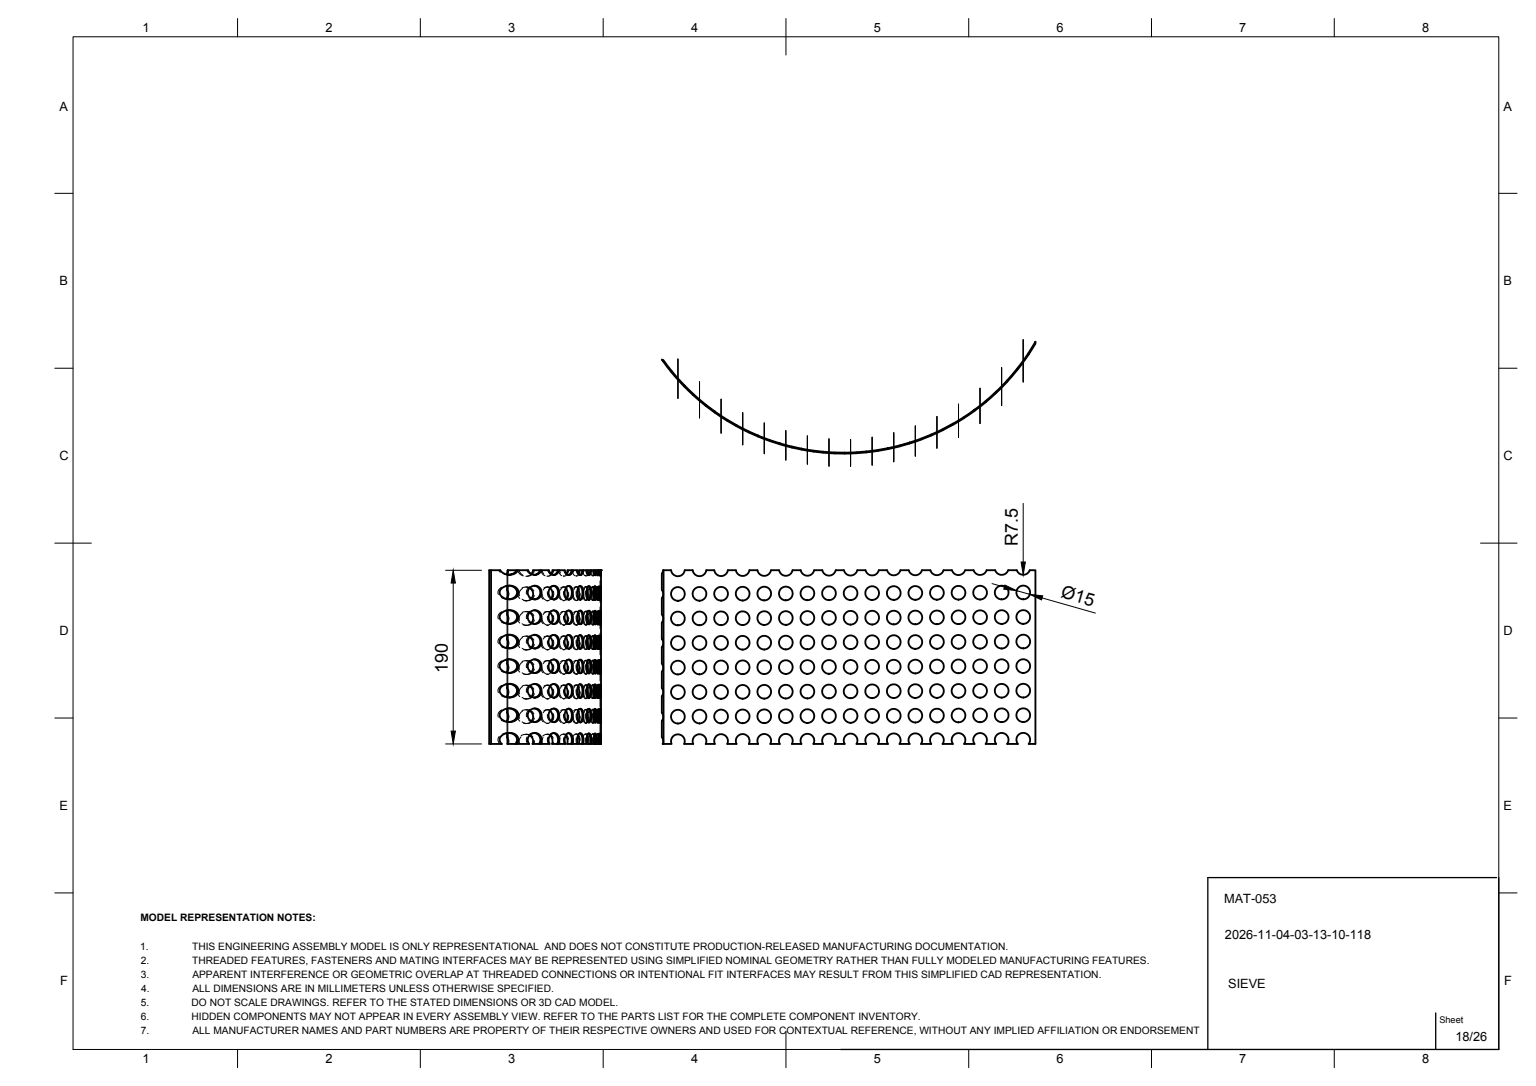
ISO-10303-21;
HEADER;
FILE_DESCRIPTION (('STEP AP214'),
    '1' );
FILE_NAME ('SIEVE.step',
    '2026-10-10T03:43:58',
    ( '' ),
    ( '' ),
    'SwSTEP 2.0',
    'SolidWorks 2026',
    '' );
FILE_SCHEMA (( 'AUTOMOTIVE_DESIGN' ));
ENDSEC;

DATA;
#1=CARTESIAN_POINT ( 'NONE',  ( 39.40195752203892710, -170.0000000000000000, -43.11981746542777927 ) ) ;
#3=EDGE_LOOP ( 'NONE', ( #61802, #31194, #2413, #55543 ) ) ;
#7=CARTESIAN_POINT ( 'NONE',  ( 157.4703587214989113, 58.92748579479261650, -51.12418429913766005 ) ) ;
#8=CARTESIAN_POINT ( 'NONE',  ( 66.29961816943398389, 13.45804302849872869, 30.55285179693984432 ) ) ;
#10=ADVANCED_FACE ( 'NONE', ( #11603 ), #16546, .F. ) ;
#11=CARTESIAN_POINT ( 'NONE',  ( -189.2739965869454579, 107.1373753350176656, -69.83507040438288982 ) ) ;
#12=EDGE_CURVE ( 'NONE', #54401, #54282, #16885, .T. ) ;
#15=CARTESIAN_POINT ( 'NONE',  ( -95.04120270830171080, 29.25306318840327791, 66.89222559579708616 ) ) ;
#20=CARTESIAN_POINT ( 'NONE',  ( -124.1095621208148572, 46.52671329146387080, 18.61778521462535352 ) ) ;
#21=AXIS2_PLACEMENT_3D ( 'NONE', #6201, #49094, #933 ) ;
#22=CARTESIAN_POINT ( 'NONE',  ( -173.9548930713590380, 88.06040582145359963, 57.70099677511350933 ) ) ;
#23=CARTESIAN_POINT ( 'NONE',  ( 15.78827728214693416, 6.500811158483328356, 18.17015708224157322 ) ) ;
#24=ORIENTED_EDGE ( 'NONE', *, *, #58760, .T. ) ;
#25=CARTESIAN_POINT ( 'NONE',  ( -24.85653282846401879, 8.603185326828743484, 94.99999999999866418 ) ) ;
#26=CARTESIAN_POINT ( 'NONE',  ( 156.5909039492010209, 56.96742803863246962, 44.40946747225338953 ) ) ;
#27=CARTESIAN_POINT ( 'NONE',  ( 70.12389542974193546, 15.47520081968151651, 34.86987470614429441 ) ) ;
#30=DIRECTION ( 'NONE',  ( -0.000000000000000000, 1.000000000000000000, -0.000000000000000000 ) ) ;
#31=CARTESIAN_POINT ( 'NONE',  ( -23.93880457192868860, 8.479983864459173404, 37.95612845895288956 ) ) ;
#32=CARTESIAN_POINT ( 'NONE',  ( -142.0084862216822614, 59.34995487985342066, -68.57895708802404044 ) ) ;
#33=ORIENTED_EDGE ( 'NONE', *, *, #68760, .T. ) ;
#35=FACE_BOUND ( 'NONE', #6574, .T. ) ;
#37=CARTESIAN_POINT ( 'NONE',  ( -180.0154536325057677, 96.73346874014741559, 68.13326579958136620 ) ) ;
#38=CARTESIAN_POINT ( 'NONE',  ( 110.2429982417149432, 28.88204397445230853, -89.61153874658103291 ) ) ;
#39=CARTESIAN_POINT ( 'NONE',  ( 133.8566784816069344, 41.42467568809808398, 29.51034083899533300 ) ) ;
#43=CARTESIAN_POINT ( 'NONE',  ( -78.66644367742111399, 22.32174330031318732, -88.80455181264524356 ) ) ;
#44=CARTESIAN_POINT ( 'NONE',  ( 70.02892116572940040, 14.40944430928136377, 13.13782541409767646 ) ) ;
#45=CARTESIAN_POINT ( 'NONE',  ( 161.7048274740120917, 61.01946783654758377, 3.857278696179094801 ) ) ;
#46=CARTESIAN_POINT ( 'NONE',  ( 92.21252738308859875, 22.47457138983956426, -21.50906452630309929 ) ) ;
#48=EDGE_CURVE ( 'NONE', #37583, #44986, #40434, .T. ) ;
#53=CARTESIAN_POINT ( 'NONE',  ( -125.8938041572051105, 46.49392987655495091, 45.61994787315711619 ) ) ;
#54=CARTESIAN_POINT ( 'NONE',  ( 114.5134543485688710, 32.02763527597250715, 84.62599922377962969 ) ) ;
#55=CARTESIAN_POINT ( 'NONE',  ( 39.40195752203891999, 9.424259417798147354, -8.775266874964067654 ) ) ;
#56=CARTESIAN_POINT ( 'NONE',  ( 66.73594759725092729, 13.56641407806656829, -9.859353299932527293 ) ) ;
#58=CARTESIAN_POINT ( 'NONE',  ( 135.6793972494602656, 43.71805072851429941, -50.81300272974607424 ) ) ;
#60=CARTESIAN_POINT ( 'NONE',  ( 208.3163574534978295, 113.2160455531247152, -90.93580564839912483 ) ) ;
#62=CARTESIAN_POINT ( 'NONE',  ( -125.8938041572051389, -170.0000000000000000, -96.10280507916131398 ) ) ;
#65=EDGE_CURVE ( 'NONE', #33282, #48266, #62999, .T. ) ;
#66=CARTESIAN_POINT ( 'NONE',  ( 35.66087318222937341, 8.964867769223225480, 57.73931627539139555 ) ) ;
#67=VECTOR ( 'NONE', #58761, 1000.000000000000000 ) ;
#68=CARTESIAN_POINT ( 'NONE',  ( 178.1321887506117889, 77.08201292995904907, 83.59636689041089141 ) ) ;
#69=DIRECTION ( 'NONE',  ( -0.000000000000000000, 1.000000000000000000, -0.000000000000000000 ) ) ;
#70=EDGE_CURVE ( 'NONE', #25573, #51909, #66497, .T. ) ;
#71=B_SPLINE_CURVE_WITH_KNOTS ( 'NONE', 3,
 ( #62149, #40352, #67112, #40690, #61801, #51606, #19236, #61465, #13288, #2379, #13619, #2725 ),
 .UNSPECIFIED., .F., .F.,
 ( 4, 2, 2, 2, 2, 4 ),
 ( 0.01013073868447747147, 0.01266158667236432465, 0.01519243466025117784, 0.01645785865419460356, 0.01772328264813802928, 0.02025413063602488073 ),
 .UNSPECIFIED. ) ;
#75=CARTESIAN_POINT ( 'NONE',  ( 70.16127872101215246, 15.48516972826856097, -94.59315289484993627 ) ) ;
#78=CARTESIAN_POINT ( 'NONE',  ( 188.5653887627528036, 88.01608521313129074, -17.48984807395640573 ) ) ;
#79=CARTESIAN_POINT ( 'NONE',  ( -82.93267503967653909, 23.99263498936122829, -9.597822780125905950 ) ) ;
#82=CARTESIAN_POINT ( 'NONE',  ( 157.4703587214989398, 58.92748579479258808, 17.56491688178971700 ) ) ;
#83=LINE ( 'NONE', #53188, #15134 ) ;
#84=CYLINDRICAL_SURFACE ( 'NONE', #8226, 7.500000000000020428 ) ;
#85=CARTESIAN_POINT ( 'NONE',  ( 164.6598737201887275, 64.78038692612516058, 61.54778376556991759 ) ) ;
#87=CARTESIAN_POINT ( 'NONE',  ( -190.6985136298601731, 109.1272424661242582, -95.00000000000133582 ) ) ;
#88=CARTESIAN_POINT ( 'NONE',  ( 91.11019107624156277, 22.06959540317787827, -37.30231510556647123 ) ) ;
#89=CARTESIAN_POINT ( 'NONE',  ( 152.8373718734504791, 55.38925997611393370, 69.67201452546140672 ) ) ;
#90=FACE_OUTER_BOUND ( 'NONE', #51593, .T. ) ;
#92=CARTESIAN_POINT ( 'NONE',  ( -10.98306470837134796, 8.126405184847016017, 84.49408135793621000 ) ) ;
#101=CARTESIAN_POINT ( 'NONE',  ( 88.52077179907878701, 21.14145351760140557, -62.90458105059150284 ) ) ;
#103=CARTESIAN_POINT ( 'NONE',  ( -55.05276343752909440, 14.68156374112638929, -77.06087458892358200 ) ) ;
#105=CARTESIAN_POINT ( 'NONE',  ( 32.29989959354725926, 7.591763852038291738, -13.85219865116375715 ) ) ;
#106=CARTESIAN_POINT ( 'NONE',  ( 179.4227152810058215, 78.36166152262364903, -51.05095273083168905 ) ) ;
#107=CARTESIAN_POINT ( 'NONE',  ( 163.7460705099150573, 62.69983247170010543, 94.71987145728411406 ) ) ;
#108=CARTESIAN_POINT ( 'NONE',  ( 93.85846834761630930, 22.01563781856521018, 35.19885710929750644 ) ) ;
#110=ORIENTED_EDGE ( 'NONE', *, *, #20958, .T. ) ;
#113=CARTESIAN_POINT ( 'NONE',  ( -52.68206656346369954, 15.09776187114412593, -35.59673745022761437 ) ) ;
#114=CARTESIAN_POINT ( 'NONE',  ( -78.66644367742111399, 23.39876645725287219, 30.41820113967310490 ) ) ;
#115=CARTESIAN_POINT ( 'NONE',  ( 8.683910719548897816, 7.383368463746306176, 35.09835667283063998 ) ) ;
#119=ORIENTED_EDGE ( 'NONE', *, *, #42370, .F. ) ;
#122=CARTESIAN_POINT ( 'NONE',  ( -8.314575874103555364, 6.922894809783093351, -23.57352014148017361 ) ) ;
#123=CARTESIAN_POINT ( 'NONE',  ( -50.51700111023804851, 13.51182830536852997, 43.81040306015482599 ) ) ;
#125=DIRECTION ( 'NONE',  ( 0.000000000000000000, 0.000000000000000000, 1.000000000000000000 ) ) ;
#127=CARTESIAN_POINT ( 'NONE',  ( -38.16652041892307778, 11.81761816422915068, 61.20925241452948740 ) ) ;
#129=CARTESIAN_POINT ( 'NONE',  ( -13.47517652744366856, 8.334971000693553123, -11.11675483260547104 ) ) ;
#130=CARTESIAN_POINT ( 'NONE',  ( 150.0973882686025433, 52.13852366454154463, -69.06737236800162805 ) ) ;
#131=CARTESIAN_POINT ( 'NONE',  ( 15.78827728214693416, 6.500811158483328356, -8.674393508222097537 ) ) ;
#134=CARTESIAN_POINT ( 'NONE',  ( -154.7998111145352595, 68.80117179139330119, -47.64861779563037203 ) ) ;
#136=EDGE_LOOP ( 'NONE', ( #56580, #33322, #40120, #29529 ) ) ;
#137=CARTESIAN_POINT ( 'NONE',  ( 69.49112875363887554, 15.30845942322122433, -20.16820370593556433 ) ) ;
#138=EDGE_CURVE ( 'NONE', #47203, #54495, #17035, .T. ) ;
#139=CARTESIAN_POINT ( 'NONE',  ( -82.93126516400695891, 25.07709093823493873, -48.78959211302295529 ) ) ;
#140=DIRECTION ( 'NONE',  ( 0.000000000000000000, 0.000000000000000000, 1.000000000000000000 ) ) ;
#141=CARTESIAN_POINT ( 'NONE',  ( -156.9900125991010498, 72.16580261738670288, 10.78960814776965549 ) ) ;
#142=CARTESIAN_POINT ( 'NONE',  ( 187.2465631085773907, 85.06582225041681511, -39.42042871992538267 ) ) ;
#144=CARTESIAN_POINT ( 'NONE',  ( -156.4614183966801022, 71.67647641794694380, 89.09562039624624674 ) ) ;
#145=VERTEX_POINT ( 'NONE', #21389 ) ;
#147=EDGE_LOOP ( 'NONE', ( #11378, #55449, #7164, #22820 ) ) ;
#148=CARTESIAN_POINT ( 'NONE',  ( -156.0209085498132140, 71.27066046086522988, -19.22534495811094146 ) ) ;
#149=CARTESIAN_POINT ( 'NONE',  ( 87.02964419696034781, 20.62171628682589386, -89.51066537983909654 ) ) ;
#153=CARTESIAN_POINT ( 'NONE',  ( -33.83558513595455253, 9.996963989836508802, 71.67202419627825805 ) ) ;
#154=CARTESIAN_POINT ( 'NONE',  ( -150.3791492925491013, 64.92185203933371440, -22.93029560069632211 ) ) ;
#156=CARTESIAN_POINT ( 'NONE',  ( 187.0788993276711665, 86.37277723143233743, 59.13935664661273250 ) ) ;
#157=CARTESIAN_POINT ( 'NONE',  ( -155.1302201283146758, 69.09929365814132041, 70.03478143350771745 ) ) ;
#159=CARTESIAN_POINT ( 'NONE',  ( 16.28382582968306380, 7.523443033994204221, 18.17015708224156612 ) ) ;
#160=CARTESIAN_POINT ( 'NONE',  ( 104.7147873368644753, 26.40702926859708199, 15.35902160271893813 ) ) ;
#161=CARTESIAN_POINT ( 'NONE',  ( -124.9927180788553756, 45.90286323198618845, 18.73480619198342367 ) ) ;
#163=CARTESIAN_POINT ( 'NONE',  ( 21.25987915030395925, 6.737472588634914494, 59.22395766586208055 ) ) ;
#165=CARTESIAN_POINT ( 'NONE',  ( 8.336882341125875229, 6.376438415325264231, -70.84698747820850429 ) ) ;
#168=VERTEX_POINT ( 'NONE', #37218 ) ;
#173=CARTESIAN_POINT ( 'NONE',  ( 218.0000000000000000, 0.000000000000000000, 0.000000000000000000 ) ) ;
#174=CARTESIAN_POINT ( 'NONE',  ( 44.34263167748003553, 9.103379693481556956, -75.62813062877941661 ) ) ;
#176=EDGE_LOOP ( 'NONE', ( #13726, #7536, #23044, #10848 ) ) ;
#177=ORIENTED_EDGE ( 'NONE', *, *, #64499, .T. ) ;
#178=CARTESIAN_POINT ( 'NONE',  ( -25.48237668717799309, 8.689083390666777262, -11.38912287515594812 ) ) ;
#179=CARTESIAN_POINT ( 'NONE',  ( 174.1688711713896964, 71.88855623114105242, 93.40745146404465515 ) ) ;
#182=CARTESIAN_POINT ( 'NONE',  ( 116.0773578185793582, 31.67580513411752463, 59.21665166914974776 ) ) ;
#184=CARTESIAN_POINT ( 'NONE',  ( 115.0485321076020568, 32.28990710985444679, 69.73487632334627051 ) ) ;
#186=CARTESIAN_POINT ( 'NONE',  ( 140.2058232509808704, 46.59155168125935376, 67.87841396662895477 ) ) ;
#188=CARTESIAN_POINT ( 'NONE',  ( -98.46684543088103680, 30.88557736720387936, 44.48182062113936297 ) ) ;
#189=CARTESIAN_POINT ( 'NONE',  ( 88.98408042523108463, 20.23787745328938570, -50.44636354873872364 ) ) ;
#191=ORIENTED_EDGE ( 'NONE', *, *, #28368, .T. ) ;
#197=CARTESIAN_POINT ( 'NONE',  ( -165.7690020878297616, 80.74028011998674970, -70.56799682258439077 ) ) ;
#198=CARTESIAN_POINT ( 'NONE',  ( -142.0251973982164202, 58.08401473564112649, -42.89990999809938188 ) ) ;
#199=ORIENTED_EDGE ( 'NONE', *, *, #29609, .T. ) ;
#208=CARTESIAN_POINT ( 'NONE',  ( 79.19345177405116942, 17.01649702043280143, -15.46643930101046038 ) ) ;
#209=CARTESIAN_POINT ( 'NONE',  ( 93.71772995179813392, 21.96265635001558181, -67.70285364061378175 ) ) ;
#210=CARTESIAN_POINT ( 'NONE',  ( 60.43099056502398980, 12.08801636090767850, -89.86627097950946563 ) ) ;
#212=CARTESIAN_POINT ( 'NONE',  ( -98.69283175933881580, 30.99524616306738878, 4.570732717346438712 ) ) ;
#213=CARTESIAN_POINT ( 'NONE',  ( -95.63568360745009045, 29.53168204475774417, -72.84711776369148595 ) ) ;
#217=ADVANCED_FACE ( 'NONE', ( #3847 ), #69303, .F. ) ;
#218=CARTESIAN_POINT ( 'NONE',  ( 188.2133404574783242, 86.12414067617878288, -68.22339036842659254 ) ) ;
#219=VECTOR ( 'NONE', #12666, 1000.000000000000000 ) ;
#224=CARTESIAN_POINT ( 'NONE',  ( 79.23200707685336397, 17.02828389812517429, 38.47447533467553171 ) ) ;
#226=CARTESIAN_POINT ( 'NONE',  ( -124.1007047332777944, 46.52282960291164926, 30.82329275154649295 ) ) ;
#227=CARTESIAN_POINT ( 'NONE',  ( 211.1200456646897123, 115.5868795682033436, 67.43584021203363932 ) ) ;
#231=CARTESIAN_POINT ( 'NONE',  ( -14.76369756425703983, 7.442560416198673146, -40.03899903455366882 ) ) ;
#233=CARTESIAN_POINT ( 'NONE',  ( 89.87840278991589571, 21.62393877508911899, 57.29260026085291457 ) ) ;
#235=CARTESIAN_POINT ( 'NONE',  ( 150.0433793199863146, 52.09973307442953683, -17.85989976896762244 ) ) ;
#236=CARTESIAN_POINT ( 'NONE',  ( 31.96192885395475614, 8.569232728322420556, 11.54728592230744688 ) ) ;
#237=CARTESIAN_POINT ( 'NONE',  ( -94.77890319529970498, 30.24118571794803145, -69.85920485586603945 ) ) ;
#243=CARTESIAN_POINT ( 'NONE',  ( 60.63380853769237433, 13.16344960520422092, 57.04161213523420315 ) ) ;
#245=CARTESIAN_POINT ( 'NONE',  ( -9.524904342798460988, 8.016391612076530393, 3.461975196507860453 ) ) ;
#246=B_SPLINE_CURVE_WITH_KNOTS ( 'NONE', 3,
 ( #24990, #25339, #47115, #47446, #36574, #58023, #9495, #14429, #20379, #68579, #26018, #52401, #25686, #36915, #46776, #68907, #62260, #42187, #63654, #14763, #4219, #36227, #52729, #30264, #15462, #41848, #9150, #30605, #9841, #46080, #14077, #8811, #4554, #29912, #62955, #67550, #35539, #52058, #68246, #56993, #8460, #20051, #41504, #51371, #3188, #24647, #19349, #57685, #51713, #46422 ),
 .UNSPECIFIED., .F., .F.,
 ( 4, 2, 2, 2, 2, 2, 2, 2, 2, 2, 2, 2, 2, 2, 2, 2, 2, 2, 2, 2, 2, 2, 2, 2, 4 ),
 ( 0.02688458561150007531, 0.02770990876165290578, 0.02853523191180573973, 0.03018587821211139027, 0.03183652451241704429, 0.03266184766256987476, 0.03348717081272270524, 0.03513781711302831068, 0.03678846341333391612, 0.03761378656348669802, 0.03843910971363948686, 0.03926443286379226877, 0.04008975601394505761, 0.04174040231425062836, 0.04256572546440341026, 0.04339104861455619216, 0.04421637176470897407, 0.04504169491486175597, 0.04586701806501453788, 0.04669234121516731978, 0.04834298751547294604, 0.04916831066562572794, 0.04999363381577851678, 0.05164428011608407365, 0.05329492641638964440 ),
 .UNSPECIFIED. ) ;
#248=CARTESIAN_POINT ( 'NONE',  ( -3.857727530059799737, 6.665032499723453796, 43.98489318319101926 ) ) ;
#250=CARTESIAN_POINT ( 'NONE',  ( 92.81046075878417412, 22.69711000191779959, 86.64015653787805604 ) ) ;
#256=CARTESIAN_POINT ( 'NONE',  ( -104.1393288135077455, 34.86912007524090029, 72.14469141808412189 ) ) ;
#258=CARTESIAN_POINT ( 'NONE',  ( -131.6253556217205016, 51.61436399519948282, -47.27706506024894395 ) ) ;
#262=B_SPLINE_CURVE_WITH_KNOTS ( 'NONE', 3,
 ( #59638, #61313, #13475, #23684, #67303, #64945, #7519, #45827, #34603, #2920, #19089, #8197, #59303, #16738, #39855, #45475, #23348, #40208, #56375, #13139, #2235, #38197, #11115, #12783, #11452, #571, #34245, #7855, #60962, #44791, #54360, #29302, #28970, #1895, #29646, #32580, #50755, #2576 ),
 .UNSPECIFIED., .F., .F.,
 ( 4, 2, 2, 2, 2, 2, 2, 2, 2, 2, 2, 2, 2, 2, 2, 2, 2, 2, 4 ),
 ( 1.430489624538199204E-17, 0.003908178031105532212, 0.005862267046658249312, 0.007816356062210967279, 0.009770445077763688715, 0.01172453409331640842, 0.01270157860109274485, 0.01367862310886907781, 0.01465566761664541424, 0.01563271212442174721, 0.01660975663219808884, 0.01758680113997443048, 0.01954089015552709294, 0.02051793466330344151, 0.02149497917107979009, 0.02344906818663248377, 0.02540315720218518786, 0.02735724621773788501, 0.03126542424884325155 ),
 .UNSPECIFIED. ) ;
#263=CARTESIAN_POINT ( 'NONE',  ( -1.088326810997878091, 6.545818265928947888, -19.40564166976581006 ) ) ;
#266=CARTESIAN_POINT ( 'NONE',  ( -153.9421172888672231, 68.03407102037994036, 85.85448269280857403 ) ) ;
#268=CARTESIAN_POINT ( 'NONE',  ( 141.3445468829085030, 46.13338528906589886, 37.51412908544414648 ) ) ;
#271=CARTESIAN_POINT ( 'NONE',  ( 82.73618382051373032, 19.18661415186669217, 16.78260538844248728 ) ) ;
#272=CARTESIAN_POINT ( 'NONE',  ( 164.4761273435911733, 64.62485394454745347, 7.335242511255203546 ) ) ;
#274=AXIS2_PLACEMENT_3D ( 'NONE', #4193, #20028, #68878 ) ;
#275=VERTEX_POINT ( 'NONE', #57999 ) ;
#276=EDGE_CURVE ( 'NONE', #33643, #59523, #9303, .T. ) ;
#277=CARTESIAN_POINT ( 'NONE',  ( 174.9099402067542997, 73.96774984027638311, 67.91937322613915740 ) ) ;
#279=CARTESIAN_POINT ( 'NONE',  ( -104.5730787903383003, 33.96058035148152499, -35.35797728948608665 ) ) ;
#281=CARTESIAN_POINT ( 'NONE',  ( 150.4542242713869200, 53.63744268572192198, 12.72894179764149847 ) ) ;
#282=ORIENTED_EDGE ( 'NONE', *, *, #4760, .T. ) ;
#283=CARTESIAN_POINT ( 'NONE',  ( 157.4703587214989113, 57.65129005721576760, 29.40946747225336466 ) ) ;
#285=CYLINDRICAL_SURFACE ( 'NONE', #42881, 7.500000000000020428 ) ;
#286=ORIENTED_EDGE ( 'NONE', *, *, #5924, .T. ) ;
#292=CARTESIAN_POINT ( 'NONE',  ( -37.79823708645147917, 10.72197716414928870, -73.64561661794576253 ) ) ;
#302=DIRECTION ( 'NONE',  ( -0.000000000000000000, 1.000000000000000000, -0.000000000000000000 ) ) ;
#303=CARTESIAN_POINT ( 'NONE',  ( 70.49702515974807682, 14.53327724265703402, 91.86127284075526234 ) ) ;
#307=CYLINDRICAL_SURFACE ( 'NONE', #24291, 7.500000000000013323 ) ;
#311=AXIS2_PLACEMENT_3D ( 'NONE', #60560, #44374, #50365 ) ;
#312=CARTESIAN_POINT ( 'NONE',  ( 211.5066273949820186, 116.1727691518062073, -73.86407362358771422 ) ) ;
#313=B_SPLINE_CURVE_WITH_KNOTS ( 'NONE', 3,
 ( #22788, #6611, #12241, #1333, #32645, #43534, #50221, #60425, #55133, #1685, #44592, #50913, #45283, #9047, #13622, #19590, #7670, #2728, #34407, #66764, #61804, #18557, #55849, #61471, #62513, #3420, #35784, #41053, #18214, #24879, #2383, #14325, #29453, #29115, #40694, #57233, #40009, #13291, #30495, #29808, #39665, #46316, #50565, #44937 ),
 .UNSPECIFIED., .F., .F.,
 ( 4, 2, 2, 2, 2, 2, 2, 2, 2, 2, 2, 2, 2, 2, 2, 2, 2, 2, 2, 2, 2, 4 ),
 ( 0.02895403260893131964, 0.03071603688922221187, 0.03247804116951310410, 0.03424004544980399634, 0.03600204973009488857, 0.03776405401038577386, 0.03864505615053119569, 0.03952605829067662446, 0.04040706043082205323, 0.04128806257096747506, 0.04216906471111290383, 0.04305006685125832566, 0.04393106899140375443, 0.04481207113154918320, 0.04569307327169461197, 0.04657407541184004074, 0.04745507755198546257, 0.04833607969213089134, 0.05009808397242175582, 0.05186008825271262723, 0.05362209253300349171, 0.05714610109358524842 ),
 .UNSPECIFIED. ) ;
#316=CARTESIAN_POINT ( 'NONE',  ( 63.01563776193091826, -170.0000000000000000, -89.40979201309708913 ) ) ;
#317=CARTESIAN_POINT ( 'NONE',  ( -124.1095621208148714, 46.52671329146387791, 72.30688639555273767 ) ) ;
#318=CARTESIAN_POINT ( 'NONE',  ( 22.62427395637551086, 7.823784829753564374, 34.41962451814575275 ) ) ;
#326=FACE_OUTER_BOUND ( 'NONE', #64859, .T. ) ;
#328=ORIENTED_EDGE ( 'NONE', *, *, #4703, .T. ) ;
#331=CARTESIAN_POINT ( 'NONE',  ( 46.85361596800672146, 10.51535167202354693, 38.39853853478529544 ) ) ;
#332=CARTESIAN_POINT ( 'NONE',  ( -27.70562707895080123, 9.007984652865424380, 58.03756985863584106 ) ) ;
#333=CARTESIAN_POINT ( 'NONE',  ( -142.3393481102175713, 58.33014244976924090, 9.152932767281312110 ) ) ;
#335=ORIENTED_EDGE ( 'NONE', *, *, #3794, .F. ) ;
#336=CARTESIAN_POINT ( 'NONE',  ( -127.6881387055492354, 48.89937523111242257, 30.83417093567260636 ) ) ;
#340=CARTESIAN_POINT ( 'NONE',  ( 55.61382797299289393, 11.07686102552912644, 62.92265474384031876 ) ) ;
#342=CARTESIAN_POINT ( 'NONE',  ( -29.96307832726302678, 10.37242130382201921, -89.14992242554669133 ) ) ;
#343=CARTESIAN_POINT ( 'NONE',  ( -188.8754233303960746, 108.3048424661242137, -95.00000000000133582 ) ) ;
#347=VERTEX_POINT ( 'NONE', #65712 ) ;
#350=VECTOR ( 'NONE', #31052, 1000.000000000000000 ) ;
#353=CARTESIAN_POINT ( 'NONE',  ( 70.26722489419890394, 14.47234958177329567, 35.33543539248424281 ) ) ;
#355=ORIENTED_EDGE ( 'NONE', *, *, #33274, .T. ) ;
#358=CARTESIAN_POINT ( 'NONE',  ( 80.30232379693107703, 17.35837133860831472, 6.332652209273762267 ) ) ;
#361=CARTESIAN_POINT ( 'NONE',  ( -71.97434903038468690, 19.88430675376529067, 34.49547489334918993 ) ) ;
#362=ORIENTED_EDGE ( 'NONE', *, *, #55841, .F. ) ;
#364=VECTOR ( 'NONE', #18440, 1000.000000000000000 ) ;
#368=CARTESIAN_POINT ( 'NONE',  ( -179.5178913137217194, 94.54206947403389449, 69.12039320224292283 ) ) ;
#370=ORIENTED_EDGE ( 'NONE', *, *, #14642, .F. ) ;
#374=DIRECTION ( 'NONE',  ( -0.000000000000000000, 1.000000000000000000, -0.000000000000000000 ) ) ;
#375=CARTESIAN_POINT ( 'NONE',  ( 150.9184679586219033, 52.73111408630721542, 40.56872817287094790 ) ) ;
#376=CARTESIAN_POINT ( 'NONE',  ( 68.63585058221465829, 15.08566240483130727, 32.32217050974968942 ) ) ;
#381=CARTESIAN_POINT ( 'NONE',  ( -23.95096213915836358, 8.481591526885939203, 38.20520003450658209 ) ) ;
#382=CARTESIAN_POINT ( 'NONE',  ( -144.7530445311634537, 61.54314312182906122, -74.96293479194935117 ) ) ;
#384=FACE_BOUND ( 'NONE', #4499, .T. ) ;
#385=CARTESIAN_POINT ( 'NONE',  ( -2.190131154568200511, 6.589492063460817839, -74.71788358249716566 ) ) ;
#386=CARTESIAN_POINT ( 'NONE',  ( -179.8926034784145997, 96.58272071140105197, 61.93007157060646506 ) ) ;
#388=CARTESIAN_POINT ( 'NONE',  ( -118.9668643994983483, 43.27909474462860828, -39.52642719331304022 ) ) ;
#389=CARTESIAN_POINT ( 'NONE',  ( -85.66184035008926401, 26.20110535976566268, 13.79000864225666589 ) ) ;
#392=CARTESIAN_POINT ( 'NONE',  ( -5.888165822225391643, 7.780336669456525023, -8.823856489658712832 ) ) ;
#393=CARTESIAN_POINT ( 'NONE',  ( 67.55134213333077753, 13.77030723107740506, 4.475137186144926282 ) ) ;
#394=CARTESIAN_POINT ( 'NONE',  ( 159.6593397521790791, 59.37286298965126718, 2.877594456964315039 ) ) ;
#395=CARTESIAN_POINT ( 'NONE',  ( 39.81822037269075309, 9.478622457786777034, -89.30891864635511013 ) ) ;
#398=CARTESIAN_POINT ( 'NONE',  ( -38.54712373114178092, 11.89174538567466932, 8.428869490921766072 ) ) ;
#399=ORIENTED_EDGE ( 'NONE', *, *, #56528, .T. ) ;
#402=CARTESIAN_POINT ( 'NONE',  ( 85.67165909753201447, 20.15791549876375655, -62.71191053415395089 ) ) ;
#404=CARTESIAN_POINT ( 'NONE',  ( 110.9260829236403936, 30.30898941444543837, 83.30420403083246583 ) ) ;
#405=CARTESIAN_POINT ( 'NONE',  ( -142.0084862216822330, 59.34995487985343487, 65.64379586429438973 ) ) ;
#406=CARTESIAN_POINT ( 'NONE',  ( 70.25990036603482736, 14.47042233282419765, -14.41847716369608001 ) ) ;
#409=CARTESIAN_POINT ( 'NONE',  ( -31.43908319763710679, 10.61114334766715928, -35.31719736520183517 ) ) ;
#410=CARTESIAN_POINT ( 'NONE',  ( -53.14657859411972396, 15.21831473227210196, -62.30310801584961666 ) ) ;
#413=EDGE_CURVE ( 'NONE', #65743, #4867, #71, .T. ) ;
#414=CARTESIAN_POINT ( 'NONE',  ( -118.4106078162223668, 42.93830006159888768, -14.99940221450364319 ) ) ;
#415=ORIENTED_EDGE ( 'NONE', *, *, #36605, .F. ) ;
#419=CARTESIAN_POINT ( 'NONE',  ( 33.31166872005967150, 8.707041209322234465, 59.87445300413067173 ) ) ;
#420=DIRECTION ( 'NONE',  ( -0.8118923937861950435, -0.5838071093367415143, 0.000000000000000000 ) ) ;
#422=CARTESIAN_POINT ( 'NONE',  ( -172.3038663181180823, 87.72015621195184565, -7.867406574286301080 ) ) ;
#427=CARTESIAN_POINT ( 'NONE',  ( 187.2296622856351860, 86.53808614709454616, -21.18754879403664404 ) ) ;
#428=CARTESIAN_POINT ( 'NONE',  ( 212.1669304543882788, 119.0398299474539243, 9.162465270872496959 ) ) ;
#432=CARTESIAN_POINT ( 'NONE',  ( -149.5074843970971301, 64.17983161892345834, -76.65738112195568021 ) ) ;
#439=CARTESIAN_POINT ( 'NONE',  ( -47.94536219817735656, 13.92422159065987408, 62.21613247434213179 ) ) ;
#441=CYLINDRICAL_SURFACE ( 'NONE', #8272, 7.500000000000013323 ) ;
#442=DIRECTION ( 'NONE',  ( -0.000000000000000000, 1.000000000000000000, -0.000000000000000000 ) ) ;
#443=B_SPLINE_CURVE_WITH_KNOTS ( 'NONE', 3,
 ( #41840, #54634, #27027, #15107, #63647, #41496, #62947, #36907, #10161, #9488, #16130, #30946, #14755, #4211, #4546, #53400, #25676, #4886, #47438, #68897, #47107, #68570, #47789, #42521, #63298, #15455, #36566, #20724, #31293, #26353, #52719, #58345, #5235, #53749, #63976, #9834, #21078, #15790, #26011, #42179, #37233, #69251, #58684 ),
 .UNSPECIFIED., .F., .F.,
 ( 4, 2, 2, 2, 2, 2, 2, 2, 2, 2, 2, 1, 2, 2, 2, 2, 2, 2, 2, 2, 2, 4 ),
 ( 0.02515559250233022348, 0.02674001423437969566, 0.02753222510040442828, 0.02832443596642916436, 0.02990885769847856715, 0.03149327943052796647, 0.03307770116257736925, 0.03386991202860207412, 0.03466212289462677898, 0.03624654462667613319, 0.03703875549270080336, 0.03783096635872546659, 0.03862317722475013676, 0.03941538809077479999, 0.04099980982282412645, 0.04258423155487345985, 0.04337644242089812308, 0.04416865328692278631, 0.04575307501897205031, 0.04733749675102130738, 0.04892191848307056445, 0.05050634021511982846 ),
 .UNSPECIFIED. ) ;
#445=CARTESIAN_POINT ( 'NONE',  ( 62.53328835682435738, 12.56090025569836932, 2.968410348757586803 ) ) ;
#446=CARTESIAN_POINT ( 'NONE',  ( -58.10608953386396536, 15.52134062643864176, 57.80724698423686903 ) ) ;
#448=EDGE_LOOP ( 'NONE', ( #53193, #25137, #33362, #38103 ) ) ;
#449=EDGE_CURVE ( 'NONE', #11991, #8386, #8441, .T. ) ;
#453=CARTESIAN_POINT ( 'NONE',  ( 91.11019107624153435, 22.06959540317787116, -64.14686569603014732 ) ) ;
#457=CARTESIAN_POINT ( 'NONE',  ( 35.44781468922820977, 7.928097401423690016, -22.65291149958800432 ) ) ;
#458=CARTESIAN_POINT ( 'NONE',  ( 173.8576514579035290, 72.97529922124003576, -41.69686196060180094 ) ) ;
#459=CARTESIAN_POINT ( 'NONE',  ( 158.7623625177564008, 58.66148101564576223, 83.18577911345145992 ) ) ;
#464=ORIENTED_EDGE ( 'NONE', *, *, #60521, .F. ) ;
#466=CARTESIAN_POINT ( 'NONE',  ( -51.34542473642584071, 14.75635007918829800, -49.24053308027907860 ) ) ;
#470=CARTESIAN_POINT ( 'NONE',  ( 13.83281508467570653, 7.452090093180185448, 44.77217603759554265 ) ) ;
#479=CARTESIAN_POINT ( 'NONE',  ( -14.32120159453990027, 7.401444311907543039, -19.83056408198577003 ) ) ;
#480=CARTESIAN_POINT ( 'NONE',  ( -49.11825192196926082, 13.17012322555986970, 42.42977472503392988 ) ) ;
#484=CARTESIAN_POINT ( 'NONE',  ( -31.93169728792083362, 10.69234447276976852, 72.06100499665291181 ) ) ;
#485=CARTESIAN_POINT ( 'NONE',  ( -15.32584732649904247, 8.506915958926388299, -15.58511460959460315 ) ) ;
#486=CARTESIAN_POINT ( 'NONE',  ( 152.8430172091323698, 54.14068524174424368, -76.37591427044367265 ) ) ;
#487=CARTESIAN_POINT ( 'NONE',  ( 16.28371206594635368, 6.516665886438622657, -8.674393508222101090 ) ) ;
#490=ORIENTED_EDGE ( 'NONE', *, *, #33090, .F. ) ;
#495=CARTESIAN_POINT ( 'NONE',  ( 110.2429982417149574, 29.99119854320843714, -9.077886975189997543 ) ) ;
#502=B_SPLINE_CURVE_WITH_KNOTS ( 'NONE', 3,
 ( #8600, #68036, #40941, #9632, #31090, #57466, #24771, #51838, #62400, #25125, #24434, #68374, #3652, #67689, #40590, #46555, #46208, #58156, #9974, #30049, #19479, #31425, #41631, #52186, #41293, #62751, #57127, #35321, #14553, #52530, #68700, #19136, #2972, #8939, #19836, #9276, #47243, #4353, #56781, #45874, #67345, #51509, #4005 ),
 .UNSPECIFIED., .F., .F.,
 ( 4, 2, 2, 2, 2, 2, 2, 2, 2, 2, 2, 2, 1, 2, 2, 2, 2, 2, 2, 2, 2, 4 ),
 ( 0.02390068823634509954, 0.02538837671117074798, 0.02613222094858357047, 0.02687606518599639643, 0.02836375366082206570, 0.02985144213564773497, 0.03059528637306056092, 0.03133913061047338688, 0.03282681908529903880, 0.03431450756012469072, 0.03580219603495034264, 0.03654604027236316860, 0.03728988450977599456, 0.03803372874718882052, 0.03877757298460164648, 0.04026526145942728452, 0.04175294993425292950, 0.04324063840907856754, 0.04398448264649139350, 0.04472832688390421252, 0.04621601535872984362, 0.04770370383355547472 ),
 .UNSPECIFIED. ) ;
#503=ORIENTED_EDGE ( 'NONE', *, *, #6828, .T. ) ;
#504=AXIS2_PLACEMENT_3D ( 'NONE', #27279, #48719, #561 ) ;
#505=CARTESIAN_POINT ( 'NONE',  ( -9.763294602873864747, 7.024900256480051119, 18.02051675412898391 ) ) ;
#506=CARTESIAN_POINT ( 'NONE',  ( 36.98541457540711974, 9.120571655722418569, -36.00309299526835360 ) ) ;
#507=CARTESIAN_POINT ( 'NONE',  ( -38.89042640463648581, 10.93374343663409043, 65.54896640531427465 ) ) ;
#512=CARTESIAN_POINT ( 'NONE',  ( -153.1121305730337383, 67.29834700374530598, 71.64627490104848562 ) ) ;
#516=CARTESIAN_POINT ( 'NONE',  ( -125.4433371161043311, 46.19736518073187170, 18.77539728269342589 ) ) ;
#517=CARTESIAN_POINT ( 'NONE',  ( -84.23431294393863311, 24.52078568147203441, -47.66442666584986654 ) ) ;
#519=CARTESIAN_POINT ( 'NONE',  ( 23.23895241123074484, 6.853530908437178049, 63.37105988032327986 ) ) ;
#521=CARTESIAN_POINT ( 'NONE',  ( 9.827939172326081163, 6.382931149346556587, -65.28444710517328531 ) ) ;
#524=ORIENTED_EDGE ( 'NONE', *, *, #39838, .T. ) ;
#530=CARTESIAN_POINT ( 'NONE',  ( 56.28782924480456984, 12.23883190161850720, -66.71350665837964300 ) ) ;
#542=CARTESIAN_POINT ( 'NONE',  ( 112.1009898303695138, 30.86414810229296890, 71.23698475841351296 ) ) ;
#543=CARTESIAN_POINT ( 'NONE',  ( 104.6431565033459492, 27.47282014102828995, -92.10596456002596710 ) ) ;
#545=CARTESIAN_POINT ( 'NONE',  ( -71.59086462055189770, 19.75139532313338719, -45.11543775482815732 ) ) ;
#546=CARTESIAN_POINT ( 'NONE',  ( -96.43148989374459745, 29.90755650959363621, 42.74068095059843841 ) ) ;
#549=ORIENTED_EDGE ( 'NONE', *, *, #6542, .T. ) ;
#550=EDGE_LOOP ( 'NONE', ( #10734, #24849 ) ) ;
#551=CARTESIAN_POINT ( 'NONE',  ( 110.2429982417149290, 28.88204397445231209, -50.92243756565370916 ) ) ;
#559=CARTESIAN_POINT ( 'NONE',  ( -142.0062637385109667, 58.06920992247430036, -41.76235797465353272 ) ) ;
#561=DIRECTION ( 'NONE',  ( 0.000000000000000000, 0.000000000000000000, 1.000000000000000000 ) ) ;
#564=VERTEX_POINT ( 'NONE', #57576 ) ;
#569=CARTESIAN_POINT ( 'NONE',  ( 137.3958226571046737, 43.60243650158411555, -23.30772740699958945 ) ) ;
#570=CARTESIAN_POINT ( 'NONE',  ( 91.51282003084288874, 21.14522045960329422, -64.45296707595953478 ) ) ;
#571=CARTESIAN_POINT ( 'NONE',  ( 198.2545923567585930, 97.90679023593582997, 6.013806333985140640 ) ) ;
#573=CARTESIAN_POINT ( 'NONE',  ( -99.97541017369788108, 31.62502926470688180, 18.32712433046064149 ) ) ;
#577=CARTESIAN_POINT ( 'NONE',  ( 42.03492317486907837, 8.766487167902370814, 30.38697801852312708 ) ) ;
#582=CARTESIAN_POINT ( 'NONE',  ( -76.10382222627278281, 22.43453174720078636, -62.40726938075579255 ) ) ;
#584=CARTESIAN_POINT ( 'NONE',  ( 46.65974587859241041, 10.48396258569371220, -45.07370360866829628 ) ) ;
#587=CARTESIAN_POINT ( 'NONE',  ( -29.74902699556085039, 10.33856194202127199, 18.18303581849161077 ) ) ;
#592=CARTESIAN_POINT ( 'NONE',  ( 151.1607415860635513, 52.90668588398087024, -20.86606007747752400 ) ) ;
#596=CARTESIAN_POINT ( 'NONE',  ( 208.5494659193436462, 111.7747784805681164, 83.93795935829461996 ) ) ;
#598=ORIENTED_EDGE ( 'NONE', *, *, #20731, .F. ) ;
#599=CARTESIAN_POINT ( 'NONE',  ( 60.61895554631705352, 13.15982272268128028, 71.28075859643588785 ) ) ;
#601=CARTESIAN_POINT ( 'NONE',  ( -8.314488422519705324, 7.931352979988700369, 3.271030448983515804 ) ) ;
#602=CARTESIAN_POINT ( 'NONE',  ( 41.09759788073309750, 9.651672055033843733, -62.65450869435315440 ) ) ;
#603=CARTESIAN_POINT ( 'NONE',  ( -2.190131154568196070, 6.589492063460817839, 32.66031877935753869 ) ) ;
#605=CARTESIAN_POINT ( 'NONE',  ( 79.14363954553030567, 18.05357752518858661, 91.47790248387103418 ) ) ;
#612=CARTESIAN_POINT ( 'NONE',  ( -170.2856292770788968, 85.50720222068218845, -49.16844864926446235 ) ) ;
#615=CARTESIAN_POINT ( 'NONE',  ( -128.1267916618074594, 49.19573276651588856, -35.23903939184793188 ) ) ;
#618=DIRECTION ( 'NONE',  ( -0.000000000000000000, 1.000000000000000000, -0.000000000000000000 ) ) ;
#624=CARTESIAN_POINT ( 'NONE',  ( 86.62931800182292363, 19.42108912189599224, -89.51066537983906812 ) ) ;
#629=VERTEX_POINT ( 'NONE', #36460 ) ;
#631=CARTESIAN_POINT ( 'NONE',  ( 82.94816950786170651, 19.25538918181908343, 16.90648424603243072 ) ) ;
#633=CARTESIAN_POINT ( 'NONE',  ( -100.4347360276019288, 32.97716872911834685, 30.73474136560336234 ) ) ;
#639=CARTESIAN_POINT ( 'NONE',  ( -75.43044859198180063, 21.11535168543637653, -9.000624265271870428 ) ) ;
#641=CARTESIAN_POINT ( 'NONE',  ( -24.85653282846401879, 9.618702155736652770, 94.99999999999866418 ) ) ;
#642=CARTESIAN_POINT ( 'NONE',  ( 154.0281735872262630, 56.28213428456460576, 16.73232576723794907 ) ) ;
#644=CARTESIAN_POINT ( 'NONE',  ( 164.9534461562628564, 63.71129898458568874, 36.33204052779463922 ) ) ;
#649=CARTESIAN_POINT ( 'NONE',  ( -144.2298831394396075, 61.12003712726058069, -90.66825305514043976 ) ) ;
#650=CARTESIAN_POINT ( 'NONE',  ( -35.99432170610150905, 10.38324794858010058, -21.95070075044081648 ) ) ;
#652=CARTESIAN_POINT ( 'NONE',  ( -38.69577193929646342, 10.89562623693160148, -71.62007173369499924 ) ) ;
#663=CARTESIAN_POINT ( 'NONE',  ( 69.20492276531108189, 14.19384449732238807, 86.75300155572325878 ) ) ;
#667=CARTESIAN_POINT ( 'NONE',  ( -52.60225734941438702, 15.07707183530729012, 84.41092461975652839 ) ) ;
#669=VECTOR ( 'NONE', #8748, 1000.000000000000000 ) ;
#673=VECTOR ( 'NONE', #25427, 1000.000000000000000 ) ;
#676=CARTESIAN_POINT ( 'NONE',  ( 210.9747454890631388, 115.3673079504856105, -66.55747008898767092 ) ) ;
#680=DIRECTION ( 'NONE',  ( -0.000000000000000000, 1.000000000000000000, -0.000000000000000000 ) ) ;
#681=CARTESIAN_POINT ( 'NONE',  ( 202.8477687489651373, 103.8400411879524228, 83.10837270847002856 ) ) ;
#683=CARTESIAN_POINT ( 'NONE',  ( 164.9540180502650912, 65.02981548735054673, -69.90027363021420115 ) ) ;
#685=ADVANCED_FACE ( 'NONE', ( #27535 ), #36810, .F. ) ;
#690=CARTESIAN_POINT ( 'NONE',  ( -86.15441609607631790, 25.31657638323081727, 37.42314418770195772 ) ) ;
#691=CARTESIAN_POINT ( 'NONE',  ( 157.0357419681844533, 58.58786672900117765, -77.95933384252394660 ) ) ;
#692=CARTESIAN_POINT ( 'NONE',  ( 46.90170507415073331, 10.52318308703818772, 37.90916503474270627 ) ) ;
#693=CARTESIAN_POINT ( 'NONE',  ( -26.88245755577922935, 8.887394979218516511, 58.58345839708251646 ) ) ;
#694=CARTESIAN_POINT ( 'NONE',  ( 131.6189313563687335, 40.08924984825277704, -9.505401706098517423 ) ) ;
#701=CARTESIAN_POINT ( 'NONE',  ( 206.7099580236349823, 109.1417833474364159, 43.94436230140331645 ) ) ;
#702=CARTESIAN_POINT ( 'NONE',  ( 141.3576134020958932, 47.34559817395930992, 90.83861031058405899 ) ) ;
#703=CARTESIAN_POINT ( 'NONE',  ( -27.40573813655178270, 9.981056867228259577, -90.17953602832123750 ) ) ;
#709=ORIENTED_EDGE ( 'NONE', *, *, #24458, .T. ) ;
#717=CARTESIAN_POINT ( 'NONE',  ( 66.08620257826613908, 13.40585338179127106, 44.15986684989842104 ) ) ;
#721=CARTESIAN_POINT ( 'NONE',  ( 83.37786665291103816, 18.33670623396830024, 17.14338525297940308 ) ) ;
#722=ORIENTED_EDGE ( 'NONE', *, *, #59330, .F. ) ;
#728=EDGE_CURVE ( 'NONE', #63173, #34225, #68915, .T. ) ;
#729=CARTESIAN_POINT ( 'NONE',  ( 94.02921784728462740, 22.08005910033071473, 11.61440990420907404 ) ) ;
#734=CYLINDRICAL_SURFACE ( 'NONE', #62377, 7.500000000000020428 ) ;
#735=CARTESIAN_POINT ( 'NONE',  ( -177.5288247523079406, 93.72924674643516596, -36.12611155980226130 ) ) ;
#737=CARTESIAN_POINT ( 'NONE',  ( -173.1211646369891355, -170.0000000000000000, -22.86740657428632773 ) ) ;
#743=FACE_BOUND ( 'NONE', #56230, .T. ) ;
#745=CARTESIAN_POINT ( 'NONE',  ( -180.5954680880247167, 97.44843622358462198, 64.52607031460266285 ) ) ;
#746=CARTESIAN_POINT ( 'NONE',  ( -146.1201263095600211, 62.66021356509621398, -8.772963640185553302 ) ) ;
#748=CARTESIAN_POINT ( 'NONE',  ( -86.15466590221106458, 26.40813842494317853, 11.56579973364435787 ) ) ;
#751=CARTESIAN_POINT ( 'NONE',  ( -72.43779980922290918, 20.04595627325881324, -92.10289429969509456 ) ) ;
#752=CARTESIAN_POINT ( 'NONE',  ( 66.08620257826611066, 13.40585338179127106, 17.31531625943474495 ) ) ;
#753=CARTESIAN_POINT ( 'NONE',  ( 159.2389084450349515, 59.03884018680375334, 17.36706718780300562 ) ) ;
#754=CARTESIAN_POINT ( 'NONE',  ( 92.95016907945944240, 22.74936990452174967, -20.52150210306960432 ) ) ;
#758=EDGE_LOOP ( 'NONE', ( #20135, #22340, #67146, #6100 ) ) ;
#762=CARTESIAN_POINT ( 'NONE',  ( 116.8402898440648841, 33.18057798316834095, 94.43274024419686441 ) ) ;
#763=CARTESIAN_POINT ( 'NONE',  ( -149.0764453401866660, 65.13297611514532548, 57.56537183036272864 ) ) ;
#764=CARTESIAN_POINT ( 'NONE',  ( 70.51484748609222208, 14.53801151001411540, -16.88811832611002117 ) ) ;
#767=CARTESIAN_POINT ( 'NONE',  ( -51.34542473642583360, 14.75635007918829622, -76.08508367074277601 ) ) ;
#769=CARTESIAN_POINT ( 'NONE',  ( -76.57252593202586866, 22.60812157331044148, -89.09011755351514239 ) ) ;
#770=CARTESIAN_POINT ( 'NONE',  ( -124.1007047332777802, 46.52282960291162084, -22.86580842938086988 ) ) ;
#773=CARTESIAN_POINT ( 'NONE',  ( 32.15284246740099405, 8.588257691344876932, 66.19772994508791442 ) ) ;
#774=CARTESIAN_POINT ( 'NONE',  ( 174.9042454172879957, 72.57746269938726869, 67.93336458024957381 ) ) ;
#776=CARTESIAN_POINT ( 'NONE',  ( -165.6397095829521504, 80.60756690931938806, 64.55706535356031850 ) ) ;
#780=VERTEX_POINT ( 'NONE', #3099 ) ;
#781=CARTESIAN_POINT ( 'NONE',  ( 109.7782172510783312, 29.77507867835874222, -50.92243756565370205 ) ) ;
#782=CARTESIAN_POINT ( 'NONE',  ( -13.47230132170245476, 7.324574289401438065, 69.42015683888705269 ) ) ;
#783=CARTESIAN_POINT ( 'NONE',  ( 205.5049354810106763, 109.1776577097391225, 2.363170148305743457 ) ) ;
#784=CARTESIAN_POINT ( 'NONE',  ( -83.06837433973049656, 25.13241508624138376, -90.21674049272554896 ) ) ;
#785=CARTESIAN_POINT ( 'NONE',  ( 46.50207827473963107, 9.439498081273466568, -18.70419972480020476 ) ) ;
#787=FACE_BOUND ( 'NONE', #41544, .T. ) ;
#789=CARTESIAN_POINT ( 'NONE',  ( 159.2258951716709987, 60.31399909112332836, 56.44886570136385018 ) ) ;
#791=EDGE_CURVE ( 'NONE', #60292, #33533, #43667, .T. ) ;
#792=ORIENTED_EDGE ( 'NONE', *, *, #874, .T. ) ;
#798=CARTESIAN_POINT ( 'NONE',  ( 154.4550750032602195, 55.34393534448155805, 16.93593135338981526 ) ) ;
#799=CARTESIAN_POINT ( 'NONE',  ( -1.184052349595404507, 7.556339067815312838, 87.80471432908419160 ) ) ;
#805=VERTEX_POINT ( 'NONE', #29820 ) ;
#808=CARTESIAN_POINT ( 'NONE',  ( 93.32756701508621688, 22.89083686918420568, -66.75542603816978726 ) ) ;
#814=EDGE_CURVE ( 'NONE', #41171, #10653, #16834, .T. ) ;
#815=CARTESIAN_POINT ( 'NONE',  ( 162.6205203824433170, 63.07332653227189212, 42.36688915199772509 ) ) ;
#819=CARTESIAN_POINT ( 'NONE',  ( -156.4966862384868591, 71.70877417666513054, -66.38460535960628306 ) ) ;
#820=CARTESIAN_POINT ( 'NONE',  ( 70.46579300139244140, 15.56614468937218909, 11.46688215326957305 ) ) ;
#823=CARTESIAN_POINT ( 'NONE',  ( 102.7446498997619955, 26.65764321315727514, -17.11449461936757999 ) ) ;
#824=CARTESIAN_POINT ( 'NONE',  ( -125.8938041572051389, 47.69968343338781125, 72.46449846362081360 ) ) ;
#825=CARTESIAN_POINT ( 'NONE',  ( 8.478575283864731915, 7.382882227715639623, 39.21115070528450985 ) ) ;
#832=CARTESIAN_POINT ( 'NONE',  ( -14.55425570676091951, 7.423011834016145727, -12.75193667354853488 ) ) ;
#833=CARTESIAN_POINT ( 'NONE',  ( -166.2425995121691642, 81.22826102820870631, 94.99999999999866418 ) ) ;
#835=CARTESIAN_POINT ( 'NONE',  ( 39.40195752203892710, -170.0000000000000000, -96.80891864635512434 ) ) ;
#836=CARTESIAN_POINT ( 'NONE',  ( -37.07436112751820190, 11.60822760208522375, 69.53422127808219955 ) ) ;
#837=CARTESIAN_POINT ( 'NONE',  ( -13.92109095214680359, 8.375243258322932149, -20.44991048438748038 ) ) ;
#838=CARTESIAN_POINT ( 'NONE',  ( -72.21652659655761397, 19.96855882996548459, -73.32001115466152896 ) ) ;
#843=ORIENTED_EDGE ( 'NONE', *, *, #16764, .T. ) ;
#844=CARTESIAN_POINT ( 'NONE',  ( 66.07923263163412742, 14.44036440558002532, -23.22621644188427226 ) ) ;
#846=CARTESIAN_POINT ( 'NONE',  ( -25.34321324147440180, 9.685523517558388917, 86.98799891496780390 ) ) ;
#847=CARTESIAN_POINT ( 'NONE',  ( -96.45845418068302024, 29.92035703021965176, -47.26932368623729985 ) ) ;
#849=CARTESIAN_POINT ( 'NONE',  ( -109.7647482398635361, 36.74843029291206165, 11.72205608543185562 ) ) ;
#850=CARTESIAN_POINT ( 'NONE',  ( 23.09541709302172308, 6.844586979481588784, 35.80722948394830496 ) ) ;
#854=ORIENTED_EDGE ( 'NONE', *, *, #55316, .F. ) ;
#857=CARTESIAN_POINT ( 'NONE',  ( -157.0069571479806996, 72.18154199622279066, -15.76883794595808652 ) ) ;
#858=CARTESIAN_POINT ( 'NONE',  ( 35.44311777160621091, 8.940232499250168274, -36.74501715293298076 ) ) ;
#861=CARTESIAN_POINT ( 'NONE',  ( -38.93922791710217268, 10.94334660650241986, 64.31909387702090442 ) ) ;
#862=CARTESIAN_POINT ( 'NONE',  ( 201.5987353083855851, 103.8544727311227405, 56.70899253505132975 ) ) ;
#864=CARTESIAN_POINT ( 'NONE',  ( 188.4374648754671000, 87.87346242052437617, 62.14831556033239934 ) ) ;
#865=CARTESIAN_POINT ( 'NONE',  ( -152.9121563765243934, 67.12206067149026012, 71.75184801906829080 ) ) ;
#866=CARTESIAN_POINT ( 'NONE',  ( -3.253130881186333312, 7.643323950922365384, -48.88322396365997236 ) ) ;
#870=CARTESIAN_POINT ( 'NONE',  ( 22.89234820949994287, 6.832052815347870123, 61.94203120367916426 ) ) ;
#873=CARTESIAN_POINT ( 'NONE',  ( 14.08699529666005823, 6.452200550165255954, -62.55491622521332573 ) ) ;
#874=EDGE_CURVE ( 'NONE', #69029, #46944, #44509, .T. ) ;
#880=CARTESIAN_POINT ( 'NONE',  ( -133.1527834403230486, 51.46311219732124442, -67.35340832687874979 ) ) ;
#881=CARTESIAN_POINT ( 'NONE',  ( -133.3149301983942223, 51.57857650535022032, -41.29510496815424148 ) ) ;
#883=CARTESIAN_POINT ( 'NONE',  ( 57.09527843067915143, 12.40436368789085897, -74.67611128734689885 ) ) ;
#884=ORIENTED_EDGE ( 'NONE', *, *, #38208, .T. ) ;
#889=VERTEX_POINT ( 'NONE', #17803 ) ;
#890=CARTESIAN_POINT ( 'NONE',  ( 175.5493994043409600, 73.18740965572595769, -38.65758324743049457 ) ) ;
#892=ORIENTED_EDGE ( 'NONE', *, *, #45337, .F. ) ;
#893=DIRECTION ( 'NONE',  ( -0.000000000000000000, 1.000000000000000000, -0.000000000000000000 ) ) ;
#894=CARTESIAN_POINT ( 'NONE',  ( 138.1901928158493433, 45.29454828899442731, 69.99416493423962038 ) ) ;
#895=CARTESIAN_POINT ( 'NONE',  ( -72.78737098446266884, 20.16853011470087864, -47.29921101198596745 ) ) ;
#898=CARTESIAN_POINT ( 'NONE',  ( 15.78827728214693416, 6.500811158483284835, -50.51894409868581448 ) ) ;
#899=CARTESIAN_POINT ( 'NONE',  ( -51.13576748034041231, 14.70354244225167761, -22.27226429992984080 ) ) ;
#908=CARTESIAN_POINT ( 'NONE',  ( -165.6754884515988522, 79.20562145685592270, -95.00000000000133582 ) ) ;
#909=CARTESIAN_POINT ( 'NONE',  ( -133.3396229538948887, 51.59616673977242129, 92.77099222264472189 ) ) ;
#911=CARTESIAN_POINT ( 'NONE',  ( 58.09877917144279280, 12.61383386832654629, 4.783940807170354859 ) ) ;
#914=CARTESIAN_POINT ( 'NONE',  ( -147.7860806339125190, 62.73248524776226276, 57.75265429496991487 ) ) ;
#915=DIRECTION ( 'NONE',  ( 0.000000000000000000, 0.000000000000000000, 1.000000000000000000 ) ) ;
#917=CARTESIAN_POINT ( 'NONE',  ( 181.5072453427590347, 79.03352099595184654, -24.38050707541595585 ) ) ;
#918=CARTESIAN_POINT ( 'NONE',  ( 83.37786665291103816, 18.33670623396829313, -9.701165337484269457 ) ) ;
#919=AXIS2_PLACEMENT_3D ( 'NONE', #25441, #41263, #40910 ) ;
#921=CARTESIAN_POINT ( 'NONE',  ( 88.99522780200243233, 20.24180937454203999, -63.04501563759147587 ) ) ;
#922=CARTESIAN_POINT ( 'NONE',  ( -97.85576954355160240, 30.58918648956191078, 17.24970366714013181 ) ) ;
#924=ORIENTED_EDGE ( 'NONE', *, *, #7720, .F. ) ;
#927=CARTESIAN_POINT ( 'NONE',  ( 13.37366753069833436, 6.435102282077984626, 30.39700900802003503 ) ) ;
#932=CARTESIAN_POINT ( 'NONE',  ( 15.78827728214693060, 7.507518794609573831, 18.17015708224157322 ) ) ;
#933=DIRECTION ( 'NONE',  ( 0.000000000000000000, 0.000000000000000000, 1.000000000000000000 ) ) ;
#934=CARTESIAN_POINT ( 'NONE',  ( -119.6801029354225108, 43.71909921132880328, 33.91237456399324657 ) ) ;
#935=CARTESIAN_POINT ( 'NONE',  ( 160.9069879467681687, 60.37290772564309549, -77.15118032727514219 ) ) ;
#938=CARTESIAN_POINT ( 'NONE',  ( -28.81071653159241563, 10.19258396314333837, 17.90053607095121180 ) ) ;
#942=CARTESIAN_POINT ( 'NONE',  ( -86.05211524933166345, 25.27371147724188916, -95.00000000000133582 ) ) ;
#943=CARTESIAN_POINT ( 'NONE',  ( 126.4757069339777757, 38.29528077539266206, 35.65345800163305512 ) ) ;
#944=CARTESIAN_POINT ( 'NONE',  ( 34.45158752686798209, 8.829194381141999060, 16.22471098832457770 ) ) ;
#950=ORIENTED_EDGE ( 'NONE', *, *, #35514, .F. ) ;
#953=LINE ( 'NONE', #37193, #3939 ) ;
#954=CARTESIAN_POINT ( 'NONE',  ( 40.38132770291769447, 9.553709436640064112, -62.51267063216231179 ) ) ;
#956=CARTESIAN_POINT ( 'NONE',  ( -3.868882431147342871, 6.665575841812236391, 31.23930121114426228 ) ) ;
#959=CARTESIAN_POINT ( 'NONE',  ( 85.04045433923197095, 19.94575836658696844, 83.56420614133747904 ) ) ;
#961=AXIS2_PLACEMENT_3D ( 'NONE', #39309, #28758, #55474 ) ;
#963=B_SPLINE_CURVE_WITH_KNOTS ( 'NONE', 3,
 ( #47061, #48411, #15742, #53355, #25961, #243, #10453, #26647, #68849, #54039, #63247, #48081, #47391, #69538, #59335, #11148, #32613, #20672, #11845, #65677, #28373, #38229, #33670, #28732, #18179, #50183, #64975, #1646, #49466, #33324, #23107, #28022, #66038, #1300, #17108, #11483, #54750, #66388, #599, #59671, #32955, #2011, #60731 ),
 .UNSPECIFIED., .F., .F.,
 ( 4, 2, 2, 2, 2, 2, 2, 2, 2, 2, 2, 2, 1, 2, 2, 2, 2, 2, 2, 2, 2, 4 ),
 ( 0.02379577142314830140, 0.02527778373276526672, 0.02601878988757374070, 0.02675979604238221121, 0.02824180835199915571, 0.02972382066161610020, 0.03046482681642458112, 0.03120583297123305858, 0.03268784528085004470, 0.03416985759046703430, 0.03565186990008403778, 0.03639287605489253952, 0.03713388220970104819, 0.03787488836450954993, 0.03861589451931805861, 0.04009790682893510372, 0.04157991913855214883, 0.04306193144816919394, 0.04380293760297770955, 0.04454394375778623905, 0.04602595606740328416, 0.04750796837702032926 ),
 .UNSPECIFIED. ) ;
#964=VERTEX_POINT ( 'NONE', #11816 ) ;
#968=CARTESIAN_POINT ( 'NONE',  ( -171.0950923142953570, 86.38958441093222973, -49.44577119986571745 ) ) ;
#971=CARTESIAN_POINT ( 'NONE',  ( -179.1930439439409781, 94.15101626040424776, 87.59719074105936443 ) ) ;
#972=ORIENTED_EDGE ( 'NONE', *, *, #43163, .F. ) ;
#973=CARTESIAN_POINT ( 'NONE',  ( -120.1497954511983437, 42.82624472369557367, -47.26276959957558432 ) ) ;
#981=CARTESIAN_POINT ( 'NONE',  ( 204.6977192012829789, 106.3443248447423315, -36.32593103262158252 ) ) ;
#982=CARTESIAN_POINT ( 'NONE',  ( -150.3831389294225289, 66.25266777263973950, 30.76890096360532922 ) ) ;
#987=CARTESIAN_POINT ( 'NONE',  ( 175.8874477961783782, 74.89984466412605002, 69.08197011996692538 ) ) ;
#988=VERTEX_POINT ( 'NONE', #32924 ) ;
#990=CARTESIAN_POINT ( 'NONE',  ( -77.71448999903256549, 21.96089801565736011, -8.316135682572610932 ) ) ;
#991=CARTESIAN_POINT ( 'NONE',  ( -37.36812455451343595, 11.66407928272600003, -91.89346562232887550 ) ) ;
#996=CARTESIAN_POINT ( 'NONE',  ( -76.79042791651910704, 22.68960395613479974, -35.34994931789273664 ) ) ;
#999=CARTESIAN_POINT ( 'NONE',  ( -38.16002576456688899, 10.79155573432543314, -19.31033324421229125 ) ) ;
#1000=CARTESIAN_POINT ( 'NONE',  ( 151.0569594231044448, 52.83149886109547566, -93.40118860444637505 ) ) ;
#1001=CARTESIAN_POINT ( 'NONE',  ( -38.55214349681828878, 10.86754840574841907, -72.09035779998554005 ) ) ;
#1002=CARTESIAN_POINT ( 'NONE',  ( 23.09590709048885770, 7.852755081912512480, 66.06499266665456105 ) ) ;
#1005=ORIENTED_EDGE ( 'NONE', *, *, #14250, .F. ) ;
#1006=DIRECTION ( 'NONE',  ( -0.000000000000000000, 1.000000000000000000, -0.000000000000000000 ) ) ;
#1011=LINE ( 'NONE', #66095, #27707 ) ;
#1014=CARTESIAN_POINT ( 'NONE',  ( -128.9786047358387009, 48.55852351614672102, 71.80467742803817544 ) ) ;
#1015=CARTESIAN_POINT ( 'NONE',  ( -49.02322089375218184, 14.18221587516665494, 86.99932311603028268 ) ) ;
#1017=CARTESIAN_POINT ( 'NONE',  ( 84.97343609940686804, 18.86260005312945154, 71.37542944298206748 ) ) ;
#1022=CYLINDRICAL_SURFACE ( 'NONE', #19496, 7.500000000000013323 ) ;
#1024=CARTESIAN_POINT ( 'NONE',  ( 210.5178985598940073, 114.6803933586780744, -65.93383091898544990 ) ) ;
#1027=CARTESIAN_POINT ( 'NONE',  ( -36.00055430895446307, 10.38468809415730831, -90.54901991010069651 ) ) ;
#1028=EDGE_CURVE ( 'NONE', #17268, #36885, #19337, .T. ) ;
#1030=CARTESIAN_POINT ( 'NONE',  ( 153.2384531768736338, 54.43344429203624202, -37.41481437027087509 ) ) ;
#1038=CARTESIAN_POINT ( 'NONE',  ( -85.34215807311493052, 24.97769003780924280, 41.34574464142236394 ) ) ;
#1039=CARTESIAN_POINT ( 'NONE',  ( -29.74902699556085039, 10.33856194202125245, -62.35061595289940328 ) ) ;
#1040=CARTESIAN_POINT ( 'NONE',  ( 42.03719354205839664, 9.783015072457470040, 44.43989967554949772 ) ) ;
#1041=CARTESIAN_POINT ( 'NONE',  ( -24.07146903340142785, 8.497560047608724076, 66.02689600193643571 ) ) ;
#1042=CARTESIAN_POINT ( 'NONE',  ( -149.2910611247328347, 63.99625741915658494, 18.87627064943540134 ) ) ;
#1045=EDGE_LOOP ( 'NONE', ( #10762, #53811 ) ) ;
#1049=CARTESIAN_POINT ( 'NONE',  ( 157.4703587214989113, 58.92748579479258808, -24.27963370867398396 ) ) ;
#1051=CARTESIAN_POINT ( 'NONE',  ( 63.01563776193091826, 12.67277567978498176, 56.65751152968497451 ) ) ;
#1052=CARTESIAN_POINT ( 'NONE',  ( -0.9897066053608937208, 7.549089325901769065, 61.36437911206027707 ) ) ;
#1054=CARTESIAN_POINT ( 'NONE',  ( 32.12337157895397866, -170.0000000000000000, -95.00000000000133582 ) ) ;
#1059=ORIENTED_EDGE ( 'NONE', *, *, #35607, .F. ) ;
#1063=CARTESIAN_POINT ( 'NONE',  ( 134.7720294983483029, 43.15885542353191084, 17.62355008800678746 ) ) ;
#1065=CIRCLE ( 'NONE', #56102, 243.4957430088094839 ) ;
#1069=CARTESIAN_POINT ( 'NONE',  ( -75.43044859198180063, 21.11535168543638363, 44.68847691565546398 ) ) ;
#1070=ORIENTED_EDGE ( 'NONE', *, *, #17625, .F. ) ;
#1075=CARTESIAN_POINT ( 'NONE',  ( 94.07616572255075482, 22.09777530676769075, 9.343156713767100996 ) ) ;
#1080=CARTESIAN_POINT ( 'NONE',  ( 33.46033188299907835, 8.722678254080106441, 32.83038915614411479 ) ) ;
#1081=CARTESIAN_POINT ( 'NONE',  ( -176.3763474213711504, 92.36993073950279154, -48.98273591874998800 ) ) ;
#1082=CARTESIAN_POINT ( 'NONE',  ( -128.7810612886106014, 48.42424427998343361, -22.49492442257137270 ) ) ;
#1091=FACE_BOUND ( 'NONE', #30911, .T. ) ;
#1092=CARTESIAN_POINT ( 'NONE',  ( -6.851003965218987801, 6.829052369041587411, -77.21532479566432983 ) ) ;
#1093=CARTESIAN_POINT ( 'NONE',  ( -177.1381400275771796, 93.26609858452819424, 58.81773603299666320 ) ) ;
#1095=CARTESIAN_POINT ( 'NONE',  ( -124.7710763417278486, 46.96042092553523162, -49.83267132162298196 ) ) ;
#1099=CARTESIAN_POINT ( 'NONE',  ( -75.76780310373240468, 21.23838321961104469, -89.37419894888229521 ) ) ;
#1101=CARTESIAN_POINT ( 'NONE',  ( -7.825402957745081878, 7.899365992529270741, 30.11558103944718923 ) ) ;
#1102=CARTESIAN_POINT ( 'NONE',  ( 116.0773578185793440, 31.67580513411751753, 5.527550488222392033 ) ) ;
#1103=CARTESIAN_POINT ( 'NONE',  ( 86.62931800182292363, 20.48449268398422163, -8.977013608448025650 ) ) ;
#1104=VERTEX_POINT ( 'NONE', #35367 ) ;
#1108=B_SPLINE_CURVE_WITH_KNOTS ( 'NONE', 3,
 ( #42123, #58294, #5180, #69193, #63582, #31920, #4829, #39199, #65944, #31569, #21019, #64265, #60640, #53349, #55003, #38486, #48074, #12457, #6484, #53005, #21350, #20664, #33917, #58630, #63923, #10446, #49720, #38851, #36853, #42798, #16073, #10112, #4493, #42464, #11746, #68841, #1549, #26301, #47385, #47730, #60295, #27932, #54657, #15735, #33226 ),
 .UNSPECIFIED., .F., .F.,
 ( 4, 2, 2, 2, 2, 2, 2, 2, 1, 2, 2, 2, 2, 2, 2, 2, 2, 2, 2, 2, 2, 2, 4 ),
 ( 0.000000000000000000, 0.001470449819620711336, 0.002205674729431056705, 0.002940899639241401856, 0.004411349458862072644, 0.005881799278482742997, 0.007352249098103413351, 0.008087474007913748528, 0.008822698917724084572, 0.009557923827534418881, 0.01029314873734475319, 0.01176359855696538191, 0.01249882346677569887, 0.01323404837658601410, 0.01470449819620668792, 0.01543972310601701009, 0.01617494801582733052, 0.01764539783544796792, 0.01911584765506860531, 0.01985107256487892574, 0.02058629747468924617, 0.02205674729430989051, 0.02352719711393053484 ),
 .UNSPECIFIED. ) ;
#1110=CARTESIAN_POINT ( 'NONE',  ( 81.76212856587197564, 18.87332718082994987, -75.87751552093126861 ) ) ;
#1111=CARTESIAN_POINT ( 'NONE',  ( 117.5606386312644247, 33.54431188492876714, 92.48088064648997886 ) ) ;
#1112=CYLINDRICAL_SURFACE ( 'NONE', #66073, 7.500000000000020428 ) ;
#1113=EDGE_CURVE ( 'NONE', #57471, #44581, #10986, .T. ) ;
#1114=CARTESIAN_POINT ( 'NONE',  ( 65.41496713438823463, 13.24164235279043744, -9.253839073797927028 ) ) ;
#1116=CARTESIAN_POINT ( 'NONE',  ( -29.74902699556085039, 10.33856194202125245, -35.50606536243572009 ) ) ;
#1117=CARTESIAN_POINT ( 'NONE',  ( -125.8938041572051105, 46.49392987655492959, -23.06915330777029638 ) ) ;
#1119=CARTESIAN_POINT ( 'NONE',  ( -190.6985136298601731, 109.1272424661242582, -73.40678087856149148 ) ) ;
#1121=ORIENTED_EDGE ( 'NONE', *, *, #19516, .T. ) ;
#1125=CARTESIAN_POINT ( 'NONE',  ( -165.7140086129057011, 80.68381997492575408, 63.95079900650693361 ) ) ;
#1130=CARTESIAN_POINT ( 'NONE',  ( 104.4006536356073980, 27.36759527624478139, -48.15181421002847628 ) ) ;
#1131=CARTESIAN_POINT ( 'NONE',  ( 188.2091813586561102, 87.61952156613880049, -14.52189767635950091 ) ) ;
#1132=CARTESIAN_POINT ( 'NONE',  ( -84.96580414052108665, 24.82184094495578108, -11.69303817377454635 ) ) ;
#1134=CARTESIAN_POINT ( 'NONE',  ( 46.42281973867195433, 9.426811321855149473, -13.62602333367861007 ) ) ;
#1135=CARTESIAN_POINT ( 'NONE',  ( 207.8675797643809915, 110.7908513421271977, -10.17102767663917540 ) ) ;
#1136=FACE_BOUND ( 'NONE', #24883, .T. ) ;
#1137=CARTESIAN_POINT ( 'NONE',  ( 157.9121974517528599, 59.27335488206246339, 56.25401806271705141 ) ) ;
#1138=ORIENTED_EDGE ( 'NONE', *, *, #24887, .T. ) ;
#1140=CARTESIAN_POINT ( 'NONE',  ( 93.08073375333745503, 22.79826000593201485, -47.15458855754309297 ) ) ;
#1142=CARTESIAN_POINT ( 'NONE',  ( -180.6209674222602075, 97.47999311542515954, 11.31048516350536381 ) ) ;
#1147=CARTESIAN_POINT ( 'NONE',  ( 55.51547041749727640, 11.05727559334830090, 10.22624786746376735 ) ) ;
#1153=CARTESIAN_POINT ( 'NONE',  ( 89.20981392318256553, 21.38519354635262459, -63.11988782574987056 ) ) ;
#1155=ORIENTED_EDGE ( 'NONE', *, *, #59225, .F. ) ;
#1157=CARTESIAN_POINT ( 'NONE',  ( 164.9540180502650912, 65.02981548735056094, 37.47792873164053873 ) ) ;
#1159=CARTESIAN_POINT ( 'NONE',  ( 104.4006536356074264, 27.36759527624477073, 5.537286970898872340 ) ) ;
#1163=CARTESIAN_POINT ( 'NONE',  ( 106.6181401479172308, 28.34160787025143335, -10.00766880435194217 ) ) ;
#1166=CARTESIAN_POINT ( 'NONE',  ( -130.2071229607962550, 50.62285182196875155, -9.415733337548060078 ) ) ;
#1167=CARTESIAN_POINT ( 'NONE',  ( -155.8069098289708165, 71.07457338077841769, -91.92448083599751385 ) ) ;
#1169=CARTESIAN_POINT ( 'NONE',  ( 92.91022130985207639, 21.66059330820416307, 94.99999999999866418 ) ) ;
#1170=CARTESIAN_POINT ( 'NONE',  ( -190.6985136298601731, 109.1272424661242582, 87.66052266422059347 ) ) ;
#1174=VERTEX_POINT ( 'NONE', #20912 ) ;
#1175=CARTESIAN_POINT ( 'NONE',  ( -12.39701069459754201, 7.231688578592713412, -22.03915780541799663 ) ) ;
#1176=CARTESIAN_POINT ( 'NONE',  ( -48.04019567818504299, 12.91272349839804434, 40.48869681787067520 ) ) ;
#1179=ADVANCED_FACE ( 'NONE', ( #58526 ), #31810, .F. ) ;
#1180=CARTESIAN_POINT ( 'NONE',  ( -34.74563762132953570, 11.17960945723135602, 71.29720797180668512 ) ) ;
#1181=EDGE_CURVE ( 'NONE', #67595, #55797, #53243, .T. ) ;
#1183=CARTESIAN_POINT ( 'NONE',  ( -75.01314391403411719, 20.96328762434828263, -76.02809170986127185 ) ) ;
#1184=CARTESIAN_POINT ( 'NONE',  ( 19.54475376904848005, 6.649964688461121654, -9.678301494481228673 ) ) ;
#1189=CARTESIAN_POINT ( 'NONE',  ( -143.8756912989387047, 60.83492035645719653, 16.33554224011767175 ) ) ;
#1191=CARTESIAN_POINT ( 'NONE',  ( -28.32971103059306373, 10.11911997875206204, 84.57276817772938671 ) ) ;
#1193=VECTOR ( 'NONE', #59745, 1000.000000000000000 ) ;
#1194=CARTESIAN_POINT ( 'NONE',  ( -95.52163045714284806, 29.47808868198299237, -45.77603188274618873 ) ) ;
#1195=CARTESIAN_POINT ( 'NONE',  ( -109.7290872258107015, 36.72869630780159156, 10.15525318343610728 ) ) ;
#1196=CARTESIAN_POINT ( 'NONE',  ( 15.29912143387263690, 7.491799981865499447, -50.51894409868582159 ) ) ;
#1204=CARTESIAN_POINT ( 'NONE',  ( 59.29597493004737885, 11.84030339376940510, -9.845320537704525421 ) ) ;
#1205=ADVANCED_FACE ( 'NONE', ( #15972 ), #37421, .F. ) ;
#1206=CARTESIAN_POINT ( 'NONE',  ( -47.56463531432804359, 12.80077789972090230, 38.30749179624960021 ) ) ;
#1208=CARTESIAN_POINT ( 'NONE',  ( 197.1975259970231775, 98.19639476549650681, 63.87880983231196552 ) ) ;
#1210=ORIENTED_EDGE ( 'NONE', *, *, #24253, .T. ) ;
#1211=CARTESIAN_POINT ( 'NONE',  ( 39.40195752203892710, -170.0000000000000000, -8.775266874964069430 ) ) ;
#1212=CARTESIAN_POINT ( 'NONE',  ( -150.3898662070192245, 64.92828409760430475, 72.56537183036274996 ) ) ;
#1214=CARTESIAN_POINT ( 'NONE',  ( -5.417282889646088506, 7.753782747238989970, -35.81092865362596456 ) ) ;
#1216=CARTESIAN_POINT ( 'NONE',  ( -165.7447522913192586, 79.27610653780159566, -94.42765512978321851 ) ) ;
#1218=FACE_BOUND ( 'NONE', #61286, .T. ) ;
#1220=CARTESIAN_POINT ( 'NONE',  ( 9.416656162223560500, 6.380306691996769253, -65.89949783066536781 ) ) ;
#1221=ORIENTED_EDGE ( 'NONE', *, *, #61362, .T. ) ;
#1224=CARTESIAN_POINT ( 'NONE',  ( -128.1219934350341703, 47.97781708504715681, -62.08223023690383258 ) ) ;
#1225=FACE_OUTER_BOUND ( 'NONE', #13546, .T. ) ;
#1227=CARTESIAN_POINT ( 'NONE',  ( 59.94652978725887493, 13.01168383647461724, -63.21766814124692502 ) ) ;
#1232=CARTESIAN_POINT ( 'NONE',  ( 182.3693118667488875, 79.91269779363329917, 83.08661189630149124 ) ) ;
#1233=EDGE_LOOP ( 'NONE', ( #15909, #46873 ) ) ;
#1236=CARTESIAN_POINT ( 'NONE',  ( 174.1364721914477229, 71.85829564941445824, -46.56446820418197774 ) ) ;
#1241=CARTESIAN_POINT ( 'NONE',  ( -75.01314391403410298, 20.96328762434827908, -49.18354111939758155 ) ) ;
#1244=CARTESIAN_POINT ( 'NONE',  ( 86.62931800182292363, 19.42108912189597092, -35.82156419891171595 ) ) ;
#1245=CARTESIAN_POINT ( 'NONE',  ( -50.14523569787234436, 14.45648954445650247, -21.56493559798800774 ) ) ;
#1251=CARTESIAN_POINT ( 'NONE',  ( -143.3980294393558950, 60.45217072626394383, -46.67054387122288261 ) ) ;
#1252=CARTESIAN_POINT ( 'NONE',  ( -167.6524579626394598, 82.69702609844095775, -74.19494829241439504 ) ) ;
#1253=CARTESIAN_POINT ( 'NONE',  ( -121.5946276578746534, 43.72760306970064192, 85.65620857137692212 ) ) ;
#1255=CARTESIAN_POINT ( 'NONE',  ( 56.94505604581133440, 12.37336791557970450, 6.057149477580686003 ) ) ;
#1257=CARTESIAN_POINT ( 'NONE',  ( -132.9409505933031710, 51.31241517713430511, 35.50028265355906143 ) ) ;
#1263=CARTESIAN_POINT ( 'NONE',  ( 81.74909803672915132, 17.81295302817861526, -22.19359623302083051 ) ) ;
#1265=CARTESIAN_POINT ( 'NONE',  ( 88.28780346671263146, 19.99350429399657614, -77.48438020982086982 ) ) ;
#1273=DIRECTION ( 'NONE',  ( -0.000000000000000000, 1.000000000000000000, -0.000000000000000000 ) ) ;
#1276=CARTESIAN_POINT ( 'NONE',  ( 210.6584452238135157, 116.7138338345753823, -48.40461618372044938 ) ) ;
#1279=CARTESIAN_POINT ( 'NONE',  ( -109.6660553119434951, 36.69391917620598775, 66.19210472742473428 ) ) ;
#1280=CARTESIAN_POINT ( 'NONE',  ( -27.70005010046225991, 9.007417901453015574, -36.31107217152676014 ) ) ;
#1288=CARTESIAN_POINT ( 'NONE',  ( -10.23867141318106455, 7.059827648235818209, -50.03618833735410476 ) ) ;
#1289=DIRECTION ( 'NONE',  ( 1.000000000000000000, 0.000000000000000000, -0.000000000000000000 ) ) ;
#1291=CARTESIAN_POINT ( 'NONE',  ( 132.9557829392755082, 42.05591979570418459, 29.55064835711428017 ) ) ;
#1292=CARTESIAN_POINT ( 'NONE',  ( 35.65622260226242446, 8.964590916200316784, 17.07156420890763115 ) ) ;
#1297=CARTESIAN_POINT ( 'NONE',  ( 63.01563776193091826, 13.70579113808094895, 29.81296093922127710 ) ) ;
#1300=CARTESIAN_POINT ( 'NONE',  ( 58.46823952472682606, 12.69204591816735572, 70.14181518529996140 ) ) ;
#1302=CARTESIAN_POINT ( 'NONE',  ( -13.77312480593388777, 8.361845410302541026, 6.195500647299365227 ) ) ;
#1303=EDGE_CURVE ( 'NONE', #59205, #889, #60969, .T. ) ;
#1306=CARTESIAN_POINT ( 'NONE',  ( 80.27480108964937244, 18.40368268764104442, 86.90318297740122944 ) ) ;
#1309=CARTESIAN_POINT ( 'NONE',  ( -125.8938041572051389, 47.69968343338778993, 57.46449846362076386 ) ) ;
#1310=CARTESIAN_POINT ( 'NONE',  ( -132.2352756077771687, 50.81350938245626025, 7.262685974171482428 ) ) ;
#1311=CARTESIAN_POINT ( 'NONE',  ( -169.1116812882276008, 84.24296059722693997, -35.85782011543879122 ) ) ;
#1312=CARTESIAN_POINT ( 'NONE',  ( -130.2071229607962550, 50.62285182196873734, -36.26028392801173084 ) ) ;
#1314=CARTESIAN_POINT ( 'NONE',  ( -118.6849742182705114, 41.92701402439732306, -40.32728246622576052 ) ) ;
#1316=DIRECTION ( 'NONE',  ( -0.000000000000000000, 1.000000000000000000, -0.000000000000000000 ) ) ;
#1317=DIRECTION ( 'NONE',  ( -0.000000000000000000, 1.000000000000000000, -0.000000000000000000 ) ) ;
#1319=ORIENTED_EDGE ( 'NONE', *, *, #24301, .T. ) ;
#1320=CARTESIAN_POINT ( 'NONE',  ( -60.95805269991219433, 17.39401718769329719, 6.342651992393583349 ) ) ;
#1321=CARTESIAN_POINT ( 'NONE',  ( 199.7255144154429161, 99.76581417577205002, -49.45988108201962774 ) ) ;
#1322=CARTESIAN_POINT ( 'NONE',  ( -95.63694837622348643, 30.64472169584718841, 41.50935696543631082 ) ) ;
#1324=CARTESIAN_POINT ( 'NONE',  ( 20.74093720376649941, 6.709541214524366026, -48.67227202248968609 ) ) ;
#1330=AXIS2_PLACEMENT_3D ( 'NONE', #4044, #15288, #14591 ) ;
#1332=VERTEX_POINT ( 'NONE', #12794 ) ;
#1333=CARTESIAN_POINT ( 'NONE',  ( 179.4227152810058215, 78.36166152262364903, 29.48269904055934276 ) ) ;
#1337=CARTESIAN_POINT ( 'NONE',  ( -8.314488422519703548, 7.931352979988683494, -77.26262132240753999 ) ) ;
#1339=CARTESIAN_POINT ( 'NONE',  ( 158.3595886390532428, 58.34525996025801220, 29.44919521104816340 ) ) ;
#1347=CARTESIAN_POINT ( 'NONE',  ( 110.7167338301704120, 30.21148223254619225, 44.61121420573734753 ) ) ;
#1348=CYLINDRICAL_SURFACE ( 'NONE', #27998, 7.500000000000013323 ) ;
#1350=CARTESIAN_POINT ( 'NONE',  ( 22.51798020284706325, 7.817376421459703018, 61.03934684355338192 ) ) ;
#1355=CARTESIAN_POINT ( 'NONE',  ( 209.2403607860319426, 112.7852583139808189, -91.53499439785448999 ) ) ;
#1356=CARTESIAN_POINT ( 'NONE',  ( -48.85180024597538306, 13.10609030261107932, 87.27526625388559012 ) ) ;
#1359=CARTESIAN_POINT ( 'NONE',  ( -103.4984104302275938, 33.40397788071886254, 84.30186542324130983 ) ) ;
#1362=CARTESIAN_POINT ( 'NONE',  ( -74.79539698934964065, 21.95498232236883496, -22.19923502380404301 ) ) ;
#1363=CARTESIAN_POINT ( 'NONE',  ( 80.73012746365746750, 17.49169339352361519, 68.71435551237969719 ) ) ;
#1365=CARTESIAN_POINT ( 'NONE',  ( 32.28603806442400526, 7.590310383548731110, 34.99384699948907240 ) ) ;
#1366=CARTESIAN_POINT ( 'NONE',  ( 187.5325688887157867, 85.37769363979907666, 40.67676355286661050 ) ) ;
#1369=LINE ( 'NONE', #21772, #32585 ) ;
#1370=CARTESIAN_POINT ( 'NONE',  ( -119.6801029354224966, 43.71909921132878907, 60.75692515445694397 ) ) ;
#1371=CARTESIAN_POINT ( 'NONE',  ( -48.56549579811110817, 13.03742088415616429, 14.76862391130607932 ) ) ;
#1374=CARTESIAN_POINT ( 'NONE',  ( 163.5944155533005642, 63.88379440759431560, -74.80571809177408227 ) ) ;
#1375=ORIENTED_EDGE ( 'NONE', *, *, #58489, .F. ) ;
#1382=CARTESIAN_POINT ( 'NONE',  ( -83.51052366780673708, 24.22613130369188994, 43.64917403576246357 ) ) ;
#1383=CARTESIAN_POINT ( 'NONE',  ( 154.6530827109543509, 56.75509330623211923, -63.51432978475487801 ) ) ;
#1384=CARTESIAN_POINT ( 'NONE',  ( 60.62939143133407072, 12.13148391928978143, -50.34764057611634058 ) ) ;
#1385=B_SPLINE_CURVE_WITH_KNOTS ( 'NONE', 3,
 ( #22950, #28571, #54595, #2196, #50023, #28212, #65519, #12396, #49659, #18715, #23994, #60232, #1488, #23308, #40167, #1857, #61275, #18020, #44756, #61624, #29268, #39820, #6419, #49311, #27873, #17674, #44394, #17314, #39471, #45087, #38785, #12045, #34565, #7816, #65881, #39139, #13099, #66573, #56007, #60923, #12746, #34207, #62311, #9194 ),
 .UNSPECIFIED., .F., .F.,
 ( 4, 2, 2, 2, 2, 2, 2, 2, 2, 2, 2, 2, 2, 2, 2, 2, 2, 2, 2, 2, 2, 4 ),
 ( 1.387778780781445676E-17, 0.004120577325733650390, 0.006180865988600449563, 0.008241154651467248737, 0.01030144331433404878, 0.01133158764576740543, 0.01236173197720076035, 0.01339187630863411874, 0.01442202064006747365, 0.01545216497150083031, 0.01648230930293418522, 0.01699738146865086355, 0.01751245363436754535, 0.01854259796580088465, 0.01957274229723423090, 0.02060288662866757020, 0.02266317529153428004, 0.02472346395440098640, 0.02678375261726769971, 0.02781389694870106330, 0.02884404128013443036, 0.03296461860586798881 ),
 .UNSPECIFIED. ) ;
#1387=CARTESIAN_POINT ( 'NONE',  ( -26.50364027666004674, 8.832969329054167318, 58.89264053224560769 ) ) ;
#1389=EDGE_LOOP ( 'NONE', ( #46759, #58270, #47068, #8834 ) ) ;
#1390=CARTESIAN_POINT ( 'NONE',  ( -55.05276343752908730, 15.72344139423347720, -8.371773407996169425 ) ) ;
#1392=CARTESIAN_POINT ( 'NONE',  ( 34.45158752686798209, 8.829194381142000836, -10.61983960213909306 ) ) ;
#1393=CARTESIAN_POINT ( 'NONE',  ( 181.0840389613909736, 78.60582251573003987, 2.464043515047718458 ) ) ;
#1395=CARTESIAN_POINT ( 'NONE',  ( -0.3255842968951683236, 7.525381170773409956, 64.95241148711420465 ) ) ;
#1396=B_SPLINE_CURVE_WITH_KNOTS ( 'NONE', 3,
 ( #47744, #20002, #42479, #31253, #4844, #63599, #41797, #42135, #57973, #47397, #36175, #25284, #4167, #68855, #69208, #36867, #15409, #9789, #14713, #20680, #9443, #63937, #25968, #62908, #57634, #58307, #10124, #30900, #52681, #35834, #52349, #25634, #36517, #53018, #30549, #21032, #4506, #47067, #68528, #31581, #46369, #9101, #26314, #30214, #63255, #67848, #14381, #20332, #15063, #62568 ),
 .UNSPECIFIED., .F., .F.,
 ( 4, 2, 2, 2, 2, 2, 2, 2, 2, 2, 2, 2, 2, 2, 2, 2, 2, 2, 2, 2, 2, 2, 2, 2, 4 ),
 ( 0.02688458561150008225, 0.02770990876165288150, 0.02853523191180568075, 0.03018587821211126537, 0.03183652451241685000, 0.03266184766256963190, 0.03348717081272241380, 0.03513781711302799149, 0.03678846341333356917, 0.03761378656348635108, 0.03843910971363913298, 0.03926443286379191488, 0.04008975601394469679, 0.04174040231425028141, 0.04256572546440307719, 0.04339104861455587991, 0.04421637176470867570, 0.04504169491486147148, 0.04586701806501427420, 0.04669234121516707692, 0.04834298751547272399, 0.04916831066562551977, 0.04999363381577832249, 0.05164428011608399038, 0.05329492641638964440 ),
 .UNSPECIFIED. ) ;
#1397=CARTESIAN_POINT ( 'NONE',  ( 198.3712756463373239, 99.67211044168692524, -93.48022478442567262 ) ) ;
#1402=EDGE_LOOP ( 'NONE', ( #21473, #51203 ) ) ;
#1406=CARTESIAN_POINT ( 'NONE',  ( 133.8566784816069060, 42.60093787723655367, 17.66579024853170310 ) ) ;
#1410=CARTESIAN_POINT ( 'NONE',  ( 80.16939877002758408, 17.31693935407229645, 14.20996114281630618 ) ) ;
#1415=EDGE_CURVE ( 'NONE', #10004, #63684, #40901, .T. ) ;
#1419=CARTESIAN_POINT ( 'NONE',  ( -144.7571537022063524, 60.25265659240449168, -74.96618912951997515 ) ) ;
#1421=DIRECTION ( 'NONE',  ( -0.000000000000000000, 1.000000000000000000, -0.000000000000000000 ) ) ;
#1426=CARTESIAN_POINT ( 'NONE',  ( 66.21212819542179773, 14.47309682125277774, 84.20943056763468348 ) ) ;
#1427=CARTESIAN_POINT ( 'NONE',  ( 35.65622260226241735, 8.964590916200318560, 43.91611479937130724 ) ) ;
#1428=CARTESIAN_POINT ( 'NONE',  ( -175.9944734395087096, 91.92390745845766276, -35.27130985876561198 ) ) ;
#1429=DIRECTION ( 'NONE',  ( -0.000000000000000000, 1.000000000000000000, -0.000000000000000000 ) ) ;
#1433=CARTESIAN_POINT ( 'NONE',  ( 128.0848616812662613, 38.04676222636083338, -65.55253114271090453 ) ) ;
#1434=ORIENTED_EDGE ( 'NONE', *, *, #24309, .T. ) ;
#1435=CARTESIAN_POINT ( 'NONE',  ( 134.7708899521910553, 43.15864772107688907, -77.81547585753226315 ) ) ;
#1436=CARTESIAN_POINT ( 'NONE',  ( -142.8492950481058870, 60.01492924994601452, -72.62007504265284297 ) ) ;
#1437=EDGE_CURVE ( 'NONE', #20980, #32549, #4275, .T. ) ;
#1438=ORIENTED_EDGE ( 'NONE', *, *, #9221, .F. ) ;
#1440=CARTESIAN_POINT ( 'NONE',  ( 8.000000000000007105, 249.8719672152120381, 94.99999999999866418 ) ) ;
#1441=CARTESIAN_POINT ( 'NONE',  ( -0.7174461528505768904, 6.532311451815526304, -67.35691283117644446 ) ) ;
#1442=CARTESIAN_POINT ( 'NONE',  ( -176.3856149167964986, 92.38076834121979175, 71.93273640432624916 ) ) ;
#1445=CARTESIAN_POINT ( 'NONE',  ( -5.183193881612057297, 7.740932022135017299, 44.63904903171023619 ) ) ;
#1448=CARTESIAN_POINT ( 'NONE',  ( -5.417282889646089394, 7.753782747238989081, -8.966378063162283141 ) ) ;
#1449=CARTESIAN_POINT ( 'NONE',  ( -11.79249160485393766, 8.191429102467035150, 43.98525602679245594 ) ) ;
#1450=CARTESIAN_POINT ( 'NONE',  ( 114.6632852039171127, 30.98120524556723510, 4.202855321170513747 ) ) ;
#1456=CARTESIAN_POINT ( 'NONE',  ( 79.39764314491563368, 18.13166883367086157, -72.17018488364679740 ) ) ;
#1457=CARTESIAN_POINT ( 'NONE',  ( 103.0076904570972687, 26.76944391674850365, 92.80592866474482605 ) ) ;
#1460=CARTESIAN_POINT ( 'NONE',  ( -23.93933407965395688, 9.495050561681672718, -42.32159819572655124 ) ) ;
#1466=CARTESIAN_POINT ( 'NONE',  ( 32.30062460741315533, 8.603096374765343057, 61.83302680985992339 ) ) ;
#1468=CARTESIAN_POINT ( 'NONE',  ( 39.81840452174282774, 8.463718892264783022, -89.30891864635512434 ) ) ;
#1470=CARTESIAN_POINT ( 'NONE',  ( -167.1619226259398943, 82.18315278115414912, -19.92833628696023496 ) ) ;
#1471=DIRECTION ( 'NONE',  ( -0.000000000000000000, 1.000000000000000000, -0.000000000000000000 ) ) ;
#1473=CARTESIAN_POINT ( 'NONE',  ( 103.1534365798308386, 26.83148826706846535, -40.92239761178424118 ) ) ;
#1474=CARTESIAN_POINT ( 'NONE',  ( 23.28809538736928175, 7.864824219997535337, -42.52675217981989420 ) ) ;
#1475=CARTESIAN_POINT ( 'NONE',  ( -85.10774223992955001, 24.88053943842882276, -19.62096145546114911 ) ) ;
#1476=CARTESIAN_POINT ( 'NONE',  ( -84.63218004431101349, 25.77252883085057533, -91.73812189727786404 ) ) ;
#1478=CARTESIAN_POINT ( 'NONE',  ( 210.5178985598939789, 114.6803933586780602, -12.24472973805804976 ) ) ;
#1479=FACE_BOUND ( 'NONE', #66534, .T. ) ;
#1480=CARTESIAN_POINT ( 'NONE',  ( -56.02358673658414290, 14.94347049174937503, -50.16887940659524503 ) ) ;
#1481=AXIS2_PLACEMENT_3D ( 'NONE', #48092, #69551, #32624 ) ;
#1486=LINE ( 'NONE', #22948, #64439 ) ;
#1487=DIRECTION ( 'NONE',  ( -0.000000000000000000, 1.000000000000000000, -0.000000000000000000 ) ) ;
#1488=CARTESIAN_POINT ( 'NONE',  ( 211.1046732743772338, 117.3965485104337176, 67.46095300389731619 ) ) ;
#1495=ORIENTED_EDGE ( 'NONE', *, *, #45979, .F. ) ;
#1498=CARTESIAN_POINT ( 'NONE',  ( -61.76386578474846800, 17.63453064612499688, -19.25649393556963318 ) ) ;
#1500=CARTESIAN_POINT ( 'NONE',  ( 103.0103829243729052, 25.67737053862328267, 39.16093723846415742 ) ) ;
#1502=EDGE_CURVE ( 'NONE', #68705, #58537, #3752, .T. ) ;
#1505=CARTESIAN_POINT ( 'NONE',  ( 163.1370549780984334, 63.50181104276889243, 31.97058753488886396 ) ) ;
#1506=CARTESIAN_POINT ( 'NONE',  ( 69.36122620657974380, 14.23458312296499528, 94.99999999999866418 ) ) ;
#1508=CARTESIAN_POINT ( 'NONE',  ( -173.1211646369891639, 87.12891641440852197, -88.40105834567665966 ) ) ;
#1509=CARTESIAN_POINT ( 'NONE',  ( 107.0447263249841541, 28.53200276018955961, -9.789778272522351443 ) ) ;
#1510=CARTESIAN_POINT ( 'NONE',  ( -48.58011387679029269, 14.07568064779664319, 7.175827997749510523 ) ) ;
#1513=CARTESIAN_POINT ( 'NONE',  ( -156.9402586331177361, 72.11962769956262775, -95.00000000000133582 ) ) ;
#1514=EDGE_CURVE ( 'NONE', #4893, #19257, #13498, .T. ) ;
#1516=CARTESIAN_POINT ( 'NONE',  ( 81.80451556658140078, 17.83033755654336261, 85.12011702748436903 ) ) ;
#1519=ORIENTED_EDGE ( 'NONE', *, *, #52020, .T. ) ;
#1522=CARTESIAN_POINT ( 'NONE',  ( -13.78709718204646961, 7.352743657744182926, -20.65034025157325459 ) ) ;
#1523=CARTESIAN_POINT ( 'NONE',  ( -165.6128944859384831, 80.58007050464003385, 92.14767930188499179 ) ) ;
#1524=CARTESIAN_POINT ( 'NONE',  ( -54.08504625707234936, 14.42374043447188114, -8.418564600962227473 ) ) ;
#1525=CARTESIAN_POINT ( 'NONE',  ( 102.7571040248400891, 25.57023079238897267, -16.05041636952068274 ) ) ;
#1526=CARTESIAN_POINT ( 'NONE',  ( -56.73868929054669508, 16.18382781951277849, -35.40422542096111869 ) ) ;
#1530=CARTESIAN_POINT ( 'NONE',  ( 21.88606409348644277, 6.772455198693825729, -20.54785372844966318 ) ) ;
#1537=CARTESIAN_POINT ( 'NONE',  ( -55.48176214950256480, 15.83928188623576894, -88.91464852580686795 ) ) ;
#1539=CARTESIAN_POINT ( 'NONE',  ( -29.85611858039614219, 10.35537958803110925, 84.06752208004112958 ) ) ;
#1548=CARTESIAN_POINT ( 'NONE',  ( -11.14445507968272153, 7.129894202659276203, 4.040923808319601740 ) ) ;
#1549=CARTESIAN_POINT ( 'NONE',  ( 35.44781468922820267, 7.928097401423682911, -76.34201268051539557 ) ) ;
#1550=CARTESIAN_POINT ( 'NONE',  ( 61.33627421985471528, 12.28939706835343770, -9.062593789058455584 ) ) ;
#1551=B_SPLINE_CURVE_WITH_KNOTS ( 'NONE', 3,
 ( #13741, #33813, #35196, #7076, #67235, #55256, #17634, #1814, #55609, #19019, #3200, #2501, #17987, #60542, #45050, #2160, #66535, #34172, #7780, #8120, #34526, #55968, #12356, #28535, #7439, #28891, #50677, #40470, #45755, #39431, #23612, #34864, #40133, #49983, #23270, #44717 ),
 .UNSPECIFIED., .F., .F.,
 ( 4, 2, 2, 2, 2, 2, 2, 2, 2, 2, 2, 2, 2, 2, 2, 2, 2, 4 ),
 ( 1.551583845779545699E-17, 0.001548367318450172845, 0.003096734636900330077, 0.004645101955350487526, 0.006193469273800644541, 0.007741836592250802423, 0.008516020251475891339, 0.009290203910700981990, 0.01083857122915114247, 0.01238693854760130643, 0.01393530586605147038, 0.01548367318450163087, 0.01703204050295179309, 0.01858040782140195704, 0.02012877513985211406, 0.02167714245830226760, 0.02322550977675242809, 0.02477387709520258510 ),
 .UNSPECIFIED. ) ;
#1553=CARTESIAN_POINT ( 'NONE',  ( -47.55235941796723154, 12.79790236059689512, 38.05499662510656123 ) ) ;
#1556=CARTESIAN_POINT ( 'NONE',  ( -56.73868929054668087, 16.18382781951278204, -62.24877601142479477 ) ) ;
#1557=CARTESIAN_POINT ( 'NONE',  ( 199.3764173596862292, 100.9540560740992134, -75.98014011034484838 ) ) ;
#1559=CARTESIAN_POINT ( 'NONE',  ( -4.502148936856956496, 7.704491846230412833, -36.17659697066419255 ) ) ;
#1560=CARTESIAN_POINT ( 'NONE',  ( 108.3906473026530080, 28.03385344351497466, 17.54929269514099133 ) ) ;
#1561=CARTESIAN_POINT ( 'NONE',  ( -167.1534554062404538, 80.72263015867910951, 16.02705747859470264 ) ) ;
#1563=FACE_BOUND ( 'NONE', #48077, .T. ) ;
#1570=CARTESIAN_POINT ( 'NONE',  ( 46.85206196242845778, 9.495795933269487676, -70.95794390456796918 ) ) ;
#1575=CYLINDRICAL_SURFACE ( 'NONE', #59147, 7.500000000000013323 ) ;
#1577=CARTESIAN_POINT ( 'NONE',  ( 188.4662191759685470, 86.40293565635343498, 89.15863815613664656 ) ) ;
#1578=EDGE_CURVE ( 'NONE', #62965, #28360, #26074, .T. ) ;
#1583=CARTESIAN_POINT ( 'NONE',  ( 151.6178224291901699, 54.48737267587419097, 41.60651290194002883 ) ) ;
#1593=CARTESIAN_POINT ( 'NONE',  ( -190.4968431727839118, 108.8425311198514720, 34.24491274770363702 ) ) ;
#1596=CARTESIAN_POINT ( 'NONE',  ( -73.81801970646054656, 21.60231032711191190, 16.80100356717971977 ) ) ;
#1597=EDGE_CURVE ( 'NONE', #58006, #60940, #60454, .T. ) ;
#1600=CARTESIAN_POINT ( 'NONE',  ( -130.5004577019969076, 49.60245395521563694, 85.88294129194291315 ) ) ;
#1601=ORIENTED_EDGE ( 'NONE', *, *, #1028, .F. ) ;
#1602=CARTESIAN_POINT ( 'NONE',  ( 82.14449817946437804, 17.93919511903895980, -37.30520553978547582 ) ) ;
#1603=EDGE_CURVE ( 'NONE', #4848, #2387, #65577, .T. ) ;
#1606=CARTESIAN_POINT ( 'NONE',  ( -147.3641864666714412, 62.38213854487950982, 57.86459567537096405 ) ) ;
#1607=CARTESIAN_POINT ( 'NONE',  ( 82.95856197793163744, 19.25847567427441120, 30.65358330111253338 ) ) ;
#1609=CARTESIAN_POINT ( 'NONE',  ( 91.12448333640237763, 22.07449368110502519, 31.18905971957590495 ) ) ;
#1610=CARTESIAN_POINT ( 'NONE',  ( 138.5721691894143817, 44.34516164557648921, -22.53138726545303427 ) ) ;
#1612=CARTESIAN_POINT ( 'NONE',  ( 88.30010642107258434, 19.99780058782974379, -62.85061619352340045 ) ) ;
#1615=CARTESIAN_POINT ( 'NONE',  ( -54.56685407443679736, 15.59259313022787907, 45.31732777293115078 ) ) ;
#1619=CARTESIAN_POINT ( 'NONE',  ( 46.42281973867196143, 9.426811321855154802, 40.06307784724872789 ) ) ;
#1623=VECTOR ( 'NONE', #26735, 1000.000000000000000 ) ;
#1624=CARTESIAN_POINT ( 'NONE',  ( 212.0779786303465926, 118.9010947973413437, -45.20355168328251239 ) ) ;
#1625=CARTESIAN_POINT ( 'NONE',  ( -72.35078170365746075, 21.08176362823952843, -73.51264129435554651 ) ) ;
#1627=CARTESIAN_POINT ( 'NONE',  ( -25.50312845906834980, 8.692070753302672870, -47.40798146362784848 ) ) ;
#1628=CARTESIAN_POINT ( 'NONE',  ( 162.0835148203876770, 61.32844276806159911, -76.40136503387930134 ) ) ;
#1631=CARTESIAN_POINT ( 'NONE',  ( -24.95010104166214404, 9.631487977190600347, 14.64071932601358128 ) ) ;
#1636=CARTESIAN_POINT ( 'NONE',  ( -85.09761763353363051, 24.87634954265997322, 68.62969091966090218 ) ) ;
#1639=CARTESIAN_POINT ( 'NONE',  ( 127.7121523762017858, -170.0000000000000000, 94.99999999999866418 ) ) ;
#1641=CARTESIAN_POINT ( 'NONE',  ( -190.6985136298601731, 109.1272424661242582, -95.00000000000133582 ) ) ;
#1642=CARTESIAN_POINT ( 'NONE',  ( 212.1739865054640006, 117.1950576737078791, 91.03382279583313164 ) ) ;
#1643=CARTESIAN_POINT ( 'NONE',  ( 133.8566784816069628, 41.42467568809806977, -36.02331093239566684 ) ) ;
#1646=CARTESIAN_POINT ( 'NONE',  ( 55.99998955208977236, 12.18058389017405396, 66.82069825596038015 ) ) ;
#1659=CARTESIAN_POINT ( 'NONE',  ( -165.6291901388946997, 79.15850773921177108, 92.52324537314119368 ) ) ;
#1661=CARTESIAN_POINT ( 'NONE',  ( -119.6995109608661352, 42.54844499216734022, -46.64985785500188342 ) ) ;
#1665=CARTESIAN_POINT ( 'NONE',  ( -6.840165690716690783, 7.836465889224639270, -77.21372475586606754 ) ) ;
#1670=CARTESIAN_POINT ( 'NONE',  ( -56.01329802674224112, 15.98369420723829570, 3.518770225379651784 ) ) ;
#1673=CARTESIAN_POINT ( 'NONE',  ( -99.10674985723791508, 32.31836975419496838, 31.20713615476282143 ) ) ;
#1675=CARTESIAN_POINT ( 'NONE',  ( 19.11168290073779019, 6.629794975642859356, -36.29099477203722302 ) ) ;
#1679=ORIENTED_EDGE ( 'NONE', *, *, #16264, .F. ) ;
#1685=CARTESIAN_POINT ( 'NONE',  ( 175.8947993867356843, 74.90689716047907609, 31.37274126135447716 ) ) ;
#1688=CARTESIAN_POINT ( 'NONE',  ( -38.07133317494998437, 11.79914672408466458, -92.97776376164446788 ) ) ;
#1698=CARTESIAN_POINT ( 'NONE',  ( -33.37566357177428955, 9.916833145467590427, -23.23467432567402824 ) ) ;
#1699=CARTESIAN_POINT ( 'NONE',  ( 157.4703587214989113, 57.65129005721575339, -89.81328548006499091 ) ) ;
#1700=CARTESIAN_POINT ( 'NONE',  ( -128.9843070188472609, 49.78011598923032466, 4.426543353926868818 ) ) ;
#1701=CARTESIAN_POINT ( 'NONE',  ( 22.51849650178394668, 7.817407610814552044, 67.67805970500643298 ) ) ;
#1703=B_SPLINE_CURVE_WITH_KNOTS ( 'NONE', 3,
 ( #20258, #36791, #32534, #68776, #26570, #53964, #47665, #16005, #41716, #48008, #10726, #4426, #48337, #32200, #5794, #31848, #5455, #53280, #64196, #14972, #21628, #64548, #36439, #69471, #57892, #25891, #31177, #47321, #52940, #20592, #15330, #58232, #10048, #31505, #21290, #42737, #27952, #48683, #39561, #21975, #17760, #17394, #61010, #38869 ),
 .UNSPECIFIED., .F., .F.,
 ( 4, 2, 2, 2, 2, 2, 2, 2, 2, 2, 2, 2, 2, 2, 2, 2, 2, 2, 2, 2, 2, 4 ),
 ( 0.000000000000000000, 0.003518733725596350382, 0.004398417156995416619, 0.005278100588394483289, 0.007037467451192677345, 0.007917150882591761363, 0.008796834313990845380, 0.01055620117678905678, 0.01231556803958726992, 0.01319525147098637476, 0.01407493490238548133, 0.01495461833378458789, 0.01583430176518369620, 0.01671398519658279930, 0.01759366862798190934, 0.01935303549078008084, 0.02111240235357825928, 0.02199208578497731728, 0.02287176921637638222, 0.02463113607917447739, 0.02639050294197256910, 0.02814986980477066428 ),
 .UNSPECIFIED. ) ;
#1704=ORIENTED_EDGE ( 'NONE', *, *, #46368, .T. ) ;
#1706=CARTESIAN_POINT ( 'NONE',  ( 205.3819056893079278, 107.2819694648321303, -90.01503221354890627 ) ) ;
#1707=CARTESIAN_POINT ( 'NONE',  ( -109.7686203588201010, 37.90089348911612888, 11.66623203320282975 ) ) ;
#1711=CARTESIAN_POINT ( 'NONE',  ( -146.1260528621668016, 61.36307454672303408, 31.51035454738589792 ) ) ;
#1712=CARTESIAN_POINT ( 'NONE',  ( -130.6002960060537248, 49.67125682092490280, 59.10497990830987192 ) ) ;
#1713=CARTESIAN_POINT ( 'NONE',  ( -71.22896441287285541, 20.69091426169410752, -16.76999692228343974 ) ) ;
#1715=CARTESIAN_POINT ( 'NONE',  ( 83.37786665291103816, 18.33670623396829313, 70.83248643390679433 ) ) ;
#1716=ORIENTED_EDGE ( 'NONE', *, *, #22252, .T. ) ;
#1718=CARTESIAN_POINT ( 'NONE',  ( 33.44983424733138122, 7.709709042132400825, 42.00358695764388983 ) ) ;
#1719=DIRECTION ( 'NONE',  ( 0.000000000000000000, 0.000000000000000000, 1.000000000000000000 ) ) ;
#1725=CARTESIAN_POINT ( 'NONE',  ( -125.4463376280758098, 47.40387005565909107, 57.47446237482950693 ) ) ;
#1726=CARTESIAN_POINT ( 'NONE',  ( -47.60396279792519181, 12.80997843568596295, 9.966546515805026374 ) ) ;
#1727=CARTESIAN_POINT ( 'NONE',  ( 150.8925291903903485, 52.71218673668933974, -47.26666548743844487 ) ) ;
#1728=AXIS2_PLACEMENT_3D ( 'NONE', #2173, #23628, #35212 ) ;
#1735=CARTESIAN_POINT ( 'NONE',  ( 63.01563776193091826, -170.0000000000000000, 64.15751152968499582 ) ) ;
#1737=DIRECTION ( 'NONE',  ( -0.000000000000000000, 1.000000000000000000, -0.000000000000000000 ) ) ;
#1741=CARTESIAN_POINT ( 'NONE',  ( 152.1381498073141358, 54.87048121475574192, -75.76501768209521970 ) ) ;
#1742=CARTESIAN_POINT ( 'NONE',  ( 43.96421756700841144, 10.06386361114660488, 31.44109886963873635 ) ) ;
#1743=CARTESIAN_POINT ( 'NONE',  ( -24.70354720400823112, 8.582324684301861240, 67.89677931424583335 ) ) ;
#1744=B_SPLINE_CURVE_WITH_KNOTS ( 'NONE', 3,
 ( #15560, #52825, #20142, #58123, #31054, #9939, #26801, #52498, #48228, #64084, #10961, #47541, #58792, #26111, #21181, #26460, #31728, #4648, #20829, #41594, #69005, #42288, #25781, #47208, #64427, #63751, #4317, #58449, #42627, #10267, #63052, #53162, #15896, #37340, #16238, #32428, #37690, #57779, #59138, #53855, #46876, #68667, #68340 ),
 .UNSPECIFIED., .F., .F.,
 ( 4, 2, 2, 2, 2, 2, 2, 2, 1, 2, 2, 2, 2, 2, 2, 2, 2, 2, 2, 2, 2, 4 ),
 ( 3.469446951953614189E-18, 0.001466285743483490599, 0.002199428615225229935, 0.002932571486966969922, 0.004398857230450423442, 0.005865142973933877395, 0.007331428717417331348, 0.008064571589159075238, 0.008797714460900817393, 0.009530857332642563018, 0.01026400020438430691, 0.01173028594786779469, 0.01319657169135128420, 0.01466285743483477372, 0.01539600030657651934, 0.01612914317831826497, 0.01759542892180175969, 0.01906171466528525787, 0.01979485753702700523, 0.02052800040876874912, 0.02199428615225222997, 0.02346057189573570734 ),
 .UNSPECIFIED. ) ;
#1745=EDGE_CURVE ( 'NONE', #50582, #41326, #16091, .T. ) ;
#1753=CARTESIAN_POINT ( 'NONE',  ( 140.9255869758567030, 47.06171785931592666, 88.16863402254999471 ) ) ;
#1754=B_SPLINE_CURVE_WITH_KNOTS ( 'NONE', 3,
 ( #19820, #14871, #13503, #35655, #3984, #51486, #45500, #19461, #30026, #41611, #2600, #41273, #67328, #63067, #13840, #36339, #25455, #57791, #40920, #8919, #35992, #3295, #66985, #24060, #18777, #31072, #40233, #62380, #8227, #67665, #40570, #57447, #29674, #61681, #34959, #62021, #62731, #56403, #51136, #2952, #46536, #14196, #20158 ),
 .UNSPECIFIED., .F., .F.,
 ( 4, 2, 2, 2, 2, 2, 2, 2, 2, 2, 2, 2, 1, 2, 2, 2, 2, 2, 2, 2, 2, 4 ),
 ( 0.02362927190606133043, 0.02510248541563190466, 0.02583909217041719872, 0.02657569892520248930, 0.02804891243477306007, 0.02952212594434362736, 0.03025873269912889713, 0.03099533945391416689, 0.03246855296348473419, 0.03394176647305530842, 0.03541497998262588265, 0.03615158673741118711, 0.03688819349219649157, 0.03762480024698179604, 0.03836140700176710744, 0.03983462051133768167, 0.04130783402090825590, 0.04278104753047883013, 0.04351765428526413459, 0.04425426104004942518, 0.04572747454962002023, 0.04720068805919060834 ),
 .UNSPECIFIED. ) ;
#1755=EDGE_CURVE ( 'NONE', #52438, #42077, #26195, .T. ) ;
#1756=CARTESIAN_POINT ( 'NONE',  ( -190.6985136298601731, 109.1272424661242582, -95.00000000000133582 ) ) ;
#1763=CARTESIAN_POINT ( 'NONE',  ( 164.0158927577712689, 62.92463143894076438, -20.47931855560399939 ) ) ;
#1767=DIRECTION ( 'NONE',  ( 1.000000000000000000, 0.000000000000000000, -0.000000000000000000 ) ) ;
#1769=ORIENTED_EDGE ( 'NONE', *, *, #50561, .T. ) ;
#1770=ORIENTED_EDGE ( 'NONE', *, *, #13048, .F. ) ;
#1771=CARTESIAN_POINT ( 'NONE',  ( 9.827939172326081163, 6.382931149346556587, 42.09375525668145457 ) ) ;
#1774=CARTESIAN_POINT ( 'NONE',  ( 63.98689050258324329, 13.93365232918668006, 71.61000602743803256 ) ) ;
#1778=CARTESIAN_POINT ( 'NONE',  ( -142.9728934044261734, 58.82891228489261692, -72.87700524141401104 ) ) ;
#1779=CARTESIAN_POINT ( 'NONE',  ( 92.21267147730743829, 21.40196534721318500, 15.39891977708759008 ) ) ;
#1780=EDGE_CURVE ( 'NONE', #45155, #31339, #43825, .T. ) ;
#1781=DIRECTION ( 'NONE',  ( -0.8160245890732938934, -0.5780171883497599028, 0.000000000000000000 ) ) ;
#1789=CARTESIAN_POINT ( 'NONE',  ( 62.71085615297809568, 13.63476094311646492, 83.50115473030093938 ) ) ;
#1792=CARTESIAN_POINT ( 'NONE',  ( -180.0094637318086939, 96.72611451757710199, -45.19277143581986422 ) ) ;
#1793=CARTESIAN_POINT ( 'NONE',  ( -180.5668408223793904, 97.41302302526328560, -95.00000000000133582 ) ) ;
#1794=CARTESIAN_POINT ( 'NONE',  ( 156.5909039492009640, 56.96742803863245541, 71.25401806271710825 ) ) ;
#1796=CARTESIAN_POINT ( 'NONE',  ( 127.2397149628677937, 37.56999625068102233, -66.79971066083803066 ) ) ;
#1798=CARTESIAN_POINT ( 'NONE',  ( 141.3036441389950539, 47.31002705502925920, -71.40782174165585161 ) ) ;
#1799=CARTESIAN_POINT ( 'NONE',  ( -85.35521056349260505, 26.07297753498038873, 94.99999999999866418 ) ) ;
#1800=ORIENTED_EDGE ( 'NONE', *, *, #68219, .F. ) ;
#1801=CARTESIAN_POINT ( 'NONE',  ( -150.5993571094983281, 66.43939758484179947, -49.73612197178368177 ) ) ;
#1802=CARTESIAN_POINT ( 'NONE',  ( -2.874437057892789138, 6.618922960888051321, -75.41744632663154846 ) ) ;
#1803=CARTESIAN_POINT ( 'NONE',  ( -38.69449158134467837, 11.92067517118077014, 35.75389334926249063 ) ) ;
#1805=CARTESIAN_POINT ( 'NONE',  ( -173.1211646369891355, 87.12891641440857882, -49.71195716475001092 ) ) ;
#1807=CARTESIAN_POINT ( 'NONE',  ( -14.96764630465879797, 7.461781624211967667, -94.16342404306476510 ) ) ;
#1811=CARTESIAN_POINT ( 'NONE',  ( 164.8471526211111211, 63.62172173173269130, 11.44683124855694523 ) ) ;
#1814=CARTESIAN_POINT ( 'NONE',  ( -97.88021438939453844, 31.71889184683102059, -36.42215870048158166 ) ) ;
#1815=ORIENTED_EDGE ( 'NONE', *, *, #68701, .T. ) ;
#1817=CARTESIAN_POINT ( 'NONE',  ( 80.15818551272217007, 18.36718314243333694, -66.34257447059830781 ) ) ;
#1819=DIRECTION ( 'NONE',  ( 0.000000000000000000, 0.000000000000000000, 1.000000000000000000 ) ) ;
#1821=FACE_OUTER_BOUND ( 'NONE', #57597, .T. ) ;
#1823=CARTESIAN_POINT ( 'NONE',  ( -118.3948752128398922, 42.92869324237092599, -15.27178645307563798 ) ) ;
#1828=CARTESIAN_POINT ( 'NONE',  ( 174.1364721914476661, 71.85829564941441561, 60.81373415767276924 ) ) ;
#1831=CARTESIAN_POINT ( 'NONE',  ( -165.6215009671260816, 80.58889799860445180, 65.48035359524065768 ) ) ;
#1833=CARTESIAN_POINT ( 'NONE',  ( -168.1811549361196967, 83.25427431521136157, -21.01567069218833694 ) ) ;
#1836=VERTEX_POINT ( 'NONE', #54735 ) ;
#1837=CARTESIAN_POINT ( 'NONE',  ( 94.06416612695406343, 23.16920323269611970, 11.38599088637463019 ) ) ;
#1839=VECTOR ( 'NONE', #27527, 1000.000000000000000 ) ;
#1840=CARTESIAN_POINT ( 'NONE',  ( -190.6985136298601731, 109.1272424661242582, 94.99999999999866418 ) ) ;
#1842=CARTESIAN_POINT ( 'NONE',  ( -173.1211646369891355, -170.0000000000000000, 11.47714401617735902 ) ) ;
#1843=CARTESIAN_POINT ( 'NONE',  ( 212.1535111375854683, 117.1635556319084657, -16.15046538589425751 ) ) ;
#1844=FACE_BOUND ( 'NONE', #16370, .T. ) ;
#1846=CARTESIAN_POINT ( 'NONE',  ( -62.48965350618343706, 16.80247907725181378, -41.71376395946558091 ) ) ;
#1847=EDGE_CURVE ( 'NONE', #43438, #48157, #42746, .T. ) ;
#1855=CARTESIAN_POINT ( 'NONE',  ( -47.60266343315662851, 13.84328785304053966, 65.66110071374279755 ) ) ;
#1856=CARTESIAN_POINT ( 'NONE',  ( -177.5100621450479252, 93.70693725195826573, 5.377500373651478149 ) ) ;
#1857=CARTESIAN_POINT ( 'NONE',  ( 211.7357196141372242, 118.3691710715567211, 66.16139203830061888 ) ) ;
#1858=CARTESIAN_POINT ( 'NONE',  ( 83.37786665291105237, 18.33670623396829669, -63.39026651841162163 ) ) ;
#1864=ORIENTED_EDGE ( 'NONE', *, *, #9538, .T. ) ;
#1866=CARTESIAN_POINT ( 'NONE',  ( -62.06231780744543869, 17.72446026058425517, -13.19249544724704037 ) ) ;
#1867=FACE_OUTER_BOUND ( 'NONE', #43871, .T. ) ;
#1870=DIRECTION ( 'NONE',  ( -0.000000000000000000, 1.000000000000000000, -0.000000000000000000 ) ) ;
#1872=CARTESIAN_POINT ( 'NONE',  ( -155.5977325361978103, 70.88311713755700794, -64.77305499973000735 ) ) ;
#1873=CARTESIAN_POINT ( 'NONE',  ( 67.93154431625912082, 14.90489441944787252, 4.782582000548346812 ) ) ;
#1875=ORIENTED_EDGE ( 'NONE', *, *, #20675, .F. ) ;
#1881=CARTESIAN_POINT ( 'NONE',  ( -133.0921934900200370, 52.65587531157186874, -13.44671944861685908 ) ) ;
#1886=ORIENTED_EDGE ( 'NONE', *, *, #48178, .F. ) ;
#1892=CARTESIAN_POINT ( 'NONE',  ( -48.04019567818505010, 12.91272349839804789, -13.20040436305664855 ) ) ;
#1893=CARTESIAN_POINT ( 'NONE',  ( 102.7425154123292543, 25.56407025871219574, -16.81959381298093348 ) ) ;
#1895=CARTESIAN_POINT ( 'NONE',  ( 201.5903370237274714, 102.1785392640257868, 3.023677376802185179 ) ) ;
#1896=CARTESIAN_POINT ( 'NONE',  ( 197.9945392102239055, 99.19564887483076632, 87.01074304022465356 ) ) ;
#1898=CARTESIAN_POINT ( 'NONE',  ( -78.19460645047365688, 22.14203592077027594, -76.96000122218154615 ) ) ;
#1899=CARTESIAN_POINT ( 'NONE',  ( -13.47680110791657881, 7.324966777230639714, 32.66010570199217256 ) ) ;
#1901=AXIS2_PLACEMENT_3D ( 'NONE', #15705, #25241, #62867 ) ;
#1907=CARTESIAN_POINT ( 'NONE',  ( -38.73578281104377652, 11.92878435305931539, 89.64055695031605353 ) ) ;
#1911=DIRECTION ( 'NONE',  ( 0.000000000000000000, 0.000000000000000000, 1.000000000000000000 ) ) ;
#1912=CARTESIAN_POINT ( 'NONE',  ( 110.2429982417149574, -170.0000000000000000, -50.92243756565370916 ) ) ;
#1914=VERTEX_POINT ( 'NONE', #24823 ) ;
#1917=LINE ( 'NONE', #33223, #50699 ) ;
#1920=EDGE_CURVE ( 'NONE', #25401, #25095, #25945, .T. ) ;
#1924=CARTESIAN_POINT ( 'NONE',  ( 197.3064269725219617, 98.33232022113060111, 64.86617095098992536 ) ) ;
#1925=ORIENTED_EDGE ( 'NONE', *, *, #34314, .T. ) ;
#1926=CARTESIAN_POINT ( 'NONE',  ( -55.05276343752909440, 15.72344139423347364, -62.06087458892354647 ) ) ;
#1927=CARTESIAN_POINT ( 'NONE',  ( 198.2588776805010298, 99.52972231602372233, -74.52680556020536073 ) ) ;
#1929=CARTESIAN_POINT ( 'NONE',  ( -2.873329055852805514, 7.626065826870670250, -48.57246868976042720 ) ) ;
#1930=CARTESIAN_POINT ( 'NONE',  ( 109.7774723066848281, 28.66666416591278477, 2.766663615273642574 ) ) ;
#1931=CARTESIAN_POINT ( 'NONE',  ( -170.0785278435570547, 83.80419503909187995, -89.03350163840394771 ) ) ;
#1933=FACE_BOUND ( 'NONE', #29391, .T. ) ;
#1934=CARTESIAN_POINT ( 'NONE',  ( -189.2641795714223178, 107.1238410236401677, 91.36523946422995834 ) ) ;
#1936=EDGE_CURVE ( 'NONE', #11965, #32966, #17681, .T. ) ;
#1940=CARTESIAN_POINT ( 'NONE',  ( -133.3392045760936355, 51.59583146030202983, -70.31251124416750997 ) ) ;
#1941=CARTESIAN_POINT ( 'NONE',  ( 133.8566784816069628, 41.42467568809806977, -62.86786152285933582 ) ) ;
#1947=CARTESIAN_POINT ( 'NONE',  ( 188.3602976857901865, 86.28604666859746430, 92.35901500848406442 ) ) ;
#1951=CARTESIAN_POINT ( 'NONE',  ( 175.8855729601531550, 73.50624012737691260, -49.15246532231710574 ) ) ;
#1952=CARTESIAN_POINT ( 'NONE',  ( 149.9683128897950155, 53.28564708287392193, 37.43972384951239718 ) ) ;
#1955=CYLINDRICAL_SURFACE ( 'NONE', #41330, 7.500000000000013323 ) ;
#1956=CARTESIAN_POINT ( 'NONE',  ( -175.1920326508033270, 89.46239303019292777, 4.256113626765591462 ) ) ;
#1957=CARTESIAN_POINT ( 'NONE',  ( -71.41745561414268195, 19.69148172991712542, -40.62644917380843168 ) ) ;
#1958=CARTESIAN_POINT ( 'NONE',  ( -102.2801239173131194, -170.0000000000000000, 18.67452391595144334 ) ) ;
#1959=CARTESIAN_POINT ( 'NONE',  ( -30.94745021534356155, 10.53010394565407459, -8.472646774738157305 ) ) ;
#1960=CARTESIAN_POINT ( 'NONE',  ( -189.2346268516247676, 107.0830361517165130, 38.63455055429937346 ) ) ;
#1963=CARTESIAN_POINT ( 'NONE',  ( -75.65611349188962720, 22.26947559308019464, 4.200113054923877876 ) ) ;
#1964=CARTESIAN_POINT ( 'NONE',  ( 46.84183314611287585, 9.494161546644493299, -42.14055136037359972 ) ) ;
#1966=CARTESIAN_POINT ( 'NONE',  ( -189.8133172329396814, 107.8858115918112901, 94.99999999999866418 ) ) ;
#1968=CARTESIAN_POINT ( 'NONE',  ( 80.17205177205136124, 17.31791394718354482, -47.14471772045799014 ) ) ;
#1970=CARTESIAN_POINT ( 'NONE',  ( -145.3279998500303520, 60.71393190715793509, 58.83337766670971547 ) ) ;
#1972=CARTESIAN_POINT ( 'NONE',  ( 80.73462811483979351, 18.54763808182592300, 32.54810887579326817 ) ) ;
#1975=CARTESIAN_POINT ( 'NONE',  ( -119.2982054035570769, 42.30181775808004119, 61.38488466982619940 ) ) ;
#1977=CARTESIAN_POINT ( 'NONE',  ( 43.35536254672136636, 9.973606330917816010, 4.191193481081563199 ) ) ;
#1978=CARTESIAN_POINT ( 'NONE',  ( -180.0094637318086370, 96.72611451757705936, -18.34822084535621300 ) ) ;
#1980=ORIENTED_EDGE ( 'NONE', *, *, #53959, .F. ) ;
#1983=B_SPLINE_CURVE_WITH_KNOTS ( 'NONE', 3,
 ( #43560, #49173, #65032, #65387, #16830, #38946, #1014, #22464, #17174, #11909, #49526, #63991, #5251, #26710, #48141, #21420, #42863, #64333, #10866, #13316, #66448, #28437, #28799, #13649, #17534, #6984, #55161, #8027, #40382, #7343, #39006, #55515, #50590, #49889, #60450, #1712, #2411, #45666, #35103, #67144, #12266, #56558, #18235, #66098, #23174, #50941 ),
 .UNSPECIFIED., .F., .F.,
 ( 4, 2, 2, 2, 2, 2, 2, 2, 2, 2, 2, 2, 2, 2, 2, 2, 2, 2, 2, 2, 2, 2, 4 ),
 ( 0.000000000000000000, 0.001615199098318991942, 0.003230398196637983884, 0.004037997745797491239, 0.004845597294956999028, 0.006460796393275994656, 0.007268395942435511986, 0.008075995491595029316, 0.009691194589914013668, 0.01049879413907353967, 0.01130639368823306568, 0.01211399323739259168, 0.01292159278655211595, 0.01453679188487112459, 0.01615199098319013496, 0.01695959053234963321, 0.01776719008150913146, 0.01938238917982806203, 0.02099758827814698914, 0.02180518782730647698, 0.02261278737646596829, 0.02422798647478494050, 0.02584318557310391617 ),
 .UNSPECIFIED. ) ;
#1984=CARTESIAN_POINT ( 'NONE',  ( 43.97326221476412655, 9.047815246749992824, 43.37997826269698010 ) ) ;
#1985=CARTESIAN_POINT ( 'NONE',  ( 197.3059626281005592, 96.72682679064189415, -15.67053974981288000 ) ) ;
#1989=CARTESIAN_POINT ( 'NONE',  ( 181.0840389613909736, -170.0000000000000000, -78.06960825634331513 ) ) ;
#1990=CARTESIAN_POINT ( 'NONE',  ( -76.78104518372332166, 22.68568622761702969, -76.73470982633753579 ) ) ;
#1991=CIRCLE ( 'NONE', #26677, 243.4957430088094839 ) ;
#1992=CARTESIAN_POINT ( 'NONE',  ( -102.2801239173131052, 32.78103895658058065, 72.36362509687883460 ) ) ;
#1993=CARTESIAN_POINT ( 'NONE',  ( -25.81763596640061209, 8.735969132042866292, -47.78813171631949785 ) ) ;
#2000=CARTESIAN_POINT ( 'NONE',  ( 15.78827728214693416, -170.0000000000000000, -96.70804527961315955 ) ) ;
#2002=CARTESIAN_POINT ( 'NONE',  ( 126.4219470349616188, 38.26519385429183018, 38.03294307216089720 ) ) ;
#2006=CARTESIAN_POINT ( 'NONE',  ( -98.67557579989349392, 32.10670856967971076, -22.26450473806611541 ) ) ;
#2007=CARTESIAN_POINT ( 'NONE',  ( 39.40195752203892710, 8.409560354027384221, 71.75838489642698903 ) ) ;
#2011=CARTESIAN_POINT ( 'NONE',  ( 62.52762183777206673, 13.59210632617624803, 71.65751152968498161 ) ) ;
#2013=CARTESIAN_POINT ( 'NONE',  ( -15.07533778868020313, 8.482826962130836534, 12.70726733519779827 ) ) ;
#2016=CARTESIAN_POINT ( 'NONE',  ( 132.9557829392755082, 42.05591979570419880, -24.13845282381304003 ) ) ;
#2023=CARTESIAN_POINT ( 'NONE',  ( -175.2564835000419805, 89.53548519733848821, 84.80368869902895312 ) ) ;
#2027=B_SPLINE_CURVE_WITH_KNOTS ( 'NONE', 3,
 ( #27187, #31785, #68718, #15950, #37745, #48618, #25834, #37395, #59190, #37061, #47262, #63457, #58499, #26164, #47596, #69054, #38447, #34222, #6441, #28949, #17695, #59535, #2214, #27534, #44772, #22610, #11352, #64834, #59884, #66249, #12762, #7131, #819, #60247, #33176, #28592, #1872, #49677, #65180, #44055, #18040, #60943, #11703, #12065, #33870, #55666, #23328, #39492 ),
 .UNSPECIFIED., .F., .F.,
 ( 4, 2, 2, 2, 2, 2, 2, 2, 2, 2, 2, 2, 2, 2, 2, 2, 2, 2, 2, 2, 2, 2, 2, 4 ),
 ( 0.02698595842317763963, 0.02784423243973405820, 0.02870250645629048025, 0.03041905448940328272, 0.03127732850595967007, 0.03213560252251606436, 0.03385215055562883907, 0.03471042457218519173, 0.03556869858874154439, 0.03728524662185422889, 0.03814352063841059542, 0.03900179465496696196, 0.03986006867152332850, 0.04071834268807969504, 0.04157661670463606157, 0.04243489072119242811, 0.04415143875430510567, 0.04500971277086143058, 0.04586798678741776936, 0.04758453482053040529, 0.04930108285364304122, 0.05101763088675567714, 0.05273417891986832001, 0.05445072695298095594 ),
 .UNSPECIFIED. ) ;
#2029=CARTESIAN_POINT ( 'NONE',  ( -0.9897066053608880587, 7.549089325901770842, -72.85837384025812469 ) ) ;
#2033=CARTESIAN_POINT ( 'NONE',  ( 163.6472217856825466, 63.92779681097861300, -93.03927632148491966 ) ) ;
#2034=CARTESIAN_POINT ( 'NONE',  ( 197.2197025888162329, 96.62026035493822462, -44.48619938706712418 ) ) ;
#2040=VERTEX_POINT ( 'NONE', #64870 ) ;
#2041=CARTESIAN_POINT ( 'NONE',  ( 63.01563776193091826, 12.67277567978498176, 29.81296093922127710 ) ) ;
#2044=AXIS2_PLACEMENT_3D ( 'NONE', #60547, #2852, #1819 ) ;
#2045=CARTESIAN_POINT ( 'NONE',  ( -73.79615177260652104, 20.52570924097571492, -10.04630520512574599 ) ) ;
#2051=CARTESIAN_POINT ( 'NONE',  ( -74.39861643904069410, 21.81123504700007487, -36.44343603524747266 ) ) ;
#2054=CARTESIAN_POINT ( 'NONE',  ( 175.5371852679042775, 74.56478031408204288, -92.34861066285949960 ) ) ;
#2055=EDGE_CURVE ( 'NONE', #23050, #32357, #4146, .T. ) ;
#2056=CARTESIAN_POINT ( 'NONE',  ( 138.1901928158493433, 45.29454828899442731, 43.14961434377592298 ) ) ;
#2057=CARTESIAN_POINT ( 'NONE',  ( -178.2448732545370831, 94.58403736950705820, 43.81829304766783650 ) ) ;
#2058=CARTESIAN_POINT ( 'NONE',  ( 132.0249343950657135, 41.49728247212333088, 71.18673643823439079 ) ) ;
#2059=CARTESIAN_POINT ( 'NONE',  ( 19.11382977197791533, 7.636807742668411336, 71.09960622632753768 ) ) ;
#2066=CARTESIAN_POINT ( 'NONE',  ( -94.85325982401134581, 29.16540057079190262, 92.80390509532465160 ) ) ;
#2067=CARTESIAN_POINT ( 'NONE',  ( -142.0251973982164770, 58.08401473564112649, 37.63374177329165349 ) ) ;
#2070=CARTESIAN_POINT ( 'NONE',  ( -78.19438069111006939, 23.21811806230638098, -23.27090004125422240 ) ) ;
#2071=ORIENTED_EDGE ( 'NONE', *, *, #14595, .T. ) ;
#2072=CARTESIAN_POINT ( 'NONE',  ( 82.94943325692331371, 18.19803534719805782, 57.51694778251922457 ) ) ;
#2076=CARTESIAN_POINT ( 'NONE',  ( 31.99894129856763314, 7.561773404408285160, 36.18667756713777806 ) ) ;
#2083=DIRECTION ( 'NONE',  ( -0.000000000000000000, 1.000000000000000000, -0.000000000000000000 ) ) ;
#2087=CARTESIAN_POINT ( 'NONE',  ( 162.0862735437574713, 62.63196145447158614, -76.39940893092133933 ) ) ;
#2089=B_SPLINE_CURVE_WITH_KNOTS ( 'NONE', 3,
 ( #49248, #16899, #65454, #54881, #66511, #60164, #1081, #44328, #22533, #28149, #66172, #18303, #28511, #39761, #1792, #17962, #54171, #11272, #39411, #12682, #65815, #34148, #11983, #55584, #28869, #17609, #38718, #5993, #22885, #39075, #43972, #22187, #17248, #33454, #50320, #735, #49596, #2138, #1428, #48892, #32741, #43627, #38360, #59805 ),
 .UNSPECIFIED., .F., .F.,
 ( 4, 2, 2, 2, 2, 2, 2, 2, 2, 2, 2, 2, 2, 2, 2, 2, 2, 2, 2, 2, 2, 4 ),
 ( 0.02908143158676660886, 0.03095422299093871649, 0.03282701439511082064, 0.03469980579928292480, 0.03657259720345503590, 0.03844538860762714005, 0.04031818001179924421, 0.04125457571388527200, 0.04219097141597129980, 0.04312736711805732759, 0.04359556496910033108, 0.04406376282014333456, 0.04500015852222933460, 0.04593655422431534852, 0.04687294992640135549, 0.04780934562848735553, 0.04968213703265940417, 0.05155492843683144588, 0.05342771984100349453, 0.05530051124517554317, 0.05717330264934758488, 0.05904609405351963353 ),
 .UNSPECIFIED. ) ;
#2091=CARTESIAN_POINT ( 'NONE',  ( 15.78827728214693416, 6.500811158483322139, -89.20804527961313113 ) ) ;
#2094=LINE ( 'NONE', #44643, #47644 ) ;
#2095=DIRECTION ( 'NONE',  ( 0.000000000000000000, 0.000000000000000000, 1.000000000000000000 ) ) ;
#2098=CARTESIAN_POINT ( 'NONE',  ( 151.8005253678162489, 54.62151558044536159, -75.40480181429586537 ) ) ;
#2099=CARTESIAN_POINT ( 'NONE',  ( -34.74312654625183683, 10.15703162223800859, 30.97899339878855329 ) ) ;
#2100=CARTESIAN_POINT ( 'NONE',  ( 141.0804878838241336, 45.96076546397620888, -41.43773930307789044 ) ) ;
#2103=EDGE_CURVE ( 'NONE', #5375, #39717, #50083, .T. ) ;
#2104=EDGE_CURVE ( 'NONE', #69562, #64513, #40275, .T. ) ;
#2111=CARTESIAN_POINT ( 'NONE',  ( 140.6568134119880824, 46.88581307642903795, 87.51626415052055563 ) ) ;
#2112=CARTESIAN_POINT ( 'NONE',  ( -25.64812644094277871, 9.728246071458697131, -91.73551276297135360 ) ) ;
#2121=CARTESIAN_POINT ( 'NONE',  ( 163.1313205310725039, 63.49733392291058465, -11.85377922317074528 ) ) ;
#2122=CARTESIAN_POINT ( 'NONE',  ( 8.670103207226933506, 6.377073801252349128, 35.10160029233258427 ) ) ;
#2124=CARTESIAN_POINT ( 'NONE',  ( 65.62985354949972816, 14.32996029952553485, 71.19137513351442692 ) ) ;
#2125=CARTESIAN_POINT ( 'NONE',  ( 126.9829467593605301, 37.42601351122073083, -94.18273480071589177 ) ) ;
#2128=CARTESIAN_POINT ( 'NONE',  ( 163.1370549780984049, 63.50181104276887822, -48.56306423650217852 ) ) ;
#2131=CARTESIAN_POINT ( 'NONE',  ( 159.6725804802005939, 59.38339663535511193, -36.44073469567691603 ) ) ;
#2132=ORIENTED_EDGE ( 'NONE', *, *, #52864, .T. ) ;
#2133=CARTESIAN_POINT ( 'NONE',  ( -95.20053778133910782, 30.43887292928076604, 8.646733277597450140 ) ) ;
#2134=B_SPLINE_CURVE_WITH_KNOTS ( 'NONE', 3,
 ( #66414, #27348, #48787, #982, #60415, #22430, #38609, #60051, #11873, #46657, #40001, #40683, #24535, #68134, #61458, #14315, #29796, #9038, #29442, #50904, #8350, #45971, #61793, #35774, #18548, #8698, #35420, #13614, #67436, #19581, #30485, #56520, #66755, #57223, #50556, #35070, #45274, #51935, #13281, #41040, #30153, #3751, #62142, #51262, #67784, #2374, #23832, #25223 ),
 .UNSPECIFIED., .F., .F.,
 ( 4, 2, 2, 2, 2, 2, 2, 2, 2, 2, 2, 2, 2, 2, 2, 2, 2, 2, 2, 2, 2, 2, 2, 4 ),
 ( 0.02698595842317764310, 0.02784423243973403739, 0.02870250645629042821, 0.03041905448940312312, 0.03127732850595946884, 0.03213560252251581456, 0.03385215055562851294, 0.03471042457218486560, 0.03556869858874121132, 0.03728524662185391664, 0.03814352063841026236, 0.03900179465496660114, 0.03986006867152294686, 0.04071834268807929258, 0.04157661670463563830, 0.04243489072119198402, 0.04415143875430466158, 0.04500971277086100730, 0.04586798678741735302, 0.04758453482053006528, 0.04930108285364277754, 0.05101763088675548286, 0.05273417891986818817, 0.05445072695298090043 ),
 .UNSPECIFIED. ) ;
#2136=ADVANCED_FACE ( 'NONE', ( #46888 ), #35297, .F. ) ;
#2137=CARTESIAN_POINT ( 'NONE',  ( 31.95163392065794739, 8.568192436298495807, 36.42221770829554117 ) ) ;
#2138=CARTESIAN_POINT ( 'NONE',  ( -176.3856149167966407, 92.38076834121984859, -35.44546595752847651 ) ) ;
#2140=CARTESIAN_POINT ( 'NONE',  ( 152.8558173410469294, 54.14978343559392471, 69.68634218349458820 ) ) ;
#2141=CARTESIAN_POINT ( 'NONE',  ( 128.4224537826253822, 38.23837035195744960, -65.17599223679393106 ) ) ;
#2143=CARTESIAN_POINT ( 'NONE',  ( 140.4769819293526893, 46.76840769395180786, -73.90161371371723931 ) ) ;
#2146=CARTESIAN_POINT ( 'NONE',  ( -154.7826623253029936, 70.14150242829518334, -47.64975679370859751 ) ) ;
#2148=CARTESIAN_POINT ( 'NONE',  ( -33.38294402636582703, 10.93918551420889607, 44.97681826711176001 ) ) ;
#2149=CARTESIAN_POINT ( 'NONE',  ( -167.9889421625799741, 81.59140042431236850, -47.70137618540091040 ) ) ;
#2152=CARTESIAN_POINT ( 'NONE',  ( -48.57297291660697880, 13.03920345822339044, -73.36987217233711078 ) ) ;
#2154=CARTESIAN_POINT ( 'NONE',  ( 208.5889601154909201, 111.8333159387241835, -50.25120141670069529 ) ) ;
#2157=CARTESIAN_POINT ( 'NONE',  ( 164.9559213734325169, 63.71338633026442722, 10.60842315000168234 ) ) ;
#2158=ADVANCED_FACE ( 'NONE', ( #31404 ), #64092, .F. ) ;
#2160=CARTESIAN_POINT ( 'NONE',  ( -95.21085197937820510, 30.44372064875429373, -39.95763492157845320 ) ) ;
#2165=CARTESIAN_POINT ( 'NONE',  ( 45.34143264614439772, 9.256465810451185661, 59.67216321036798377 ) ) ;
#2173=CARTESIAN_POINT ( 'NONE',  ( 63.01563776193091826, -170.0000000000000000, 64.15751152968499582 ) ) ;
#2174=CARTESIAN_POINT ( 'NONE',  ( 173.5837434292114096, 71.34409607026155697, 63.36509229591028003 ) ) ;
#2176=CARTESIAN_POINT ( 'NONE',  ( 108.3753929817421096, 29.13179266688723956, 71.23489859707926541 ) ) ;
#2177=CARTESIAN_POINT ( 'NONE',  ( -167.6524579626395166, 82.69702609844094354, -20.50584711148702510 ) ) ;
#2178=AXIS2_PLACEMENT_3D ( 'NONE', #46569, #25483, #26158 ) ;
#2184=CARTESIAN_POINT ( 'NONE',  ( 104.7227067006896561, 27.50728936118535373, -48.52285352452530276 ) ) ;
#2185=CARTESIAN_POINT ( 'NONE',  ( -8.314575874103551811, 6.922894809783093351, 56.96013162991087597 ) ) ;
#2186=CARTESIAN_POINT ( 'NONE',  ( -86.06489347855099936, 25.27905598459107139, -17.02718089029554704 ) ) ;
#2189=FACE_BOUND ( 'NONE', #62448, .T. ) ;
#2195=DIRECTION ( 'NONE',  ( 0.000000000000000000, 0.000000000000000000, 1.000000000000000000 ) ) ;
#2196=CARTESIAN_POINT ( 'NONE',  ( 207.4610690199662031, 111.9701171077052066, 70.53645963308595412 ) ) ;
#2198=CARTESIAN_POINT ( 'NONE',  ( 82.34195123877069022, 18.00239921638039675, -64.00762485161624227 ) ) ;
#2199=ORIENTED_EDGE ( 'NONE', *, *, #61849, .F. ) ;
#2205=CARTESIAN_POINT ( 'NONE',  ( -83.51052366780672287, 24.22613130369187218, -63.72902832609224077 ) ) ;
#2206=CARTESIAN_POINT ( 'NONE',  ( -56.96436614829622158, 16.24647150911285465, -23.12810583680024479 ) ) ;
#2207=DIRECTION ( 'NONE',  ( 0.000000000000000000, 0.000000000000000000, 1.000000000000000000 ) ) ;
#2211=CARTESIAN_POINT ( 'NONE',  ( 45.76405797021009647, 10.34101216371941945, 68.23763830739490288 ) ) ;
#2214=CARTESIAN_POINT ( 'NONE',  ( -156.7435307435793845, 71.93726016406964163, -71.14971855428032654 ) ) ;
#2215=CARTESIAN_POINT ( 'NONE',  ( 66.73467315386238852, 14.60276727483218728, 16.99948571587159307 ) ) ;
#2219=CARTESIAN_POINT ( 'NONE',  ( -47.80251179448168131, 13.89045662648309154, 12.95678486719901912 ) ) ;
#2220=CARTESIAN_POINT ( 'NONE',  ( -130.5904357464317513, 50.88938808445628581, -9.701552378028926782 ) ) ;
#2221=CARTESIAN_POINT ( 'NONE',  ( -154.4602569667544856, 69.84957963938288117, -90.35317075896763583 ) ) ;
#2222=CARTESIAN_POINT ( 'NONE',  ( 116.0773578185793724, 31.67580513411751753, -21.31700010224128050 ) ) ;
#2223=B_SPLINE_CURVE_WITH_KNOTS ( 'NONE', 3,
 ( #69474, #64199, #16008, #53634, #43772, #37124, #17039, #58566, #49042, #31852, #69122, #53285, #37459, #883, #11773, #11074, #21631, #58916, #27251, #43078, #5458, #48340, #10731, #48011, #16360, #59262, #20950, #48686, #530, #43426, #64904, #38508, #38156, #59595, #11415, #59953, #34293, #1227, #38872, #60315, #6849, #12481, #18454 ),
 .UNSPECIFIED., .F., .F.,
 ( 4, 2, 2, 2, 2, 2, 2, 2, 2, 2, 2, 2, 1, 2, 2, 2, 2, 2, 2, 2, 2, 4 ),
 ( 0.02379577142314830487, 0.02527778373276535345, 0.02601878988757387254, 0.02675979604238239162, 0.02824180835199942979, 0.02972382066161646449, 0.03046482681642496276, 0.03120583297123346103, 0.03268784528085046104, 0.03416985759046747145, 0.03565186990008447493, 0.03639287605489297667, 0.03713388220970148534, 0.03787488836450998708, 0.03861589451931848882, 0.04009790682893545760, 0.04157991913855242638, 0.04306193144816939516, 0.04380293760297787609, 0.04454394375778636395, 0.04602595606740334661, 0.04750796837702032926 ),
 .UNSPECIFIED. ) ;
#2225=CARTESIAN_POINT ( 'NONE',  ( 85.37210774275131087, 18.99570166535387727, 83.50014660744342621 ) ) ;
#2226=CARTESIAN_POINT ( 'NONE',  ( -180.5668408223793904, -170.0000000000000000, -95.00000000000133582 ) ) ;
#2231=DIRECTION ( 'NONE',  ( 0.000000000000000000, -1.000000000000000000, 0.000000000000000000 ) ) ;
#2232=CARTESIAN_POINT ( 'NONE',  ( 181.0840389613909736, 80.03940679743416808, 2.464043515047717570 ) ) ;
#2233=CARTESIAN_POINT ( 'NONE',  ( -132.6811329440527061, -170.0000000000000000, 94.99999999999866418 ) ) ;
#2234=CARTESIAN_POINT ( 'NONE',  ( 105.4375968828853729, 26.72149058755202944, -10.81446374568332125 ) ) ;
#2235=CARTESIAN_POINT ( 'NONE',  ( 197.2197025888162045, 96.62026035493816778, 9.202901793860229773 ) ) ;
#2237=CARTESIAN_POINT ( 'NONE',  ( 202.3256005306661223, 104.8219372317010141, 83.25897611976662915 ) ) ;
#2239=CARTESIAN_POINT ( 'NONE',  ( -72.78737098446268305, 20.16853011470087864, -74.14376160244967195 ) ) ;
#2240=CARTESIAN_POINT ( 'NONE',  ( -14.92903005859421128, 7.458185427130750611, 40.03400615406091134 ) ) ;
#2242=CARTESIAN_POINT ( 'NONE',  ( 12.68603346975295132, 7.427591953486040843, -9.341698521599035132 ) ) ;
#2244=ADVANCED_FACE ( 'NONE', ( #10616 ), #59149, .F. ) ;
#2247=CARTESIAN_POINT ( 'NONE',  ( 66.30230369578302430, 14.49551544185123753, -23.12206507395049826 ) ) ;
#2248=CARTESIAN_POINT ( 'NONE',  ( 186.0827296088606886, 85.28826835108064586, -64.97338836740433976 ) ) ;
#2249=CARTESIAN_POINT ( 'NONE',  ( -37.70624945308918541, 11.72883674540529242, 87.27307330636284632 ) ) ;
#2255=CARTESIAN_POINT ( 'NONE',  ( 139.1306635769909690, 45.89653412152168244, -22.01677782650911652 ) ) ;
#2259=CARTESIAN_POINT ( 'NONE',  ( -14.94265033805045562, 7.459411036484909552, 8.355115657452357070 ) ) ;
#2263=CARTESIAN_POINT ( 'NONE',  ( -188.6739852773920347, 108.2139733222100517, 40.12819175787510062 ) ) ;
#2267=CARTESIAN_POINT ( 'NONE',  ( -102.2801239173131194, -170.0000000000000000, 64.86362509687882039 ) ) ;
#2268=CARTESIAN_POINT ( 'NONE',  ( -61.77164219855452387, 17.63686644795249236, -66.19097850481081480 ) ) ;
#2269=CARTESIAN_POINT ( 'NONE',  ( 199.2049631873263138, 100.7347227143600037, -65.55741041441223160 ) ) ;
#2273=LINE ( 'NONE', #23023, #26383 ) ;
#2275=FACE_BOUND ( 'NONE', #51080, .T. ) ;
#2276=EDGE_CURVE ( 'NONE', #17473, #12095, #34441, .T. ) ;
#2278=CARTESIAN_POINT ( 'NONE',  ( -4.725257700476002576, 6.708862164351558910, 71.29377542245961763 ) ) ;
#2279=ORIENTED_EDGE ( 'NONE', *, *, #15630, .F. ) ;
#2281=CARTESIAN_POINT ( 'NONE',  ( -125.8938041572051105, 46.49392987655492959, -76.75825448869764500 ) ) ;
#2286=VERTEX_POINT ( 'NONE', #66207 ) ;
#2287=CARTESIAN_POINT ( 'NONE',  ( -190.6985136298601731, 109.1272424661242582, 7.126870892829554549 ) ) ;
#2291=PLANE ( 'NONE',  #63395 ) ;
#2292=CARTESIAN_POINT ( 'NONE',  ( 154.0281735872262061, 56.28213428456460576, 43.57687635770160739 ) ) ;
#2300=CARTESIAN_POINT ( 'NONE',  ( 87.11228333101213650, 19.58587579906928511, -35.82156419891172305 ) ) ;
#2301=CARTESIAN_POINT ( 'NONE',  ( 141.2470358420065395, 46.06959063280891797, 11.47092469016289407 ) ) ;
#2302=EDGE_CURVE ( 'NONE', #1174, #36237, #24878, .T. ) ;
#2305=CARTESIAN_POINT ( 'NONE',  ( 113.8748103246145007, 30.59837980920002209, -36.84266853766591510 ) ) ;
#2307=CARTESIAN_POINT ( 'NONE',  ( -77.71801202538874520, 23.03755222122951452, 18.52846565512617971 ) ) ;
#2308=CARTESIAN_POINT ( 'NONE',  ( 40.38414441725700499, 8.538832720399529563, -35.66810678251472666 ) ) ;
#2310=CARTESIAN_POINT ( 'NONE',  ( -119.1443287577880739, 42.20738984040679043, 88.47138527478010417 ) ) ;
#2312=CARTESIAN_POINT ( 'NONE',  ( 79.19345177405118363, 17.01649702043280143, -42.31098989147414358 ) ) ;
#2315=CARTESIAN_POINT ( 'NONE',  ( -146.5268141329886191, 61.69196909035591148, 71.95141080427552538 ) ) ;
#2316=CARTESIAN_POINT ( 'NONE',  ( 83.38619203015943526, 19.39783821526630447, 30.43258577136558074 ) ) ;
#2318=CARTESIAN_POINT ( 'NONE',  ( 188.4389256074244372, 86.37278721358589451, -15.38304180145345867 ) ) ;
#2319=CARTESIAN_POINT ( 'NONE',  ( 139.2921620648436942, 44.80435067172500396, -21.86958038675194871 ) ) ;
#2320=CARTESIAN_POINT ( 'NONE',  ( 39.40195752203892710, 9.424259417798131366, 3.069283715499574239 ) ) ;
#2321=CARTESIAN_POINT ( 'NONE',  ( 16.62903674119167263, 7.535646975941353354, -89.24366362108607120 ) ) ;
#2327=CARTESIAN_POINT ( 'NONE',  ( 107.0471828278920441, 27.43080724084231647, 70.75761023996984989 ) ) ;
#2328=CARTESIAN_POINT ( 'NONE',  ( 164.4615316623334991, 63.29763980349832764, 61.02503964407276982 ) ) ;
#2329=CARTESIAN_POINT ( 'NONE',  ( -189.9638655956219964, 108.0957249433520673, 62.03588848252969967 ) ) ;
#2330=DIRECTION ( 'NONE',  ( -0.000000000000000000, 1.000000000000000000, -0.000000000000000000 ) ) ;
#2332=CARTESIAN_POINT ( 'NONE',  ( -108.6909373351217027, 36.15835109565442451, 60.93927029289248765 ) ) ;
#2336=VERTEX_POINT ( 'NONE', #32777 ) ;
#2337=ORIENTED_EDGE ( 'NONE', *, *, #28584, .T. ) ;
#2339=CARTESIAN_POINT ( 'NONE',  ( -71.16326860233392892, 19.60396142827894295, 91.85506027016724317 ) ) ;
#2341=B_SPLINE_CURVE_WITH_KNOTS ( 'NONE', 3,
 ( #56471, #55786, #30099, #35025, #29396, #2327, #13567, #56125, #46605, #68086, #61404, #50849, #24484, #19886, #45922, #41344, #19179, #62796, #7944, #8646, #13229, #40633, #3360, #8989, #2667, #34343, #24818, #46255, #40298, #40992, #45222, #18496, #24128, #67733, #7608, #62450, #66701, #39951, #14264, #35724, #57174, #30436, #29062, #50506 ),
 .UNSPECIFIED., .F., .F.,
 ( 4, 2, 2, 2, 2, 2, 2, 2, 2, 2, 2, 2, 2, 2, 2, 2, 2, 2, 2, 2, 2, 4 ),
 ( 0.000000000000000000, 0.001533942663855623412, 0.003067885327711246824, 0.004601827991566870453, 0.005368799323494680316, 0.006135770655422489311, 0.007669713319278136793, 0.008436684651205958799, 0.009203655983133782539, 0.01073759864698937277, 0.01150456997891716876, 0.01227154131084496475, 0.01303851264277275900, 0.01380548397470055325, 0.01533942663855618338, 0.01687336930241181004, 0.01840731196626744018, 0.01994125463012307031, 0.02070822596205088018, 0.02147519729397868657, 0.02300913995783433405, 0.02454308262168998500 ),
 .UNSPECIFIED. ) ;
#2343=CARTESIAN_POINT ( 'NONE',  ( -78.66644367742111399, 23.39876645725286153, -61.96000122218157458 ) ) ;
#2346=CARTESIAN_POINT ( 'NONE',  ( -95.88693721180811735, 30.76307528361166632, -11.74052076892611218 ) ) ;
#2347=CARTESIAN_POINT ( 'NONE',  ( 37.70762885381311236, 8.195134395012278361, 71.56854745327594003 ) ) ;
#2348=CARTESIAN_POINT ( 'NONE',  ( 32.05329076859800352, 7.567153360545789909, 89.56790089374254649 ) ) ;
#2352=CARTESIAN_POINT ( 'NONE',  ( -5.401648928593171028, 6.744888135494087500, -35.80373528830617857 ) ) ;
#2354=CARTESIAN_POINT ( 'NONE',  ( -189.3111515777349894, 107.1887855376296841, -41.02269173539261260 ) ) ;
#2356=LINE ( 'NONE', #23808, #45615 ) ;
#2357=CARTESIAN_POINT ( 'NONE',  ( 217.9999999999999716, 126.6235316737731580, 94.99999999999866418 ) ) ;
#2358=CARTESIAN_POINT ( 'NONE',  ( 127.4669243510812890, 38.85312661085428232, -12.71959053557455022 ) ) ;
#2362=CARTESIAN_POINT ( 'NONE',  ( -189.3111515777350462, 107.1887855376297125, -14.17814114492894184 ) ) ;
#2363=CARTESIAN_POINT ( 'NONE',  ( -34.74023699876256899, 11.17830703027882855, -49.56910944950720932 ) ) ;
#2365=CARTESIAN_POINT ( 'NONE',  ( -166.2425995121691642, 79.78465616981384301, 94.99999999999866418 ) ) ;
#2366=ORIENTED_EDGE ( 'NONE', *, *, #19208, .F. ) ;
#2367=CARTESIAN_POINT ( 'NONE',  ( -119.2982054035571338, 42.30181775808006961, -45.99331769202854758 ) ) ;
#2369=CARTESIAN_POINT ( 'NONE',  ( -0.5178428571329644070, 7.532057582089303871, -68.05658183845606857 ) ) ;
#2370=CARTESIAN_POINT ( 'NONE',  ( 164.9466788279801790, 65.02358717534978894, 91.30755230343568485 ) ) ;
#2372=CARTESIAN_POINT ( 'NONE',  ( 164.4555644730588710, 64.60768971797665472, -94.57351069396484888 ) ) ;
#2374=CARTESIAN_POINT ( 'NONE',  ( -150.3850953947692233, 66.25368649589884740, 45.68226874722795827 ) ) ;
#2375=CARTESIAN_POINT ( 'NONE',  ( 19.10216788411013411, 6.629360741291161041, -49.75156701922125535 ) ) ;
#2376=CARTESIAN_POINT ( 'NONE',  ( 115.7612476187723871, 32.64200929566223408, 15.36962448049462182 ) ) ;
#2378=B_SPLINE_CURVE_WITH_KNOTS ( 'NONE', 3,
 ( #44626, #17897, #61154, #8032, #56216, #49894, #34082, #45315, #55882, #22821, #60457, #12271, #1718, #61831, #2760, #18588, #33733, #12977, #12620, #23181, #7699, #7349, #40045, #39352, #34443, #2076, #55520, #1365, #65746, #28805, #6990, #24225, #45672, #29146, #67149, #50595, #50253, #18938, #40387, #34779, #2416, #39011, #13655, #23871, #60795 ),
 .UNSPECIFIED., .F., .F.,
 ( 4, 2, 2, 2, 2, 2, 2, 2, 1, 2, 2, 2, 2, 2, 2, 2, 2, 2, 2, 2, 2, 2, 4 ),
 ( 0.000000000000000000, 0.001470449819620651055, 0.002205674729430986882, 0.002940899639241323360, 0.004411349458861975499, 0.005881799278482627638, 0.007352249098103279777, 0.008087474007913614954, 0.008822698917723949263, 0.009557923827534283573, 0.01029314873734461962, 0.01176359855696526915, 0.01249882346677560346, 0.01323404837658594298, 0.01470449819620661507, 0.01543972310601695805, 0.01617494801582729930, 0.01764539783544796098, 0.01911584765506862613, 0.01985107256487894656, 0.02058629747468926699, 0.02205674729430991132, 0.02352719711393055912 ),
 .UNSPECIFIED. ) ;
#2379=CARTESIAN_POINT ( 'NONE',  ( -1.000020675113008961, 7.549072000771346325, -93.38318693586774089 ) ) ;
#2381=VERTEX_POINT ( 'NONE', #22569 ) ;
#2383=CARTESIAN_POINT ( 'NONE',  ( 174.2468109002382448, 73.34092405459588804, 39.90336194450533469 ) ) ;
#2384=ADVANCED_FACE ( 'NONE', ( #38397 ), #59837, .F. ) ;
#2385=CARTESIAN_POINT ( 'NONE',  ( 21.44031696305384571, 6.747195267824409370, -64.90930529496827717 ) ) ;
#2387=VERTEX_POINT ( 'NONE', #18333 ) ;
#2388=CYLINDRICAL_SURFACE ( 'NONE', #7245, 7.500000000000013323 ) ;
#2390=CARTESIAN_POINT ( 'NONE',  ( -23.95089599695169014, 9.496585844566148182, 37.22793919491487458 ) ) ;
#2394=CARTESIAN_POINT ( 'NONE',  ( 204.6977192012829505, 108.0580384837234931, -78.17048162308530834 ) ) ;
#2395=VECTOR ( 'NONE', #42182, 1000.000000000000000 ) ;
#2397=CARTESIAN_POINT ( 'NONE',  ( 136.7507824285649178, 44.38599729999916121, 43.93330792897594250 ) ) ;
#2400=CARTESIAN_POINT ( 'NONE',  ( 22.15926701483429895, 7.796117250416237709, 68.32426611714438991 ) ) ;
#2408=CARTESIAN_POINT ( 'NONE',  ( -34.51918258780364823, 10.11719938103012417, -49.65991457455191238 ) ) ;
#2409=DIRECTION ( 'NONE',  ( 0.000000000000000000, -0.000000000000000000, 1.000000000000000000 ) ) ;
#2410=CARTESIAN_POINT ( 'NONE',  ( -149.5074843970971301, 64.17983161892345834, 30.72082123989904900 ) ) ;
#2411=CARTESIAN_POINT ( 'NONE',  ( -130.2196570250629577, 49.40815211106350091, 58.81961367888054326 ) ) ;
#2412=CARTESIAN_POINT ( 'NONE',  ( -62.20000168511805327, 17.76605013184458315, 93.80264320643617282 ) ) ;
#2413=ORIENTED_EDGE ( 'NONE', *, *, #24190, .F. ) ;
#2416=CARTESIAN_POINT ( 'NONE',  ( 36.99625334683020839, 8.108440754877200618, 30.29321116345249720 ) ) ;
#2417=CARTESIAN_POINT ( 'NONE',  ( 84.74089592029041285, 19.84571403269345424, 56.79428774094038346 ) ) ;
#2418=CARTESIAN_POINT ( 'NONE',  ( 181.5127080940606845, 79.03904173130082711, 44.30859410551142474 ) ) ;
#2421=CARTESIAN_POINT ( 'NONE',  ( -118.3918229753715252, 42.92682904595257298, 64.45486351284331761 ) ) ;
#2422=CARTESIAN_POINT ( 'NONE',  ( -11.13714165684777768, 8.138643170880698108, -49.65174624528041392 ) ) ;
#2425=CARTESIAN_POINT ( 'NONE',  ( -104.3671396759760910, 33.85343629185614134, -88.98748543686591006 ) ) ;
#2429=CARTESIAN_POINT ( 'NONE',  ( -59.58556642339447507, 16.99097764963621060, 70.65714236767303191 ) ) ;
#2433=CARTESIAN_POINT ( 'NONE',  ( 151.6178224291901131, 54.48737267587417676, -65.77168945991468263 ) ) ;
#2434=CARTESIAN_POINT ( 'NONE',  ( -33.37566357177431087, 9.916833145467597532, 30.45442685525332038 ) ) ;
#2435=CARTESIAN_POINT ( 'NONE',  ( 140.4897729434289886, 45.57634363643750675, -39.98413189135570889 ) ) ;
#2436=EDGE_LOOP ( 'NONE', ( #28978, #59934, #27975, #24956 ) ) ;
#2438=CARTESIAN_POINT ( 'NONE',  ( -120.4586945679390482, 43.01762219615311267, 43.31108851025778250 ) ) ;
#2440=CARTESIAN_POINT ( 'NONE',  ( 36.98541457540711264, 9.120571655722415016, -9.158542404804654424 ) ) ;
#2443=CARTESIAN_POINT ( 'NONE',  ( -1.095583923122879888, 7.553030873957006897, 14.09065126040307270 ) ) ;
#2445=CARTESIAN_POINT ( 'NONE',  ( 126.8687677780346093, 38.51583040706892547, 93.44669519883952091 ) ) ;
#2455=CARTESIAN_POINT ( 'NONE',  ( 67.92995549349548412, 13.86623459444475337, 58.47094168735598174 ) ) ;
#2456=CARTESIAN_POINT ( 'NONE',  ( 138.2204650371259049, 44.12203217345472694, -64.24952538475335473 ) ) ;
#2462=EDGE_CURVE ( 'NONE', #66935, #36885, #51734, .T. ) ;
#2463=CARTESIAN_POINT ( 'NONE',  ( 8.336882341125877005, 6.376438415325264231, 36.53121488364622138 ) ) ;
#2466=LINE ( 'NONE', #23918, #19606 ) ;
#2468=CARTESIAN_POINT ( 'NONE',  ( 157.4703587214989113, 58.92748579479260229, -36.12418429913763163 ) ) ;
#2469=EDGE_CURVE ( 'NONE', #68633, #48880, #31068, .T. ) ;
#2474=CARTESIAN_POINT ( 'NONE',  ( -97.86516199987804043, 31.71158167298306907, 5.092746270469413972 ) ) ;
#2475=CARTESIAN_POINT ( 'NONE',  ( 70.47378276567178546, 15.56829108688369345, 91.86182244508080430 ) ) ;
#2476=CARTESIAN_POINT ( 'NONE',  ( 157.4703587214989113, 57.65129005721576760, 29.40946747225336466 ) ) ;
#2477=CARTESIAN_POINT ( 'NONE',  ( 79.18180043629683951, 18.06526831600449157, -17.49560269492410924 ) ) ;
#2478=CARTESIAN_POINT ( 'NONE',  ( -131.6508182719823594, 50.40277850441007246, -20.40230296405928101 ) ) ;
#2479=CARTESIAN_POINT ( 'NONE',  ( -149.5074843970971301, 64.17983161892347255, -88.50193171241930656 ) ) ;
#2480=CARTESIAN_POINT ( 'NONE',  ( 126.8947007444828614, 37.37669340849691224, -73.16922649445019999 ) ) ;
#2484=CYLINDRICAL_SURFACE ( 'NONE', #43335, 7.500000000000020428 ) ;
#2485=ORIENTED_EDGE ( 'NONE', *, *, #16200, .T. ) ;
#2488=DIRECTION ( 'NONE',  ( 0.000000000000000000, 0.000000000000000000, 1.000000000000000000 ) ) ;
#2493=CARTESIAN_POINT ( 'NONE',  ( -8.252323494751598432, 6.918840298267292965, -89.10717191287119476 ) ) ;
#2494=CARTESIAN_POINT ( 'NONE',  ( -51.78153763344965910, 13.82841714689605084, -76.32711335290281340 ) ) ;
#2495=CARTESIAN_POINT ( 'NONE',  ( -1.328627985309863258, 7.561890325089884790, -19.82887340779442198 ) ) ;
#2497=CARTESIAN_POINT ( 'NONE',  ( -7.825402957745085430, 7.899365992529246761, 45.11558103944722120 ) ) ;
#2501=CARTESIAN_POINT ( 'NONE',  ( -96.02159028238557426, 30.82695531378849552, -38.37423410059079032 ) ) ;
#2505=CARTESIAN_POINT ( 'NONE',  ( 41.33434189587760699, 9.684413566891869607, -9.024336741280105656 ) ) ;
#2506=CARTESIAN_POINT ( 'NONE',  ( 46.41758729921143356, 9.425975226414241348, 61.59540596826231962 ) ) ;
#2509=VECTOR ( 'NONE', #66846, 1000.000000000000000 ) ;
#2512=CARTESIAN_POINT ( 'NONE',  ( -169.8791831685531122, 83.59058982490286382, 71.94396900893276836 ) ) ;
#2513=ORIENTED_EDGE ( 'NONE', *, *, #2918, .F. ) ;
#2518=CARTESIAN_POINT ( 'NONE',  ( 102.7938674513918613, 26.67851209377771227, 64.96700818474666050 ) ) ;
#2520=CARTESIAN_POINT ( 'NONE',  ( 58.09877917144281412, 12.61383386832655518, -22.06060978329331235 ) ) ;
#2521=ORIENTED_EDGE ( 'NONE', *, *, #2569, .T. ) ;
#2523=CARTESIAN_POINT ( 'NONE',  ( -14.55390976651257162, 7.422979442794212623, 61.13778679154074780 ) ) ;
#2524=CARTESIAN_POINT ( 'NONE',  ( -84.23431294393863311, 24.52078568147205218, -20.81987607538617624 ) ) ;
#2526=CARTESIAN_POINT ( 'NONE',  ( 212.1707951106656935, 117.1901534358505899, -16.32344178605950091 ) ) ;
#2528=CARTESIAN_POINT ( 'NONE',  ( 9.229352927370984006, 6.379222623903515021, -93.04627149865262936 ) ) ;
#2529=EDGE_CURVE ( 'NONE', #48794, #67246, #9433, .T. ) ;
#2534=CARTESIAN_POINT ( 'NONE',  ( 31.91383250562746099, 8.564461488296995384, -69.47600483345588884 ) ) ;
#2537=CARTESIAN_POINT ( 'NONE',  ( 82.14449817946434962, 17.93919511903895980, -64.14975613024911638 ) ) ;
#2541=CARTESIAN_POINT ( 'NONE',  ( 197.1979149960397706, 98.19687999752001417, -44.16128514133923488 ) ) ;
#2548=CARTESIAN_POINT ( 'NONE',  ( -59.95412189755936794, 17.09836075175410031, -21.56948105266851812 ) ) ;
#2554=CARTESIAN_POINT ( 'NONE',  ( 45.35621884287174055, 10.27694987765648449, 59.67183030682132738 ) ) ;
#2557=CARTESIAN_POINT ( 'NONE',  ( 21.88606409348644277, 6.772455198693823952, 6.296696862013998697 ) ) ;
#2558=B_SPLINE_CURVE_WITH_KNOTS ( 'NONE', 3,
 ( #36675, #58126, #50510, #31395, #4651, #30359, #47546, #45226, #20832, #66704, #65484, #44006, #53858, #27138, #53166, #33128, #26463, #17277, #58452, #21516, #764, #31731, #6386, #43656, #59143, #406, #4999, #64782, #59489, #42630, #32431, #22563, #37693, #48231, #21863, #56, #5675, #22218, #1114, #48571, #53518, #64430, #65134 ),
 .UNSPECIFIED., .F., .F.,
 ( 4, 2, 2, 2, 2, 2, 2, 2, 2, 2, 2, 2, 1, 2, 2, 2, 2, 2, 2, 2, 2, 4 ),
 ( 0.02371951416048007424, 0.02520633211177539593, 0.02594974108742303595, 0.02669315006307067598, 0.02817996801436595949, 0.02966678596566124648, 0.03041019494130889345, 0.03115360391695653694, 0.03264042186825182740, 0.03412723981954712132, 0.03561405777084241525, 0.03635746674649006221, 0.03710087572213770918, 0.03784428469778534920, 0.03858769367343299617, 0.04007451162472830397, 0.04156132957602360484, 0.04304814752731890570, 0.04379155650296656654, 0.04453496547861421351, 0.04602178342990952131, 0.04750860138120482218 ),
 .UNSPECIFIED. ) ;
#2561=CARTESIAN_POINT ( 'NONE',  ( -48.34250119710923599, 14.01879126850789348, 7.613551659782504366 ) ) ;
#2562=CARTESIAN_POINT ( 'NONE',  ( -132.2161740628506266, 52.03204870034953444, -19.61185874996504452 ) ) ;
#2563=CARTESIAN_POINT ( 'NONE',  ( 117.7411475730015553, 32.50808475802735131, -17.12051833154609426 ) ) ;
#2564=LINE ( 'NONE', #55321, #48891 ) ;
#2569=EDGE_CURVE ( 'NONE', #13609, #53396, #62064, .T. ) ;
#2571=CARTESIAN_POINT ( 'NONE',  ( 46.84183314611289006, 9.494161546644502181, 11.54854982055374535 ) ) ;
#2572=CARTESIAN_POINT ( 'NONE',  ( -179.9869519326159946, 96.69839571505836773, 88.97430052463283801 ) ) ;
#2573=CARTESIAN_POINT ( 'NONE',  ( -48.32993240732256623, 12.98137013984324639, -12.50980678800987000 ) ) ;
#2574=CARTESIAN_POINT ( 'NONE',  ( 102.7551177910568470, 25.56939188780867767, -17.07542069066059298 ) ) ;
#2576=CARTESIAN_POINT ( 'NONE',  ( 204.6977192012829789, 106.3443248447423599, 2.363170148305747009 ) ) ;
#2577=CARTESIAN_POINT ( 'NONE',  ( 211.4199041905045249, 117.8812456326728721, 87.06571698777939616 ) ) ;
#2580=CARTESIAN_POINT ( 'NONE',  ( -13.78709718204646428, 7.352743657744177597, 33.03876092935409758 ) ) ;
#2582=CARTESIAN_POINT ( 'NONE',  ( 8.336237313193160858, 7.382629160459395656, -15.19676915959678709 ) ) ;
#2585=CARTESIAN_POINT ( 'NONE',  ( -146.1140637052938587, 62.65471088530799904, 4.672121997598104315 ) ) ;
#2587=CARTESIAN_POINT ( 'NONE',  ( -38.93057666883864698, 11.96714560916617742, 90.92290394697204192 ) ) ;
#2588=CARTESIAN_POINT ( 'NONE',  ( -99.31850058233801803, 31.30166762705811223, -35.62007679328529974 ) ) ;
#2589=AXIS2_PLACEMENT_3D ( 'NONE', #56553, #52313, #9067 ) ;
#2594=ORIENTED_EDGE ( 'NONE', *, *, #1303, .F. ) ;
#2600=CARTESIAN_POINT ( 'NONE',  ( -26.50364027666005029, 8.832969329054181529, -75.33011242007280828 ) ) ;
#2602=CARTESIAN_POINT ( 'NONE',  ( -47.60396279792516339, 12.80997843568594874, 36.81109710626871134 ) ) ;
#2603=CARTESIAN_POINT ( 'NONE',  ( 10.13846145460683523, 6.385368868491637429, 15.62687571206995329 ) ) ;
#2605=CARTESIAN_POINT ( 'NONE',  ( 44.34689728705971845, 10.12166135033765002, -64.30425762756091501 ) ) ;
#2606=CARTESIAN_POINT ( 'NONE',  ( -59.95412189755936083, 17.09836075175411807, -75.25858223359590227 ) ) ;
#2607=CARTESIAN_POINT ( 'NONE',  ( 197.9843579228224542, 99.18296459057403069, -67.31460967885617208 ) ) ;
#2609=CARTESIAN_POINT ( 'NONE',  ( 109.3047266816501377, 28.44977739115299187, 2.810780713438274070 ) ) ;
#2610=CARTESIAN_POINT ( 'NONE',  ( -169.3420190433745063, 83.01791327558585465, -89.40959992967984249 ) ) ;
#2613=EDGE_CURVE ( 'NONE', #65931, #57935, #59366, .T. ) ;
#2617=CARTESIAN_POINT ( 'NONE',  ( 150.2193536046551969, 53.46717047532150957, 61.81829156147041715 ) ) ;
#2623=ADVANCED_FACE ( 'NONE', ( #38664 ), #5943, .F. ) ;
#2630=ADVANCED_FACE ( 'NONE', ( #17556 ), #16849, .F. ) ;
#2636=CARTESIAN_POINT ( 'NONE',  ( -4.081377963939790909, 6.676029627840591729, 4.267774825659859772 ) ) ;
#2638=CARTESIAN_POINT ( 'NONE',  ( 55.51528220483959331, 12.08323518953686104, -42.98226798348757427 ) ) ;
#2640=CARTESIAN_POINT ( 'NONE',  ( 150.7492521598543078, 52.60853770899247905, 87.25043900936348962 ) ) ;
#2642=CARTESIAN_POINT ( 'NONE',  ( 136.1310312718401576, 42.81430973242785853, 17.32757056502941495 ) ) ;
#2647=CARTESIAN_POINT ( 'NONE',  ( -76.78104518372332166, 22.68568622761702969, 3.798941945053491143 ) ) ;
#2650=CARTESIAN_POINT ( 'NONE',  ( -149.5074843970971017, 64.17983161892347255, -34.81283053149196149 ) ) ;
#2655=ORIENTED_EDGE ( 'NONE', *, *, #23784, .F. ) ;
#2657=CARTESIAN_POINT ( 'NONE',  ( 84.26390409839190454, 19.68678207880321906, 44.34546724818678598 ) ) ;
#2659=EDGE_CURVE ( 'NONE', #40482, #29355, #17910, .T. ) ;
#2661=CARTESIAN_POINT ( 'NONE',  ( -125.0023254877051215, 45.90912477771774292, 57.50388153796715329 ) ) ;
#2662=CARTESIAN_POINT ( 'NONE',  ( -125.8938041572051389, -170.0000000000000000, 38.11994787315708777 ) ) ;
#2663=CARTESIAN_POINT ( 'NONE',  ( 19.76786553127199042, 7.667850394326512387, -90.33727694201498082 ) ) ;
#2664=CARTESIAN_POINT ( 'NONE',  ( -48.34500911884043006, 14.01939034823941910, 41.18154736179070596 ) ) ;
#2666=EDGE_LOOP ( 'NONE', ( #64992, #17344, #63519, #7045 ) ) ;
#2667=CARTESIAN_POINT ( 'NONE',  ( 102.7551177910568470, 25.56939188780867056, 63.45823108073047081 ) ) ;
#2672=CARTESIAN_POINT ( 'NONE',  ( -29.04258984626623175, 9.210213971636685315, -49.92821304749501365 ) ) ;
#2677=CARTESIAN_POINT ( 'NONE',  ( -7.825402957745083654, 6.891034867348166060, -50.41807073194384259 ) ) ;
#2678=CARTESIAN_POINT ( 'NONE',  ( -79.92369693322969226, 22.80368560911615816, 84.18822230409878671 ) ) ;
#2680=CARTESIAN_POINT ( 'NONE',  ( 70.26722489419891815, 14.47234958177329212, -45.19821637890682808 ) ) ;
#2682=CARTESIAN_POINT ( 'NONE',  ( -61.77164219855452387, 17.63686644795249236, 41.18722385704388955 ) ) ;
#2683=CARTESIAN_POINT ( 'NONE',  ( -94.83091526606385457, 30.26550147229322363, -16.68601127600661371 ) ) ;
#2688=CARTESIAN_POINT ( 'NONE',  ( -190.6985136298602015, 109.1272424661243434, -91.34903848884556510 ) ) ;
#2690=CARTESIAN_POINT ( 'NONE',  ( -5.871577929436018195, 6.771181646175758573, -35.66018690998220819 ) ) ;
#2694=CARTESIAN_POINT ( 'NONE',  ( -78.66644367742109978, 22.32174330031318732, -50.11545063171791270 ) ) ;
#2697=CARTESIAN_POINT ( 'NONE',  ( -108.6909373351217170, 36.15835109565441741, -73.28348265942591411 ) ) ;
#2699=CARTESIAN_POINT ( 'NONE',  ( 131.6115093721024891, 41.25402743071401801, -23.83854876421534996 ) ) ;
#2703=SHAPE_DEFINITION_REPRESENTATION ( #64721, #45199 ) ;
#2706=CARTESIAN_POINT ( 'NONE',  ( -37.93379515072632557, 11.77251734620211643, -46.60018604761813066 ) ) ;
#2708=CARTESIAN_POINT ( 'NONE',  ( 204.6977192012829789, -170.0000000000000000, 9.863170148305760776 ) ) ;
#2710=CARTESIAN_POINT ( 'NONE',  ( 129.1310456962235094, 39.80382822048398594, 4.321560090366997287 ) ) ;
#2711=CARTESIAN_POINT ( 'NONE',  ( -144.9287131874382055, 60.39056348581543432, -9.508616525343073889 ) ) ;
#2712=CARTESIAN_POINT ( 'NONE',  ( 199.7286177451876199, 101.4075663537892211, 4.226501175219063100 ) ) ;
#2715=CARTESIAN_POINT ( 'NONE',  ( 150.0309095590486663, 53.33084854625626292, 91.62168867483059387 ) ) ;
#2717=CARTESIAN_POINT ( 'NONE',  ( 204.6977192012829789, 108.0580384837234931, 71.05227132923315025 ) ) ;
#2721=CARTESIAN_POINT ( 'NONE',  ( 23.28869764673362042, 6.856674305776598644, -42.53058434114498709 ) ) ;
#2722=CARTESIAN_POINT ( 'NONE',  ( 84.73231936899556160, 18.78199960571076943, 3.095663364362381653 ) ) ;
#2725=CARTESIAN_POINT ( 'NONE',  ( -0.4996266546846081513, 7.531422798935177632, -95.00000000000133582 ) ) ;
#2728=CARTESIAN_POINT ( 'NONE',  ( 173.9457771591584958, 73.05793967547529633, 34.48989055565348139 ) ) ;
#2730=CARTESIAN_POINT ( 'NONE',  ( -34.14504207561676452, 11.07284558078377579, -89.50818587954944405 ) ) ;
#2731=CARTESIAN_POINT ( 'NONE',  ( -14.92860730136983527, 8.468845235798742266, -72.18242109116805239 ) ) ;
#2733=CARTESIAN_POINT ( 'NONE',  ( -95.09829086201085602, 30.39089736475074943, 89.52221081825875615 ) ) ;
#2734=CARTESIAN_POINT ( 'NONE',  ( -24.03640295269299898, 9.507963273819770578, 36.48715109637453224 ) ) ;
#2738=CARTESIAN_POINT ( 'NONE',  ( 174.6490316376289513, 73.72059609105147615, -93.55543838724517514 ) ) ;
#2739=VECTOR ( 'NONE', #26466, 1000.000000000000000 ) ;
#2741=CARTESIAN_POINT ( 'NONE',  ( 141.2361973397653401, 47.26569015399785911, 38.37501290123390874 ) ) ;
#2742=B_SPLINE_CURVE_WITH_KNOTS ( 'NONE', 3,
 ( #61198, #28488, #45360, #12314, #6333, #17939, #49578, #18284, #23568, #22861, #34482, #60842, #65431, #7033, #49935, #66150, #13021, #11960 ),
 .UNSPECIFIED., .F., .F.,
 ( 4, 2, 2, 2, 2, 2, 2, 2, 4 ),
 ( 0.000000000000000000, 0.001486129123402290652, 0.002972258246804581304, 0.004458387370206871522, 0.005944516493609162608, 0.007430645617011453694, 0.008916774740413743044, 0.01040290386381603413, 0.01188903298721832522 ),
 .UNSPECIFIED. ) ;
#2745=CARTESIAN_POINT ( 'NONE',  ( 129.4887940973039804, 40.01039828304092794, 69.97058656504017904 ) ) ;
#2747=ORIENTED_EDGE ( 'NONE', *, *, #46120, .F. ) ;
#2756=CARTESIAN_POINT ( 'NONE',  ( -71.86568654225717978, 20.91200104397924164, -18.94308595472579881 ) ) ;
#2758=CARTESIAN_POINT ( 'NONE',  ( -104.5740066103012254, 35.09687312794776659, 30.87461852538474005 ) ) ;
#2760=CARTESIAN_POINT ( 'NONE',  ( 32.90878072717891456, 7.653588083204844850, 41.17538734954451485 ) ) ;
#2762=EDGE_LOOP ( 'NONE', ( #38333, #62039 ) ) ;
#2763=CARTESIAN_POINT ( 'NONE',  ( 186.6118452967672283, 84.37814701615440072, 41.90269769157806934 ) ) ;
#2766=CARTESIAN_POINT ( 'NONE',  ( 38.42384008295177722, 8.283891555743471358, 18.02114195686916176 ) ) ;
#2767=CARTESIAN_POINT ( 'NONE',  ( -13.79190010541702627, 8.363435739308560102, -38.34741394315791752 ) ) ;
#2768=CARTESIAN_POINT ( 'NONE',  ( 152.1190604254709910, 53.60705199010333644, -48.88494239191637547 ) ) ;
#2772=CARTESIAN_POINT ( 'NONE',  ( -156.9252506979472344, 70.73559306219775067, -16.61248648017295082 ) ) ;
#2775=CARTESIAN_POINT ( 'NONE',  ( -62.41727141396690826, 17.83188754031766976, 66.14490890585253169 ) ) ;
#2776=CYLINDRICAL_SURFACE ( 'NONE', #37568, 7.500000000000020428 ) ;
#2779=CARTESIAN_POINT ( 'NONE',  ( 155.7167524447090727, 57.56687707799949294, -63.16317902508508553 ) ) ;
#2781=CARTESIAN_POINT ( 'NONE',  ( -96.02415295709705845, 29.71480036090586907, -19.81432279787944140 ) ) ;
#2782=CARTESIAN_POINT ( 'NONE',  ( 136.9934874058118055, 43.35050367224292955, -36.69511880788390812 ) ) ;
#2784=ADVANCED_FACE ( 'NONE', ( #326 ), #64702, .F. ) ;
#2792=CARTESIAN_POINT ( 'NONE',  ( 186.2722199822850655, 84.01218714714246971, 15.40014518578409763 ) ) ;
#2794=CARTESIAN_POINT ( 'NONE',  ( 126.4418792563097327, 38.27634703522673476, 89.51384704393026936 ) ) ;
#2798=VECTOR ( 'NONE', #35005, 1000.000000000000000 ) ;
#2800=CARTESIAN_POINT ( 'NONE',  ( -124.9927180788553756, 45.90286323198616003, -61.79884557940761880 ) ) ;
#2802=CARTESIAN_POINT ( 'NONE',  ( 204.6977192012829789, -170.0000000000000000, -90.01503221354893469 ) ) ;
#2804=CARTESIAN_POINT ( 'NONE',  ( 68.63487067129264574, 14.04635751989140502, 69.14883297453368982 ) ) ;
#2805=CARTESIAN_POINT ( 'NONE',  ( 134.7708899521910837, 43.15864772107691749, 2.718175913858767778 ) ) ;
#2811=CARTESIAN_POINT ( 'NONE',  ( 69.49112875363887554, 15.30845942322119591, 60.36544806545548880 ) ) ;
#2812=CARTESIAN_POINT ( 'NONE',  ( 140.6983622512872785, 45.71183921003505191, 93.79223251056832567 ) ) ;
#2814=CARTESIAN_POINT ( 'NONE',  ( 164.8444104055694481, 64.93678790243657772, -45.02061212871966944 ) ) ;
#2817=CARTESIAN_POINT ( 'NONE',  ( 160.9069879467681119, 60.37290772564306707, -50.30662973681143768 ) ) ;
#2818=ORIENTED_EDGE ( 'NONE', *, *, #1514, .F. ) ;
#2823=CARTESIAN_POINT ( 'NONE',  ( 79.22872707466395070, 18.07970189365807201, -15.23444678155258103 ) ) ;
#2824=CARTESIAN_POINT ( 'NONE',  ( -176.7403177620948895, 92.79785224917912956, -89.32883995899774732 ) ) ;
#2825=CARTESIAN_POINT ( 'NONE',  ( -143.1937182229694656, 59.00378877849532699, -91.94668305751585535 ) ) ;
#2826=CARTESIAN_POINT ( 'NONE',  ( 126.3541873520044305, 37.07520218256171773, -70.86737662479835365 ) ) ;
#2828=CARTESIAN_POINT ( 'NONE',  ( -96.02159028238558847, 30.82695531378847775, 69.00396826126393535 ) ) ;
#2832=CARTESIAN_POINT ( 'NONE',  ( -153.6946616617039183, 69.16142959008689672, -48.55193879071696017 ) ) ;
#2841=CARTESIAN_POINT ( 'NONE',  ( -51.13073217147961458, 13.66490163179657635, -63.16339902663095529 ) ) ;
#2842=CARTESIAN_POINT ( 'NONE',  ( 205.5004956747122264, 107.4493581495447785, -51.29378026339399810 ) ) ;
#2843=CARTESIAN_POINT ( 'NONE',  ( 173.7246046907419839, 71.47482343504563573, 11.43823586838169426 ) ) ;
#2844=CARTESIAN_POINT ( 'NONE',  ( -58.33245019990697244, 15.58496056636070293, 17.73516165329973759 ) ) ;
#2849=CARTESIAN_POINT ( 'NONE',  ( 103.5839822277949764, 25.92130892112108853, -66.80704105902555057 ) ) ;
#2850=CARTESIAN_POINT ( 'NONE',  ( 45.35146934743632841, 10.27620685439442028, -11.68218203743552586 ) ) ;
#2851=CARTESIAN_POINT ( 'NONE',  ( 46.76970795284344717, 9.482505412758895247, 65.72351425996377827 ) ) ;
#2852=DIRECTION ( 'NONE',  ( -0.000000000000000000, 1.000000000000000000, -0.000000000000000000 ) ) ;
#2855=CARTESIAN_POINT ( 'NONE',  ( 59.12362561977391096, 12.83186343420200970, -90.44545082695854887 ) ) ;
#2856=CARTESIAN_POINT ( 'NONE',  ( -166.7068579965636843, 80.26142964949320913, 61.27046711184852512 ) ) ;
#2858=EDGE_LOOP ( 'NONE', ( #46250, #47296, #53615, #9063 ) ) ;
#2862=CARTESIAN_POINT ( 'NONE',  ( 177.7960900018544521, 75.34533826015461955, -10.13599328491967277 ) ) ;
#2863=CARTESIAN_POINT ( 'NONE',  ( 102.7446498997619813, 26.65764321315729646, 63.41915715202346604 ) ) ;
#2869=CARTESIAN_POINT ( 'NONE',  ( -12.77647591501652791, 7.263973827022343954, 58.80487624720162643 ) ) ;
#2870=CARTESIAN_POINT ( 'NONE',  ( -86.17927978631391284, 25.32700573188351001, -15.75888056856657471 ) ) ;
#2872=FACE_BOUND ( 'NONE', #12550, .T. ) ;
#2874=B_SPLINE_CURVE_WITH_KNOTS ( 'NONE', 3,
 ( #17395, #12133, #33596, #6845, #44483, #65963, #17761, #7200, #50112, #63086, #9973, #8599, #30738, #68699, #46554, #40589, #14552, #25124, #36709, #67344, #14890, #36011, #19135, #57465, #35320, #62750, #57812, #19478, #36355, #47242, #68035, #62042, #13858, #31424, #9631, #52185, #41974, #62399, #9275, #63436, #40940, #20176, #14213, #35675 ),
 .UNSPECIFIED., .F., .F.,
 ( 4, 2, 2, 2, 2, 2, 2, 2, 2, 2, 2, 2, 2, 2, 2, 2, 2, 2, 2, 2, 2, 4 ),
 ( 0.02477387709520258163, 0.02633314402883776828, 0.02711277749565536854, 0.02789241096247296534, 0.02945167789610817627, 0.03023131136292576265, 0.03101094482974335251, 0.03257021176337856344, 0.03334984523019616370, 0.03412947869701375703, 0.03568874563064895755, 0.03646837909746653006, 0.03724801256428410257, 0.03802764603110168201, 0.03880727949791926146, 0.04036654643155440647, 0.04192581336518955148, 0.04348508029882469650, 0.04504434723245984151, 0.04660361416609498653, 0.04816288109973011766, 0.04972214803336524880 ),
 .UNSPECIFIED. ) ;
#2880=VECTOR ( 'NONE', #59830, 1000.000000000000000 ) ;
#2882=LINE ( 'NONE', #63353, #38839 ) ;
#2883=CARTESIAN_POINT ( 'NONE',  ( 8.290168341070513591, 6.376397093466350086, 91.57150589958799003 ) ) ;
#2885=CARTESIAN_POINT ( 'NONE',  ( 81.03898448521320574, 17.58847173596443625, -75.19045902363498612 ) ) ;
#2888=VERTEX_POINT ( 'NONE', #50960 ) ;
#2892=CARTESIAN_POINT ( 'NONE',  ( 200.4590013143046292, 102.3556155835302945, -50.03054843160261811 ) ) ;
#2895=CARTESIAN_POINT ( 'NONE',  ( -7.825402957745087207, -170.0000000000000000, 18.27103044898354511 ) ) ;
#2897=AXIS2_PLACEMENT_3D ( 'NONE', #60259, #12078, #17706 ) ;
#2898=CARTESIAN_POINT ( 'NONE',  ( -85.46258339457288855, 25.02772366257410752, -72.64209979375846160 ) ) ;
#2901=ORIENTED_EDGE ( 'NONE', *, *, #42078, .F. ) ;
#2903=CARTESIAN_POINT ( 'NONE',  ( 46.90208227351340042, 10.52324439420451263, 64.01647544768613329 ) ) ;
#2904=CARTESIAN_POINT ( 'NONE',  ( -102.2801239173131052, 33.91021738430208643, -88.70367844590326456 ) ) ;
#2905=CARTESIAN_POINT ( 'NONE',  ( 21.25987915030397701, 6.737472588634917159, 5.534856484934720378 ) ) ;
#2906=VERTEX_POINT ( 'NONE', #2091 ) ;
#2907=CARTESIAN_POINT ( 'NONE',  ( 178.1965488566140436, 77.14488558164481447, -77.50486268625550679 ) ) ;
#2910=CARTESIAN_POINT ( 'NONE',  ( 80.15818551272214165, 18.36718314243333694, -39.49802388013461041 ) ) ;
#2911=CARTESIAN_POINT ( 'NONE',  ( 8.000000000000007105, 249.8719672152120381, -95.00000000000133582 ) ) ;
#2915=CARTESIAN_POINT ( 'NONE',  ( 46.13856685535759539, 9.381502944822527112, 13.90276314609397268 ) ) ;
#2916=DIRECTION ( 'NONE',  ( -0.000000000000000000, 1.000000000000000000, -0.000000000000000000 ) ) ;
#2917=CARTESIAN_POINT ( 'NONE',  ( -49.11825192196926082, 13.17012322555987325, -11.25932645589339565 ) ) ;
#2918=EDGE_CURVE ( 'NONE', #60277, #49052, #10721, .T. ) ;
#2919=CARTESIAN_POINT ( 'NONE',  ( 109.3047266816501377, 28.44977739115299542, -24.03376987702539225 ) ) ;
#2920=CARTESIAN_POINT ( 'NONE',  ( 198.7029050523552485, 98.46895521196213963, 14.39901884897147788 ) ) ;
#2922=CARTESIAN_POINT ( 'NONE',  ( 207.5555325562649500, 112.1057321206939292, 83.44071583484532084 ) ) ;
#2929=CARTESIAN_POINT ( 'NONE',  ( 15.78827728214693416, 7.507518794609588042, -23.67439350822212774 ) ) ;
#2930=ORIENTED_EDGE ( 'NONE', *, *, #52098, .F. ) ;
#2933=CIRCLE ( 'NONE', #64677, 242.4895526022646379 ) ;
#2934=CARTESIAN_POINT ( 'NONE',  ( 188.2962140587030149, 87.71627202537840162, -72.64852955523822686 ) ) ;
#2935=CARTESIAN_POINT ( 'NONE',  ( -165.6404838346739439, 80.60836113891892296, 38.93951364949523253 ) ) ;
#2936=CARTESIAN_POINT ( 'NONE',  ( -94.77925136849377452, 29.13093715379786630, -42.28272860464903005 ) ) ;
#2939=CARTESIAN_POINT ( 'NONE',  ( -24.32776401346967887, 9.546905915310563984, 13.30497887696894210 ) ) ;
#2941=CARTESIAN_POINT ( 'NONE',  ( 9.275903038161098735, 7.385619229189525292, -39.26677353779081159 ) ) ;
#2943=CARTESIAN_POINT ( 'NONE',  ( 130.3019683985926349, 39.31883119822049366, -50.14450225213496992 ) ) ;
#2944=ORIENTED_EDGE ( 'NONE', *, *, #30928, .T. ) ;
#2946=ORIENTED_EDGE ( 'NONE', *, *, #38816, .F. ) ;
#2949=CARTESIAN_POINT ( 'NONE',  ( 188.1640390495057602, 87.56943377085097779, 88.01576467520247604 ) ) ;
#2950=CARTESIAN_POINT ( 'NONE',  ( -13.47680110791657349, 7.324966777230637049, 5.815555111528495580 ) ) ;
#2952=CARTESIAN_POINT ( 'NONE',  ( -29.49620345460276027, 9.280093073089044964, -62.40110739915159144 ) ) ;
#2959=CARTESIAN_POINT ( 'NONE',  ( -61.10880364359507411, 17.43879918625640357, -73.99209842384989599 ) ) ;
#2960=CARTESIAN_POINT ( 'NONE',  ( 200.4574930424075490, 102.3536505870638393, -64.46692893376646794 ) ) ;
#2961=CARTESIAN_POINT ( 'NONE',  ( -175.9852529046322616, 90.37283472601130541, -35.26747372587856688 ) ) ;
#2962=CARTESIAN_POINT ( 'NONE',  ( 105.4193882736796155, 26.71329717705294726, 4.502293189513017602 ) ) ;
#2965=CARTESIAN_POINT ( 'NONE',  ( -52.68007207639879397, 14.05813534436550327, 57.54295262752664541 ) ) ;
#2966=ADVANCED_FACE ( 'NONE', ( #16340 ), #20929, .F. ) ;
#2967=CARTESIAN_POINT ( 'NONE',  ( -0.3734056954813063101, 6.520221844775928588, 65.43821756026045477 ) ) ;
#2970=CARTESIAN_POINT ( 'NONE',  ( 156.3797504404255960, 58.07856685387021400, 56.33044317893267561 ) ) ;
#2972=CARTESIAN_POINT ( 'NONE',  ( -50.13771638889890880, 13.41835215703894413, -37.03013167601228162 ) ) ;
#2973=ADVANCED_FACE ( 'NONE', ( #69104 ), #47989, .F. ) ;
#2975=EDGE_CURVE ( 'NONE', #60490, #50015, #69523, .T. ) ;
#2978=ORIENTED_EDGE ( 'NONE', *, *, #21048, .T. ) ;
#2984=CARTESIAN_POINT ( 'NONE',  ( -7.825402957745087207, -170.0000000000000000, 10.77103044898353090 ) ) ;
#2990=CARTESIAN_POINT ( 'NONE',  ( -180.0179082103088319, 95.14811732286301549, 14.43829403818141444 ) ) ;
#2991=CARTESIAN_POINT ( 'NONE',  ( -4.070918861171930914, 6.675509947362630925, 17.26827648209658506 ) ) ;
#2992=CARTESIAN_POINT ( 'NONE',  ( 59.73312635112155533, 12.96464920523511388, -49.98156322790594430 ) ) ;
#2995=CARTESIAN_POINT ( 'NONE',  ( 141.3707934840545022, 46.15056991286792965, 10.13612274068955443 ) ) ;
#2996=CARTESIAN_POINT ( 'NONE',  ( 205.5105258529713694, 107.4632495673648549, 44.17461234944981641 ) ) ;
#3002=CARTESIAN_POINT ( 'NONE',  ( -71.46567093091299228, 20.77283810584936319, 93.80455591633044321 ) ) ;
#3007=CARTESIAN_POINT ( 'NONE',  ( -142.0081215801270389, 58.07066293384868061, 64.76555490188158615 ) ) ;
#3008=LINE ( 'NONE', #45911, #69307 ) ;
#3010=CARTESIAN_POINT ( 'NONE',  ( 188.5837490358996149, 86.53279111916964439, -17.19126881223536785 ) ) ;
#3012=CARTESIAN_POINT ( 'NONE',  ( -80.54915509118116290, 24.12810583352864313, -23.03467912020122554 ) ) ;
#3013=CARTESIAN_POINT ( 'NONE',  ( -180.6215424137752166, 97.48070480470863686, -15.06146349129376638 ) ) ;
#3015=CARTESIAN_POINT ( 'NONE',  ( -47.55316895016325418, 13.83165595246916979, 38.31999599868878192 ) ) ;
#3020=CARTESIAN_POINT ( 'NONE',  ( 163.7464701930790909, 62.69993100427430477, 59.61700847725186492 ) ) ;
#3021=CARTESIAN_POINT ( 'NONE',  ( -173.1211646369891355, -170.0000000000000000, 65.16624519710472896 ) ) ;
#3022=CARTESIAN_POINT ( 'NONE',  ( 184.3941060377211727, 82.01604625189463604, -50.46965181017390023 ) ) ;
#3024=CARTESIAN_POINT ( 'NONE',  ( 158.3604774538084712, 58.34594647925806754, -63.00838262857361372 ) ) ;
#3026=EDGE_CURVE ( 'NONE', #34992, #7668, #60298, .T. ) ;
#3028=ORIENTED_EDGE ( 'NONE', *, *, #67045, .F. ) ;
#3033=CARTESIAN_POINT ( 'NONE',  ( -7.825402957745085430, 7.899365992529246761, 71.96013162991091860 ) ) ;
#3034=CARTESIAN_POINT ( 'NONE',  ( 175.1402005715378891, 72.80033409921840359, -92.83546321808604773 ) ) ;
#3035=CARTESIAN_POINT ( 'NONE',  ( 63.49940197359695304, 12.78497925206076502, -50.72069083216975827 ) ) ;
#3039=CARTESIAN_POINT ( 'NONE',  ( -62.15063206372445137, 17.75106610013994057, 35.34437635207743966 ) ) ;
#3040=CARTESIAN_POINT ( 'NONE',  ( -97.49665543375859045, 31.53324358035374075, -9.872370814404565209 ) ) ;
#3042=CARTESIAN_POINT ( 'NONE',  ( 38.90894112122322213, 8.345444037631242651, 71.75838489642697482 ) ) ;
#3045=AXIS2_PLACEMENT_3D ( 'NONE', #12113, #49371, #37184 ) ;
#3048=CARTESIAN_POINT ( 'NONE',  ( -189.2352924136013144, 107.0839554967701019, -42.55778393734637177 ) ) ;
#3050=LINE ( 'NONE', #24157, #28594 ) ;
#3051=CARTESIAN_POINT ( 'NONE',  ( 18.19858669090299941, 7.596860100017451600, -9.067989001026109719 ) ) ;
#3052=CARTESIAN_POINT ( 'NONE',  ( 197.5334904971816457, 97.00846725096931777, 65.79350108939836161 ) ) ;
#3060=CARTESIAN_POINT ( 'NONE',  ( -175.7433116402202700, 90.09372610121394587, 84.96528934235752217 ) ) ;
#3062=CARTESIAN_POINT ( 'NONE',  ( 127.2358066117906503, 38.72257733469227503, 6.605040416640627576 ) ) ;
#3065=CARTESIAN_POINT ( 'NONE',  ( -143.3925773749111556, 59.16144459815140522, -11.11823926598882650 ) ) ;
#3066=CARTESIAN_POINT ( 'NONE',  ( 203.9228889538744909, 106.9879579748728418, 2.392848837412264285 ) ) ;
#3067=VERTEX_POINT ( 'NONE', #28640 ) ;
#3068=CARTESIAN_POINT ( 'NONE',  ( 155.1915247301153045, 57.16500775723477545, 83.44643162593852992 ) ) ;
#3070=CARTESIAN_POINT ( 'NONE',  ( -62.49137879463567202, 17.85440472148629354, 11.96262358591842734 ) ) ;
#3078=CARTESIAN_POINT ( 'NONE',  ( 55.51597771111714508, 11.05737652677076177, 37.81267142505173240 ) ) ;
#3082=CARTESIAN_POINT ( 'NONE',  ( -169.8972248494843029, 85.08697738648012887, 18.26369148981731882 ) ) ;
#3083=CARTESIAN_POINT ( 'NONE',  ( 16.27765348919936983, 6.516472002017811960, -77.36349468914950478 ) ) ;
#3085=FACE_OUTER_BOUND ( 'NONE', #4736, .T. ) ;
#3086=ORIENTED_EDGE ( 'NONE', *, *, #62668, .F. ) ;
#3087=CARTESIAN_POINT ( 'NONE',  ( -98.33967698037261584, 31.94276620606871475, 85.31931532774478910 ) ) ;
#3088=CARTESIAN_POINT ( 'NONE',  ( -77.71490760329793090, 23.03637365463981013, -50.07002586140477263 ) ) ;
#3092=CARTESIAN_POINT ( 'NONE',  ( 212.0075063341773784, 118.7912820769029594, -72.37935731155032215 ) ) ;
#3095=CARTESIAN_POINT ( 'NONE',  ( 138.5684226926155418, 45.53585076428272771, 42.86542189636780620 ) ) ;
#3098=CARTESIAN_POINT ( 'NONE',  ( -128.7724923851857000, 49.63576597317771189, 18.20476702891221521 ) ) ;
#3099=CARTESIAN_POINT ( 'NONE',  ( 181.0840389613909736, 80.03940679743418229, -63.06960825634327961 ) ) ;
#3102=CARTESIAN_POINT ( 'NONE',  ( -144.9417090887490644, 61.69631066549398213, -21.42304724940910532 ) ) ;
#3104=FACE_OUTER_BOUND ( 'NONE', #8174, .T. ) ;
#3105=CARTESIAN_POINT ( 'NONE',  ( -51.19577760053109472, 14.71865550854504257, -89.96963771126178244 ) ) ;
#3107=CARTESIAN_POINT ( 'NONE',  ( -146.5341851369306312, 61.69744206542953435, 31.32122742849548303 ) ) ;
#3108=CARTESIAN_POINT ( 'NONE',  ( -123.0348077379026961, 45.83489305753316501, 45.05744747576095222 ) ) ;
#3109=CARTESIAN_POINT ( 'NONE',  ( -167.9889421625799741, 81.59140042431229745, -74.54592677586461491 ) ) ;
#3110=EDGE_CURVE ( 'NONE', #61225, #18664, #27538, .T. ) ;
#3111=VERTEX_POINT ( 'NONE', #13507 ) ;
#3112=CARTESIAN_POINT ( 'NONE',  ( -105.8879245385188455, 35.79035667534149923, 44.61188123920754833 ) ) ;
#3114=CARTESIAN_POINT ( 'NONE',  ( -38.87848244732136749, 10.93141945332450327, 9.888487578027829628 ) ) ;
#3115=CARTESIAN_POINT ( 'NONE',  ( 81.76212856587194722, 18.87332718082995342, 58.34523743138716867 ) ) ;
#3123=CARTESIAN_POINT ( 'NONE',  ( 34.84173759613683075, 7.859847277726518477, 16.54372376058861605 ) ) ;
#3124=CARTESIAN_POINT ( 'NONE',  ( -13.92109095214680181, 8.375243258322926820, -47.29446107485116357 ) ) ;
#3132=LINE ( 'NONE', #61171, #3890 ) ;
#3136=CARTESIAN_POINT ( 'NONE',  ( -56.53161132927532861, 15.08292330397246594, -89.04960089425232184 ) ) ;
#3143=( LENGTH_UNIT ( ) NAMED_UNIT ( * ) SI_UNIT ( .MILLI., .METRE. ) );
#3144=CARTESIAN_POINT ( 'NONE',  ( -149.5074843970971017, 65.50121172469319220, 57.56537183036274286 ) ) ;
#3145=CARTESIAN_POINT ( 'NONE',  ( -118.6849742182704972, 41.92701402439728042, 40.20636930516527485 ) ) ;
#3147=CARTESIAN_POINT ( 'NONE',  ( -61.39252081892700375, 16.47343302442958546, -46.73105210731662851 ) ) ;
#3149=CARTESIAN_POINT ( 'NONE',  ( -179.2210908201801374, 95.76260491022615895, -64.66443386884608913 ) ) ;
#3150=CARTESIAN_POINT ( 'NONE',  ( 132.6781767539480654, 41.88870008768979147, 83.26602666350336790 ) ) ;
#3152=CARTESIAN_POINT ( 'NONE',  ( 117.6916924104495479, 32.48309187151382105, 38.12703603328098012 ) ) ;
#3158=CARTESIAN_POINT ( 'NONE',  ( 66.30567821786758032, 13.45988234822862317, 70.90175730764632078 ) ) ;
#3159=CARTESIAN_POINT ( 'NONE',  ( 182.8363374612695793, 80.39432370332461630, -90.11314248946574423 ) ) ;
#3162=CARTESIAN_POINT ( 'NONE',  ( -31.43908319763710679, -170.0000000000000000, 57.06100499665286208 ) ) ;
#3164=CARTESIAN_POINT ( 'NONE',  ( 181.0840389613909736, -170.0000000000000000, 36.80859410551140343 ) ) ;
#3165=CARTESIAN_POINT ( 'NONE',  ( 138.0718262224615103, 44.02755351423877528, 84.46378310921993204 ) ) ;
#3168=CARTESIAN_POINT ( 'NONE',  ( -144.2029146819478456, 59.80706661873672658, -63.83344705439064626 ) ) ;
#3170=CARTESIAN_POINT ( 'NONE',  ( 164.8942204024298803, 63.66138186734713855, -42.52176649176428214 ) ) ;
#3172=CARTESIAN_POINT ( 'NONE',  ( -101.8140949286062380, 33.67224128592400945, 18.67452391595143979 ) ) ;
#3174=CARTESIAN_POINT ( 'NONE',  ( 55.63918192129861495, 12.10794348580856905, 92.51693346615715541 ) ) ;
#3175=VECTOR ( 'NONE', #11581, 1000.000000000000000 ) ;
#3176=CARTESIAN_POINT ( 'NONE',  ( 151.0575564466925869, 54.07682166848538685, -93.41829839593862062 ) ) ;
#3180=CARTESIAN_POINT ( 'NONE',  ( -32.41627406084101892, 9.753381371531530064, -62.20983653673231117 ) ) ;
#3181=CARTESIAN_POINT ( 'NONE',  ( 94.02861641584117081, 23.15570573563316259, 35.96120553985514334 ) ) ;
#3186=EDGE_LOOP ( 'NONE', ( #35248, #68104 ) ) ;
#3188=CARTESIAN_POINT ( 'NONE',  ( 154.6530827109543225, 56.75509330623209792, -9.825228603827484974 ) ) ;
#3189=VECTOR ( 'NONE', #65915, 1000.000000000000000 ) ;
#3191=CARTESIAN_POINT ( 'NONE',  ( -36.00304714721387711, 11.40794940913596278, 43.68818208324128705 ) ) ;
#3192=CARTESIAN_POINT ( 'NONE',  ( -155.1302201283145905, 69.09929365814132041, -64.18797151881071272 ) ) ;
#3193=CARTESIAN_POINT ( 'NONE',  ( 58.68582878687972482, 11.70927268415886502, 84.84224536443331033 ) ) ;
#3194=CARTESIAN_POINT ( 'NONE',  ( -50.52927270563907314, 13.51486287463704450, -75.56336441046521202 ) ) ;
#3195=CARTESIAN_POINT ( 'NONE',  ( -0.3255842968951678240, 7.525381170773407291, -15.58124028427686447 ) ) ;
#3200=CARTESIAN_POINT ( 'NONE',  ( -96.45303203827904781, 31.03218867996498176, -37.76676309982019575 ) ) ;
#3204=CARTESIAN_POINT ( 'NONE',  ( 42.03719354205839664, 9.783015072457470040, -9.249201505377850907 ) ) ;
#3208=CARTESIAN_POINT ( 'NONE',  ( 18.19858669090298520, 7.596860100017449824, 44.62111217990123890 ) ) ;
#3209=CARTESIAN_POINT ( 'NONE',  ( -108.9145525555662459, 37.42858360505776716, -19.17698904105195368 ) ) ;
#3210=ORIENTED_EDGE ( 'NONE', *, *, #30839, .T. ) ;
#3212=CARTESIAN_POINT ( 'NONE',  ( -167.6413528428655013, 81.22881971256910560, 60.01989802298776766 ) ) ;
#3215=CYLINDRICAL_SURFACE ( 'NONE', #1728, 7.500000000000020428 ) ;
#3217=CARTESIAN_POINT ( 'NONE',  ( 180.2572128312847894, 77.77323980479701504, -24.34663789818131363 ) ) ;
#3218=CARTESIAN_POINT ( 'NONE',  ( 104.3759779378692372, 27.35691041569131343, 68.65435695942450423 ) ) ;
#3220=CARTESIAN_POINT ( 'NONE',  ( 57.09527843067914432, 12.40436368789086785, -20.98701010641955733 ) ) ;
#3223=ORIENTED_EDGE ( 'NONE', *, *, #30107, .T. ) ;
#3225=CARTESIAN_POINT ( 'NONE',  ( 10.13563904803030447, 7.391572367417535538, 69.31278184914521034 ) ) ;
#3226=FACE_BOUND ( 'NONE', #24376, .T. ) ;
#3227=B_SPLINE_CURVE_WITH_KNOTS ( 'NONE', 3,
 ( #41962, #5696, #42308, #59503, #64104, #5363, #16601, #21200, #63423, #26820, #48247, #58469, #21530, #15228, #10281, #42975, #64446, #10977, #27154, #7099, #1837, #33500, #65499, #33143, #38405, #39125, #60563, #55629, #12379, #28199, #65149, #38770, #6404, #12031, #7460, #54577, #50368, #39457, #55990, #22934, #34196, #61263, #33839, #16943, #34549 ),
 .UNSPECIFIED., .F., .F.,
 ( 4, 2, 2, 2, 2, 2, 2, 2, 2, 2, 2, 1, 2, 2, 2, 2, 2, 2, 2, 2, 2, 2, 4 ),
 ( 0.000000000000000000, 0.001510509505236004449, 0.002265764257853984665, 0.003021019010471965097, 0.004531528515707889532, 0.005286783268325863892, 0.006042038020943839120, 0.007552547526179752280, 0.009063057031415664572, 0.01057356653665157860, 0.01132882128926953128, 0.01208407604188748395, 0.01283933079450543663, 0.01359458554712339277, 0.01510509505235930854, 0.01586034980497727509, 0.01661560455759524338, 0.01812611406283117996, 0.01963662356806712347, 0.02039187832068507789, 0.02114713307330302883, 0.02265764257853897234, 0.02416815208377491586 ),
 .UNSPECIFIED. ) ;
#3228=VERTEX_POINT ( 'NONE', #59158 ) ;
#3232=CARTESIAN_POINT ( 'NONE',  ( -129.7676077573642317, 50.31906829115933988, 85.38013851079792005 ) ) ;
#3234=DIRECTION ( 'NONE',  ( 0.000000000000000000, 0.000000000000000000, 1.000000000000000000 ) ) ;
#3235=CARTESIAN_POINT ( 'NONE',  ( 22.60048481713442925, 6.814323260940660099, 88.04925594562278945 ) ) ;
#3236=CARTESIAN_POINT ( 'NONE',  ( 23.26327404354069017, 7.863253330465858504, 91.89846529273600595 ) ) ;
#3238=ORIENTED_EDGE ( 'NONE', *, *, #449, .T. ) ;
#3241=CARTESIAN_POINT ( 'NONE',  ( 197.5344630110112689, 98.61758706718750034, -46.07028429264449443 ) ) ;
#3242=EDGE_LOOP ( 'NONE', ( #5036, #23690, #1221, #58718 ) ) ;
#3243=CARTESIAN_POINT ( 'NONE',  ( 109.4689210239672832, 29.63125812599453823, -89.61153874658103291 ) ) ;
#3245=CARTESIAN_POINT ( 'NONE',  ( -86.06489347855097094, 25.27905598459106429, -70.71628207122289211 ) ) ;
#3246=CARTESIAN_POINT ( 'NONE',  ( -55.05276343752910151, -170.0000000000000000, -35.21632399845986328 ) ) ;
#3248=B_SPLINE_CURVE_WITH_KNOTS ( 'NONE', 3,
 ( #59426, #53792, #31670, #11238, #47836, #49214, #32705, #5959, #43597, #65066, #63688, #15503, #60825, #49559, #23899, #11944, #44662, #65416, #40075, #7726, #23211, #61532, #34468, #13350, #33417, #55197, #65778, #17925, #54845, #12298, #28831, #66137, #7020, #22500, #1392, #6669, #66477, #28473, #29177, #28118, #2440, #50622, #55547, #61182, #45346 ),
 .UNSPECIFIED., .F., .F.,
 ( 4, 2, 2, 2, 2, 2, 2, 2, 2, 2, 2, 2, 2, 1, 2, 2, 2, 2, 2, 2, 2, 2, 4 ),
 ( 0.02356759485890610670, 0.02503765354686410607, 0.02577268289084311964, 0.02650771223482212974, 0.02797777092278016728, 0.02944782961073820482, 0.03018285895471723226, 0.03091788829869625971, 0.03238794698665432847, 0.03312297633063336633, 0.03385800567461240418, 0.03532806436257047294, 0.03606309370654950386, 0.03679812305052854171, 0.03753315239450757956, 0.03826818173848661048, 0.03973824042644467924, 0.04120829911440275495, 0.04267835780236083065, 0.04341338714633986851, 0.04414841649031891330, 0.04561847517827700288, 0.04708853386623509246 ),
 .UNSPECIFIED. ) ;
#3250=CARTESIAN_POINT ( 'NONE',  ( 9.288975942802419894, 6.379608420846962780, -39.26802939540083770 ) ) ;
#3253=EDGE_LOOP ( 'NONE', ( #43790, #62406 ) ) ;
#3256=CARTESIAN_POINT ( 'NONE',  ( -52.67596829228261868, 15.09584868440939331, 3.842776829869207766 ) ) ;
#3259=CARTESIAN_POINT ( 'NONE',  ( 117.6916924104495479, 32.48309187151382105, -15.56206514764637205 ) ) ;
#3260=CARTESIAN_POINT ( 'NONE',  ( 86.15454111412294935, 20.32174891186167898, -50.82156419891173726 ) ) ;
#3261=CARTESIAN_POINT ( 'NONE',  ( -171.5972879015330079, 86.93873520575962743, -88.51518996746024470 ) ) ;
#3265=CARTESIAN_POINT ( 'NONE',  ( 9.319975126229035567, -170.0000000000000000, 94.99999999999866418 ) ) ;
#3266=CARTESIAN_POINT ( 'NONE',  ( -179.1803008299640396, 95.71362642995448766, 87.57955674619184094 ) ) ;
#3269=LINE ( 'NONE', #67986, #50541 ) ;
#3270=CARTESIAN_POINT ( 'NONE',  ( -31.22562209718039128, 9.556395044504670366, -89.00629854612922998 ) ) ;
#3271=CARTESIAN_POINT ( 'NONE',  ( 201.2735851903138666, 103.4250806913139940, 83.71735717358380668 ) ) ;
#3272=CARTESIAN_POINT ( 'NONE',  ( 206.3053863259450225, 110.3084416756849748, 44.07829468878483681 ) ) ;
#3273=CYLINDRICAL_SURFACE ( 'NONE', #52235, 7.500000000000013323 ) ;
#3276=CARTESIAN_POINT ( 'NONE',  ( 13.37708032728286511, 7.441924986912760609, -23.28047698542330579 ) ) ;
#3281=AXIS2_PLACEMENT_3D ( 'NONE', #23321, #66243, #2207 ) ;
#3282=CARTESIAN_POINT ( 'NONE',  ( -142.5042386072303771, 59.74110826975217492, 8.639212595881256007 ) ) ;
#3283=CARTESIAN_POINT ( 'NONE',  ( 182.7745872728868335, 81.77554423487160307, -63.21223272561038442 ) ) ;
#3284=CARTESIAN_POINT ( 'NONE',  ( -147.7895256390024770, 64.04409735547015714, 72.42034331570219763 ) ) ;
#3285=CARTESIAN_POINT ( 'NONE',  ( -98.67723517640904163, 30.98797878696539243, -35.93232513735526368 ) ) ;
#3287=CARTESIAN_POINT ( 'NONE',  ( 32.14349651933088126, 7.576119504381656711, -45.07096977590022391 ) ) ;
#3288=CARTESIAN_POINT ( 'NONE',  ( -108.1144194775597640, 35.84457139767598477, 6.435316743732402145 ) ) ;
#3290=CARTESIAN_POINT ( 'NONE',  ( 126.4754729582248132, 37.14269484129875565, -42.16813892752784909 ) ) ;
#3291=ORIENTED_EDGE ( 'NONE', *, *, #18989, .F. ) ;
#3293=CARTESIAN_POINT ( 'NONE',  ( 187.0823097343935331, 86.37667841017882608, 94.99999999999866418 ) ) ;
#3295=CARTESIAN_POINT ( 'NONE',  ( -23.93880457192868860, 8.479983864459175180, -69.42207390290181479 ) ) ;
#3296=CARTESIAN_POINT ( 'NONE',  ( 10.13405324523498763, 6.385324379632245417, 5.717892688488246833 ) ) ;
#3297=CARTESIAN_POINT ( 'NONE',  ( 43.96421756700839722, 10.06386361114659778, -75.93710349221596800 ) ) ;
#3299=CARTESIAN_POINT ( 'NONE',  ( 175.8855729601531550, 73.50624012737689839, -75.99701591278079604 ) ) ;
#3301=CARTESIAN_POINT ( 'NONE',  ( 104.7034219878852213, 26.40210929103715998, 5.186479124812725772 ) ) ;
#3302=CARTESIAN_POINT ( 'NONE',  ( -25.79929641484368830, 9.749255553662434792, 59.59226522692620165 ) ) ;
#3305=CARTESIAN_POINT ( 'NONE',  ( -7.336760511143397778, 6.859209474528205952, 56.96013162991089018 ) ) ;
#3308=CARTESIAN_POINT ( 'NONE',  ( 152.8672128926847904, 55.41186463791521533, 57.82799647549036592 ) ) ;
#3309=DIRECTION ( 'NONE',  ( 0.000000000000000000, 0.000000000000000000, 1.000000000000000000 ) ) ;
#3310=CARTESIAN_POINT ( 'NONE',  ( 86.62931800182293784, -170.0000000000000000, 37.21208757247931942 ) ) ;
#3318=EDGE_CURVE ( 'NONE', #27441, #34992, #35911, .T. ) ;
#3321=CARTESIAN_POINT ( 'NONE',  ( -178.7483298110140595, 93.61800926271538970, -74.02109263234427772 ) ) ;
#3327=CARTESIAN_POINT ( 'NONE',  ( -0.3258398948454875321, 6.518608385615802803, 10.26970237692722598 ) ) ;
#3329=CARTESIAN_POINT ( 'NONE',  ( -81.01931326044683601, 24.31309346877659294, 45.04357807855111417 ) ) ;
#3330=VECTOR ( 'NONE', #15934, 1000.000000000000000 ) ;
#3331=CARTESIAN_POINT ( 'NONE',  ( -28.13527276074847450, 10.08983026464524890, -22.71023329608813057 ) ) ;
#3332=CARTESIAN_POINT ( 'NONE',  ( 133.8566784816069344, 41.42467568809808398, 2.665790248531674678 ) ) ;
#3335=EDGE_CURVE ( 'NONE', #49023, #5910, #12029, .T. ) ;
#3336=CARTESIAN_POINT ( 'NONE',  ( 112.1164716692773453, 29.75790342121400656, -36.14479581440889433 ) ) ;
#3337=CARTESIAN_POINT ( 'NONE',  ( 12.03194517566455701, 6.409266703743584870, 70.86927069785514277 ) ) ;
#3339=CARTESIAN_POINT ( 'NONE',  ( -77.17954427531354611, 22.83512059001850503, 84.24976070025458341 ) ) ;
#3340=CARTESIAN_POINT ( 'NONE',  ( -118.8429087385162148, 42.02330229425614050, 94.38756965892528683 ) ) ;
#3341=ORIENTED_EDGE ( 'NONE', *, *, #16818, .T. ) ;
#3342=CARTESIAN_POINT ( 'NONE',  ( 69.72564955710446100, 15.37006465677308498, 40.67263069985552448 ) ) ;
#3343=ORIENTED_EDGE ( 'NONE', *, *, #29208, .T. ) ;
#3347=CARTESIAN_POINT ( 'NONE',  ( -144.9287131874382055, 60.39056348581544142, 71.02503524604800589 ) ) ;
#3349=CARTESIAN_POINT ( 'NONE',  ( 197.3059626281005592, 96.72682679064187994, -69.35964093074025527 ) ) ;
#3351=CARTESIAN_POINT ( 'NONE',  ( -124.3250225421925563, 45.46958056770280621, 72.30208039458051417 ) ) ;
#3352=CARTESIAN_POINT ( 'NONE',  ( -80.32755469740936860, 24.04130076192507204, -8.453244365720355091 ) ) ;
#3353=CARTESIAN_POINT ( 'NONE',  ( -179.2210908201801089, 95.76260491022613053, -10.97533268791872274 ) ) ;
#3354=B_SPLINE_CURVE_WITH_KNOTS ( 'NONE', 3,
 ( #66889, #66539, #13404, #13745, #2505, #41175, #3204, #61246, #14444, #51036, #13067, #18327, #2850, #46094, #56305, #24317, #34867, #39785, #35201, #67238, #62634, #19364, #62275, #55971, #30278, #51726, #7783, #56656, #55613, #7442, #28894, #50347, #23955, #50681, #45405, #47127, #15478, #31996, #26718, #35897, #68590, #36932, #41863, #36591 ),
 .UNSPECIFIED., .F., .F.,
 ( 4, 2, 2, 2, 2, 2, 2, 2, 2, 2, 2, 2, 2, 2, 2, 2, 2, 2, 2, 2, 2, 4 ),
 ( 0.000000000000000000, 0.001472974678681649233, 0.002209462018022473849, 0.002945949357363298465, 0.004418924036044928616, 0.005891898714726559634, 0.007364873393408188050, 0.008101360732749003993, 0.008837848072089820803, 0.01031082275077145095, 0.01178379742945308284, 0.01252028476879389271, 0.01325677210813470605, 0.01472974678681633447, 0.01546623412615715301, 0.01620272146549796982, 0.01767569614417959997, 0.01914867082286123359, 0.01988515816220204346, 0.02062164550154285333, 0.02209462018022448002, 0.02356759485890610670 ),
 .UNSPECIFIED. ) ;
#3360=CARTESIAN_POINT ( 'NONE',  ( 102.7435092758398127, 25.56449004647817702, 64.22656014339364106 ) ) ;
#3369=CARTESIAN_POINT ( 'NONE',  ( 164.6499013411308852, 63.45576988183555756, -68.28286819017297660 ) ) ;
#3372=VERTEX_POINT ( 'NONE', #38403 ) ;
#3373=CARTESIAN_POINT ( 'NONE',  ( -152.4930836497867404, 68.09400557494208783, -22.35209726688142950 ) ) ;
#3374=CARTESIAN_POINT ( 'NONE',  ( -85.10774223992955001, 24.88053943842881566, 60.91269031592988625 ) ) ;
#3377=CARTESIAN_POINT ( 'NONE',  ( -62.41727141396692247, 17.83188754031766976, 39.30035831538882007 ) ) ;
#3379=VECTOR ( 'NONE', #14810, 1000.000000000000000 ) ;
#3380=CARTESIAN_POINT ( 'NONE',  ( 55.91133443650748802, 12.16263767238152838, 34.85883350782107470 ) ) ;
#3384=CARTESIAN_POINT ( 'NONE',  ( -102.2801239173131194, 33.91021738430207222, -23.17002667451225406 ) ) ;
#3386=CARTESIAN_POINT ( 'NONE',  ( 69.74037587279238437, 14.33355757956373999, -66.70732824439824071 ) ) ;
#3387=CARTESIAN_POINT ( 'NONE',  ( 133.6288034103010034, 41.28708886999548611, -24.17876034193200852 ) ) ;
#3388=CARTESIAN_POINT ( 'NONE',  ( 20.74561700410411191, 7.717362891868937425, -10.52513384833799748 ) ) ;
#3389=CARTESIAN_POINT ( 'NONE',  ( -105.4589068214114462, 34.42476264325678414, -76.16844833364910983 ) ) ;
#3392=CIRCLE ( 'NONE', #57276, 242.4895526022646379 ) ;
#3397=CARTESIAN_POINT ( 'NONE',  ( 186.7642514597452532, 86.02880938169744240, -38.82112059087446454 ) ) ;
#3398=EDGE_LOOP ( 'NONE', ( #5312, #26253 ) ) ;
#3402=CARTESIAN_POINT ( 'NONE',  ( 198.2588776805010582, 99.52972231602373654, 6.006846211185677298 ) ) ;
#3404=ADVANCED_FACE ( 'NONE', ( #59848 ), #16941, .F. ) ;
#3405=CARTESIAN_POINT ( 'NONE',  ( 150.3314594630236343, 53.54839609209004436, 92.90526760572284104 ) ) ;
#3407=CARTESIAN_POINT ( 'NONE',  ( 126.3732561463888686, 38.23795180971327312, -70.93242266372757854 ) ) ;
#3408=CARTESIAN_POINT ( 'NONE',  ( 126.6576865394845584, 37.24426596493989905, 39.13016143230759525 ) ) ;
#3411=DIRECTION ( 'NONE',  ( -0.000000000000000000, 1.000000000000000000, -0.000000000000000000 ) ) ;
#3413=CARTESIAN_POINT ( 'NONE',  ( -78.66644367742111399, 22.32174330031319798, 18.57365054920947500 ) ) ;
#3416=CARTESIAN_POINT ( 'NONE',  ( 61.33627421985470818, 12.28939706835343237, 44.62650739186889837 ) ) ;
#3418=EDGE_CURVE ( 'NONE', #41404, #63707, #39455, .T. ) ;
#3420=CARTESIAN_POINT ( 'NONE',  ( 173.6700117628886346, 72.79957362875113347, 37.97907060391748502 ) ) ;
#3421=CARTESIAN_POINT ( 'NONE',  ( 17.48889770758266593, 6.561062909825351674, -77.17229571346548767 ) ) ;
#3423=CARTESIAN_POINT ( 'NONE',  ( -132.4776673493542773, 52.21763813822160216, 61.36330782950730622 ) ) ;
#3427=ORIENTED_EDGE ( 'NONE', *, *, #48793, .T. ) ;
#3428=CARTESIAN_POINT ( 'NONE',  ( 210.9608386442062908, 117.1762372255315654, -66.53635089985841944 ) ) ;
#3429=CARTESIAN_POINT ( 'NONE',  ( 140.2058232509808704, 46.59155168125933244, 41.03386337616525736 ) ) ;
#3430=CARTESIAN_POINT ( 'NONE',  ( 115.7612476187723729, 32.64200929566222698, 42.21417507095826949 ) ) ;
#3432=CARTESIAN_POINT ( 'NONE',  ( 70.11969827741708627, 15.47408882293423993, -67.61050290499292714 ) ) ;
#3436=CARTESIAN_POINT ( 'NONE',  ( -142.0227972901369071, 59.36121938936274489, -16.02476559944369328 ) ) ;
#3437=CARTESIAN_POINT ( 'NONE',  ( -125.6703656163501677, 47.55170550253210138, -49.91370389823395470 ) ) ;
#3440=EDGE_CURVE ( 'NONE', #63135, #33282, #23294, .T. ) ;
#3444=EDGE_CURVE ( 'NONE', #31875, #38167, #35289, .T. ) ;
#3445=CARTESIAN_POINT ( 'NONE',  ( -146.7345109736526183, 61.86270848728295135, 45.19291357465738201 ) ) ;
#3446=CARTESIAN_POINT ( 'NONE',  ( 157.4703587214989113, 57.65129005721576760, 2.564916881789689018 ) ) ;
#3447=CARTESIAN_POINT ( 'NONE',  ( -171.0814041607219451, 84.88598211196838861, -76.28622867029723409 ) ) ;
#3449=CARTESIAN_POINT ( 'NONE',  ( -109.7790042512817905, 37.90666514836944145, 37.72788903940714533 ) ) ;
#3451=CARTESIAN_POINT ( 'NONE',  ( -37.38262509017739177, 10.64263598035110192, 15.47271197860792036 ) ) ;
#3452=CARTESIAN_POINT ( 'NONE',  ( 79.63513233364429311, 18.20496177163924401, 61.33758711607030989 ) ) ;
#3454=CARTESIAN_POINT ( 'NONE',  ( -79.09141991249970260, 22.48360285952615811, -88.80455181264525777 ) ) ;
#3456=DIRECTION ( 'NONE',  ( -0.000000000000000000, 1.000000000000000000, -0.000000000000000000 ) ) ;
#3459=CARTESIAN_POINT ( 'NONE',  ( -14.33576511807126153, 8.413127487936190363, -39.16238487774285204 ) ) ;
#3461=CARTESIAN_POINT ( 'NONE',  ( -37.07436112751821611, 11.60822760208522553, -10.99943049330883582 ) ) ;
#3464=ORIENTED_EDGE ( 'NONE', *, *, #39061, .F. ) ;
#3466=CARTESIAN_POINT ( 'NONE',  ( -58.75378739419585372, 16.75118858561005553, 58.12022478182042562 ) ) ;
#3467=CARTESIAN_POINT ( 'NONE',  ( -189.9554299271398179, 108.0836897899587825, 14.80701051291223891 ) ) ;
#3468=EDGE_LOOP ( 'NONE', ( #65720, #3807, #12439, #3464 ) ) ;
#3470=CARTESIAN_POINT ( 'NONE',  ( -8.314575874103553588, 6.922894809783094239, -77.26262132240753999 ) ) ;
#3471=CARTESIAN_POINT ( 'NONE',  ( -32.41982179707237322, 9.753975577087190985, 30.26490829174940345 ) ) ;
#3475=CARTESIAN_POINT ( 'NONE',  ( -156.9919426121902575, 72.16759471857098163, 65.62823907942903645 ) ) ;
#3476=CARTESIAN_POINT ( 'NONE',  ( -118.9649285217356294, 42.09781191014327817, 35.23770179663537760 ) ) ;
#3480=CARTESIAN_POINT ( 'NONE',  ( 90.91465859190770971, 20.92790537681858609, 57.89667315351857724 ) ) ;
#3483=CARTESIAN_POINT ( 'NONE',  ( -121.5677746760273834, 43.71038933438990171, -63.11338067390871487 ) ) ;
#3485=CARTESIAN_POINT ( 'NONE',  ( 203.9276061909315274, 105.2889220654478919, 29.20772073876941377 ) ) ;
#3488=CARTESIAN_POINT ( 'NONE',  ( 140.8855094313932739, 47.03549517811091363, 12.79525956615474236 ) ) ;
#3494=CARTESIAN_POINT ( 'NONE',  ( 162.0862735437575850, 62.63196145447161456, -22.71030774999397650 ) ) ;
#3495=ORIENTED_EDGE ( 'NONE', *, *, #8743, .F. ) ;
#3496=CARTESIAN_POINT ( 'NONE',  ( 70.26639875985988226, 15.51307715494295358, 66.13948629930069956 ) ) ;
#3497=CARTESIAN_POINT ( 'NONE',  ( 126.9909055734727019, 37.43041694803015673, 93.80275659116571774 ) ) ;
#3499=EDGE_CURVE ( 'NONE', #37504, #7511, #66212, .T. ) ;
#3502=CARTESIAN_POINT ( 'NONE',  ( 163.1313205310724470, 63.49733392291054201, -38.69832981363442315 ) ) ;
#3505=CARTESIAN_POINT ( 'NONE',  ( 160.4963793545268800, 60.04225845346905999, -50.50113425675434797 ) ) ;
#3507=CARTESIAN_POINT ( 'NONE',  ( -96.02159028238558847, 30.82695531378848841, 15.31486708033657784 ) ) ;
#3508=CARTESIAN_POINT ( 'NONE',  ( 55.59973583101010774, 12.10012336970133262, 89.83280078296678539 ) ) ;
#3509=CARTESIAN_POINT ( 'NONE',  ( 150.6472384575835122, 53.77757500042995531, -94.17017552904665934 ) ) ;
#3510=CARTESIAN_POINT ( 'NONE',  ( 82.34401416830215226, 19.05992892018826623, -22.63702806220790364 ) ) ;
#3511=CARTESIAN_POINT ( 'NONE',  ( -178.9182503768213621, 95.39606678475963975, -91.13644876916208659 ) ) ;
#3512=CARTESIAN_POINT ( 'NONE',  ( 150.0889146124742695, 52.13243511955542431, 62.39775547893556507 ) ) ;
#3513=CARTESIAN_POINT ( 'NONE',  ( -142.0747101610765242, 59.40211529287933701, -95.00000000000133582 ) ) ;
#3515=CARTESIAN_POINT ( 'NONE',  ( -101.8187363387487494, 33.67461140603123937, 57.36362509687881328 ) ) ;
#3516=CARTESIAN_POINT ( 'NONE',  ( 181.0840389613909736, -170.0000000000000000, -97.41415884680698412 ) ) ;
#3519=CARTESIAN_POINT ( 'NONE',  ( -56.33023788822384859, 15.02754539266624789, 84.10929812850636722 ) ) ;
#3522=CARTESIAN_POINT ( 'NONE',  ( 59.54768723222450433, 11.89486923077556035, 84.34372402572785177 ) ) ;
#3524=CARTESIAN_POINT ( 'NONE',  ( 185.1710994180822638, 84.30654632312743502, 16.26852148075597171 ) ) ;
#3525=CARTESIAN_POINT ( 'NONE',  ( 210.6475357757681763, 114.8748261044495962, -48.39950946580693625 ) ) ;
#3526=CARTESIAN_POINT ( 'NONE',  ( 173.5837434292113528, 71.34409607026157119, 9.675991114982885222 ) ) ;
#3527=CARTESIAN_POINT ( 'NONE',  ( -61.86845765289634613, 16.61548683002699534, 7.833006060118358427 ) ) ;
#3536=CARTESIAN_POINT ( 'NONE',  ( -10.99038543402095058, 7.117699646488151011, 84.49731268521362892 ) ) ;
#3539=CARTESIAN_POINT ( 'NONE',  ( -71.67841390531690138, 19.78168466957075822, 62.02784106711190049 ) ) ;
#3540=CARTESIAN_POINT ( 'NONE',  ( -169.1041038606267648, 82.76530082651282783, 58.81708485632820071 ) ) ;
#3542=VERTEX_POINT ( 'NONE', #55148 ) ;
#3543=CARTESIAN_POINT ( 'NONE',  ( -156.6692143066620702, 70.50016761530885390, 35.97663252705407899 ) ) ;
#3546=CARTESIAN_POINT ( 'NONE',  ( 174.6176230994777541, 72.30829341023246570, -13.04120643648126965 ) ) ;
#3548=CARTESIAN_POINT ( 'NONE',  ( -170.2856292770789821, 85.50720222068220266, 58.20975371259029174 ) ) ;
#3550=CARTESIAN_POINT ( 'NONE',  ( 55.52751777340359496, 12.08567914268656729, -15.88646113736828447 ) ) ;
#3551=ORIENTED_EDGE ( 'NONE', *, *, #14250, .T. ) ;
#3554=CARTESIAN_POINT ( 'NONE',  ( 212.1700216741375300, 117.1889356120871497, 9.135482143913240094 ) ) ;
#3555=CARTESIAN_POINT ( 'NONE',  ( 14.80291736570134731, 7.477373894757625372, 71.81068398635675010 ) ) ;
#3557=CARTESIAN_POINT ( 'NONE',  ( 15.36604569585143309, 6.487299053250196401, -89.20804527961311692 ) ) ;
#3561=B_SPLINE_CURVE_WITH_KNOTS ( 'NONE', 3,
 ( #18057, #50751, #28966, #29297, #13471, #51106, #18394, #34241, #56727, #39510, #40887, #39851, #61309, #46158, #60957, #23679, #61652, #7514, #35269, #24028, #67633, #56371, #34929, #34599, #29641, #2571, #7851, #8193, #62348, #50060, #2915, #29993, #13134, #45823, #51454, #12779, #14161, #35622, #55682, #15877, #4975, #19782, #25069, #52477, #63032 ),
 .UNSPECIFIED., .F., .F.,
 ( 4, 2, 2, 2, 2, 2, 2, 2, 2, 2, 2, 2, 2, 1, 2, 2, 2, 2, 2, 2, 2, 2, 4 ),
 ( 0.02352719711393054525, 0.02499986300757018470, 0.02573619595438999402, 0.02647252890120980334, 0.02794519479484942198, 0.02941786068848904062, 0.03015419363530885341, 0.03089052658212866620, 0.03236319247576828484, 0.03309952542258809416, 0.03383585836940790348, 0.03530852426304752212, 0.03604485720986733144, 0.03678119015668713382, 0.03751752310350694314, 0.03825385605032674552, 0.03972652194396637804, 0.04119918783760599668, 0.04267185373124562919, 0.04340818667806543157, 0.04414451962488523395, 0.04561718551852482484, 0.04708985141216440878 ),
 .UNSPECIFIED. ) ;
#3563=ORIENTED_EDGE ( 'NONE', *, *, #52893, .T. ) ;
#3566=CARTESIAN_POINT ( 'NONE',  ( 39.40195752203892710, 9.424259417798133143, -77.46436805589148378 ) ) ;
#3567=CARTESIAN_POINT ( 'NONE',  ( 181.0840389613909736, -170.0000000000000000, -97.41415884680698412 ) ) ;
#3568=CARTESIAN_POINT ( 'NONE',  ( 16.44502386301708086, 6.521830180776601260, 83.70387535602117168 ) ) ;
#3569=CARTESIAN_POINT ( 'NONE',  ( 23.17379743143359505, 7.857626726498480707, 92.54999467873835783 ) ) ;
#3571=FACE_OUTER_BOUND ( 'NONE', #7865, .T. ) ;
#3572=CARTESIAN_POINT ( 'NONE',  ( 197.3064269725218765, 98.33232022113057269, -42.51203141086486426 ) ) ;
#3573=ORIENTED_EDGE ( 'NONE', *, *, #17782, .T. ) ;
#3576=CARTESIAN_POINT ( 'NONE',  ( -85.45399718454959270, 25.02415453493130570, -66.25966646325893805 ) ) ;
#3577=CARTESIAN_POINT ( 'NONE',  ( -55.05276343752908730, 15.72344139423347720, -8.371773407996169425 ) ) ;
#3578=EDGE_CURVE ( 'NONE', #9829, #58885, #61487, .T. ) ;
#3579=ORIENTED_EDGE ( 'NONE', *, *, #59019, .T. ) ;
#3580=EDGE_CURVE ( 'NONE', #63871, #16484, #61932, .T. ) ;
#3583=CARTESIAN_POINT ( 'NONE',  ( 44.34362023773823580, 10.12115849931653067, 58.59490733264918561 ) ) ;
#3585=CARTESIAN_POINT ( 'NONE',  ( 22.52576749827964164, 6.809805260274345073, 7.338887533324804480 ) ) ;
#3587=ORIENTED_EDGE ( 'NONE', *, *, #68829, .T. ) ;
#3591=CARTESIAN_POINT ( 'NONE',  ( -28.04483122278597662, 9.058704822772433829, 84.70984886725781848 ) ) ;
#3592=CARTESIAN_POINT ( 'NONE',  ( 173.6007744016332595, 72.73482010729017588, -69.98774395762167444 ) ) ;
#3594=CARTESIAN_POINT ( 'NONE',  ( 108.3906473026529653, 28.03385344351496400, -36.13980848578636085 ) ) ;
#3595=B_SPLINE_CURVE_WITH_KNOTS ( 'NONE', 3,
 ( #22887, #61570, #39763, #40113, #55948, #7763, #61898, #66863, #18662, #40453, #13385, #61220 ),
 .UNSPECIFIED., .F., .F.,
 ( 4, 2, 2, 2, 2, 4 ),
 ( 0.000000000000000000, 0.002486957010932606960, 0.004973914021865213919, 0.007460871032797820011, 0.008704349538264120889, 0.009947828043730422634 ),
 .UNSPECIFIED. ) ;
#3597=CARTESIAN_POINT ( 'NONE',  ( 79.12879321038293767, 18.04902206524925745, -43.08565838544853221 ) ) ;
#3598=CARTESIAN_POINT ( 'NONE',  ( -165.7614670400926684, 80.73254387118949182, -94.42993858856560507 ) ) ;
#3599=ORIENTED_EDGE ( 'NONE', *, *, #2055, .F. ) ;
#3600=ORIENTED_EDGE ( 'NONE', *, *, #15027, .F. ) ;
#3601=CARTESIAN_POINT ( 'NONE',  ( -79.14638003838382474, 23.58242782405880078, -61.96000122218159589 ) ) ;
#3607=CARTESIAN_POINT ( 'NONE',  ( -119.5563837756079693, 43.64229894412652300, -65.21578466046432254 ) ) ;
#3608=CARTESIAN_POINT ( 'NONE',  ( 211.7357196141372242, 118.3691710715567211, 39.31684144783690726 ) ) ;
#3609=CARTESIAN_POINT ( 'NONE',  ( -84.53753601793931693, 25.73343139558517478, 60.06906254790580135 ) ) ;
#3611=ORIENTED_EDGE ( 'NONE', *, *, #13648, .T. ) ;
#3612=CARTESIAN_POINT ( 'NONE',  ( 11.20486344102687504, 7.403248964808831545, -10.21748692402197634 ) ) ;
#3613=VERTEX_POINT ( 'NONE', #28786 ) ;
#3614=CARTESIAN_POINT ( 'NONE',  ( 198.7084915431530305, 98.47675983942194478, -21.50361554362704553 ) ) ;
#3615=ORIENTED_EDGE ( 'NONE', *, *, #30109, .T. ) ;
#3616=DIRECTION ( 'NONE',  ( -0.000000000000000000, 1.000000000000000000, -0.000000000000000000 ) ) ;
#3617=CARTESIAN_POINT ( 'NONE',  ( 183.1873354889582686, 82.20882912211249050, -77.78155292010042388 ) ) ;
#3618=CARTESIAN_POINT ( 'NONE',  ( -190.6985136298601731, 109.1272424661242582, -95.00000000000133582 ) ) ;
#3620=CARTESIAN_POINT ( 'NONE',  ( 34.45817031441434608, 7.817703378455679086, -48.78147938101668757 ) ) ;
#3622=CARTESIAN_POINT ( 'NONE',  ( 9.045716588192243890, 7.384596431530736638, -39.69777131749945198 ) ) ;
#3623=CARTESIAN_POINT ( 'NONE',  ( 128.9253503890652439, 38.52561778336671239, -49.17949685352920852 ) ) ;
#3628=PLANE ( 'NONE',  #3844 ) ;
#3634=CARTESIAN_POINT ( 'NONE',  ( 186.0827296088607170, 85.28826835108064586, -11.28428718647697693 ) ) ;
#3635=CARTESIAN_POINT ( 'NONE',  ( 209.6698611676810629, 115.2210955123518090, 15.49623849697043632 ) ) ;
#3637=CARTESIAN_POINT ( 'NONE',  ( -180.6011569556094969, 95.85968111394265634, -42.84200977746586858 ) ) ;
#3638=CARTESIAN_POINT ( 'NONE',  ( 91.51282003084293137, 21.14522045960332264, -10.76386589503217728 ) ) ;
#3639=CARTESIAN_POINT ( 'NONE',  ( -23.93895920923072751, 9.495000752338448535, 64.31892236427358966 ) ) ;
#3640=FACE_OUTER_BOUND ( 'NONE', #7061, .T. ) ;
#3641=CARTESIAN_POINT ( 'NONE',  ( -55.05276343752910151, 14.68156374112636797, 72.16187836339486239 ) ) ;
#3645=CARTESIAN_POINT ( 'NONE',  ( -3.244108878396729345, 6.635632329121485817, 70.41866219491829781 ) ) ;
#3650=CARTESIAN_POINT ( 'NONE',  ( 157.2533363798599169, 58.75760182111574892, 56.25401806271707272 ) ) ;
#3652=CARTESIAN_POINT ( 'NONE',  ( -49.45858366215606594, 13.25262207532078484, -47.71791105718050119 ) ) ;
#3655=EDGE_LOOP ( 'NONE', ( #54292, #41870 ) ) ;
#3656=CARTESIAN_POINT ( 'NONE',  ( -189.5593729888621510, 107.5326066953720527, -93.58956526689634359 ) ) ;
#3660=CYLINDRICAL_SURFACE ( 'NONE', #51048, 7.500000000000013323 ) ;
#3661=CARTESIAN_POINT ( 'NONE',  ( -178.0658882571760842, 92.80593104957419825, -74.70044367160248555 ) ) ;
#3668=CARTESIAN_POINT ( 'NONE',  ( 58.47885130911550533, 12.69429933094348328, -49.21325034717124680 ) ) ;
#3670=CARTESIAN_POINT ( 'NONE',  ( -23.98747857548121942, 9.501432345103355104, -14.98739851332648954 ) ) ;
#3671=CARTESIAN_POINT ( 'NONE',  ( 135.6651581599210488, 42.52720121194705882, 2.883460403371903347 ) ) ;
#3674=CARTESIAN_POINT ( 'NONE',  ( 15.29293866748104236, 6.484959508098437020, 71.85925826316895382 ) ) ;
#3679=CARTESIAN_POINT ( 'NONE',  ( 63.98689050258324329, 13.93365232918667651, 44.76545543697432095 ) ) ;
#3680=ORIENTED_EDGE ( 'NONE', *, *, #8167, .T. ) ;
#3682=VERTEX_POINT ( 'NONE', #15998 ) ;
#3684=CARTESIAN_POINT ( 'NONE',  ( -143.2464978228198902, 59.04559547356110727, 69.20284246303761222 ) ) ;
#3687=CARTESIAN_POINT ( 'NONE',  ( 184.3994103300443328, 82.02159554764421046, -10.13810525658259465 ) ) ;
#3689=CARTESIAN_POINT ( 'NONE',  ( -118.9468627709228912, 42.08677365399179848, 67.80319248315890945 ) ) ;
#3690=CARTESIAN_POINT ( 'NONE',  ( -84.55783695959767954, 25.74181993349144904, -11.10319101795209029 ) ) ;
#3691=FACE_OUTER_BOUND ( 'NONE', #25914, .T. ) ;
#3693=CARTESIAN_POINT ( 'NONE',  ( -51.77431913897919458, 14.86466849149170955, 44.58036524786519550 ) ) ;
#3695=ORIENTED_EDGE ( 'NONE', *, *, #26987, .F. ) ;
#3699=CARTESIAN_POINT ( 'NONE',  ( 105.2351883444108722, 26.63316404209145460, 85.20707925349449852 ) ) ;
#3700=CARTESIAN_POINT ( 'NONE',  ( -55.05276343752910151, -170.0000000000000000, 10.97277718246748890 ) ) ;
#3701=EDGE_CURVE ( 'NONE', #25401, #56789, #25051, .T. ) ;
#3704=CARTESIAN_POINT ( 'NONE',  ( -145.1827711476570641, 61.89240998680990913, 85.77519060852361577 ) ) ;
#3706=ORIENTED_EDGE ( 'NONE', *, *, #48102, .T. ) ;
#3708=CARTESIAN_POINT ( 'NONE',  ( 175.5364600822697412, 73.17492830764774681, -92.34967047772518356 ) ) ;
#3711=B_SPLINE_CURVE_WITH_KNOTS ( 'NONE', 3,
 ( #43384, #22634, #7155, #22285, #5749, #44073, #64854, #28616, #65556, #27554, #11031, #48998, #39176, #64506, #11371, #43723, #11724, #28251, #22989, #33556, #16654, #65200, #21583, #54982, #16995, #17349, #27205, #6800, #38464, #59902, #38110, #50065, #16313, #33197, #54635, #6462, #65921, #49696, #38823, #60619, #1526, #44433, #37769, #34246 ),
 .UNSPECIFIED., .F., .F.,
 ( 4, 2, 2, 2, 2, 2, 2, 2, 2, 2, 2, 2, 1, 2, 2, 2, 2, 2, 2, 1, 2, 2, 4 ),
 ( 0.02381751147647563974, 0.02531129726520767523, 0.02605819015957369644, 0.02680508305393972113, 0.02829886884267175662, 0.02979265463140379211, 0.03053954752576980639, 0.03128644042013582066, 0.03278022620886785615, 0.03427401199759988470, 0.03576779778633192713, 0.03651469068069795182, 0.03726158357506398344, 0.03800847646943000813, 0.03875536936379603975, 0.04024915515252809606, 0.04174294094126015930, 0.04323672672999220867, 0.04398361962435823336, 0.04473051251872425804, 0.04547740541309028273, 0.04622429830745630741, 0.04771808409618833596 ),
 .UNSPECIFIED. ) ;
#3712=CARTESIAN_POINT ( 'NONE',  ( -59.95412189755933952, 17.09836075175410386, 32.11962012825880919 ) ) ;
#3713=CARTESIAN_POINT ( 'NONE',  ( -38.54712373114178803, 11.89174538567465689, -72.10478228046926574 ) ) ;
#3715=CARTESIAN_POINT ( 'NONE',  ( 9.288975942802414565, 6.379608420846960115, -12.42347880493715806 ) ) ;
#3717=CARTESIAN_POINT ( 'NONE',  ( -0.3258398948454875876, 6.518608385615804579, -43.41939880400013863 ) ) ;
#3718=CARTESIAN_POINT ( 'NONE',  ( 182.7720841008444381, 80.32850885226594073, 56.34244215664639199 ) ) ;
#3719=CARTESIAN_POINT ( 'NONE',  ( -118.3960663196800880, 41.75130200162919891, 10.70744975955315148 ) ) ;
#3721=CARTESIAN_POINT ( 'NONE',  ( 17.48889770758268014, 6.561062909825351674, 57.05045723885289988 ) ) ;
#3722=CARTESIAN_POINT ( 'NONE',  ( 23.24047374271773236, 7.861801299833793166, -15.19526073016659140 ) ) ;
#3723=CARTESIAN_POINT ( 'NONE',  ( 9.045716588192243890, 7.384596431530730420, 13.99132986342793572 ) ) ;
#3724=EDGE_CURVE ( 'NONE', #45155, #23284, #31659, .T. ) ;
#3726=B_SPLINE_CURVE_WITH_KNOTS ( 'NONE', 3,
 ( #4730, #26196, #9327, #68744, #41681, #47630, #30437, #51886, #5075, #58202, #36063, #58531, #47975, #25522, #52233, #69084, #69441, #3699, #20561, #63829, #14942, #42024, #21257, #20917, #42368, #57175, #15641, #31143, #8990, #52578, #46606, #68087, #19887, #41345, #62797, #14601, #57518, #30788, #57860, #36407, #68421, #20223, #4397, #63484, #59564, #5428, #32167, #21944, #53936, #43734, #10692, #37781, #54991, #59916, #27566, #11735 ),
 .UNSPECIFIED., .F., .F.,
 ( 4, 2, 2, 2, 2, 2, 2, 2, 2, 2, 2, 2, 2, 2, 2, 2, 2, 2, 2, 2, 2, 2, 2, 2, 2, 2, 2, 4 ),
 ( 0.000000000000000000, 0.002104237472784967113, 0.003156356209177476474, 0.004208474945569985401, 0.005260593681962493461, 0.006312712418355004122, 0.007364831154747513049, 0.008416949891140022844, 0.01052118736392504070, 0.01157330610031757911, 0.01262542483671011927, 0.01367754357310265942, 0.01472966230949519784, 0.01683389978228026426, 0.01788601851867279574, 0.01893813725506532722, 0.01999025599145785870, 0.02104237472785039018, 0.02314661220063543579, 0.02419873093702797420, 0.02525084967342050915, 0.02630296840981304410, 0.02735508714620558252, 0.02840720588259811746, 0.02945932461899065241, 0.03051144335538318736, 0.03156356209177572231, 0.03366779956456074363 ),
 .UNSPECIFIED. ) ;
#3733=CARTESIAN_POINT ( 'NONE',  ( -103.2164890789475606, 34.39030697009940951, -35.05845294305762394 ) ) ;
#3735=CARTESIAN_POINT ( 'NONE',  ( 188.4920037102894241, 87.93425473911916868, -42.51552582893779686 ) ) ;
#3739=AXIS2_PLACEMENT_3D ( 'NONE', #60067, #28413, #22097 ) ;
#3740=CARTESIAN_POINT ( 'NONE',  ( -27.70562707895080479, 9.007984652865417274, -22.49608191275522628 ) ) ;
#3746=CARTESIAN_POINT ( 'NONE',  ( 163.9480004224415666, 64.17952544697072881, 94.44126775434629906 ) ) ;
#3751=CARTESIAN_POINT ( 'NONE',  ( -152.9143627383495527, 68.46626892668658115, 44.91786962733564792 ) ) ;
#3752=CIRCLE ( 'NONE', #29602, 243.4957430088094839 ) ;
#3761=EDGE_LOOP ( 'NONE', ( #20378, #17915 ) ) ;
#3763=CARTESIAN_POINT ( 'NONE',  ( -32.29264255508331871, 10.75330965162339147, -89.05198297107156691 ) ) ;
#3764=CARTESIAN_POINT ( 'NONE',  ( -132.5976199670998881, 52.30296609017646148, 61.59159971231706265 ) ) ;
#3766=CARTESIAN_POINT ( 'NONE',  ( -104.6733177284973522, 35.14812073506915624, 84.57539980412138902 ) ) ;
#3770=CARTESIAN_POINT ( 'NONE',  ( -131.2955621888335429, 51.38237199780173370, -74.48357675656784238 ) ) ;
#3772=CARTESIAN_POINT ( 'NONE',  ( 112.1100957124161397, 30.86846953551571104, 29.83213851092833835 ) ) ;
#3774=CARTESIAN_POINT ( 'NONE',  ( 64.69738688745238164, 14.10375742873388383, -62.75224125784992424 ) ) ;
#3775=VERTEX_POINT ( 'NONE', #7191 ) ;
#3776=VERTEX_POINT ( 'NONE', #34281 ) ;
#3779=CARTESIAN_POINT ( 'NONE',  ( -166.7049310409072405, 80.25944422923581101, -38.31930149277814479 ) ) ;
#3781=AXIS2_PLACEMENT_3D ( 'NONE', #3700, #24820, #24487 ) ;
#3782=CARTESIAN_POINT ( 'NONE',  ( -48.84172885504641215, 13.10362374101116956, -92.17860550746377157 ) ) ;
#3783=CARTESIAN_POINT ( 'NONE',  ( -50.65633458199173589, 14.58352428224076114, -90.32529372262172274 ) ) ;
#3786=CARTESIAN_POINT ( 'NONE',  ( 69.72789637502502558, 15.37065610545704253, -46.57588281048915491 ) ) ;
#3789=CARTESIAN_POINT ( 'NONE',  ( 210.6475357757681763, 114.8748261044495678, 58.97869289604779652 ) ) ;
#3794=EDGE_CURVE ( 'NONE', #9029, #24506, #17753, .T. ) ;
#3795=CARTESIAN_POINT ( 'NONE',  ( 79.40386128751609363, 18.13359811229536689, -95.00000000000133582 ) ) ;
#3797=CARTESIAN_POINT ( 'NONE',  ( 79.12879321038292346, 18.04902206524926811, 64.29254397640617924 ) ) ;
#3799=CARTESIAN_POINT ( 'NONE',  ( -83.74395355181556511, 24.32073993326131855, -90.76757344677447747 ) ) ;
#3803=CARTESIAN_POINT ( 'NONE',  ( 34.83825437341838693, 7.859462995505725580, 4.597600571500676025 ) ) ;
#3807=ORIENTED_EDGE ( 'NONE', *, *, #56294, .T. ) ;
#3808=CARTESIAN_POINT ( 'NONE',  ( -118.9946151492785162, 43.29610461813053490, -93.12245335861705087 ) ) ;
#3810=CARTESIAN_POINT ( 'NONE',  ( 63.01563776193091826, -170.0000000000000000, 44.81296093922130552 ) ) ;
#3811=CARTESIAN_POINT ( 'NONE',  ( 11.21312910819262498, 7.403355431336988701, -75.82688043949028156 ) ) ;
#3812=CARTESIAN_POINT ( 'NONE',  ( -189.2346268516247392, 107.0830361517164988, 11.78999996383570092 ) ) ;
#3814=CARTESIAN_POINT ( 'NONE',  ( 15.78827728214693060, 6.500811158483329244, 71.85925826316895382 ) ) ;
#3815=CARTESIAN_POINT ( 'NONE',  ( -15.32550079334879456, 7.496023944924843363, -70.00453783701779287 ) ) ;
#3822=CARTESIAN_POINT ( 'NONE',  ( -156.4797890011541313, 71.69341087347112307, 62.28821244478771746 ) ) ;
#3823=CARTESIAN_POINT ( 'NONE',  ( 173.8623159076319382, 72.97967239795016781, -18.92509683218599292 ) ) ;
#3824=CARTESIAN_POINT ( 'NONE',  ( -119.6995109608661352, 42.54844499216734022, 33.88379391638913773 ) ) ;
#3826=ORIENTED_EDGE ( 'NONE', *, *, #64880, .T. ) ;
#3827=CARTESIAN_POINT ( 'NONE',  ( -174.7817412490651918, 90.52199442492062076, -76.38243644640435548 ) ) ;
#3828=CARTESIAN_POINT ( 'NONE',  ( 127.5112704970419486, 38.87838270771662508, 94.71298516231503584 ) ) ;
#3829=CARTESIAN_POINT ( 'NONE',  ( 116.5096233816161941, 31.89062767870468917, 32.98306140069937697 ) ) ;
#3832=B_SPLINE_CURVE_WITH_KNOTS ( 'NONE', 3,
 ( #4490, #35113, #59611, #11427, #53647, #6154, #65621, #64917, #53983, #894, #43096, #22347, #38170, #186, #33615, #43784, #37832, #59273, #32552, #21997, #60329, #27616, #37477, #59967, #16023, #28314, #65258, #42751, #17051, #38521, #10746, #26927, #11784, #11090, #32897, #55041, #6864, #16712, #48701, #32216, #54335, #33260, #5472, #48353, #5809, #21642, #49059, #17408 ),
 .UNSPECIFIED., .F., .F.,
 ( 4, 2, 2, 2, 2, 2, 2, 2, 2, 2, 2, 2, 2, 2, 2, 2, 2, 2, 2, 2, 2, 2, 2, 4 ),
 ( 0.000000000000000000, 0.001591515129442197789, 0.003183030258884395579, 0.003978787823605494690, 0.004774545388326592935, 0.006366060517768843199, 0.007957575647211093464, 0.009549090776653343729, 0.01034484834137447233, 0.01114060590609559920, 0.01193636347081672780, 0.01273212103553785467, 0.01432363616498015003, 0.01591515129442242979, 0.01671090885914355492, 0.01750666642386468699, 0.01830242398858581906, 0.01909818155330694767, 0.02068969668274926385, 0.02148545424747042368, 0.02228121181219158004, 0.02387272694163383377, 0.02466848450635492074, 0.02546424207107600771 ),
 .UNSPECIFIED. ) ;
#3833=CARTESIAN_POINT ( 'NONE',  ( -123.4416615615273116, 44.90042688650401459, -62.16667402822235289 ) ) ;
#3836=CARTESIAN_POINT ( 'NONE',  ( 198.7029050523553053, 98.46895521196215384, 41.24356943943517706 ) ) ;
#3837=CARTESIAN_POINT ( 'NONE',  ( 117.6916924104495479, 32.48309187151382105, -69.25116632857373133 ) ) ;
#3838=AXIS2_PLACEMENT_3D ( 'NONE', #23707, #33916, #6824 ) ;
#3839=FACE_OUTER_BOUND ( 'NONE', #25670, .T. ) ;
#3840=CARTESIAN_POINT ( 'NONE',  ( 140.4641697461913168, 46.75994457266055093, 13.75233122400834240 ) ) ;
#3842=EDGE_CURVE ( 'NONE', #19257, #9227, #44476, .T. ) ;
#3844=AXIS2_PLACEMENT_3D ( 'NONE', #9257, #52168, #68354 ) ;
#3847=FACE_OUTER_BOUND ( 'NONE', #29740, .T. ) ;
#3848=AXIS2_PLACEMENT_3D ( 'NONE', #39912, #7213, #45186 ) ;
#3851=CARTESIAN_POINT ( 'NONE',  ( 141.3359578064694233, 46.12776601070872573, 91.36406821307745929 ) ) ;
#3855=CARTESIAN_POINT ( 'NONE',  ( -180.4643341113398094, 95.69224917234934935, 39.87708186227253293 ) ) ;
#3857=CARTESIAN_POINT ( 'NONE',  ( 117.6924004117966263, 33.61107268965020722, -44.43629281926136088 ) ) ;
#3861=CARTESIAN_POINT ( 'NONE',  ( 55.52491259852590133, 12.08515669078798460, 90.50025533462843441 ) ) ;
#3865=CARTESIAN_POINT ( 'NONE',  ( 151.1607415860635228, 52.90668588398091288, 59.66759169391354334 ) ) ;
#3868=CARTESIAN_POINT ( 'NONE',  ( -97.49665543375864729, 31.53324358035376918, 70.66128095698653055 ) ) ;
#3872=CARTESIAN_POINT ( 'NONE',  ( -61.09101882797757099, 16.38378112650486784, 87.01151449968797635 ) ) ;
#3873=CARTESIAN_POINT ( 'NONE',  ( 107.0447263249841257, 28.53200276018954895, 43.89932290840497586 ) ) ;
#3876=CARTESIAN_POINT ( 'NONE',  ( 188.5651904823862139, 88.01586411309102687, 10.57501070353481509 ) ) ;
#3878=CARTESIAN_POINT ( 'NONE',  ( 173.6718135456487175, 71.42581476597409562, 11.14533547892623488 ) ) ;
#3881=AXIS2_PLACEMENT_3D ( 'NONE', #38901, #22708, #12166 ) ;
#3888=CARTESIAN_POINT ( 'NONE',  ( 15.78827728214693416, 7.507518794609575608, 45.01470767270524931 ) ) ;
#3889=CARTESIAN_POINT ( 'NONE',  ( -109.7643866341847172, 37.89854104106755273, -16.22134575533492651 ) ) ;
#3890=VECTOR ( 'NONE', #56233, 1000.000000000000000 ) ;
#3893=CARTESIAN_POINT ( 'NONE',  ( 199.6034222400379861, 99.61037244215080477, -91.99663670549787753 ) ) ;
#3898=B_SPLINE_CURVE_WITH_KNOTS ( 'NONE', 3,
 ( #34732, #13272, #3066, #45964, #56169, #19575, #7986, #35411, #56877, #2712, #30145, #24174, #51595, #45623, #3402, #41032, #53973, #52612, #5116, #43087, #20957, #26579, #11080, #64203, #16015, #59266, #32209, #10387, #41726, #58573, #9721, #37824, #36447, #48693, #4437, #21635, #69127, #57899, #63184, #15339, #64556, #5463, #31184, #37467, #31859, #25899, #47328, #42410, #52949, #42744 ),
 .UNSPECIFIED., .F., .F.,
 ( 4, 2, 2, 2, 2, 2, 2, 2, 2, 2, 2, 2, 2, 2, 2, 2, 2, 2, 2, 2, 2, 2, 2, 2, 4 ),
 ( 0.03296461860586794024, 0.03492857779726578349, 0.03689253698866362674, 0.03885649618006146999, 0.04082045537145931324, 0.04278441456285715649, 0.04376639415855611281, 0.04474837375425506913, 0.04573035334995402545, 0.04671233294565298177, 0.04720332274350245300, 0.04769431254135192422, 0.04867629213705086666, 0.04965827173274981604, 0.05064025132844876542, 0.05162223092414770786, 0.05260421051984665031, 0.05358619011554559969, 0.05456816971124454907, 0.05555014930694349151, 0.05653212890264243395, 0.05849608809404029108, 0.06046004728543815515, 0.06242400647683601922, 0.06438796566823387635 ),
 .UNSPECIFIED. ) ;
#3899=CARTESIAN_POINT ( 'NONE',  ( -155.7495771807047333, 69.65980221699319941, 34.03292314250037975 ) ) ;
#3900=DIRECTION ( 'NONE',  ( -0.000000000000000000, 1.000000000000000000, -0.000000000000000000 ) ) ;
#3901=CARTESIAN_POINT ( 'NONE',  ( 173.7227242028391174, 71.47307702680407715, -18.34505588493575345 ) ) ;
#3907=DIRECTION ( 'NONE',  ( -0.000000000000000000, 1.000000000000000000, -0.000000000000000000 ) ) ;
#3909=CARTESIAN_POINT ( 'NONE',  ( 212.1962110266999559, 117.2292732107321314, 9.486508075812803753 ) ) ;
#3910=CARTESIAN_POINT ( 'NONE',  ( 8.287863202055538281, 7.382585476140732794, 64.84750261709777419 ) ) ;
#3911=CARTESIAN_POINT ( 'NONE',  ( 204.6977192012829789, 106.3443248447423599, 29.20772073876942088 ) ) ;
#3912=FACE_BOUND ( 'NONE', #27307, .T. ) ;
#3916=CARTESIAN_POINT ( 'NONE',  ( -119.6460721175663480, 43.69798148487400624, 87.64758983319130436 ) ) ;
#3917=CARTESIAN_POINT ( 'NONE',  ( -166.3175803736862406, 79.86140754556168986, -12.19923997767886981 ) ) ;
#3918=CARTESIAN_POINT ( 'NONE',  ( -31.43908319763710679, 9.591432048623758533, 45.21645440618919309 ) ) ;
#3919=CARTESIAN_POINT ( 'NONE',  ( 11.47034038687561441, 6.400817013728348215, 85.06273559740630219 ) ) ;
#3922=CARTESIAN_POINT ( 'NONE',  ( 22.25657943806483274, 7.801867731668604478, 94.99999999999866418 ) ) ;
#3926=CARTESIAN_POINT ( 'NONE',  ( -95.05546640093037070, 29.25972325950976582, 62.78387324367114530 ) ) ;
#3928=DIRECTION ( 'NONE',  ( 0.000000000000000000, 0.000000000000000000, 1.000000000000000000 ) ) ;
#3931=CARTESIAN_POINT ( 'NONE',  ( -60.98168946575806615, 17.40090852531920618, -11.25214144170228714 ) ) ;
#3935=CARTESIAN_POINT ( 'NONE',  ( 8.848532525911927848, 6.377649276597439965, -40.14341413102923894 ) ) ;
#3937=CARTESIAN_POINT ( 'NONE',  ( 18.19980344696536534, 6.589834367837005935, 3.564186700565433519 ) ) ;
#3939=VECTOR ( 'NONE', #54041, 1000.000000000000000 ) ;
#3942=CARTESIAN_POINT ( 'NONE',  ( -35.68454966275956508, 10.32676244612189187, 85.21450729991012452 ) ) ;
#3946=CARTESIAN_POINT ( 'NONE',  ( 106.0171289417044136, 26.97542621030655141, -37.22168915489021401 ) ) ;
#3948=CARTESIAN_POINT ( 'NONE',  ( -173.1211646369891355, 88.63826465341151106, -88.40105834567734178 ) ) ;
#3949=EDGE_LOOP ( 'NONE', ( #17413, #41981, #67353, #11189 ) ) ;
#3952=CARTESIAN_POINT ( 'NONE',  ( -80.56139928459657540, 24.13290941644247667, -62.19941343312095228 ) ) ;
#3957=CARTESIAN_POINT ( 'NONE',  ( -152.5046761101291679, 66.76407727525179325, 18.25504938878692940 ) ) ;
#3958=CARTESIAN_POINT ( 'NONE',  ( -118.4470345550925998, 42.96051736048243441, -70.30058100330663251 ) ) ;
#3961=DIRECTION ( 'NONE',  ( -0.000000000000000000, 1.000000000000000000, -0.000000000000000000 ) ) ;
#3962=CARTESIAN_POINT ( 'NONE',  ( -104.5827168854524416, 33.96561401163047123, 30.86578353306401112 ) ) ;
#3965=CARTESIAN_POINT ( 'NONE',  ( -62.55024818870805348, 17.87229771727388794, 91.88754048207763958 ) ) ;
#3966=EDGE_LOOP ( 'NONE', ( #4112, #51745 ) ) ;
#3967=CARTESIAN_POINT ( 'NONE',  ( 198.8687991397276562, 98.67887821384415759, -21.70767789263648950 ) ) ;
#3969=CARTESIAN_POINT ( 'NONE',  ( -145.3246383987844865, 62.00818849034185121, 5.146554988373365447 ) ) ;
#3973=CARTESIAN_POINT ( 'NONE',  ( 139.7883986595927865, 46.32091287009615144, -48.11977978458424587 ) ) ;
#3975=CARTESIAN_POINT ( 'NONE',  ( 198.0640335990182450, 97.66860687174101940, 93.90131546401161700 ) ) ;
#3976=CARTESIAN_POINT ( 'NONE',  ( 8.478575283864733692, 7.382882227715644063, -41.32250106610652551 ) ) ;
#3978=CARTESIAN_POINT ( 'NONE',  ( 129.6961120139404215, 38.96846414226720157, -49.76800638012151268 ) ) ;
#3980=ORIENTED_EDGE ( 'NONE', *, *, #34314, .F. ) ;
#3982=CARTESIAN_POINT ( 'NONE',  ( 178.4097654444205432, 77.35573068857576118, 83.48439424739329695 ) ) ;
#3984=CARTESIAN_POINT ( 'NONE',  ( -29.51060362117876679, 9.282716514427262311, -76.91369189782112414 ) ) ;
#3988=CARTESIAN_POINT ( 'NONE',  ( 13.84937401517046851, 6.446378549072246500, 17.91938108381891936 ) ) ;
#3993=CARTESIAN_POINT ( 'NONE',  ( 174.6127059037622189, 72.30368563770913681, -74.39996846163762712 ) ) ;
#3995=CARTESIAN_POINT ( 'NONE',  ( 88.52345267551656605, 20.07594890262054577, -23.73786243512815020 ) ) ;
#3996=CARTESIAN_POINT ( 'NONE',  ( -25.07901552294941894, 9.649193085547803861, 68.54352610857644379 ) ) ;
#4003=DIRECTION ( 'NONE',  ( -0.000000000000000000, 1.000000000000000000, -0.000000000000000000 ) ) ;
#4005=CARTESIAN_POINT ( 'NONE',  ( -55.05276343752909440, 14.68156374112638041, -35.21632399845986328 ) ) ;
#4009=ADVANCED_FACE ( 'NONE', ( #3640 ), #46547, .F. ) ;
#4010=CARTESIAN_POINT ( 'NONE',  ( -78.66644367742111399, 22.32174330031316956, 45.41820113967312977 ) ) ;
#4011=CARTESIAN_POINT ( 'NONE',  ( -58.33245019990696534, 15.58496056636070470, 71.42426283422710753 ) ) ;
#4014=CARTESIAN_POINT ( 'NONE',  ( -149.5074843970971301, 64.17983161892345834, 30.72082123989904900 ) ) ;
#4016=CARTESIAN_POINT ( 'NONE',  ( 133.8566784816069060, 42.60093787723656789, -89.71241211332301191 ) ) ;
#4017=VERTEX_POINT ( 'NONE', #31083 ) ;
#4020=CARTESIAN_POINT ( 'NONE',  ( 56.29445224195347919, 12.24017809212662655, -46.58514210915670617 ) ) ;
#4021=CARTESIAN_POINT ( 'NONE',  ( -85.90077524418997257, 26.30132018890136081, 39.91278707234438627 ) ) ;
#4022=CARTESIAN_POINT ( 'NONE',  ( -24.95029760921699591, 9.631514785009935409, -19.74184417840635675 ) ) ;
#4024=PRODUCT ( 'SIEVE', 'SIEVE', '', ( #61095 ) ) ;
#4025=ORIENTED_EDGE ( 'NONE', *, *, #11025, .T. ) ;
#4027=CARTESIAN_POINT ( 'NONE',  ( 10.13846145460683168, 6.385368868491635652, 69.31597689299731258 ) ) ;
#4028=DIRECTION ( 'NONE',  ( -0.000000000000000000, 1.000000000000000000, -0.000000000000000000 ) ) ;
#4034=CARTESIAN_POINT ( 'NONE',  ( 70.41705859591010608, 15.55317472777718280, 36.07559689591754903 ) ) ;
#4038=B_SPLINE_CURVE_WITH_KNOTS ( 'NONE', 3,
 ( #60997, #18435, #34966, #13845, #45157, #66304, #56409, #29006, #44470, #30032, #2606, #51143, #34634, #40240, #2959, #62029, #13166, #17749, #35307, #24065, #13510, #8231, #40575, #12462, #50448, #12822, #66993, #24418, #2268, #39890, #34276, #56765, #23715, #56071, #8585, #33926, #18781, #7888, #45509, #29334, #1556, #50785, #23018, #1926 ),
 .UNSPECIFIED., .F., .F.,
 ( 4, 2, 2, 2, 2, 2, 2, 2, 2, 2, 2, 2, 1, 2, 2, 2, 2, 2, 2, 1, 2, 2, 4 ),
 ( 0.02381751147647563280, 0.02531129726520771686, 0.02605819015957376236, 0.02680508305393981133, 0.02829886884267190580, 0.02979265463140400028, 0.03053954752577002496, 0.03128644042013604964, 0.03278022620886809901, 0.03427401199760014838, 0.03576779778633219775, 0.03651469068069820856, 0.03726158357506421243, 0.03800847646943021629, 0.03875536936379622016, 0.04024915515252823484, 0.04174294094126024257, 0.04323672672999225031, 0.04398361962435824724, 0.04473051251872425804, 0.04547740541309026191, 0.04622429830745626578, 0.04771808409618829433 ),
 .UNSPECIFIED. ) ;
#4044=CARTESIAN_POINT ( 'NONE',  ( -102.2801239173131194, -170.0000000000000000, 38.01907450641511588 ) ) ;
#4046=CARTESIAN_POINT ( 'NONE',  ( -118.3960663196801306, 41.75130200162922023, 64.39655094048056583 ) ) ;
#4056=ADVANCED_FACE ( 'NONE', ( #5018 ), #84, .F. ) ;
#4057=CARTESIAN_POINT ( 'NONE',  ( -86.06525741550314024, 26.37048289224654951, -41.36178332953014092 ) ) ;
#4058=CARTESIAN_POINT ( 'NONE',  ( 157.9160637431159273, 57.99786926216935967, 71.25401806271709404 ) ) ;
#4059=CARTESIAN_POINT ( 'NONE',  ( -149.5074843970971017, 65.50121172469319220, 3.876270649435370252 ) ) ;
#4060=CARTESIAN_POINT ( 'NONE',  ( 181.0840389613909736, 78.60582251573003987, -36.22505766587961062 ) ) ;
#4061=CARTESIAN_POINT ( 'NONE',  ( -166.2425995121691642, 79.78465616981384301, 94.99999999999866418 ) ) ;
#4062=CARTESIAN_POINT ( 'NONE',  ( 161.7209903610255139, 61.03262545641849357, -64.27214371681093041 ) ) ;
#4068=ADVANCED_FACE ( 'NONE', ( #32106 ), #32794, .F. ) ;
#4069=CARTESIAN_POINT ( 'NONE',  ( 70.11766033381771024, 14.43277633974326513, -45.68147077570210257 ) ) ;
#4073=CARTESIAN_POINT ( 'NONE',  ( -38.17232309348610642, 11.81874355808868771, -66.32131283007623779 ) ) ;
#4075=CARTESIAN_POINT ( 'NONE',  ( 31.90217595456442012, 7.552213897210512172, 64.75245333076260579 ) ) ;
#4076=CARTESIAN_POINT ( 'NONE',  ( 11.21387192505586761, 6.397095920409659797, -22.13791506854233049 ) ) ;
#4079=CARTESIAN_POINT ( 'NONE',  ( 188.4904153916304210, 86.42965364612516055, 62.43372719721995168 ) ) ;
#4080=CARTESIAN_POINT ( 'NONE',  ( -119.2682179969168601, 42.28333404791699479, 14.82846940081925347 ) ) ;
#4081=CARTESIAN_POINT ( 'NONE',  ( 70.02892116572941461, 14.40944430928135489, -67.39582635729337312 ) ) ;
#4082=CARTESIAN_POINT ( 'NONE',  ( 126.3737790127712515, 37.08609730334947585, -16.10780632754811847 ) ) ;
#4084=CARTESIAN_POINT ( 'NONE',  ( 8.537735592981558597, 7.383000420390738228, 12.60408504631577742 ) ) ;
#4087=CARTESIAN_POINT ( 'NONE',  ( 187.5325688887158151, 85.37769363979911930, 13.83221296240295572 ) ) ;
#4093=CARTESIAN_POINT ( 'NONE',  ( 185.5457097283155008, 84.70846743303874860, -37.67841935146066135 ) ) ;
#4094=ORIENTED_EDGE ( 'NONE', *, *, #39694, .T. ) ;
#4099=CARTESIAN_POINT ( 'NONE',  ( -147.3614567344829140, 62.37986555269943523, -8.268114818102619168 ) ) ;
#4102=CARTESIAN_POINT ( 'NONE',  ( 112.5721302457195634, 29.97407549554798933, 71.10054341115458953 ) ) ;
#4104=CARTESIAN_POINT ( 'NONE',  ( 131.3924949472283004, 41.12442122814100287, -77.45525042326674736 ) ) ;
#4110=ORIENTED_EDGE ( 'NONE', *, *, #50020, .T. ) ;
#4112=ORIENTED_EDGE ( 'NONE', *, *, #10677, .F. ) ;
#4114=CARTESIAN_POINT ( 'NONE',  ( -122.8118341587044711, 44.49743491855734590, -22.42191975060944031 ) ) ;
#4116=CARTESIAN_POINT ( 'NONE',  ( -179.2177980985565000, 94.18084789436638005, -19.74344003203561471 ) ) ;
#4117=CARTESIAN_POINT ( 'NONE',  ( -132.4896623150433754, 52.22616402022728010, 68.54373966055456435 ) ) ;
#4120=CARTESIAN_POINT ( 'NONE',  ( 86.62931800182293784, -170.0000000000000000, 64.05663816294301682 ) ) ;
#4122=CARTESIAN_POINT ( 'NONE',  ( -57.43251939610647128, 15.33203492375494648, -23.00071778682259094 ) ) ;
#4124=VECTOR ( 'NONE', #23446, 1000.000000000000000 ) ;
#4125=CARTESIAN_POINT ( 'NONE',  ( -130.5904357464317798, 50.88938808445630713, -63.39065355895628784 ) ) ;
#4126=CARTESIAN_POINT ( 'NONE',  ( 58.79612034558317646, 11.73326361111144145, -90.69579281747449784 ) ) ;
#4133=CARTESIAN_POINT ( 'NONE',  ( 181.0840389613909736, -170.0000000000000000, 63.65314469597510794 ) ) ;
#4134=CARTESIAN_POINT ( 'NONE',  ( -165.7138623879809529, 79.24467249981145756, -40.99702868041568138 ) ) ;
#4138=CARTESIAN_POINT ( 'NONE',  ( -72.35078170365750339, 21.08176362823952488, 33.86556106749917205 ) ) ;
#4141=CARTESIAN_POINT ( 'NONE',  ( 63.98689050258322908, 13.93365232918667473, -35.76819633441670732 ) ) ;
#4142=CARTESIAN_POINT ( 'NONE',  ( -173.1211646369891355, 88.63826465341152527, -34.71195716474998960 ) ) ;
#4143=CARTESIAN_POINT ( 'NONE',  ( 211.7419975634644516, 116.5322580952101248, 60.89782388646611366 ) ) ;
#4145=CARTESIAN_POINT ( 'NONE',  ( -108.0980548770427845, 35.83569586822709141, -10.91122087686984976 ) ) ;
#4146=B_SPLINE_CURVE_WITH_KNOTS ( 'NONE', 3,
 ( #52912, #4735, #22303, #45144, #60979, #54290, #33573, #6817, #66623, #28267, #59921, #17364, #18419, #59569, #34261, #17735, #11739, #28988, #23703, #60289, #33218, #22650, #44089, #43740, #65218, #32855, #55706, #38480, #54652, #23367, #7535, #6477, #50434, #12805, #2255, #60634, #12450, #65573, #11385, #28629, #6112, #38842, #33909, #23003, #17009, #49013, #7174, #39529 ),
 .UNSPECIFIED., .F., .F.,
 ( 4, 2, 2, 2, 2, 2, 2, 2, 2, 2, 2, 2, 2, 2, 2, 2, 2, 2, 2, 2, 2, 2, 2, 4 ),
 ( 7.757919228897728493E-18, 0.001591515129442220991, 0.003183030258884434176, 0.003978787823605536324, 0.004774545388326638037, 0.006366060517768890037, 0.007957575647211142036, 0.009549090776653395771, 0.01034484834137452437, 0.01114060590609565297, 0.01193636347081678331, 0.01273212103553791712, 0.01432363616498018473, 0.01591515129442245061, 0.01671090885914358615, 0.01750666642386471822, 0.01830242398858585723, 0.01909818155330698930, 0.02068969668274931242, 0.02148545424747046878, 0.02228121181219162514, 0.02387272694163386499, 0.02466848450635494502, 0.02546424207107601811 ),
 .UNSPECIFIED. ) ;
#4148=CARTESIAN_POINT ( 'NONE',  ( -179.2175250771078936, 94.18012766206246056, -91.50370824807137637 ) ) ;
#4150=CARTESIAN_POINT ( 'NONE',  ( 82.73618382051374454, 19.18661415186669572, 70.47170656936988564 ) ) ;
#4154=CARTESIAN_POINT ( 'NONE',  ( 33.46033188299906413, 8.722678254080099336, 5.985838565680452916 ) ) ;
#4157=FACE_OUTER_BOUND ( 'NONE', #4605, .T. ) ;
#4163=CARTESIAN_POINT ( 'NONE',  ( -190.6985136298601731, 109.1272424661242582, -95.00000000000133582 ) ) ;
#4165=CARTESIAN_POINT ( 'NONE',  ( -58.91195363087619086, 15.75019387706849727, -89.97097185737439418 ) ) ;
#4167=CARTESIAN_POINT ( 'NONE',  ( 152.6804161981489472, 55.27286404993342472, -49.40040420956763256 ) ) ;
#4170=CARTESIAN_POINT ( 'NONE',  ( -157.0069571479806996, 72.18154199622281908, 64.76481382543292398 ) ) ;
#4173=CARTESIAN_POINT ( 'NONE',  ( -7.825402957745081878, 7.899365992529270741, 30.11558103944718923 ) ) ;
#4174=ORIENTED_EDGE ( 'NONE', *, *, #26295, .F. ) ;
#4175=CARTESIAN_POINT ( 'NONE',  ( -175.1968289912784940, 90.99944698359489337, -61.83708215555294885 ) ) ;
#4176=CARTESIAN_POINT ( 'NONE',  ( 93.85846834761625246, 22.01563781856520663, 62.04340769976120384 ) ) ;
#4179=CARTESIAN_POINT ( 'NONE',  ( 202.7540649946182896, 105.3989460363904698, -24.23651903053695378 ) ) ;
#4183=CARTESIAN_POINT ( 'NONE',  ( 201.5903370237273862, 102.1785392640257584, 29.86822796726585594 ) ) ;
#4186=CARTESIAN_POINT ( 'NONE',  ( 182.7745872728868051, 81.77554423487158886, 44.16596963624431993 ) ) ;
#4187=CARTESIAN_POINT ( 'NONE',  ( 141.3036441389950824, 47.31002705502925920, 9.125830029735173099 ) ) ;
#4193=CARTESIAN_POINT ( 'NONE',  ( 133.8566784816069344, -170.0000000000000000, 10.16579024853168889 ) ) ;
#4196=VECTOR ( 'NONE', #55684, 1000.000000000000000 ) ;
#4197=CARTESIAN_POINT ( 'NONE',  ( -109.7078892845591582, 36.71702188566216307, -41.44327227783652745 ) ) ;
#4198=CARTESIAN_POINT ( 'NONE',  ( 126.5497923654802008, 37.18409895203431148, 92.42836552067784339 ) ) ;
#4199=CARTESIAN_POINT ( 'NONE',  ( -56.96214175905167565, 15.20165595797839586, 45.07424718572830358 ) ) ;
#4202=CARTESIAN_POINT ( 'NONE',  ( -179.2177980985565284, 94.18084789436638005, 33.94566114889175878 ) ) ;
#4204=CARTESIAN_POINT ( 'NONE',  ( 110.7167338301704120, 30.21148223254619225, -35.92243756565369495 ) ) ;
#4207=ADVANCED_FACE ( 'NONE', ( #5370, #26826, #10984, #27860, #50009, #49651, #18013, #44746, #16949, #38776, #49303, #66225, #28564, #18352, #1844, #59858, #55996, #44382, #6755, #65506, #1136, #54934, #1479, #65871, #22940, #39814, #65155, #22587, #29261, #60220, #17666, #33507, #34201, #55635, #23641, #23301, #39130, #38413, #39462, #7468, #12038, #787, #2189, #55285, #34556, #60569, #11678, #44027, #22240, #28921, #33149, #12385, #33844, #66563, #17304, #28205, #7105, #61268, #60913, #45080, #12736, #50373, #13091, #7810, #43679, #54585, #6411, #24685, #61948, #3912, #14467, #19737, #23981, #2872, #46119, #41199, #24341, #35924, #25381, #34892, #67590, #8500, #51062, #14800, #13767, #8852, #45784, #50710, #51751, #30644, #62304, #40161, #9534, #3226, #51417, #67259, #40847, #52092, #19389, #35225, #14116, #35578, #9187 ), #57375, .T. ) ;
#4211=CARTESIAN_POINT ( 'NONE',  ( 140.0614732283738704, 45.29930344725075742, 59.63437826547444587 ) ) ;
#4212=CARTESIAN_POINT ( 'NONE',  ( -169.8842709557924877, 83.59602878049474839, 31.54149301594271648 ) ) ;
#4216=CARTESIAN_POINT ( 'NONE',  ( 157.4703587214989398, -170.0000000000000000, 17.56491688178971700 ) ) ;
#4217=VERTEX_POINT ( 'NONE', #19045 ) ;
#4218=EDGE_CURVE ( 'NONE', #2906, #61020, #61068, .T. ) ;
#4219=CARTESIAN_POINT ( 'NONE',  ( 150.2193536046551685, 53.46717047532148825, -18.71536020992064309 ) ) ;
#4220=CARTESIAN_POINT ( 'NONE',  ( 208.0306608271317259, 112.7988899307264887, -23.70348385667363189 ) ) ;
#4221=CARTESIAN_POINT ( 'NONE',  ( 107.0555969502564722, 28.53646637607231895, 30.30581710560821662 ) ) ;
#4225=CARTESIAN_POINT ( 'NONE',  ( 183.9887307715836471, 83.05100282186906213, 16.88219682803630306 ) ) ;
#4230=CARTESIAN_POINT ( 'NONE',  ( 110.2429982417149574, -170.0000000000000000, -70.26698815611737814 ) ) ;
#4232=CARTESIAN_POINT ( 'NONE',  ( -75.65611349188969825, 22.26947559308020530, 57.88921423585124160 ) ) ;
#4234=CARTESIAN_POINT ( 'NONE',  ( 62.04326772936977363, 12.44884401098615534, -77.51769772343732257 ) ) ;
#4238=CARTESIAN_POINT ( 'NONE',  ( -9.133021071383323530, 6.979519547623484144, 83.91237909771824377 ) ) ;
#4246=CARTESIAN_POINT ( 'NONE',  ( 204.0464538518397148, 105.4549945320416953, -90.03620575426465678 ) ) ;
#4248=B_SPLINE_CURVE_WITH_KNOTS ( 'NONE', 3,
 ( #45934, #62104, #9336, #13579, #68096, #51219, #67399, #4407, #41007, #62461, #3708, #3034, #68758, #30114, #25186, #56483, #20234, #35385 ),
 .UNSPECIFIED., .F., .F.,
 ( 4, 2, 2, 2, 2, 2, 2, 2, 4 ),
 ( 0.01201226291592704873, 0.01492726547989151054, 0.01638476676187372236, 0.01784226804385593418, 0.01929976932583814253, 0.02075727060782035782, 0.02148602124881145159, 0.02221477188980254883, 0.02367227317178470167 ),
 .UNSPECIFIED. ) ;
#4249=ORIENTED_EDGE ( 'NONE', *, *, #48713, .T. ) ;
#4250=CARTESIAN_POINT ( 'NONE',  ( -150.3791492925491298, 64.92185203933372861, 30.75880558023102296 ) ) ;
#4251=CARTESIAN_POINT ( 'NONE',  ( 60.40277045393652600, 12.08176563382370183, -36.18631425159986037 ) ) ;
#4252=CYLINDRICAL_SURFACE ( 'NONE', #48497, 7.500000000000013323 ) ;
#4256=CARTESIAN_POINT ( 'NONE',  ( -132.2161740628506550, 52.03204870034952734, 34.07724243096232186 ) ) ;
#4258=CARTESIAN_POINT ( 'NONE',  ( 22.62427395637551086, 7.823784829753562597, -46.11402725324526131 ) ) ;
#4259=CARTESIAN_POINT ( 'NONE',  ( -145.9181947914995874, 62.49417193455359154, 44.81018965788452846 ) ) ;
#4260=B_SPLINE_CURVE_WITH_KNOTS ( 'NONE', 3,
 ( #27856, #37359, #43675, #5014, #16945, #33145, #53185, #11674, #54581, #79, #47916, #59162, #6406, #32101, #49299, #1132, #58818, #44023, #22583, #58471, #69380, #10283, #54930, #23977, #2870, #44378, #33502, #2186, #7101, #17300, #44743, #13088, #1475, #45429, #66909, #2524, #8146, #39811, #28918, #18704, #7465, #34890, #29258, #50006, #49647, #56330, #60910 ),
 .UNSPECIFIED., .F., .F.,
 ( 4, 2, 2, 2, 2, 2, 2, 2, 2, 2, 2, 2, 1, 2, 2, 2, 2, 2, 2, 2, 2, 2, 2, 4 ),
 ( 0.000000000000000000, 0.001520400357568930287, 0.002280600536353414188, 0.003040800715137898305, 0.004561201072706868274, 0.005321401251491338080, 0.006081601430275807886, 0.007602001787844721477, 0.008362201966629193017, 0.009122402145413663690, 0.01064280250298261024, 0.01140300268176708612, 0.01216320286055155853, 0.01292340303933604308, 0.01368360321812052589, 0.01520400357568950193, 0.01596420375447399342, 0.01672440393325848665, 0.01824480429082747657, 0.01976520464839646649, 0.02052540482718095971, 0.02128560500596544947, 0.02280600536353444285, 0.02432640572110343624 ),
 .UNSPECIFIED. ) ;
#4263=ORIENTED_EDGE ( 'NONE', *, *, #2659, .T. ) ;
#4265=CARTESIAN_POINT ( 'NONE',  ( -127.3773789194800372, 48.68981405637768489, 84.45179168653085355 ) ) ;
#4266=CARTESIAN_POINT ( 'NONE',  ( -167.6413528428656150, 81.22881971256914824, -20.51375374840328547 ) ) ;
#4268=CARTESIAN_POINT ( 'NONE',  ( 14.47678578469710864, 6.462159579077012772, 83.81204869879134378 ) ) ;
#4269=CARTESIAN_POINT ( 'NONE',  ( 80.16939877002758408, 17.31693935407226448, -66.32369062857475228 ) ) ;
#4275=B_SPLINE_CURVE_WITH_KNOTS ( 'NONE', 3,
 ( #2929, #35972, #39863, #35636, #67310, #3276, #56739, #62359, #56045, #13482, #67994, #50761, #61320, #19096, #46519, #40550, #13146, #24041, #57087, #13818, #35283, #34943, #30351, #41257, #45134, #2582, #34609, #30008, #18760, #61663, #24736, #46171, #7863, #51804, #56383, #3612, #29310, #7526, #25082, #2242, #19440, #28976, #66963, #50423, #23691 ),
 .UNSPECIFIED., .F., .F.,
 ( 4, 2, 2, 1, 2, 2, 2, 2, 2, 2, 2, 2, 2, 2, 2, 2, 2, 2, 2, 2, 2, 2, 4 ),
 ( 0.02346057189573569693, 0.02492590417315493703, 0.02565857031186456055, 0.02639123645057418407, 0.02712390258928380760, 0.02785656872799342765, 0.02932190100541267816, 0.03005456714412230862, 0.03078723328283193561, 0.03225256556025118959, 0.03298523169896081658, 0.03371789783767044357, 0.03518323011508970449, 0.03664856239250896541, 0.03738122853121858546, 0.03811389466992821246, 0.03957922694734747338, 0.04104455922476672736, 0.04250989150218598134, 0.04324255764089560833, 0.04397522377960523532, 0.04544055605702450318, 0.04690588833444375716 ),
 .UNSPECIFIED. ) ;
#4277=CARTESIAN_POINT ( 'NONE',  ( -85.35127931077727226, 24.98147633332999717, 7.663918504084784367 ) ) ;
#4280=CARTESIAN_POINT ( 'NONE',  ( -60.66101049381765620, 17.30588917955502382, -10.86812352032706741 ) ) ;
#4284=CARTESIAN_POINT ( 'NONE',  ( -120.1650841064593891, 44.02024060322521848, 16.12247377298220030 ) ) ;
#4285=CARTESIAN_POINT ( 'NONE',  ( -180.6009936245623635, 95.85948119829087943, 65.79761809826371177 ) ) ;
#4287=CARTESIAN_POINT ( 'NONE',  ( 133.3990214534116774, 41.14886683286415092, 56.36538236340677344 ) ) ;
#4288=ORIENTED_EDGE ( 'NONE', *, *, #58975, .F. ) ;
#4291=ADVANCED_FACE ( 'NONE', ( #53795 ), #52766, .F. ) ;
#4292=CARTESIAN_POINT ( 'NONE',  ( -38.73622948742834637, 10.90353827065863968, 89.64304421912086696 ) ) ;
#4294=CARTESIAN_POINT ( 'NONE',  ( 173.8623159076320235, 72.97967239795021044, -72.61419801311336641 ) ) ;
#4298=CARTESIAN_POINT ( 'NONE',  ( -28.81317668042940028, 9.175023678939295380, 30.68696444450949201 ) ) ;
#4300=ORIENTED_EDGE ( 'NONE', *, *, #23587, .F. ) ;
#4302=CARTESIAN_POINT ( 'NONE',  ( -85.95621526752228192, 26.32462117888283260, -71.24159791805112718 ) ) ;
#4303=CARTESIAN_POINT ( 'NONE',  ( -1.901316136557078540, 6.577199328112531163, -91.92888192959523508 ) ) ;
#4305=CARTESIAN_POINT ( 'NONE',  ( -190.6985136298601731, 109.1272424661242582, -19.71767969763411799 ) ) ;
#4306=CARTESIAN_POINT ( 'NONE',  ( 129.4987365823222092, 38.85470922756778833, 4.057026465556845984 ) ) ;
#4307=CARTESIAN_POINT ( 'NONE',  ( 32.60744088438708133, 7.622802803743367051, -93.62651044593049221 ) ) ;
#4308=CARTESIAN_POINT ( 'NONE',  ( -123.0348077379026535, 45.83489305753316501, -62.32075488609377345 ) ) ;
#4310=CARTESIAN_POINT ( 'NONE',  ( 162.6190874793280727, 61.76782592053314147, 4.606215609171663949 ) ) ;
#4311=CARTESIAN_POINT ( 'NONE',  ( -108.9136445001389859, 36.28030794288191174, 41.52760062685047870 ) ) ;
#4313=CARTESIAN_POINT ( 'NONE',  ( -62.43646393413946782, 17.83771684480761976, 92.86132313336962341 ) ) ;
#4317=CARTESIAN_POINT ( 'NONE',  ( 22.62427395637552507, 7.823784829753567927, -72.95857784370898003 ) ) ;
#4318=DIRECTION ( 'NONE',  ( -0.8160245890732938934, -0.5780171883497599028, 0.000000000000000000 ) ) ;
#4324=CARTESIAN_POINT ( 'NONE',  ( 31.90217595456442012, 7.552213897210508620, -42.62574903109214830 ) ) ;
#4329=ORIENTED_EDGE ( 'NONE', *, *, #68056, .F. ) ;
#4332=CARTESIAN_POINT ( 'NONE',  ( 173.9006248317893437, 73.01561032181524524, 92.66295374434788812 ) ) ;
#4335=CIRCLE ( 'NONE', #22295, 243.4957430088094839 ) ;
#4336=B_SPLINE_CURVE_WITH_KNOTS ( 'NONE', 3,
 ( #53270, #159, #31494, #52594, #14960, #64183, #68437, #42727, #53620, #20581, #30809, #68766, #63852, #63166, #52256, #20243, #37109, #58899, #48325, #10714, #25543, #21617, #52926, #4415, #36425, #15995, #43063, #25879, #58222, #64534, #41703, #32188, #4752, #37444, #26215, #26899, #36086, #47654, #42043, #47996, #46978, #57542, #9345 ),
 .UNSPECIFIED., .F., .F.,
 ( 4, 2, 2, 2, 2, 2, 2, 2, 1, 2, 2, 2, 2, 2, 2, 2, 2, 2, 2, 2, 2, 4 ),
 ( 3.469446951953614189E-18, 0.001466285743483479757, 0.002199428615225219093, 0.002932571486966958647, 0.004398857230450446860, 0.005865142973933935508, 0.007331428717417423288, 0.008064571589159165443, 0.008797714460900907599, 0.009530857332642649754, 0.01026400020438439191, 0.01173028594786787449, 0.01319657169135135533, 0.01466285743483483790, 0.01539600030657657832, 0.01612914317831831701, 0.01759542892180180479, 0.01906171466528529257, 0.01979485753702703299, 0.02052800040876876994, 0.02199428615225223690, 0.02346057189573570387 ),
 .UNSPECIFIED. ) ;
#4338=CARTESIAN_POINT ( 'NONE',  ( 67.88711180968651604, 14.89360689134522353, -91.19259204464900392 ) ) ;
#4342=CARTESIAN_POINT ( 'NONE',  ( 210.9608386442062340, 117.1762372255315938, 13.99730087153263369 ) ) ;
#4343=CARTESIAN_POINT ( 'NONE',  ( -78.66644367742109978, 23.39876645725288284, -76.96000122218160300 ) ) ;
#4344=CARTESIAN_POINT ( 'NONE',  ( 93.08533330311587406, 21.72562315962718671, -20.32652723706974029 ) ) ;
#4345=CARTESIAN_POINT ( 'NONE',  ( -31.43908319763709969, 10.61114334766715928, 72.06100499665289760 ) ) ;
#4351=CARTESIAN_POINT ( 'NONE',  ( -53.38065169970958834, 15.27943072477081365, 71.97705297215981091 ) ) ;
#4353=CARTESIAN_POINT ( 'NONE',  ( -51.99406906667275052, 13.88268392809766283, -35.86411590326191856 ) ) ;
#4356=DIRECTION ( 'NONE',  ( -0.000000000000000000, 1.000000000000000000, -0.000000000000000000 ) ) ;
#4359=ORIENTED_EDGE ( 'NONE', *, *, #48104, .F. ) ;
#4360=EDGE_CURVE ( 'NONE', #40284, #69371, #53442, .T. ) ;
#4361=CARTESIAN_POINT ( 'NONE',  ( 46.75120595639165089, 10.49875654307468231, 89.57072679854206854 ) ) ;
#4362=CARTESIAN_POINT ( 'NONE',  ( -178.5835577246388084, 93.42126246260832545, -74.20141784023681453 ) ) ;
#4363=CARTESIAN_POINT ( 'NONE',  ( 135.7265100247341536, 43.74748294124387371, -89.93937249815461143 ) ) ;
#4365=CARTESIAN_POINT ( 'NONE',  ( -173.1211646369891071, 87.12891641440859303, -7.867406574286297527 ) ) ;
#4367=CARTESIAN_POINT ( 'NONE',  ( -6.840165690716681013, 7.836465889224657921, 3.319927015524997138 ) ) ;
#4370=CARTESIAN_POINT ( 'NONE',  ( 93.71772995179811971, 21.96265635001559247, 39.67534872124095813 ) ) ;
#4371=B_SPLINE_CURVE_WITH_KNOTS ( 'NONE', 3,
 ( #58627, #10443, #43831, #65311, #64262, #5855, #6209, #27662, #54385, #32943, #31917, #53345, #32264, #26296, #53696, #60016, #17098, #43490, #16759, #64966, #31565, #16070, #38220, #4825, #26971, #69528, #47726, #59661, #69188, #48401, #43142, #21016, #27311, #5176, #26638, #11475, #64611, #54029, #233, #42461, #63918, #21347, #21691, #16422, #42794 ),
 .UNSPECIFIED., .F., .F.,
 ( 4, 2, 2, 2, 2, 2, 2, 2, 2, 2, 2, 1, 2, 2, 2, 2, 2, 2, 2, 2, 2, 2, 4 ),
 ( 0.000000000000000000, 0.001510509505235922700, 0.002265764257853866703, 0.003021019010471810273, 0.004531528515707697845, 0.005286783268325657460, 0.006042038020943617076, 0.007552547526179537174, 0.009063057031415456405, 0.01057356653665137737, 0.01132882128926933699, 0.01208407604188729660, 0.01283933079450525622, 0.01359458554712321930, 0.01510509505235920619, 0.01586034980497719182, 0.01661560455759517399, 0.01812611406283112792, 0.01963662356806708184, 0.02039187832068503972, 0.02114713307330299760, 0.02265764257853894806, 0.02416815208377490198 ),
 .UNSPECIFIED. ) ;
#4373=VERTEX_POINT ( 'NONE', #7022 ) ;
#4374=CARTESIAN_POINT ( 'NONE',  ( 9.416656162223551618, 6.380306691996769253, 68.32325512165303394 ) ) ;
#4377=CARTESIAN_POINT ( 'NONE',  ( 197.3700262219430783, 98.41176242030789467, 38.33750891837946284 ) ) ;
#4379=EDGE_CURVE ( 'NONE', #12998, #41403, #48441, .T. ) ;
#4380=CARTESIAN_POINT ( 'NONE',  ( -76.28906486289076838, 22.50303357844624230, 84.48732397307654196 ) ) ;
#4387=CARTESIAN_POINT ( 'NONE',  ( 201.9777685760379882, 102.6876480786892927, -77.67199324841566010 ) ) ;
#4388=CARTESIAN_POINT ( 'NONE',  ( 204.6977192012829789, -170.0000000000000000, -51.32593103262161094 ) ) ;
#4389=CYLINDRICAL_SURFACE ( 'NONE', #65772, 7.500000000000013323 ) ;
#4390=CARTESIAN_POINT ( 'NONE',  ( -85.12122836439577611, 25.97531040437156591, -11.91969542759261280 ) ) ;
#4392=CARTESIAN_POINT ( 'NONE',  ( -151.6716822472524484, 66.03661194063731443, -49.50755342994084884 ) ) ;
#4394=ORIENTED_EDGE ( 'NONE', *, *, #65093, .T. ) ;
#4397=CARTESIAN_POINT ( 'NONE',  ( 117.0725462099858447, 32.17176564273682260, 87.68110821929519716 ) ) ;
#4398=CARTESIAN_POINT ( 'NONE',  ( 117.0069443446175512, 33.26475960880694771, -13.32765567664555029 ) ) ;
#4407=CARTESIAN_POINT ( 'NONE',  ( 176.7302122685738652, 74.31432059049257077, -91.29563362033026408 ) ) ;
#4409=CARTESIAN_POINT ( 'NONE',  ( -38.92718193365330848, 11.96647478777220286, -69.17238878754035625 ) ) ;
#4411=CARTESIAN_POINT ( 'NONE',  ( -153.1121305730337383, 67.29834700374526335, -8.887376870342574620 ) ) ;
#4413=CARTESIAN_POINT ( 'NONE',  ( 13.14401442664831343, 6.430459733718342008, -9.151694974088321999 ) ) ;
#4415=CARTESIAN_POINT ( 'NONE',  ( 23.23965501943000689, 7.861749956303025755, 9.686424920567322516 ) ) ;
#4417=CARTESIAN_POINT ( 'NONE',  ( -118.4622862908118606, 41.79153065058246597, 12.32190642974081030 ) ) ;
#4421=CARTESIAN_POINT ( 'NONE',  ( 9.050324533885207856, 7.384616180193985358, 7.339830793012372290 ) ) ;
#4426=CARTESIAN_POINT ( 'NONE',  ( 175.5493994043410737, 73.18740965572601453, 41.87606852396054080 ) ) ;
#4428=CARTESIAN_POINT ( 'NONE',  ( -102.2801239173131052, 33.91021738430207222, -50.01457726497594081 ) ) ;
#4430=CARTESIAN_POINT ( 'NONE',  ( 184.3966782763552317, 83.48172388049826509, -50.46844882507220831 ) ) ;
#4434=EDGE_CURVE ( 'NONE', #10004, #46743, #54311, .T. ) ;
#4436=EDGE_CURVE ( 'NONE', #67011, #61969, #24948, .T. ) ;
#4437=CARTESIAN_POINT ( 'NONE',  ( 198.4059165548112276, 99.71594270191990006, 13.95396656640263089 ) ) ;
#4441=ORIENTED_EDGE ( 'NONE', *, *, #62368, .F. ) ;
#4443=CARTESIAN_POINT ( 'NONE',  ( 133.6288034103010602, 41.28708886999552163, 29.51034083899532590 ) ) ;
#4452=ORIENTED_EDGE ( 'NONE', *, *, #34660, .T. ) ;
#4453=CARTESIAN_POINT ( 'NONE',  ( -118.7011677090247019, 41.93687969120205850, -17.71047622372893215 ) ) ;
#4459=B_SPLINE_CURVE_WITH_KNOTS ( 'NONE', 3,
 ( #49447, #67058, #44887, #17816, #18504, #2672, #44171, #39271, #49802, #29068, #60715, #60374, #1993, #1627, #24135, #12531, #66021, #45576, #65659, #50513, #66368, #17448, #33993, #54734, #23092, #18854, #33652, #61063, #40303, #28003, #38925, #12188, #39957, #50855, #55431, #1280, #7262, #12891, #55080, #22737, #6900, #50164, #61413 ),
 .UNSPECIFIED., .F., .F.,
 ( 4, 2, 2, 2, 2, 2, 2, 2, 2, 2, 2, 2, 1, 2, 2, 2, 2, 2, 2, 2, 2, 4 ),
 ( 0.02362927190606132002, 0.02510248541563188038, 0.02583909217041715708, 0.02657569892520243032, 0.02804891243477299068, 0.02952212594434355103, 0.03025873269912882774, 0.03099533945391410791, 0.03246855296348467868, 0.03394176647305525985, 0.03541497998262583408, 0.03615158673741113160, 0.03688819349219642912, 0.03762480024698172665, 0.03836140700176702417, 0.03983462051133762616, 0.04130783402090822121, 0.04278104753047881625, 0.04351765428526410684, 0.04425426104004940436, 0.04572747454961999247, 0.04720068805919058752 ),
 .UNSPECIFIED. ) ;
#4460=CARTESIAN_POINT ( 'NONE',  ( -147.7845268487069461, 62.73119438705056439, -35.00051754678168692 ) ) ;
#4466=CARTESIAN_POINT ( 'NONE',  ( -62.48965350618346548, 16.80247907725182799, -14.86921336900190482 ) ) ;
#4467=CARTESIAN_POINT ( 'NONE',  ( -127.4644500646575125, 48.74852676951795161, -76.59546237094302512 ) ) ;
#4468=CARTESIAN_POINT ( 'NONE',  ( 39.40195752203892710, 9.424259417798138472, -89.30891864635511013 ) ) ;
#4469=CARTESIAN_POINT ( 'NONE',  ( -101.3602137809054540, 32.31558061113913283, 3.716661569264940734 ) ) ;
#4470=CARTESIAN_POINT ( 'NONE',  ( -94.88380767928869375, 29.17964217339916999, -68.08975550236192475 ) ) ;
#4474=CARTESIAN_POINT ( 'NONE',  ( 187.9007786055418592, 85.78077355327280884, -67.43016102822709001 ) ) ;
#4475=CARTESIAN_POINT ( 'NONE',  ( -167.9853834315979384, 81.58767916550894483, -36.72585540580842434 ) ) ;
#4478=CARTESIAN_POINT ( 'NONE',  ( 103.0004140566503139, 26.76634862952791494, -68.25275454392931351 ) ) ;
#4479=CARTESIAN_POINT ( 'NONE',  ( -75.65611349188965562, 22.26947559308018043, 31.04466364538752288 ) ) ;
#4480=CARTESIAN_POINT ( 'NONE',  ( 86.62931800182293784, 19.42108912189597092, 29.71208757247930521 ) ) ;
#4482=DIRECTION ( 'NONE',  ( 0.000000000000000000, -1.000000000000000000, 0.000000000000000000 ) ) ;
#4483=CARTESIAN_POINT ( 'NONE',  ( -165.7138623879809529, 79.24467249981142913, -67.84157927087939299 ) ) ;
#4487=CARTESIAN_POINT ( 'NONE',  ( 85.83322572930757133, 20.21160859307071789, -89.51066537983908233 ) ) ;
#4490=CARTESIAN_POINT ( 'NONE',  ( 133.8566784816069060, 42.60093787723655367, 71.35489142945907304 ) ) ;
#4493=CARTESIAN_POINT ( 'NONE',  ( 33.44527180510250020, 7.709232309484699286, -74.54778285784610148 ) ) ;
#4496=CARTESIAN_POINT ( 'NONE',  ( -33.36965723649377935, 10.93726715887721568, -23.22402601025658697 ) ) ;
#4498=CARTESIAN_POINT ( 'NONE',  ( -123.6557841886868658, 46.23505328920332147, -88.94146719048309535 ) ) ;
#4499=EDGE_LOOP ( 'NONE', ( #31374, #26256 ) ) ;
#4502=CARTESIAN_POINT ( 'NONE',  ( -24.07146903340143496, 8.497560047608732958, 12.33779482100903735 ) ) ;
#4503=DIRECTION ( 'NONE',  ( -0.8118923937861950435, -0.5838071093367415143, 0.000000000000000000 ) ) ;
#4504=CARTESIAN_POINT ( 'NONE',  ( -15.31363169557738502, 7.494880774891999664, -70.25007158120349970 ) ) ;
#4505=CARTESIAN_POINT ( 'NONE',  ( -100.4262673593280368, 31.84860241619272969, -8.387597469391586458 ) ) ;
#4506=CARTESIAN_POINT ( 'NONE',  ( 151.7783534118502189, 54.60545177578660514, -38.73408018630978233 ) ) ;
#4511=CARTESIAN_POINT ( 'NONE',  ( 174.4912080999798718, 73.57140295268874297, -13.29444283027056883 ) ) ;
#4512=CARTESIAN_POINT ( 'NONE',  ( -109.3386876948163717, 37.66246927061208538, 62.27823371598848468 ) ) ;
#4516=CARTESIAN_POINT ( 'NONE',  ( -0.8011128725815461760, 6.535315321814184841, -13.43344384470691111 ) ) ;
#4517=CARTESIAN_POINT ( 'NONE',  ( 112.5554747942045850, 29.96654954475021171, 29.97270286920888438 ) ) ;
#4519=CARTESIAN_POINT ( 'NONE',  ( -157.0046402715469753, 70.80872207626528336, 91.63790604792896488 ) ) ;
#4521=CARTESIAN_POINT ( 'NONE',  ( 135.6842057900327347, 42.53841116629840968, 44.29889548343480499 ) ) ;
#4523=CARTESIAN_POINT ( 'NONE',  ( 199.3743599161302882, 99.31857334527873604, 42.01559847254342372 ) ) ;
#4525=CARTESIAN_POINT ( 'NONE',  ( 187.5165082312810512, 86.85340440641662951, 32.94302383692840408 ) ) ;
#4526=CARTESIAN_POINT ( 'NONE',  ( 155.7265855639938934, 57.57443315515126159, 29.60160751965668524 ) ) ;
#4531=CARTESIAN_POINT ( 'NONE',  ( 173.9457771591584390, 73.05793967547532475, 61.33444114611717879 ) ) ;
#4533=CARTESIAN_POINT ( 'NONE',  ( -109.5142642360664098, 36.61018064014776741, -44.56230308795456097 ) ) ;
#4535=ADVANCED_FACE ( 'NONE', ( #49836 ), #6595, .F. ) ;
#4536=CYLINDRICAL_SURFACE ( 'NONE', #13736, 7.500000000000020428 ) ;
#4538=VERTEX_POINT ( 'NONE', #28390 ) ;
#4539=CARTESIAN_POINT ( 'NONE',  ( -177.5259994307673423, 92.16784265327251546, 32.23362038954493158 ) ) ;
#4541=CARTESIAN_POINT ( 'NONE',  ( 15.78827728214693416, 6.500811158483284835, -23.67439350822212774 ) ) ;
#4546=CARTESIAN_POINT ( 'NONE',  ( 140.1999945597798956, 45.38880890490929687, 59.84517000566086153 ) ) ;
#4548=FACE_OUTER_BOUND ( 'NONE', #35942, .T. ) ;
#4551=CARTESIAN_POINT ( 'NONE',  ( 46.89016064832840414, 10.52130577388959409, 10.08109367583877969 ) ) ;
#4552=ORIENTED_EDGE ( 'NONE', *, *, #15580, .F. ) ;
#4554=CARTESIAN_POINT ( 'NONE',  ( 150.9013375937531123, 53.96275732797608526, -13.15108574339470060 ) ) ;
#4556=CARTESIAN_POINT ( 'NONE',  ( 102.7938674513918755, 26.67851209377774424, 38.12245759428292757 ) ) ;
#4557=B_SPLINE_CURVE_WITH_KNOTS ( 'NONE', 3,
 ( #1103, #38384, #53848, #64772, #69356, #59480, #54191, #37334, #27128, #17267, #32422, #42950, #16579, #64420, #48561, #16920, #65476, #6013, #38741, #32763, #27473, #12004, #48916, #11640, #38036, #22209, #54550, #43998, #43296, #21175, #60186, #754, #15889, #46, #11291, #5340, #47890, #53153, #37684, #49269, #16231, #43647, #5666, #42620, #65124 ),
 .UNSPECIFIED., .F., .F.,
 ( 4, 2, 2, 2, 2, 2, 2, 2, 2, 2, 2, 1, 2, 2, 2, 2, 2, 2, 2, 2, 2, 2, 4 ),
 ( 1.440969542111313559E-17, 0.001510509505235931157, 0.002265764257853871907, 0.003021019010471812441, 0.004531528515707694375, 0.005286783268325651389, 0.006042038020943608402, 0.007552547526179553654, 0.009063057031415498038, 0.01057356653665144156, 0.01132882128926941678, 0.01208407604188739722, 0.01283933079450537591, 0.01359458554712335808, 0.01510509505235932415, 0.01586034980497731325, 0.01661560455759529889, 0.01812611406283125629, 0.01963662356806721021, 0.02039187832068517156, 0.02114713307330312944, 0.02265764257853901745, 0.02416815208377490892 ),
 .UNSPECIFIED. ) ;
#4558=CARTESIAN_POINT ( 'NONE',  ( -150.3791492925491298, 64.92185203933370019, -76.61939678162372047 ) ) ;
#4560=CARTESIAN_POINT ( 'NONE',  ( 184.3966782763551464, 83.48172388049827930, 3.220652355855141202 ) ) ;
#4561=CARTESIAN_POINT ( 'NONE',  ( 209.4789161463551181, 113.1367444519303689, -49.60865656310190985 ) ) ;
#4566=CARTESIAN_POINT ( 'NONE',  ( -74.39861643904070831, 21.81123504700009264, 70.93476632660724590 ) ) ;
#4567=CARTESIAN_POINT ( 'NONE',  ( -94.79166046756729713, 29.13671350128076654, -42.02362451379906361 ) ) ;
#4568=CARTESIAN_POINT ( 'NONE',  ( 58.47673920847982743, 11.66523265296354772, -76.05570035470118739 ) ) ;
#4572=CARTESIAN_POINT ( 'NONE',  ( 164.8444104055694481, 64.93678790243656351, -71.86516271918338816 ) ) ;
#4576=CARTESIAN_POINT ( 'NONE',  ( 198.4942811600313064, 98.20737091473505131, -93.29402655745694517 ) ) ;
#4578=ORIENTED_EDGE ( 'NONE', *, *, #67425, .F. ) ;
#4579=CARTESIAN_POINT ( 'NONE',  ( -31.43908319763709969, 10.61114334766717171, -62.16174795566551836 ) ) ;
#4583=CARTESIAN_POINT ( 'NONE',  ( -142.2626321327577159, 58.26997216742665842, 9.417068183414567528 ) ) ;
#4585=ORIENTED_EDGE ( 'NONE', *, *, #35200, .F. ) ;
#4586=CARTESIAN_POINT ( 'NONE',  ( -132.9126122820979106, 52.52752252041127434, 35.46337234881715972 ) ) ;
#4588=CARTESIAN_POINT ( 'NONE',  ( 209.9944361927104808, 113.8994774711241291, 4.548133007360330993 ) ) ;
#4589=CARTESIAN_POINT ( 'NONE',  ( -143.8756912989386763, 60.83492035645721074, 43.18009283058132297 ) ) ;
#4591=CARTESIAN_POINT ( 'NONE',  ( 212.0180052085437694, 116.9552462415714871, 38.37144164438262095 ) ) ;
#4599=CARTESIAN_POINT ( 'NONE',  ( -165.9986675144416211, 79.53506019208356292, -13.00008028462095133 ) ) ;
#4600=DIRECTION ( 'NONE',  ( 0.000000000000000000, 0.000000000000000000, 1.000000000000000000 ) ) ;
#4602=CARTESIAN_POINT ( 'NONE',  ( 66.94779593213115731, 13.61918177102165650, 43.70422013568025221 ) ) ;
#4604=CARTESIAN_POINT ( 'NONE',  ( -190.0468231512975876, 108.2116162189844886, -72.35473219539915135 ) ) ;
#4605=EDGE_LOOP ( 'NONE', ( #59725, #21567, #9865, #35561 ) ) ;
#4607=CARTESIAN_POINT ( 'NONE',  ( -94.79534239005249674, 29.13842790650043924, 64.32042552946333558 ) ) ;
#4609=CARTESIAN_POINT ( 'NONE',  ( -80.55742067659895156, 23.05042616197510696, 3.800353480099713632 ) ) ;
#4610=EDGE_LOOP ( 'NONE', ( #55131, #56451, #22653, #24646 ) ) ;
#4614=CARTESIAN_POINT ( 'NONE',  ( -118.9668643994983341, 43.27909474462860828, 14.16267398761431195 ) ) ;
#4615=ADVANCED_FACE ( 'NONE', ( #20512 ), #30386, .F. ) ;
#4616=CARTESIAN_POINT ( 'NONE',  ( -176.3896317155479210, 90.84057090619016606, 58.40173573172133814 ) ) ;
#4618=CARTESIAN_POINT ( 'NONE',  ( 19.54475376904847650, 6.649964688461120765, 17.16624909598245097 ) ) ;
#4623=CARTESIAN_POINT ( 'NONE',  ( 107.0471828278920583, 27.43080724084234490, -36.62059212188487578 ) ) ;
#4624=CARTESIAN_POINT ( 'NONE',  ( -25.81763596640060854, 8.735969132042862739, 32.74552005507152330 ) ) ;
#4629=CARTESIAN_POINT ( 'NONE',  ( -81.24432217070636852, 24.40203426192926628, -62.41292138135722922 ) ) ;
#4630=AXIS2_PLACEMENT_3D ( 'NONE', #37735, #47583, #63792 ) ;
#4631=CARTESIAN_POINT ( 'NONE',  ( 173.8576514579035575, 72.97529922124009261, 11.99223922032557255 ) ) ;
#4634=CARTESIAN_POINT ( 'NONE',  ( 138.4794054115212703, 44.28634680695354575, -91.29333943486163605 ) ) ;
#4635=CARTESIAN_POINT ( 'NONE',  ( -156.4841188516942623, 70.33041971808550841, 8.609805402347420866 ) ) ;
#4636=CARTESIAN_POINT ( 'NONE',  ( 198.7765072002625288, 100.1872738704526427, 94.99999999999866418 ) ) ;
#4638=CARTESIAN_POINT ( 'NONE',  ( 64.93495251696904802, 13.12601614965099373, 3.214085396426615837 ) ) ;
#4640=CARTESIAN_POINT ( 'NONE',  ( -85.96384504792885650, 26.32782846176031200, 66.51262591793364720 ) ) ;
#4641=CARTESIAN_POINT ( 'NONE',  ( -109.6660553119435377, 36.69391917620600196, 39.34755413696105109 ) ) ;
#4644=CARTESIAN_POINT ( 'NONE',  ( -54.76617051175221462, 15.64622803826644670, 84.00532038758548481 ) ) ;
#4648=CARTESIAN_POINT ( 'NONE',  ( 22.89270809252619898, 7.840160460323052583, -67.44744513715251344 ) ) ;
#4651=CARTESIAN_POINT ( 'NONE',  ( 64.93495251696904802, 13.12601614965099373, -23.63046519403706469 ) ) ;
#4652=CARTESIAN_POINT ( 'NONE',  ( 136.9822423813093337, 44.53121110416872597, -50.34504590549451564 ) ) ;
#4653=CARTESIAN_POINT ( 'NONE',  ( 31.95008798096002423, 7.556925044648911793, -42.13730592359904392 ) ) ;
#4660=EDGE_CURVE ( 'NONE', #9825, #16384, #502, .T. ) ;
#4661=CARTESIAN_POINT ( 'NONE',  ( 176.5251334471615223, 75.51433118793448784, 84.53325931958181627 ) ) ;
#4662=CARTESIAN_POINT ( 'NONE',  ( -167.4860113959264538, 82.52233889531183308, -10.41155452729346820 ) ) ;
#4666=CARTESIAN_POINT ( 'NONE',  ( 175.8963338753314360, 73.51705463274394958, -65.14750092172043594 ) ) ;
#4667=CARTESIAN_POINT ( 'NONE',  ( -179.0654441437004891, 93.99779465816536117, -46.79209166540439924 ) ) ;
#4668=CARTESIAN_POINT ( 'NONE',  ( 90.31682503704263354, 20.71196693118261223, -9.927970538514026444 ) ) ;
#4669=DIRECTION ( 'NONE',  ( -0.000000000000000000, 1.000000000000000000, -0.000000000000000000 ) ) ;
#4672=CARTESIAN_POINT ( 'NONE',  ( 160.4986104110022893, 61.33701824525266488, 70.61926442309403740 ) ) ;
#4674=EDGE_CURVE ( 'NONE', #347, #60092, #5713, .T. ) ;
#4676=CARTESIAN_POINT ( 'NONE',  ( 132.0563630623057065, 41.51825634609595284, 2.881408396022717255 ) ) ;
#4682=CARTESIAN_POINT ( 'NONE',  ( 149.9872551245000807, 52.05943539582079893, 10.63948890275607795 ) ) ;
#4683=CARTESIAN_POINT ( 'NONE',  ( -8.481162655887866109, 7.942265590435539480, 83.80506270299520111 ) ) ;
#4685=B_SPLINE_CURVE_WITH_KNOTS ( 'NONE', 3,
 ( #58289, #42796, #69189, #69529, #53697, #21692, #58628, #4826, #27313, #31566, #59662, #10444, #31918, #43491, #63578, #63919, #32265, #47727, #37882, #64263, #16760, #26972, #5517, #5177, #235, #16071, #58978, #43143, #64967, #27663, #26639, #592, #15733, #64612, #48756, #16423, #59325, #32603, #38221, #6210, #11476, #53002, #32944, #36850, #54030, #26297, #5856 ),
 .UNSPECIFIED., .F., .F.,
 ( 4, 2, 2, 2, 2, 2, 2, 2, 2, 2, 2, 1, 2, 2, 2, 2, 2, 2, 2, 2, 2, 2, 2, 4 ),
 ( 0.000000000000000000, 0.003297771944418886533, 0.004122214930523581712, 0.004946657916628276891, 0.006595543888837667248, 0.007419986874942389316, 0.008244429861047111383, 0.009068872847151831715, 0.009893315833256553782, 0.01154220180546602914, 0.01236664479157077029, 0.01319108777767551144, 0.01401553076378025085, 0.01483997374988498853, 0.01566441673598972795, 0.01648885972209446910, 0.01813774569430390976, 0.01896218868040865438, 0.01978663166651340247, 0.02061107465261814709, 0.02143551763872289170, 0.02308440361093238441, 0.02473328958314187712, 0.02638217555535137329 ),
 .UNSPECIFIED. ) ;
#4688=CARTESIAN_POINT ( 'NONE',  ( -60.97011009284707939, 16.34812508431679134, 69.29634183800428104 ) ) ;
#4689=ORIENTED_EDGE ( 'NONE', *, *, #15095, .T. ) ;
#4692=ORIENTED_EDGE ( 'NONE', *, *, #24012, .F. ) ;
#4693=CARTESIAN_POINT ( 'NONE',  ( 40.07437664823315515, 9.512804923423081149, 83.62581982957500770 ) ) ;
#4700=CARTESIAN_POINT ( 'NONE',  ( -7.336630171688589996, 7.867399454768227329, 3.271030448983515804 ) ) ;
#4702=CARTESIAN_POINT ( 'NONE',  ( 176.6156959113760365, 75.60152827082541194, -37.68265618882365686 ) ) ;
#4703=EDGE_CURVE ( 'NONE', #59711, #8166, #66737, .T. ) ;
#4705=CARTESIAN_POINT ( 'NONE',  ( 164.9484057732149438, 63.70705320020925200, 91.28889419560704255 ) ) ;
#4707=ADVANCED_FACE ( 'NONE', ( #10643 ), #441, .F. ) ;
#4711=CARTESIAN_POINT ( 'NONE',  ( 8.337549025192453556, 7.382630697225778249, 36.52698723587364071 ) ) ;
#4712=CARTESIAN_POINT ( 'NONE',  ( 197.9868529032975744, 99.18611233336802968, 33.34703807473912462 ) ) ;
#4713=CARTESIAN_POINT ( 'NONE',  ( -86.07103743106915772, 26.37291038375863650, 92.84346461836889830 ) ) ;
#4715=ORIENTED_EDGE ( 'NONE', *, *, #59441, .F. ) ;
#4718=CARTESIAN_POINT ( 'NONE',  ( -55.05276343752910151, -170.0000000000000000, -42.71632399845987749 ) ) ;
#4719=CARTESIAN_POINT ( 'NONE',  ( 197.2200752504830916, 96.62072041958360558, -70.00624559352947074 ) ) ;
#4720=CARTESIAN_POINT ( 'NONE',  ( -33.12994257348895388, 10.89587983539684046, 57.24998983726293034 ) ) ;
#4721=CARTESIAN_POINT ( 'NONE',  ( 110.2429982417149574, -170.0000000000000000, 71.45576479620103783 ) ) ;
#4722=CARTESIAN_POINT ( 'NONE',  ( 155.7262569076171701, 56.30477153194512852, -63.11863533963168749 ) ) ;
#4724=CARTESIAN_POINT ( 'NONE',  ( -156.0171627975468027, 69.90368824761765154, -38.57899779329219569 ) ) ;
#4727=B_SPLINE_CURVE_WITH_KNOTS ( 'NONE', 3,
 ( #56541, #40020, #34417, #7327, #18566, #39673, #51619, #30169, #18223, #55863, #29465, #3428, #13303, #67459, #24204, #34757, #46325, #13632, #61130, #56194, #8010, #24891, #23854, #29124, #45292, #56901, #3092, #12956, #67801, #39332, #8369, #7678, #50924, #29816, #51279, #8719, #40704, #60774, #18918, #12599, #34055, #67128, #50574, #2394 ),
 .UNSPECIFIED., .F., .F.,
 ( 4, 2, 2, 2, 2, 2, 2, 2, 2, 2, 2, 2, 2, 2, 2, 2, 2, 2, 2, 2, 2, 4 ),
 ( 1.387778780781445676E-17, 0.004120577325733522020, 0.006180865988600256142, 0.008241154651466991998, 0.01030144331433372612, 0.01133158764576704981, 0.01236173197720037524, 0.01339187630863369893, 0.01442202064006702263, 0.01545216497150034632, 0.01648230930293367175, 0.01699738146865035354, 0.01751245363436703534, 0.01854259796580040934, 0.01957274229723378334, 0.02060288662866715387, 0.02266317529153390881, 0.02472346395440066374, 0.02678375261726741868, 0.02781389694870082738, 0.02884404128013423607, 0.03296461860586797493 ),
 .UNSPECIFIED. ) ;
#4728=CARTESIAN_POINT ( 'NONE',  ( 69.83260694998128315, 15.39825517924928988, -13.23929702939983954 ) ) ;
#4730=CARTESIAN_POINT ( 'NONE',  ( 104.0290905220488469, 26.11184870228230892, 94.99999999999866418 ) ) ;
#4731=CARTESIAN_POINT ( 'NONE',  ( 117.4711568421290053, 33.49899443629671936, -14.51207208499641332 ) ) ;
#4734=CARTESIAN_POINT ( 'NONE',  ( 21.25987915030395925, 6.737472588634914494, 32.37940707539839735 ) ) ;
#4735=CARTESIAN_POINT ( 'NONE',  ( 134.3182571105339491, 42.88121222759021833, -9.178760341931971212 ) ) ;
#4736=EDGE_LOOP ( 'NONE', ( #52229, #39664, #60234, #6306 ) ) ;
#4742=CARTESIAN_POINT ( 'NONE',  ( 36.99999522780156269, 9.122638774496635961, -50.22900309971504385 ) ) ;
#4746=CARTESIAN_POINT ( 'NONE',  ( 197.2199163281728147, 98.22431253015354002, 62.88886963507403749 ) ) ;
#4747=B_SPLINE_CURVE_WITH_KNOTS ( 'NONE', 3,
 ( #57970, #62906, #20678, #3136, #67496, #35482, #56943, #8763, #30212, #4165, #24931, #62565, #14377, #51663, #46365, #35832, #30547, #51998, #25631, #47065, #69543, #38586, #27676, #64979 ),
 .UNSPECIFIED., .F., .F.,
 ( 4, 2, 2, 2, 2, 2, 2, 2, 2, 2, 2, 4 ),
 ( 0.01050068220271658387, 0.01181995631628032263, 0.01247959337306220329, 0.01313923042984408221, 0.01445850454340786087, 0.01511814160018975020, 0.01577777865697164300, 0.01709705277053541819, 0.01775668982731730752, 0.01841632688409919338, 0.01973560099766296164, 0.02105487511122672642 ),
 .UNSPECIFIED. ) ;
#4749=CARTESIAN_POINT ( 'NONE',  ( 36.99625334683020839, 8.108440754877200618, 57.13776175391618750 ) ) ;
#4750=CARTESIAN_POINT ( 'NONE',  ( 14.08699529666005823, 6.452200550165255954, -8.865815044285954016 ) ) ;
#4752=CARTESIAN_POINT ( 'NONE',  ( 20.74185656603722450, 7.717159106492280429, 5.017094231853548081 ) ) ;
#4753=CARTESIAN_POINT ( 'NONE',  ( 188.0081045302011091, 85.89855126821611009, 60.75689848136790516 ) ) ;
#4755=CARTESIAN_POINT ( 'NONE',  ( -79.61931371420119774, 22.68640080971621487, -35.16116692163456037 ) ) ;
#4760=EDGE_CURVE ( 'NONE', #56686, #52761, #69269, .T. ) ;
#4763=CARTESIAN_POINT ( 'NONE',  ( 187.2465631085773339, 85.06582225041682932, 14.26867246100197661 ) ) ;
#4767=CARTESIAN_POINT ( 'NONE',  ( -107.7886332494339570, 36.81249801143973599, -37.40149486631479192 ) ) ;
#4772=CARTESIAN_POINT ( 'NONE',  ( 173.9662866282169205, 71.69964987613715834, 88.12574805637403585 ) ) ;
#4774=CARTESIAN_POINT ( 'NONE',  ( 117.6916924104495479, 32.48309187151379973, 64.97158662374468463 ) ) ;
#4779=VECTOR ( 'NONE', #45800, 1000.000000000000000 ) ;
#4781=CARTESIAN_POINT ( 'NONE',  ( -99.10260179032844974, 31.19580119595418211, 44.81688323301395371 ) ) ;
#4786=EDGE_CURVE ( 'NONE', #50015, #60490, #1385, .T. ) ;
#4790=ORIENTED_EDGE ( 'NONE', *, *, #32185, .T. ) ;
#4791=CARTESIAN_POINT ( 'NONE',  ( -118.8504142000305563, 42.02789424825281372, -12.97858553378794610 ) ) ;
#4796=CARTESIAN_POINT ( 'NONE',  ( -7.825402957745087207, 6.891034867348158954, 45.11558103944722120 ) ) ;
#4798=CARTESIAN_POINT ( 'NONE',  ( -103.8075682002152007, 34.69679037577547831, 84.35934033286845590 ) ) ;
#4801=CARTESIAN_POINT ( 'NONE',  ( -55.05276343752909440, 14.68156374112637330, -8.371773407996169425 ) ) ;
#4802=CARTESIAN_POINT ( 'NONE',  ( -133.1566699306513328, 52.70203339370771545, -71.14848980824044133 ) ) ;
#4804=CARTESIAN_POINT ( 'NONE',  ( -100.4466073551323007, 31.85873123265078277, 3.887263631221759663 ) ) ;
#4807=ORIENTED_EDGE ( 'NONE', *, *, #63113, .T. ) ;
#4809=CARTESIAN_POINT ( 'NONE',  ( -170.2747214445849693, 84.01465441107040988, -35.26017206050354247 ) ) ;
#4812=CARTESIAN_POINT ( 'NONE',  ( -76.33235143960695268, 22.51916353135074900, 45.04974780934608702 ) ) ;
#4813=CARTESIAN_POINT ( 'NONE',  ( 80.73012746365749592, 17.49169339352364716, 41.86980492191601400 ) ) ;
#4814=CARTESIAN_POINT ( 'NONE',  ( 70.11969827741708627, 15.47408882293423993, -40.76595231452924395 ) ) ;
#4815=CARTESIAN_POINT ( 'NONE',  ( 42.48820792780864508, 9.847387255477766388, -49.95978026808956685 ) ) ;
#4816=CARTESIAN_POINT ( 'NONE',  ( 206.7099580236350107, 109.1417833474364443, 70.78891289186701385 ) ) ;
#4818=ORIENTED_EDGE ( 'NONE', *, *, #27003, .F. ) ;
#4821=CARTESIAN_POINT ( 'NONE',  ( -15.22871623201694469, 7.486724405784662473, -44.14333518623142538 ) ) ;
#4822=EDGE_CURVE ( 'NONE', #52905, #31875, #62567, .T. ) ;
#4825=CARTESIAN_POINT ( 'NONE',  ( 94.11733320392093560, 23.18939451097131155, 63.56296009108370981 ) ) ;
#4826=CARTESIAN_POINT ( 'NONE',  ( 153.2384531768735769, 54.43344429203622781, -10.57026377980718657 ) ) ;
#4829=CARTESIAN_POINT ( 'NONE',  ( 36.76746179515744473, 8.081433644308901876, -62.93801830221686089 ) ) ;
#4830=CARTESIAN_POINT ( 'NONE',  ( -99.10674985723794350, 32.31836975419496838, -76.17106620709191134 ) ) ;
#4832=CARTESIAN_POINT ( 'NONE',  ( -36.37229078872273647, 11.47648211215765812, -21.64289120047060067 ) ) ;
#4833=ORIENTED_EDGE ( 'NONE', *, *, #30042, .F. ) ;
#4839=CARTESIAN_POINT ( 'NONE',  ( -24.18258876560172155, 8.512344710720682883, 8.913579529955121927 ) ) ;
#4841=EDGE_CURVE ( 'NONE', #8386, #11991, #57577, .T. ) ;
#4842=CARTESIAN_POINT ( 'NONE',  ( -5.416136198635861376, 6.745992685878681172, 30.50884761992566752 ) ) ;
#4844=CARTESIAN_POINT ( 'NONE',  ( 156.3797504404255392, 58.07856685387020690, -51.04775918292205716 ) ) ;
#4846=EDGE_CURVE ( 'NONE', #5410, #10221, #63300, .T. ) ;
#4848=VERTEX_POINT ( 'NONE', #21141 ) ;
#4851=CARTESIAN_POINT ( 'NONE',  ( -189.9638655956220532, 108.0957249433520815, -18.49776328886134280 ) ) ;
#4852=CARTESIAN_POINT ( 'NONE',  ( 173.5836858989432017, 72.71885240881779566, -16.59373086107160944 ) ) ;
#4853=CARTESIAN_POINT ( 'NONE',  ( -107.2385267828037030, 36.51474259889401708, 59.23132442209924164 ) ) ;
#4858=CARTESIAN_POINT ( 'NONE',  ( 88.99522780200244654, 20.24180937454204354, 71.17773731472695431 ) ) ;
#4859=CARTESIAN_POINT ( 'NONE',  ( 204.3091227790962421, 107.5190503136782354, -9.481380442157895772 ) ) ;
#4860=CARTESIAN_POINT ( 'NONE',  ( -142.7660513839927034, 58.66578555228782221, 88.60591720006654270 ) ) ;
#4861=CARTESIAN_POINT ( 'NONE',  ( 139.6203063421347110, 45.01495791936839908, 32.18546459676473148 ) ) ;
#4864=CARTESIAN_POINT ( 'NONE',  ( 82.95856197793166587, 19.25847567427442542, 3.809032710648850184 ) ) ;
#4865=CARTESIAN_POINT ( 'NONE',  ( 161.1112535418156710, 61.83422628788727593, 16.62590986968896090 ) ) ;
#4867=VERTEX_POINT ( 'NONE', #37293 ) ;
#4869=CARTESIAN_POINT ( 'NONE',  ( 178.1965488566139868, 77.14488558164480025, 56.71789026606290918 ) ) ;
#4871=CARTESIAN_POINT ( 'NONE',  ( -108.9136445001389859, 36.28030794288191174, -39.00605114454056377 ) ) ;
#4873=AXIS2_PLACEMENT_3D ( 'NONE', #1842, #50708, #55633 ) ;
#4876=CARTESIAN_POINT ( 'NONE',  ( 150.9013375937531407, 53.96275732797613500, 13.69346484706898437 ) ) ;
#4878=FACE_OUTER_BOUND ( 'NONE', #57232, .T. ) ;
#4883=CARTESIAN_POINT ( 'NONE',  ( -102.2801239173131052, 33.91021738430207222, 3.674523915951417585 ) ) ;
#4886=CARTESIAN_POINT ( 'NONE',  ( 140.8984307802396359, 45.84194788389002895, 61.22238341269675743 ) ) ;
#4887=CARTESIAN_POINT ( 'NONE',  ( -176.3763474213711504, 92.36993073950279154, 31.55091585264105447 ) ) ;
#4889=CARTESIAN_POINT ( 'NONE',  ( -35.17600017528511813, 10.23461991275926763, -76.16909263517460715 ) ) ;
#4890=CARTESIAN_POINT ( 'NONE',  ( 88.53025347111697840, 21.14438024052372711, 29.94122557606181800 ) ) ;
#4892=CARTESIAN_POINT ( 'NONE',  ( 46.12611922993085045, 10.39838587005582049, 7.238115754011925418 ) ) ;
#4893=VERTEX_POINT ( 'NONE', #58403 ) ;
#4895=VECTOR ( 'NONE', #6302, 1000.000000000000000 ) ;
#4898=CARTESIAN_POINT ( 'NONE',  ( 212.1669304543881651, 119.0398299474538959, -17.68208531959118091 ) ) ;
#4900=CARTESIAN_POINT ( 'NONE',  ( -152.9119739516381173, 67.12135129037710612, -75.85561049297035652 ) ) ;
#4903=CARTESIAN_POINT ( 'NONE',  ( 204.6977192012829789, 106.3443248447423315, -36.32593103262158252 ) ) ;
#4907=CYLINDRICAL_SURFACE ( 'NONE', #36334, 7.500000000000020428 ) ;
#4910=CARTESIAN_POINT ( 'NONE',  ( -71.57025115638938928, 20.80908992785612099, 62.28357928173872438 ) ) ;
#4911=CARTESIAN_POINT ( 'NONE',  ( 207.4696221732442609, 110.2206209205161969, -77.65139825956335073 ) ) ;
#4912=CARTESIAN_POINT ( 'NONE',  ( 56.30011474572736319, 11.21470186335419683, -73.41388707145787862 ) ) ;
#4913=CARTESIAN_POINT ( 'NONE',  ( -121.2119672714299270, 44.67540322905997385, 70.84369768003189449 ) ) ;
#4915=PLANE ( 'NONE',  #62582 ) ;
#4918=CARTESIAN_POINT ( 'NONE',  ( -71.37402418445425667, 19.67651958824263758, 62.99220628321225490 ) ) ;
#4919=CARTESIAN_POINT ( 'NONE',  ( -173.1211646369891355, 87.12891641440857882, 72.66624519710475738 ) ) ;
#4923=CARTESIAN_POINT ( 'NONE',  ( 55.51547041749725508, 11.05727559334826893, -43.46285331346358305 ) ) ;
#4924=FACE_OUTER_BOUND ( 'NONE', #68709, .T. ) ;
#4932=CARTESIAN_POINT ( 'NONE',  ( -128.1282195935087600, 49.19720162550165554, 30.95687802063085670 ) ) ;
#4945=ORIENTED_EDGE ( 'NONE', *, *, #30263, .T. ) ;
#4949=CARTESIAN_POINT ( 'NONE',  ( -169.1041038606267648, 82.76530082651285625, -21.71656691506287018 ) ) ;
#4951=CARTESIAN_POINT ( 'NONE',  ( 64.93495251696903381, 13.12601614965099017, 30.05863598689030880 ) ) ;
#4956=ORIENTED_EDGE ( 'NONE', *, *, #22874, .T. ) ;
#4957=CARTESIAN_POINT ( 'NONE',  ( -81.90266786693713641, 23.58030232261292980, 17.85658396585434105 ) ) ;
#4960=CARTESIAN_POINT ( 'NONE',  ( 8.336882341125877005, 6.376438415325265119, -44.00243688774482820 ) ) ;
#4961=CARTESIAN_POINT ( 'NONE',  ( -180.4654253355436424, 95.69358270527506249, 63.61568511560930261 ) ) ;
#4962=CARTESIAN_POINT ( 'NONE',  ( 127.1040286383415037, 37.49395136275125395, 60.58097942537040126 ) ) ;
#4965=CARTESIAN_POINT ( 'NONE',  ( -36.19806511523993464, 10.42097839459253983, 85.59994145001356003 ) ) ;
#4966=CARTESIAN_POINT ( 'NONE',  ( 157.4703587214989113, 57.65129005721575339, 44.40946747225338953 ) ) ;
#4967=AXIS2_PLACEMENT_3D ( 'NONE', #36555, #36209, #9132 ) ;
#4970=CARTESIAN_POINT ( 'NONE',  ( 140.4641697461913452, 46.75994457266057225, -66.78132054738273382 ) ) ;
#4975=CARTESIAN_POINT ( 'NONE',  ( 41.81982603358027006, 8.735900550613179050, 17.68552455925381039 ) ) ;
#4976=CARTESIAN_POINT ( 'NONE',  ( 176.6156959113759513, 75.60152827082541194, 16.00644499210370597 ) ) ;
#4977=CARTESIAN_POINT ( 'NONE',  ( -118.4470345550925856, 42.96051736048244152, -43.45603041284294932 ) ) ;
#4981=CARTESIAN_POINT ( 'NONE',  ( 34.63049175740484742, 7.836802300168049129, -91.01871974183544012 ) ) ;
#4982=CARTESIAN_POINT ( 'NONE',  ( -120.6739978760426055, 44.33795494230366074, -63.86731139866689944 ) ) ;
#4985=CARTESIAN_POINT ( 'NONE',  ( 66.30567821786753768, 13.45988234822861251, 17.21265612671894019 ) ) ;
#4986=CARTESIAN_POINT ( 'NONE',  ( -85.36298448216594181, 26.07611629625833416, 68.17787176330473642 ) ) ;
#4987=CARTESIAN_POINT ( 'NONE',  ( 41.04421810250191527, 9.644095118781809362, -89.47936863587655409 ) ) ;
#4996=DIRECTION ( 'NONE',  ( 0.000000000000000000, 0.000000000000000000, 1.000000000000000000 ) ) ;
#4997=CARTESIAN_POINT ( 'NONE',  ( -148.6471085600700519, 64.76880961642444845, 57.60225718838557896 ) ) ;
#4999=CARTESIAN_POINT ( 'NONE',  ( 70.11438327604406595, 14.43198353181102433, -13.94311793805158040 ) ) ;
#5000=CARTESIAN_POINT ( 'NONE',  ( 135.6647932137618113, 43.70902528961477174, -36.23038487884888781 ) ) ;
#5001=CARTESIAN_POINT ( 'NONE',  ( -48.58011387679029269, 14.07568064779664851, -73.35782377364151330 ) ) ;
#5002=CARTESIAN_POINT ( 'NONE',  ( -31.43908319763710679, -170.0000000000000000, -77.16174795566554678 ) ) ;
#5006=CARTESIAN_POINT ( 'NONE',  ( 183.4883381146856891, 82.52303242823217033, 83.37056451303936910 ) ) ;
#5008=CARTESIAN_POINT ( 'NONE',  ( -171.4943428135323416, 86.82484920477511992, -7.997380618965306276 ) ) ;
#5013=CARTESIAN_POINT ( 'NONE',  ( -9.763294602873866523, 7.024900256480053784, 71.70961793505638582 ) ) ;
#5014=CARTESIAN_POINT ( 'NONE',  ( -80.31691774066408129, 22.95709084517030618, -8.450926537141361550 ) ) ;
#5015=CARTESIAN_POINT ( 'NONE',  ( -86.05211524933166345, 26.36495896184001708, -95.00000000000133582 ) ) ;
#5016=CARTESIAN_POINT ( 'NONE',  ( 41.80536115778106421, 8.734184316430665618, -23.38395991615332647 ) ) ;
#5017=CARTESIAN_POINT ( 'NONE',  ( -78.66644367742111399, -170.0000000000000000, 11.07365054920946079 ) ) ;
#5018=FACE_OUTER_BOUND ( 'NONE', #39727, .T. ) ;
#5019=CARTESIAN_POINT ( 'NONE',  ( 162.6205203824432317, 63.07332653227192054, 69.21143974246140829 ) ) ;
#5021=EDGE_LOOP ( 'NONE', ( #61322, #21114 ) ) ;
#5022=CARTESIAN_POINT ( 'NONE',  ( -125.4433371161043311, 46.19736518073186460, -34.91370389823390497 ) ) ;
#5024=FACE_OUTER_BOUND ( 'NONE', #51493, .T. ) ;
#5025=DIRECTION ( 'NONE',  ( 0.000000000000000000, 0.000000000000000000, 1.000000000000000000 ) ) ;
#5026=CARTESIAN_POINT ( 'NONE',  ( 150.0973882686025149, 52.13852366454154463, 11.46627940338942153 ) ) ;
#5027=CARTESIAN_POINT ( 'NONE',  ( -11.83735969105690167, 8.195029568776297069, 84.95963025573755090 ) ) ;
#5029=VECTOR ( 'NONE', #25803, 1000.000000000000000 ) ;
#5034=CARTESIAN_POINT ( 'NONE',  ( -71.28077210551055032, 20.70883253687733117, -95.00000000000133582 ) ) ;
#5035=ORIENTED_EDGE ( 'NONE', *, *, #9397, .T. ) ;
#5036=ORIENTED_EDGE ( 'NONE', *, *, #34058, .F. ) ;
#5037=VECTOR ( 'NONE', #55405, 1000.000000000000000 ) ;
#5042=CARTESIAN_POINT ( 'NONE',  ( -58.32860549785896609, 15.58423118879329294, -76.31204309374547279 ) ) ;
#5043=FACE_OUTER_BOUND ( 'NONE', #147, .T. ) ;
#5044=CARTESIAN_POINT ( 'NONE',  ( 33.03621582719333816, 7.666716336587136027, -20.24858811402686953 ) ) ;
#5045=CARTESIAN_POINT ( 'NONE',  ( 173.9457771591584674, 73.05793967547533896, -46.04376121573756819 ) ) ;
#5046=CARTESIAN_POINT ( 'NONE',  ( 163.4909271546005698, 62.48739187115877058, 86.07095713937944481 ) ) ;
#5049=EDGE_LOOP ( 'NONE', ( #1005, #792, #45442, #14583 ) ) ;
#5052=CARTESIAN_POINT ( 'NONE',  ( -27.70185240367227664, 10.02491413133431486, 31.20927824995889921 ) ) ;
#5053=CARTESIAN_POINT ( 'NONE',  ( 197.3756653044963514, 98.41886189307120958, 35.07559596873900176 ) ) ;
#5054=CARTESIAN_POINT ( 'NONE',  ( -86.16954081945932842, 26.41440641755240293, 91.85847073401009766 ) ) ;
#5056=EDGE_LOOP ( 'NONE', ( #42269, #24175, #40184, #42974 ) ) ;
#5066=CARTESIAN_POINT ( 'NONE',  ( 20.74093720376649941, 6.709541214524348263, -21.82772143202600290 ) ) ;
#5067=AXIS2_PLACEMENT_3D ( 'NONE', #6785, #12072, #61300 ) ;
#5068=CARTESIAN_POINT ( 'NONE',  ( 198.7765072002625288, -170.0000000000000000, 94.99999999999866418 ) ) ;
#5072=CARTESIAN_POINT ( 'NONE',  ( 68.62997155117723480, 15.08415013720829201, -11.37927540543296701 ) ) ;
#5074=CARTESIAN_POINT ( 'NONE',  ( -86.16710354151692286, 26.41338104675946852, -42.38095692992142460 ) ) ;
#5075=CARTESIAN_POINT ( 'NONE',  ( 102.7472068462325012, 25.56604832181697162, 90.36773254186026350 ) ) ;
#5077=CARTESIAN_POINT ( 'NONE',  ( 112.5537757279407458, 31.07998172410697535, -9.426844704073509718 ) ) ;
#5080=CARTESIAN_POINT ( 'NONE',  ( 181.9406741394861058, 79.47484497224790800, -36.26201039870598919 ) ) ;
#5082=CARTESIAN_POINT ( 'NONE',  ( -155.6080424972482774, 70.89247817759412840, 87.53634334609833445 ) ) ;
#5087=CARTESIAN_POINT ( 'NONE',  ( -156.6644740249450649, 71.86407434531901117, -17.72729415336047865 ) ) ;
#5088=CARTESIAN_POINT ( 'NONE',  ( 36.09469435220864852, 9.015003538710487874, -49.86883716977957448 ) ) ;
#5089=CARTESIAN_POINT ( 'NONE',  ( 179.4207200232661137, 76.93724985992177778, 71.01710357248663286 ) ) ;
#5094=ADVANCED_FACE ( 'NONE', ( #38341 ), #61199, .T. ) ;
#5097=CARTESIAN_POINT ( 'NONE',  ( 39.40195752203892710, 8.409560354027400209, 56.75838489642694640 ) ) ;
#5098=CARTESIAN_POINT ( 'NONE',  ( -152.2964402771108610, 66.58174574061952455, 72.03110441543591946 ) ) ;
#5100=CARTESIAN_POINT ( 'NONE',  ( 185.5572090022886016, 83.24697331286186852, 69.69128790936149187 ) ) ;
#5105=CARTESIAN_POINT ( 'NONE',  ( 14.81290967676422277, 7.477658233646008235, 3.217552154449582424 ) ) ;
#5109=DIRECTION ( 'NONE',  ( 1.000000000000000000, 0.000000000000000000, -0.000000000000000000 ) ) ;
#5110=CARTESIAN_POINT ( 'NONE',  ( -132.9109786433856755, 51.29129389542017492, -39.75304253929575538 ) ) ;
#5111=CARTESIAN_POINT ( 'NONE',  ( -108.5248383251030901, 37.21456094989613206, -46.67577077482953030 ) ) ;
#5113=VERTEX_POINT ( 'NONE', #68215 ) ;
#5115=CARTESIAN_POINT ( 'NONE',  ( -23.99924996210628336, 8.487987924059016365, -14.99299851994305577 ) ) ;
#5116=CARTESIAN_POINT ( 'NONE',  ( 197.5344630110112973, 98.61758706718747192, 7.618816888282892386 ) ) ;
#5121=CARTESIAN_POINT ( 'NONE',  ( 129.4887940973039235, 40.01039828304091373, -64.25216638727819429 ) ) ;
#5122=CARTESIAN_POINT ( 'NONE',  ( 132.7179291807801746, 40.74118679001691845, 29.59377605348581142 ) ) ;
#5125=CARTESIAN_POINT ( 'NONE',  ( 157.4703587214989113, 57.65129005721575339, -89.81328548006499091 ) ) ;
#5127=CIRCLE ( 'NONE', #24237, 242.4895526022646379 ) ;
#5129=CARTESIAN_POINT ( 'NONE',  ( 8.000000000000007105, 249.8719672152120381, -95.00000000000133582 ) ) ;
#5131=( GEOMETRIC_REPRESENTATION_CONTEXT ( 3 ) GLOBAL_UNCERTAINTY_ASSIGNED_CONTEXT ( ( #65583 ) ) GLOBAL_UNIT_ASSIGNED_CONTEXT ( ( #3143, #55544, #13007 ) ) REPRESENTATION_CONTEXT ( 'NONE', 'WORKASPACE' ) );
#5136=CARTESIAN_POINT ( 'NONE',  ( -167.0073208999199608, 82.02183861952778443, 7.124899887039663149 ) ) ;
#5140=CARTESIAN_POINT ( 'NONE',  ( -178.7458319892713803, 93.61502008198021940, -10.39986922783644374 ) ) ;
#5141=CARTESIAN_POINT ( 'NONE',  ( -166.3231866619663890, 81.31146386205588783, -65.87609374347549362 ) ) ;
#5144=CARTESIAN_POINT ( 'NONE',  ( -106.2831548001319959, 36.00138616880182241, 85.35841622373546045 ) ) ;
#5146=CARTESIAN_POINT ( 'NONE',  ( 56.48986020701288169, 12.27998416584893704, 94.71400107496813803 ) ) ;
#5147=CYLINDRICAL_SURFACE ( 'NONE', #1901, 7.500000000000020428 ) ;
#5151=CARTESIAN_POINT ( 'NONE',  ( 79.11678624235125312, 16.99307331934756604, -16.46842441967982751 ) ) ;
#5152=CARTESIAN_POINT ( 'NONE',  ( -132.9227230387960788, 52.53474289881228287, -66.62845719056252847 ) ) ;
#5154=CARTESIAN_POINT ( 'NONE',  ( -97.47339919287389876, 30.40512551257286944, 16.95259712630159044 ) ) ;
#5155=CARTESIAN_POINT ( 'NONE',  ( -154.4518102898914549, 68.48895432927903926, -90.34576860233968887 ) ) ;
#5160=CARTESIAN_POINT ( 'NONE',  ( 11.82322073186613309, 6.406156243758797331, 31.14383489137281202 ) ) ;
#5165=CARTESIAN_POINT ( 'NONE',  ( 84.28078136020371858, 18.63296074526051527, 44.33893942252232989 ) ) ;
#5167=CARTESIAN_POINT ( 'NONE',  ( 41.34269507549202416, 9.685203600174698835, -50.38080312760155266 ) ) ;
#5171=DIRECTION ( 'NONE',  ( -0.000000000000000000, 1.000000000000000000, -0.000000000000000000 ) ) ;
#5174=CARTESIAN_POINT ( 'NONE',  ( -34.51918258780364823, 10.11719938103014904, 4.029186606375436241 ) ) ;
#5175=CARTESIAN_POINT ( 'NONE',  ( 83.59652366361571296, 19.46709838196855813, 70.92029102677756214 ) ) ;
#5176=CARTESIAN_POINT ( 'NONE',  ( 92.21252738308864139, 22.47457138983957137, 59.02458724508797872 ) ) ;
#5177=CARTESIAN_POINT ( 'NONE',  ( 149.9838583332407893, 52.05699766415857255, -17.30813132279020294 ) ) ;
#5180=CARTESIAN_POINT ( 'NONE',  ( 38.42384008295177011, 8.283891555743467805, -62.51250981452189137 ) ) ;
#5191=CARTESIAN_POINT ( 'NONE',  ( 9.689943677145722134, 7.388265075009365468, -74.23619429177909979 ) ) ;
#5195=CARTESIAN_POINT ( 'NONE',  ( -0.8011128725815451768, 6.535315321814186618, 40.25565733622043041 ) ) ;
#5197=CARTESIAN_POINT ( 'NONE',  ( 80.46041939316872060, 18.46168943176929034, 86.62235641862685043 ) ) ;
#5198=AXIS2_PLACEMENT_3D ( 'NONE', #13319, #8030, #50945 ) ;
#5202=CARTESIAN_POINT ( 'NONE',  ( 179.4227152810057930, 78.36166152262363482, -24.20640214036799520 ) ) ;
#5203=CARTESIAN_POINT ( 'NONE',  ( -109.7790042512817905, 37.90666514836944145, 64.57243962987085695 ) ) ;
#5205=CARTESIAN_POINT ( 'NONE',  ( -132.8150886319751578, 52.45790550853840273, -45.31429239349645144 ) ) ;
#5207=DIRECTION ( 'NONE',  ( -0.000000000000000000, 1.000000000000000000, -0.000000000000000000 ) ) ;
#5208=CARTESIAN_POINT ( 'NONE',  ( 94.07616572255072640, 22.09777530676767654, 63.03225789469448159 ) ) ;
#5209=CARTESIAN_POINT ( 'NONE',  ( -154.6244975120027902, 68.64332268850641583, 86.39598974807935861 ) ) ;
#5211=VERTEX_POINT ( 'NONE', #46391 ) ;
#5213=CARTESIAN_POINT ( 'NONE',  ( 82.34401416830218068, 19.05992892018826979, 4.207522528255770666 ) ) ;
#5214=CARTESIAN_POINT ( 'NONE',  ( 159.2258951716709703, 60.31399909112331414, 2.759764520436461588 ) ) ;
#5216=ORIENTED_EDGE ( 'NONE', *, *, #11597, .F. ) ;
#5218=ORIENTED_EDGE ( 'NONE', *, *, #23199, .F. ) ;
#5220=CARTESIAN_POINT ( 'NONE',  ( -76.78936026062118003, 21.61552955137052479, -23.03615461302700851 ) ) ;
#5227=CARTESIAN_POINT ( 'NONE',  ( -178.2381786520593892, 93.01028335822118720, 43.81022153523580442 ) ) ;
#5232=CARTESIAN_POINT ( 'NONE',  ( -143.3980294393558950, 60.45217072626398647, 33.86310790016815275 ) ) ;
#5235=CARTESIAN_POINT ( 'NONE',  ( 139.3067271572849108, 44.81402783181196980, 69.01324371968860305 ) ) ;
#5236=CARTESIAN_POINT ( 'NONE',  ( -167.9853834315979384, 81.58767916550894483, 43.80779636558261103 ) ) ;
#5237=CARTESIAN_POINT ( 'NONE',  ( 128.0882145863933488, 39.20607399008169125, 59.03564582321932619 ) ) ;
#5239=ORIENTED_EDGE ( 'NONE', *, *, #60440, .T. ) ;
#5240=CARTESIAN_POINT ( 'NONE',  ( 45.76405797021010358, 10.34101216371941767, 14.54853712646751340 ) ) ;
#5248=CARTESIAN_POINT ( 'NONE',  ( -102.2801239173131194, -170.0000000000000000, -15.67002667451224163 ) ) ;
#5251=CARTESIAN_POINT ( 'NONE',  ( -131.2803255164624545, 50.14412978403778709, 70.18912820271620490 ) ) ;
#5256=CARTESIAN_POINT ( 'NONE',  ( -78.19438069111009781, 23.21811806230639164, 57.26275173013681297 ) ) ;
#5257=CARTESIAN_POINT ( 'NONE',  ( 181.5072453427591199, 79.03352099595181812, 29.30859410551139277 ) ) ;
#5258=CARTESIAN_POINT ( 'NONE',  ( 60.63507185982732040, 12.13307030573224310, -62.94891509126097873 ) ) ;
#5259=CARTESIAN_POINT ( 'NONE',  ( -78.18913509716431065, 22.13995206110505265, 18.57365054920947145 ) ) ;
#5261=CARTESIAN_POINT ( 'NONE',  ( 21.75198946226450403, 7.772524967554921282, 32.94053441732803833 ) ) ;
#5262=CARTESIAN_POINT ( 'NONE',  ( 202.3068201863369495, 103.1211636617681791, 83.26500311953536482 ) ) ;
#5263=CARTESIAN_POINT ( 'NONE',  ( 164.8908506817023749, 64.97619709085124384, -69.34418866066772580 ) ) ;
#5269=ORIENTED_EDGE ( 'NONE', *, *, #7319, .T. ) ;
#5270=CARTESIAN_POINT ( 'NONE',  ( -28.13527276074848160, 10.08983026464525068, -76.39933447701551472 ) ) ;
#5271=CARTESIAN_POINT ( 'NONE',  ( 55.90536342106781831, 11.13510150712953184, -45.65778433454865848 ) ) ;
#5282=DIRECTION ( 'NONE',  ( -1.000000000000000000, 0.000000000000000000, 0.000000000000000000 ) ) ;
#5283=CARTESIAN_POINT ( 'NONE',  ( 186.6289143948428944, 85.88097584402285634, -92.34696716306295627 ) ) ;
#5284=CARTESIAN_POINT ( 'NONE',  ( 61.33627421985470818, 12.28939706835342882, 71.47105798233256735 ) ) ;
#5295=LINE ( 'NONE', #63702, #33005 ) ;
#5298=CARTESIAN_POINT ( 'NONE',  ( 11.47475555585564422, 7.407171684781389764, 85.05957700157702561 ) ) ;
#5299=ORIENTED_EDGE ( 'NONE', *, *, #15797, .T. ) ;
#5301=CARTESIAN_POINT ( 'NONE',  ( -102.2801239173131052, 32.78103895658057354, 57.36362509687880618 ) ) ;
#5304=CARTESIAN_POINT ( 'NONE',  ( -71.56718866013693514, 19.74312628447962936, 40.38945691434815899 ) ) ;
#5306=ADVANCED_FACE ( 'NONE', ( #30234 ), #63957, .F. ) ;
#5308=ORIENTED_EDGE ( 'NONE', *, *, #60924, .T. ) ;
#5309=CARTESIAN_POINT ( 'NONE',  ( -122.3994536713185255, 45.42826354555018042, 17.91575039578479078 ) ) ;
#5310=CARTESIAN_POINT ( 'NONE',  ( -180.2252811616041868, 95.40045830523432357, 67.58802342263081187 ) ) ;
#5311=CARTESIAN_POINT ( 'NONE',  ( 129.1381264900935264, 38.64720302602608371, 69.70481210122846960 ) ) ;
#5312=ORIENTED_EDGE ( 'NONE', *, *, #36471, .F. ) ;
#5313=VECTOR ( 'NONE', #51755, 1000.000000000000000 ) ;
#5322=CARTESIAN_POINT ( 'NONE',  ( -30.46060138092288838, 9.432375387772214737, 45.16858539813694051 ) ) ;
#5324=CARTESIAN_POINT ( 'NONE',  ( -144.2155061717026001, 61.10843690942975570, -63.83700193691978342 ) ) ;
#5327=DIRECTION ( 'NONE',  ( 0.000000000000000000, 0.000000000000000000, 1.000000000000000000 ) ) ;
#5330=CARTESIAN_POINT ( 'NONE',  ( -173.5372686962700470, 89.10569330281724376, 57.66624519710474317 ) ) ;
#5332=CARTESIAN_POINT ( 'NONE',  ( -118.6302575928420424, 43.07263081214308897, -40.52659648218294564 ) ) ;
#5333=CARTESIAN_POINT ( 'NONE',  ( -85.90077524418997257, 26.30132018890136791, 13.06823648188070131 ) ) ;
#5339=CARTESIAN_POINT ( 'NONE',  ( 159.2319614735955611, 59.03334608081209467, 2.761277528605094567 ) ) ;
#5340=CARTESIAN_POINT ( 'NONE',  ( 91.12448333640236342, 22.07449368110502519, -22.50004146135145433 ) ) ;
#5343=CARTESIAN_POINT ( 'NONE',  ( -34.74023699876256899, 11.17830703027882677, 4.119991731420149073 ) ) ;
#5345=LINE ( 'NONE', #25777, #10448 ) ;
#5348=CARTESIAN_POINT ( 'NONE',  ( 116.9226937574463392, 33.22232883683771121, 87.37277608428736642 ) ) ;
#5351=CARTESIAN_POINT ( 'NONE',  ( 137.4031600461561027, 44.79620770172218869, -50.13600223372191778 ) ) ;
#5352=CARTESIAN_POINT ( 'NONE',  ( -55.05276343752909440, 15.72344139423348786, -77.06087458892358200 ) ) ;
#5357=CARTESIAN_POINT ( 'NONE',  ( 36.09469435220862010, 9.015003538710470110, 57.50936519207515829 ) ) ;
#5358=CARTESIAN_POINT ( 'NONE',  ( 173.7956935488108741, 72.91723771116217279, 92.27808959496401542 ) ) ;
#5359=B_SPLINE_CURVE_WITH_KNOTS ( 'NONE', 3,
 ( #54404, #32625, #32970, #33334, #27683, #54052, #60037, #17119, #44204, #22415, #11855, #55112, #16782, #65689, #10818, #26656, #69552, #6229, #54758, #42816, #38957, #16449, #21370, #38241, #22762, #27335, #49126, #6589, #16093, #64285, #37901, #1310, #58999, #17477, #43161, #32285, #53717, #5539, #59348, #11159, #39986, #45954, #67420, #39641, #50883, #51243 ),
 .UNSPECIFIED., .F., .F.,
 ( 4, 2, 2, 2, 2, 2, 2, 2, 2, 2, 2, 2, 2, 2, 2, 2, 2, 2, 2, 2, 2, 2, 4 ),
 ( 6.938893903907228378E-18, 0.001615199098318937949, 0.003230398196637868959, 0.004037997745797339451, 0.004845597294956811678, 0.006460796393275753530, 0.007268395942435259584, 0.008075995491594763903, 0.009691194589913741317, 0.01049879413907324130, 0.01130639368823274302, 0.01211399323739224473, 0.01292159278655174819, 0.01453679188487075509, 0.01615199098318976373, 0.01695959053234924810, 0.01776719008150873594, 0.01938238917982776019, 0.02099758827814678791, 0.02180518782730633473, 0.02261278737646588155, 0.02422798647478491621, 0.02584318557310394740 ),
 .UNSPECIFIED. ) ;
#5361=CARTESIAN_POINT ( 'NONE',  ( 68.75860316153080021, 15.11750091268465113, -92.06867044945352063 ) ) ;
#5362=ORIENTED_EDGE ( 'NONE', *, *, #32620, .F. ) ;
#5363=CARTESIAN_POINT ( 'NONE',  ( 88.98064924903390249, 21.30386569031177402, 17.49345524372335703 ) ) ;
#5364=CARTESIAN_POINT ( 'NONE',  ( 184.9757174666826813, 84.09845285279330085, -23.29565043318131146 ) ) ;
#5365=CARTESIAN_POINT ( 'NONE',  ( 209.6642862813004911, 115.2127693334914085, 4.225474144247091779 ) ) ;
#5367=CARTESIAN_POINT ( 'NONE',  ( -177.1540936177023298, 91.73126115633630207, -48.55048610981354784 ) ) ;
#5370=FACE_BOUND ( 'NONE', #67995, .T. ) ;
#5371=B_SPLINE_CURVE_WITH_KNOTS ( 'NONE', 3,
 ( #67885, #45727, #46066, #18647, #19333, #3505, #2817, #23925, #56980, #40786, #41141, #18994, #40445, #28863, #51358, #61210, #29204, #67536, #61891, #8445, #13712, #35165, #62243, #55938, #56625, #3170, #55578, #14059, #7408, #50312, #35520, #8797, #30246, #51697, #24974, #46405, #19679, #62607, #14414, #2131, #23583, #66855, #45023, #66506 ),
 .UNSPECIFIED., .F., .F.,
 ( 4, 2, 2, 2, 2, 2, 2, 2, 2, 2, 2, 2, 2, 2, 2, 2, 2, 2, 2, 2, 2, 4 ),
 ( 0.02638217555535139064, 0.02805347641364859881, 0.02972477727194580352, 0.03139607813024301169, 0.03306737898854021640, 0.03390302941768884304, 0.03473867984683746968, 0.03640998070513472989, 0.03724563113428334959, 0.03808128156343197623, 0.03891693199258059593, 0.03975258242172921563, 0.04058823285087784227, 0.04142388328002646197, 0.04225953370917508167, 0.04309518413832370831, 0.04476648499662094771, 0.04643778585491818711, 0.04810908671321541957, 0.04978038757151265897, 0.05145168842980989143, 0.05312298928810713083 ),
 .UNSPECIFIED. ) ;
#5375=VERTEX_POINT ( 'NONE', #11173 ) ;
#5377=CARTESIAN_POINT ( 'NONE',  ( 55.76286625948333864, -170.0000000000000000, -95.00000000000133582 ) ) ;
#5380=CYLINDRICAL_SURFACE ( 'NONE', #54519, 7.500000000000013323 ) ;
#5381=CARTESIAN_POINT ( 'NONE',  ( 152.8558173410470147, 54.14978343559395313, 15.99724100256723780 ) ) ;
#5382=CARTESIAN_POINT ( 'NONE',  ( -15.32772194461970194, 8.507097118773966571, 91.57259910632232902 ) ) ;
#5387=VERTEX_POINT ( 'NONE', #64656 ) ;
#5390=CARTESIAN_POINT ( 'NONE',  ( 33.62702447824805319, 8.740302253715633185, 86.30590074997479633 ) ) ;
#5393=CARTESIAN_POINT ( 'NONE',  ( 102.8111940033034273, 25.59308899183601937, 38.15290668819717013 ) ) ;
#5396=EDGE_CURVE ( 'NONE', #8866, #12095, #27008, .T. ) ;
#5397=CARTESIAN_POINT ( 'NONE',  ( 32.67604596315971577, 7.629767358313817915, -19.60289529770304995 ) ) ;
#5398=CARTESIAN_POINT ( 'NONE',  ( 173.9405361758638264, 73.05302209498819366, -41.42269835059776284 ) ) ;
#5400=CARTESIAN_POINT ( 'NONE',  ( 93.08533330311594511, 21.72562315962721513, 33.36257394385762609 ) ) ;
#5401=ORIENTED_EDGE ( 'NONE', *, *, #14159, .F. ) ;
#5402=CARTESIAN_POINT ( 'NONE',  ( -48.71337292867760738, 14.10768470390589435, -38.70095378530758978 ) ) ;
#5407=CARTESIAN_POINT ( 'NONE',  ( -31.43908319763710679, -170.0000000000000000, -69.66174795566553257 ) ) ;
#5410=VERTEX_POINT ( 'NONE', #41821 ) ;
#5413=CARTESIAN_POINT ( 'NONE',  ( -165.9072201026428957, 80.88235209323546826, 89.92767665983485870 ) ) ;
#5414=CARTESIAN_POINT ( 'NONE',  ( -31.43908319763710679, -170.0000000000000000, -15.97264677473816974 ) ) ;
#5419=CARTESIAN_POINT ( 'NONE',  ( 151.1607415860635228, 52.90668588398089867, -74.55516125840486552 ) ) ;
#5422=CARTESIAN_POINT ( 'NONE',  ( -153.6931187576189188, 67.81270084382356345, -48.54057641887556684 ) ) ;
#5426=CARTESIAN_POINT ( 'NONE',  ( 69.48877314113910586, 15.30784187978995448, -12.58006891014075812 ) ) ;
#5427=CARTESIAN_POINT ( 'NONE',  ( -79.61235761536671873, 23.76245710489568808, -50.07082761529047588 ) ) ;
#5428=CARTESIAN_POINT ( 'NONE',  ( 117.6070629920123025, 32.44042087193796675, 89.33694317982141797 ) ) ;
#5429=CARTESIAN_POINT ( 'NONE',  ( -154.6085044440278864, 69.98390342970672862, 5.873012740166642764 ) ) ;
#5433=CARTESIAN_POINT ( 'NONE',  ( -152.2429173757935530, 67.87244971895253798, 84.90521448722901710 ) ) ;
#5434=ORIENTED_EDGE ( 'NONE', *, *, #7493, .F. ) ;
#5436=EDGE_LOOP ( 'NONE', ( #5744, #64775 ) ) ;
#5437=CARTESIAN_POINT ( 'NONE',  ( -10.23402954931276554, 7.059791383763807993, 17.87799841423737490 ) ) ;
#5438=CARTESIAN_POINT ( 'NONE',  ( -109.0191069781766657, 36.33811634972921922, 94.99999999999866418 ) ) ;
#5440=CARTESIAN_POINT ( 'NONE',  ( -153.5002794404626627, 67.64160439471096709, -21.82117646152210000 ) ) ;
#5447=DIRECTION ( 'NONE',  ( 0.000000000000000000, 0.000000000000000000, 1.000000000000000000 ) ) ;
#5449=CARTESIAN_POINT ( 'NONE',  ( 21.75684465274324353, 6.764994602232766496, 68.92719249320558106 ) ) ;
#5451=CARTESIAN_POINT ( 'NONE',  ( 9.823983574062868485, 6.382904402091121199, -74.43691175599163046 ) ) ;
#5455=CARTESIAN_POINT ( 'NONE',  ( 173.9288990958749537, 71.66475105971929338, 39.13067012050992588 ) ) ;
#5456=CARTESIAN_POINT ( 'NONE',  ( -125.8938041572051105, 46.49392987655492959, -49.91370389823397602 ) ) ;
#5458=CARTESIAN_POINT ( 'NONE',  ( 55.51637278631174155, 12.08345311280958789, -70.57488892405791603 ) ) ;
#5459=ORIENTED_EDGE ( 'NONE', *, *, #48172, .F. ) ;
#5462=CARTESIAN_POINT ( 'NONE',  ( -24.94151142167917001, 8.614613465433025752, -19.75076858682908920 ) ) ;
#5463=CARTESIAN_POINT ( 'NONE',  ( 200.4574930424076058, 102.3536505870638393, 16.06672283762458875 ) ) ;
#5467=CARTESIAN_POINT ( 'NONE',  ( 111.1767565371974626, 29.31586421952252408, 56.49927049809659252 ) ) ;
#5469=CARTESIAN_POINT ( 'NONE',  ( 116.0822834687217266, 32.80169113915575707, 68.68829875601142021 ) ) ;
#5472=CARTESIAN_POINT ( 'NONE',  ( 135.6793972494603224, 43.71805072851434204, 56.56519963210866564 ) ) ;
#5475=CARTESIAN_POINT ( 'NONE',  ( -95.86612279493098754, 29.64021615886203165, 41.91453243627326941 ) ) ;
#5477=CARTESIAN_POINT ( 'NONE',  ( 93.08533330311593090, 21.72562315962721158, -47.17107782753343770 ) ) ;
#5481=CARTESIAN_POINT ( 'NONE',  ( -125.4433371161043596, 46.19736518073187881, -8.069153307770243089 ) ) ;
#5484=CARTESIAN_POINT ( 'NONE',  ( -146.7404675333698378, 63.17262273741975065, -35.33834636302898957 ) ) ;
#5485=CARTESIAN_POINT ( 'NONE',  ( -165.6208371326873703, 80.58821715390999429, -69.35434424568703093 ) ) ;
#5486=CARTESIAN_POINT ( 'NONE',  ( -149.0782809666403637, 63.81577337591402710, -49.81283053149199702 ) ) ;
#5488=CARTESIAN_POINT ( 'NONE',  ( 59.94652978725889625, 13.01168383647461901, 17.31598363014413522 ) ) ;
#5489=EDGE_CURVE ( 'NONE', #34109, #59711, #68551, .T. ) ;
#5490=EDGE_CURVE ( 'NONE', #63292, #51274, #27269, .T. ) ;
#5494=CARTESIAN_POINT ( 'NONE',  ( 82.74007713545064746, 18.13042311233562032, -22.89437781078106582 ) ) ;
#5495=CARTESIAN_POINT ( 'NONE',  ( 86.62931800182293784, 19.42108912189599579, -62.66611478937537782 ) ) ;
#5498=CARTESIAN_POINT ( 'NONE',  ( -95.05546640093039912, 29.25972325950975517, -71.43887970864732040 ) ) ;
#5502=CARTESIAN_POINT ( 'NONE',  ( 9.290502160020464473, 6.379616279862538875, 33.76109296599172183 ) ) ;
#5506=CARTESIAN_POINT ( 'NONE',  ( 104.4006536356074122, 27.36759527624478849, -74.99636480049218790 ) ) ;
#5507=CARTESIAN_POINT ( 'NONE',  ( -72.78270026377325053, 21.23376443558121096, -64.78274740210713389 ) ) ;
#5509=CARTESIAN_POINT ( 'NONE',  ( -119.5404913382140109, 43.63271406506962080, 34.12591518711677452 ) ) ;
#5512=CARTESIAN_POINT ( 'NONE',  ( -109.7647482398635503, 36.74843029291200480, -15.12249450503182935 ) ) ;
#5514=CARTESIAN_POINT ( 'NONE',  ( -14.32241591711282247, 7.401556312061832621, -39.16318076575544893 ) ) ;
#5515=CARTESIAN_POINT ( 'NONE',  ( -84.79701208522806155, 24.75216251823110269, 87.27508272618359797 ) ) ;
#5517=CARTESIAN_POINT ( 'NONE',  ( 149.9552318559267121, 52.03645904563055780, -16.75648080528598172 ) ) ;
#5518=CARTESIAN_POINT ( 'NONE',  ( 32.03384598935271299, 8.576372641735996893, 12.03241481110506328 ) ) ;
#5520=CARTESIAN_POINT ( 'NONE',  ( -95.52093927227217307, 30.58993121475388577, -66.09890349134650478 ) ) ;
#5523=VERTEX_POINT ( 'NONE', #49490 ) ;
#5529=CARTESIAN_POINT ( 'NONE',  ( 12.46490660984525789, 7.423426948220651411, -63.13552371036534794 ) ) ;
#5531=CARTESIAN_POINT ( 'NONE',  ( 45.35146934743634972, 10.27620685439441850, -65.37128321836291889 ) ) ;
#5534=CARTESIAN_POINT ( 'NONE',  ( 94.12422088577032753, 23.19200960350636365, 90.45949129094441332 ) ) ;
#5536=EDGE_LOOP ( 'NONE', ( #5362, #49166, #56506, #37143 ) ) ;
#5539=CARTESIAN_POINT ( 'NONE',  ( -129.6165111262477296, 48.99406349865701316, 4.760252937733464584 ) ) ;
#5540=CARTESIAN_POINT ( 'NONE',  ( -105.8879245385188739, 35.79035667534147791, 71.45643182967125995 ) ) ;
#5541=CARTESIAN_POINT ( 'NONE',  ( -179.9997297618090784, 95.12611598520665268, 94.99999999999866418 ) ) ;
#5542=ORIENTED_EDGE ( 'NONE', *, *, #16575, .T. ) ;
#5543=CYLINDRICAL_SURFACE ( 'NONE', #36905, 7.500000000000013323 ) ;
#5544=CARTESIAN_POINT ( 'NONE',  ( -3.868882431147342871, 6.665575841812233726, -22.44979996978308634 ) ) ;
#5546=CARTESIAN_POINT ( 'NONE',  ( -156.8280449791103877, 70.64611012537017132, 90.24344703734034567 ) ) ;
#5549=CARTESIAN_POINT ( 'NONE',  ( 139.7928618793172859, 45.12615179300589574, 41.60106151571937261 ) ) ;
#5553=CARTESIAN_POINT ( 'NONE',  ( 82.12277968641507186, 18.98848723477813394, 16.38247655469762520 ) ) ;
#5556=EDGE_LOOP ( 'NONE', ( #119, #63196, #51370, #42776 ) ) ;
#5559=CARTESIAN_POINT ( 'NONE',  ( -109.0297561673456386, 36.34391931706015555, -39.23453111580145958 ) ) ;
#5560=CARTESIAN_POINT ( 'NONE',  ( 70.50372867914784081, 14.53505678900968867, -69.57474953973002130 ) ) ;
#5561=CARTESIAN_POINT ( 'NONE',  ( -58.76005811686688673, 15.70653557534867595, 44.35498545959168837 ) ) ;
#5562=CIRCLE ( 'NONE', #21286, 242.4895526022646379 ) ;
#5565=CARTESIAN_POINT ( 'NONE',  ( 158.3604774538084712, 58.34594647925810307, 44.36981973328110485 ) ) ;
#5566=LINE ( 'NONE', #11886, #48501 ) ;
#5569=AXIS2_PLACEMENT_3D ( 'NONE', #8247, #67349, #57472 ) ;
#5570=DIRECTION ( 'NONE',  ( -0.000000000000000000, 1.000000000000000000, -0.000000000000000000 ) ) ;
#5572=EDGE_CURVE ( 'NONE', #49668, #69259, #2134, .T. ) ;
#5573=CARTESIAN_POINT ( 'NONE',  ( -142.1451960690342560, 59.45765244009941597, -94.47710424355705072 ) ) ;
#5575=CARTESIAN_POINT ( 'NONE',  ( -172.7116702014380110, 86.67317892691259829, 45.82169460664105287 ) ) ;
#5576=CARTESIAN_POINT ( 'NONE',  ( 126.7877523219523823, 38.47018873135926498, 66.41478141192939688 ) ) ;
#5577=ORIENTED_EDGE ( 'NONE', *, *, #19439, .F. ) ;
#5581=CARTESIAN_POINT ( 'NONE',  ( -107.7677210873465583, 36.80113675102404613, 6.039296874237338741 ) ) ;
#5583=CARTESIAN_POINT ( 'NONE',  ( -109.6894192603215998, 36.70681195612597492, 90.49915744604948031 ) ) ;
#5585=CARTESIAN_POINT ( 'NONE',  ( -7.825402957745087207, 6.891034867348159842, -35.41807073194381417 ) ) ;
#5589=ORIENTED_EDGE ( 'NONE', *, *, #45424, .T. ) ;
#5590=FACE_OUTER_BOUND ( 'NONE', #17343, .T. ) ;
#5591=CARTESIAN_POINT ( 'NONE',  ( 210.0292194063021896, 113.9511645670926185, -65.39028459387030523 ) ) ;
#5595=CYLINDRICAL_SURFACE ( 'NONE', #50220, 7.500000000000013323 ) ;
#5599=ORIENTED_EDGE ( 'NONE', *, *, #35041, .T. ) ;
#5601=DIRECTION ( 'NONE',  ( 0.000000000000000000, 0.000000000000000000, 1.000000000000000000 ) ) ;
#5604=CARTESIAN_POINT ( 'NONE',  ( -27.70185240367227308, 10.02491413133431486, -76.16892411189579093 ) ) ;
#5605=CARTESIAN_POINT ( 'NONE',  ( 58.09607305250595033, 11.58497620657515981, -48.90344441354543648 ) ) ;
#5606=DIRECTION ( 'NONE',  ( -0.000000000000000000, 1.000000000000000000, -0.000000000000000000 ) ) ;
#5611=B_SPLINE_CURVE_WITH_KNOTS ( 'NONE', 3,
 ( #17562, #55188, #40404, #49911, #61851, #35130, #34104, #28824, #66469, #18260, #13001, #42133, #15406, #25282, #57285, #19292, #46721, #41453, #10122, #24597, #19643, #40749, #3815, #4504, #15061, #46029, #9787, #63252, #36172, #20330, #68194, #62206, #14022, #9099, #36515, #36864, #57631, #31249, #58305, #9441, #25965, #68525, #30897, #3470, #63597 ),
 .UNSPECIFIED., .F., .F.,
 ( 4, 2, 2, 2, 2, 2, 2, 2, 1, 2, 2, 2, 2, 2, 2, 2, 2, 2, 2, 2, 2, 2, 4 ),
 ( 1.734723475976807094E-18, 0.001467747071934227387, 0.002201620607901337828, 0.002935494143868448268, 0.004403241215802658308, 0.005870988287736867914, 0.007338735359671077520, 0.008072608895638166276, 0.008806482431605255901, 0.009540355967572345525, 0.01027422950353943515, 0.01174197657547365430, 0.01247585011144078382, 0.01320972364740791508, 0.01467747071934213422, 0.01541134425530924466, 0.01614521779127635337, 0.01761296486321053956, 0.01908071193514472574, 0.01981458547111182578, 0.02054845900707892581, 0.02201620607901315363, 0.02348395315094737451 ),
 .UNSPECIFIED. ) ;
#5612=VECTOR ( 'NONE', #45632, 1000.000000000000000 ) ;
#5613=CARTESIAN_POINT ( 'NONE',  ( -128.9843070188472325, 49.78011598923033887, 31.27109394439055734 ) ) ;
#5615=CARTESIAN_POINT ( 'NONE',  ( 205.1049299651095055, 106.9023875785545954, 17.36317014830576966 ) ) ;
#5617=CARTESIAN_POINT ( 'NONE',  ( 58.09607305250594322, 11.58497620657515803, 58.47475794830932472 ) ) ;
#5621=DIRECTION ( 'NONE',  ( -0.000000000000000000, 1.000000000000000000, -0.000000000000000000 ) ) ;
#5623=CARTESIAN_POINT ( 'NONE',  ( -149.5074843970971017, 65.50121172469319220, 3.876270649435370252 ) ) ;
#5624=EDGE_LOOP ( 'NONE', ( #24042, #23283 ) ) ;
#5626=VERTEX_POINT ( 'NONE', #67105 ) ;
#5627=DIRECTION ( 'NONE',  ( 0.000000000000000000, 0.000000000000000000, 1.000000000000000000 ) ) ;
#5628=DIRECTION ( 'NONE',  ( -1.000000000000000000, 0.000000000000000000, 0.000000000000000000 ) ) ;
#5631=CARTESIAN_POINT ( 'NONE',  ( 68.95451040317568925, 14.12887482153123742, 41.91971055821581871 ) ) ;
#5633=CARTESIAN_POINT ( 'NONE',  ( 19.27211902843862035, 7.644382812444131758, 84.55400850847075844 ) ) ;
#5638=CARTESIAN_POINT ( 'NONE',  ( -76.77329340382468104, 21.60914066444074422, 45.19114480031347370 ) ) ;
#5644=ORIENTED_EDGE ( 'NONE', *, *, #6081, .T. ) ;
#5646=DIRECTION ( 'NONE',  ( 0.000000000000000000, 0.000000000000000000, 1.000000000000000000 ) ) ;
#5647=CARTESIAN_POINT ( 'NONE',  ( 69.35866309798977625, 15.27376159675663203, 41.32255262261386264 ) ) ;
#5650=CARTESIAN_POINT ( 'NONE',  ( -173.1211646369891355, -170.0000000000000000, -7.867406574286299303 ) ) ;
#5651=CARTESIAN_POINT ( 'NONE',  ( -29.04258984626623530, 9.210213971636683539, 30.60543872389602171 ) ) ;
#5652=CARTESIAN_POINT ( 'NONE',  ( -146.5230751932349165, 62.99205605665035534, -76.05256278801076064 ) ) ;
#5653=VERTEX_POINT ( 'NONE', #15687 ) ;
#5655=FACE_BOUND ( 'NONE', #7861, .T. ) ;
#5656=CARTESIAN_POINT ( 'NONE',  ( -0.5780275525703881812, 6.527356703336900878, -71.70849423231535980 ) ) ;
#5657=CARTESIAN_POINT ( 'NONE',  ( -180.6158171975815776, 97.47361786002630879, 64.84187048422768385 ) ) ;
#5660=CARTESIAN_POINT ( 'NONE',  ( -81.00768240531205322, 24.30850321514432366, 3.944436707959213084 ) ) ;
#5664=CARTESIAN_POINT ( 'NONE',  ( 66.72974708835174340, 13.56459745268606376, 3.934091007171761412 ) ) ;
#5665=CARTESIAN_POINT ( 'NONE',  ( -83.53167274806556009, 25.32068190668985608, 70.49144734754210617 ) ) ;
#5666=CARTESIAN_POINT ( 'NONE',  ( 87.59078297315399197, 20.81577753000345155, -23.93050775134987163 ) ) ;
#5668=CARTESIAN_POINT ( 'NONE',  ( -37.39246151129641760, 11.66872370876247800, 15.45975854931544546 ) ) ;
#5671=EDGE_LOOP ( 'NONE', ( #40192, #35934, #36153, #9226 ) ) ;
#5672=CARTESIAN_POINT ( 'NONE',  ( 79.54836217416615796, 18.17815803851260625, -72.65076421043085020 ) ) ;
#5673=CARTESIAN_POINT ( 'NONE',  ( 105.4784409469015003, 27.83725412974951396, 84.96893711368112179 ) ) ;
#5674=CARTESIAN_POINT ( 'NONE',  ( -142.9756886485677398, 60.11539876121631210, 61.37017874365231052 ) ) ;
#5675=CARTESIAN_POINT ( 'NONE',  ( 66.30567821786759453, 13.45988234822861429, -9.631894463744744783 ) ) ;
#5680=CARTESIAN_POINT ( 'NONE',  ( -52.68206656346369243, 15.09776187114412593, -62.44128804069127625 ) ) ;
#5687=CARTESIAN_POINT ( 'NONE',  ( 39.40195752203892710, 9.424259417798131366, 56.75838489642694640 ) ) ;
#5691=CARTESIAN_POINT ( 'NONE',  ( 133.1078597672272394, 42.14624897798367442, -89.71241211332299770 ) ) ;
#5694=CARTESIAN_POINT ( 'NONE',  ( 63.83262973450582223, 13.89724595143439245, -89.44344974266579129 ) ) ;
#5695=ORIENTED_EDGE ( 'NONE', *, *, #26987, .T. ) ;
#5696=CARTESIAN_POINT ( 'NONE',  ( 87.11239765416381431, 20.65008247340817604, 17.86753698201565399 ) ) ;
#5697=CARTESIAN_POINT ( 'NONE',  ( -8.320652113663527416, 6.923290556636831461, 71.96013162991091860 ) ) ;
#5698=CARTESIAN_POINT ( 'NONE',  ( 211.3710169359754047, 117.8057917113659698, 6.428924886512843884 ) ) ;
#5700=DIRECTION ( 'NONE',  ( 0.000000000000000000, 0.000000000000000000, 1.000000000000000000 ) ) ;
#5706=VERTEX_POINT ( 'NONE', #32217 ) ;
#5708=FACE_OUTER_BOUND ( 'NONE', #25869, .T. ) ;
#5709=CARTESIAN_POINT ( 'NONE',  ( 88.98064924903394513, 21.30386569031177046, -36.19564593720401291 ) ) ;
#5710=B_SPLINE_CURVE_WITH_KNOTS ( 'NONE', 3,
 ( #45960, #58478, #57808, #40335, #4676, #68695, #9628, #31086, #56167, #41971, #2710, #52526, #7984, #29436, #3062, #15245, #45616, #61782, #47239, #24523, #8338, #13605, #35062, #29782, #68370, #36706, #58152, #9969, #31421, #52852, #22246, #21540, #10638, #48599, #48259, #33513, #59512, #38780 ),
 .UNSPECIFIED., .F., .F.,
 ( 4, 2, 2, 2, 2, 2, 2, 2, 2, 2, 2, 2, 2, 2, 2, 2, 2, 2, 4 ),
 ( 0.02546424207107604240, 0.02703543426729210220, 0.02782103036540016852, 0.02860662646350823485, 0.03017781865972442995, 0.03174901085594063199, 0.03332020305215682709, 0.03489139524837302220, 0.03646258744458922424, 0.03724818354269731485, 0.03803377964080539853, 0.03881937573891348914, 0.03960497183702157975, 0.04117616403323776098, 0.04274735622945394914, 0.04431854842567013730, 0.04588974062188632547, 0.04746093281810251363, 0.05060331721053488302 ),
 .UNSPECIFIED. ) ;
#5713=LINE ( 'NONE', #48956, #45316 ) ;
#5714=CARTESIAN_POINT ( 'NONE',  ( -149.5074843970971301, -170.0000000000000000, -42.31283053149197571 ) ) ;
#5716=CARTESIAN_POINT ( 'NONE',  ( 60.63507185982729197, 12.13307030573223955, 17.58473668013007796 ) ) ;
#5717=CARTESIAN_POINT ( 'NONE',  ( -55.53469534616548486, 14.81076603075806197, 57.16187836339482686 ) ) ;
#5720=CARTESIAN_POINT ( 'NONE',  ( 46.15699773797793881, 10.40307558352962580, 94.42940818875426601 ) ) ;
#5722=CARTESIAN_POINT ( 'NONE',  ( 106.0171289417044136, 26.97542621030656207, 43.31196261650080714 ) ) ;
#5724=CARTESIAN_POINT ( 'NONE',  ( -62.54085973597663184, 16.81797209566546059, -70.05212444181948683 ) ) ;
#5726=CARTESIAN_POINT ( 'NONE',  ( 32.15641333221389431, 7.577415570152253643, -14.32268503797624604 ) ) ;
#5727=CARTESIAN_POINT ( 'NONE',  ( 173.6737675136087091, 72.80308721038093722, -44.91943839559014151 ) ) ;
#5734=CARTESIAN_POINT ( 'NONE',  ( -47.80251179448167420, 13.89045662648308976, -40.73231631372835437 ) ) ;
#5736=CARTESIAN_POINT ( 'NONE',  ( 12.03162622199372933, 7.415834979634796653, 44.01070327993329556 ) ) ;
#5739=DIRECTION ( 'NONE',  ( 0.000000000000000000, 0.000000000000000000, 1.000000000000000000 ) ) ;
#5744=ORIENTED_EDGE ( 'NONE', *, *, #30818, .T. ) ;
#5745=CARTESIAN_POINT ( 'NONE',  ( -14.55390976651257162, 7.422979442794209959, -19.39586497985030888 ) ) ;
#5746=CARTESIAN_POINT ( 'NONE',  ( -172.7861182744952941, 88.26094898553817814, 84.50184874253974954 ) ) ;
#5749=CARTESIAN_POINT ( 'NONE',  ( -56.96436614829624290, 16.24647150911285820, -49.97265642726394219 ) ) ;
#5750=CARTESIAN_POINT ( 'NONE',  ( -14.33576511807126685, 8.413127487936186810, -12.31783428727917951 ) ) ;
#5751=CARTESIAN_POINT ( 'NONE',  ( 156.5909039492010209, 56.96742803863248383, -62.96873488960130771 ) ) ;
#5752=CARTESIAN_POINT ( 'NONE',  ( 23.03864809957654458, 6.841061756139156458, -14.23981446476811108 ) ) ;
#5754=CARTESIAN_POINT ( 'NONE',  ( -156.1462053606562392, 70.02140399657012892, -38.81290798880835524 ) ) ;
#5756=ORIENTED_EDGE ( 'NONE', *, *, #23587, .T. ) ;
#5760=CARTESIAN_POINT ( 'NONE',  ( -149.7268278745401631, 65.68859631971236013, 3.876270649435373361 ) ) ;
#5763=CARTESIAN_POINT ( 'NONE',  ( 22.52576749827963809, 6.809805260274345073, 34.18343812378846280 ) ) ;
#5764=CARTESIAN_POINT ( 'NONE',  ( -156.8955115693747757, 72.07810529072631311, 90.57258849307295634 ) ) ;
#5767=EDGE_CURVE ( 'NONE', #59702, #34459, #42070, .T. ) ;
#5769=CARTESIAN_POINT ( 'NONE',  ( -154.7826623253030505, 70.14150242829521176, -20.80520620324490366 ) ) ;
#5775=CARTESIAN_POINT ( 'NONE',  ( -31.93184248720558216, 9.672312402099825235, 72.06100499665288339 ) ) ;
#5776=CARTESIAN_POINT ( 'NONE',  ( -155.1355020251929488, 69.10372769512068203, -20.45101316398983116 ) ) ;
#5777=ORIENTED_EDGE ( 'NONE', *, *, #40759, .F. ) ;
#5778=CARTESIAN_POINT ( 'NONE',  ( 188.4365915667139006, 87.87248959723056885, 65.16220424045542359 ) ) ;
#5779=CARTESIAN_POINT ( 'NONE',  ( -156.4841188516943191, 70.33041971808555104, 62.29890658327479258 ) ) ;
#5780=VECTOR ( 'NONE', #26931, 1000.000000000000000 ) ;
#5784=CARTESIAN_POINT ( 'NONE',  ( -83.51052366780668024, 24.22613130369187218, -36.88447773562854337 ) ) ;
#5785=CARTESIAN_POINT ( 'NONE',  ( 23.03578842369135060, 6.840884649289439068, 62.41390671365888210 ) ) ;
#5787=CARTESIAN_POINT ( 'NONE',  ( 8.000000000000007105, 249.8719672152120381, -95.00000000000133582 ) ) ;
#5794=CARTESIAN_POINT ( 'NONE',  ( 174.6176230994777825, 72.30829341023250834, 40.64789474444607009 ) ) ;
#5795=CARTESIAN_POINT ( 'NONE',  ( -132.2199390322348904, 50.80243550247269013, -38.35397204430816487 ) ) ;
#5796=CARTESIAN_POINT ( 'NONE',  ( 39.40195752203892710, 8.409560354027393103, -62.46436805589144114 ) ) ;
#5797=CARTESIAN_POINT ( 'NONE',  ( 164.6046919270428930, -170.0000000000000000, -95.00000000000133582 ) ) ;
#5800=CARTESIAN_POINT ( 'NONE',  ( -25.81763596640060143, 8.735969132042855634, -20.94358112585581821 ) ) ;
#5801=CARTESIAN_POINT ( 'NONE',  ( 174.0956405974778534, 71.82022412301054715, 93.22721250497485812 ) ) ;
#5804=CARTESIAN_POINT ( 'NONE',  ( 184.9757174666826813, 84.09845285279330085, 30.39345074774602651 ) ) ;
#5808=CARTESIAN_POINT ( 'NONE',  ( 103.6830219322541353, 27.05818465022135655, -93.45235881085721985 ) ) ;
#5809=CARTESIAN_POINT ( 'NONE',  ( 134.7708899521910837, 43.15864772107689618, 56.40727709478612439 ) ) ;
#5810=CARTESIAN_POINT ( 'NONE',  ( -73.09185868250601459, 20.27574131633382493, -37.57414808074971546 ) ) ;
#5811=CARTESIAN_POINT ( 'NONE',  ( 83.53262254759448524, 18.38732384439404655, -90.16803647247536446 ) ) ;
#5812=CARTESIAN_POINT ( 'NONE',  ( 94.06703982324147262, 22.09435144471462920, -42.32417742623751167 ) ) ;
#5818=CARTESIAN_POINT ( 'NONE',  ( -142.9843132609582597, 60.12226089556227748, -38.60248188077854081 ) ) ;
#5819=CARTESIAN_POINT ( 'NONE',  ( -168.0052514572427356, 83.06849406765627464, -63.56670774126097001 ) ) ;
#5822=CARTESIAN_POINT ( 'NONE',  ( 59.08202327466405279, 12.82375733818953734, 16.85878258424966702 ) ) ;
#5825=FACE_OUTER_BOUND ( 'NONE', #5988, .T. ) ;
#5827=FACE_OUTER_BOUND ( 'NONE', #21085, .T. ) ;
#5831=CARTESIAN_POINT ( 'NONE',  ( 136.3292018078239778, 42.93753790426541883, -23.76329299397318096 ) ) ;
#5833=FACE_OUTER_BOUND ( 'NONE', #31509, .T. ) ;
#5834=CARTESIAN_POINT ( 'NONE',  ( -96.78198318406110445, 30.07417864442859212, 6.050221078145685105 ) ) ;
#5835=CARTESIAN_POINT ( 'NONE',  ( -96.78198318406114709, 30.07417864442863475, -74.48343069324536714 ) ) ;
#5837=VERTEX_POINT ( 'NONE', #64212 ) ;
#5844=CARTESIAN_POINT ( 'NONE',  ( 103.9685899589048006, 27.18106603025992385, -74.38333352377321717 ) ) ;
#5845=CARTESIAN_POINT ( 'NONE',  ( 79.19345177405118363, 17.01649702043280499, 38.22266187991689179 ) ) ;
#5846=CYLINDRICAL_SURFACE ( 'NONE', #21, 7.500000000000013323 ) ;
#5847=CARTESIAN_POINT ( 'NONE',  ( 46.51377856795993182, 10.46037936279324754, -40.68832589467017158 ) ) ;
#5849=ORIENTED_EDGE ( 'NONE', *, *, #61635, .F. ) ;
#5850=CARTESIAN_POINT ( 'NONE',  ( -31.43908319763711390, 10.61114334766715928, 18.37190381572551701 ) ) ;
#5853=CARTESIAN_POINT ( 'NONE',  ( -12.77647591501652613, 7.263973827022342178, -48.57332611465309924 ) ) ;
#5854=DIRECTION ( 'NONE',  ( 0.000000000000000000, 0.000000000000000000, 1.000000000000000000 ) ) ;
#5855=CARTESIAN_POINT ( 'NONE',  ( 88.98064924903393091, 21.30386569031177402, 71.18255642465075539 ) ) ;
#5856=CARTESIAN_POINT ( 'NONE',  ( 157.4703587214989113, 57.65129005721575339, -24.27963370867398396 ) ) ;
#5858=CARTESIAN_POINT ( 'NONE',  ( -99.98584758882481083, 32.75338129098887663, -76.51518145783863645 ) ) ;
#5859=EDGE_CURVE ( 'NONE', #1836, #10264, #48023, .T. ) ;
#5860=CARTESIAN_POINT ( 'NONE',  ( 114.9572297719016092, 32.24508028227645440, -91.26492051213512013 ) ) ;
#5869=CARTESIAN_POINT ( 'NONE',  ( -0.5751131641471373124, 6.527254166626918597, 39.55046635746396788 ) ) ;
#5870=CARTESIAN_POINT ( 'NONE',  ( -106.6781182590523258, 35.07133425426472684, -63.26553636263061975 ) ) ;
#5874=CARTESIAN_POINT ( 'NONE',  ( -190.6985136298601731, 109.1272424661242582, -19.71767969763411799 ) ) ;
#5877=CARTESIAN_POINT ( 'NONE',  ( -166.2065256787326746, 81.19093426984588291, -39.29294834308091566 ) ) ;
#5879=ORIENTED_EDGE ( 'NONE', *, *, #50038, .T. ) ;
#5880=LINE ( 'NONE', #58315, #33558 ) ;
#5881=VECTOR ( 'NONE', #1006, 1000.000000000000000 ) ;
#5883=CARTESIAN_POINT ( 'NONE',  ( 197.3119541548905715, 98.33923235143191732, -18.29545015563770960 ) ) ;
#5885=CARTESIAN_POINT ( 'NONE',  ( -156.1201442861361386, 69.99755458545364206, 88.35662595570710209 ) ) ;
#5889=CARTESIAN_POINT ( 'NONE',  ( 79.63513233364427890, 18.20496177163925111, 7.648485935142918635 ) ) ;
#5892=ORIENTED_EDGE ( 'NONE', *, *, #10677, .T. ) ;
#5893=CARTESIAN_POINT ( 'NONE',  ( 177.0027897064244087, 75.97676392242543386, 69.96163413657492924 ) ) ;
#5896=CARTESIAN_POINT ( 'NONE',  ( -71.96390573417174608, 19.88067451234326555, -12.36759105974787154 ) ) ;
#5897=CARTESIAN_POINT ( 'NONE',  ( 204.6977192012829789, -170.0000000000000000, 29.20772073876942088 ) ) ;
#5898=CARTESIAN_POINT ( 'NONE',  ( 154.6530827109543225, 56.75509330623210502, 17.01932198663618223 ) ) ;
#5899=ORIENTED_EDGE ( 'NONE', *, *, #35205, .T. ) ;
#5900=CARTESIAN_POINT ( 'NONE',  ( 163.7607557204680404, 62.71181783708028235, 41.02505403109415028 ) ) ;
#5905=CARTESIAN_POINT ( 'NONE',  ( -148.7135390649993667, 64.82294617398349601, -88.50193171241927814 ) ) ;
#5907=CARTESIAN_POINT ( 'NONE',  ( -34.51918258780365534, 10.11719938103014726, -22.81536398408823274 ) ) ;
#5908=CARTESIAN_POINT ( 'NONE',  ( -179.5109681715918555, 96.11572638569522553, 34.35669452023326187 ) ) ;
#5909=CARTESIAN_POINT ( 'NONE',  ( -38.84150381976581201, 10.92416363971239157, -70.89272716398475893 ) ) ;
#5910=VERTEX_POINT ( 'NONE', #26248 ) ;
#5914=CARTESIAN_POINT ( 'NONE',  ( -49.44946307590714696, 13.25037070100582426, 86.51077810379730693 ) ) ;
#5917=CARTESIAN_POINT ( 'NONE',  ( -156.9252506979472628, 70.73559306219776488, -70.30158766110032786 ) ) ;
#5920=EDGE_CURVE ( 'NONE', #23284, #45155, #59903, .T. ) ;
#5924=EDGE_CURVE ( 'NONE', #6748, #46944, #15146, .T. ) ;
#5929=CARTESIAN_POINT ( 'NONE',  ( 63.01563776193091826, -170.0000000000000000, 10.46841034875760279 ) ) ;
#5930=CARTESIAN_POINT ( 'NONE',  ( 186.2651679807462131, 84.00458780104314371, 31.36535250390706153 ) ) ;
#5933=CARTESIAN_POINT ( 'NONE',  ( -71.22878586122430988, 19.62649588091172248, 12.07173733644329516 ) ) ;
#5938=LINE ( 'NONE', #15816, #48381 ) ;
#5943=CYLINDRICAL_SURFACE ( 'NONE', #44202, 7.500000000000013323 ) ;
#5946=CARTESIAN_POINT ( 'NONE',  ( -84.96580414052107244, 24.82184094495578464, 41.99606300715279872 ) ) ;
#5950=B_SPLINE_CURVE_WITH_KNOTS ( 'NONE', 3,
 ( #17168, #10861, #27378, #60082, #11902, #59040, #33382, #28077, #60445, #12262, #48136, #32330, #53758, #5581, #30435, #8988, #66093, #60785, #46602, #17886, #46957, #52230, #49883, #30098, #62449, #45921, #1707, #67389, #14263, #51206, #68419, #57173, #39342, #63137, #56832, #12608, #44613, #8645, #51883, #35370, #51553, #19531, #30786, #25520 ),
 .UNSPECIFIED., .F., .F.,
 ( 4, 2, 2, 2, 2, 2, 2, 2, 2, 2, 2, 2, 2, 2, 2, 2, 2, 2, 2, 2, 2, 4 ),
 ( 0.02477387709520257816, 0.02633314402883776828, 0.02711277749565536160, 0.02789241096247295146, 0.02945167789610816933, 0.03023131136292576265, 0.03101094482974335598, 0.03257021176337854262, 0.03334984523019612207, 0.03412947869701370152, 0.03568874563064885347, 0.03646837909746643291, 0.03724801256428400542, 0.03802764603110158487, 0.03880727949791916431, 0.04036654643155432320, 0.04192581336518948210, 0.04348508029882463405, 0.04504434723245979988, 0.04660361416609495183, 0.04816288109973011766, 0.04972214803336526961 ),
 .UNSPECIFIED. ) ;
#5951=CARTESIAN_POINT ( 'NONE',  ( 133.8566784816069628, 41.42467568809809819, -9.178760341931967659 ) ) ;
#5954=VERTEX_POINT ( 'NONE', #64566 ) ;
#5956=ADVANCED_FACE ( 'NONE', ( #64918 ), #16713, .F. ) ;
#5959=CARTESIAN_POINT ( 'NONE',  ( 36.09469435220862010, 9.015003538710468334, -23.02428657931588063 ) ) ;
#5960=CARTESIAN_POINT ( 'NONE',  ( -149.0764453401867513, 65.13297611514538232, 30.72082123989904545 ) ) ;
#5962=CARTESIAN_POINT ( 'NONE',  ( -0.8863172752569253854, 7.545240277686255048, 67.33728230589369446 ) ) ;
#5963=CARTESIAN_POINT ( 'NONE',  ( -28.14339584226772928, 10.09086145081589159, -89.75580143143783118 ) ) ;
#5968=ORIENTED_EDGE ( 'NONE', *, *, #49778, .T. ) ;
#5969=CARTESIAN_POINT ( 'NONE',  ( 63.01563776193091826, -170.0000000000000000, -43.22069083216975116 ) ) ;
#5972=CARTESIAN_POINT ( 'NONE',  ( -169.8791831685530838, 83.59058982490282119, -8.589682762458334508 ) ) ;
#5973=CARTESIAN_POINT ( 'NONE',  ( 140.4586216751744701, 45.55624550472996503, -73.93575597659268794 ) ) ;
#5974=CARTESIAN_POINT ( 'NONE',  ( 70.51484748609223630, 14.53801151001411718, 36.80098285481733456 ) ) ;
#5980=CARTESIAN_POINT ( 'NONE',  ( -71.43874587651170316, 19.69883891272894516, 35.89975146121849292 ) ) ;
#5986=CARTESIAN_POINT ( 'NONE',  ( 92.53566308513174477, 21.52138666710686365, 15.01619406867864903 ) ) ;
#5988=EDGE_LOOP ( 'NONE', ( #52983, #7010, #65966, #3563 ) ) ;
#5992=CARTESIAN_POINT ( 'NONE',  ( 152.1190604254710195, 53.60705199010335065, 31.64870937947464924 ) ) ;
#5993=CARTESIAN_POINT ( 'NONE',  ( -180.3161328724957571, 97.10341277064809162, -40.07322758584183475 ) ) ;
#5996=PLANE ( 'NONE',  #19250 ) ;
#5998=CARTESIAN_POINT ( 'NONE',  ( 135.6793972494602656, 43.71805072851428520, -77.65755332020975743 ) ) ;
#6000=ORIENTED_EDGE ( 'NONE', *, *, #47399, .F. ) ;
#6001=FACE_BOUND ( 'NONE', #25507, .T. ) ;
#6002=CARTESIAN_POINT ( 'NONE',  ( -5.416136198635858712, 6.745992685878683837, -76.86935474192905815 ) ) ;
#6003=CARTESIAN_POINT ( 'NONE',  ( -180.6021503146988607, 97.45669259943417728, 65.78653073592644773 ) ) ;
#6005=CARTESIAN_POINT ( 'NONE',  ( -120.0051930351106648, 43.92079660368833061, -37.76205108401183708 ) ) ;
#6006=CARTESIAN_POINT ( 'NONE',  ( -81.01931326044685022, 24.31309346877660005, 18.19902748808744875 ) ) ;
#6008=CARTESIAN_POINT ( 'NONE',  ( -149.5074843970971017, 64.17983161892348676, 3.876270649435373361 ) ) ;
#6009=EDGE_CURVE ( 'NONE', #21211, #2336, #24787, .T. ) ;
#6010=CARTESIAN_POINT ( 'NONE',  ( -120.1346137380982384, 44.00127440773567855, -74.06905664438973247 ) ) ;
#6011=CARTESIAN_POINT ( 'NONE',  ( 67.56108154898468854, 13.77276756375644595, 16.45415915286800157 ) ) ;
#6012=CARTESIAN_POINT ( 'NONE',  ( 164.8942204024298235, 63.66138186734712434, 11.16733468916308247 ) ) ;
#6013=CARTESIAN_POINT ( 'NONE',  ( 93.72059824125564376, 23.03897520779757357, -13.98440811075808377 ) ) ;
#6016=CARTESIAN_POINT ( 'NONE',  ( -33.83721310978698682, 11.01869210665940635, 3.761447440691132904 ) ) ;
#6020=CARTESIAN_POINT ( 'NONE',  ( 79.12879321038293767, 18.04902206524926811, -69.93020897591220830 ) ) ;
#6021=CARTESIAN_POINT ( 'NONE',  ( 112.7929653408798174, 31.19474750060521728, 83.73979164330758351 ) ) ;
#6022=CARTESIAN_POINT ( 'NONE',  ( -142.0070007485041401, 59.34878529741516928, 64.79586851560435434 ) ) ;
#6024=CARTESIAN_POINT ( 'NONE',  ( -29.04400972079232446, 10.22852224114065045, -35.70569127779752705 ) ) ;
#6025=CARTESIAN_POINT ( 'NONE',  ( -49.44484229820456989, 14.28460989390480051, -64.55669302136469412 ) ) ;
#6033=CARTESIAN_POINT ( 'NONE',  ( 33.75794032130629319, 8.754084575552406378, 69.22175981326891758 ) ) ;
#6034=CARTESIAN_POINT ( 'NONE',  ( -166.2065256787326746, 81.19093426984591133, 68.08525401877383842 ) ) ;
#6036=CARTESIAN_POINT ( 'NONE',  ( -167.0073208999199323, 82.02183861952775601, -19.71965070342400494 ) ) ;
#6039=ORIENTED_EDGE ( 'NONE', *, *, #52098, .T. ) ;
#6042=CARTESIAN_POINT ( 'NONE',  ( -8.807541152391518580, 6.956521193351525412, 71.91155975037588632 ) ) ;
#6045=CARTESIAN_POINT ( 'NONE',  ( 86.62931800182293784, -170.0000000000000000, -16.47701360844803986 ) ) ;
#6046=CARTESIAN_POINT ( 'NONE',  ( 46.85206196242844356, 9.495795933269466360, -17.26884272364058504 ) ) ;
#6047=CARTESIAN_POINT ( 'NONE',  ( 210.9506883977752807, 115.3310071214937693, -21.13087597562173414 ) ) ;
#6048=DIRECTION ( 'NONE',  ( -0.000000000000000000, 1.000000000000000000, -0.000000000000000000 ) ) ;
#6050=CARTESIAN_POINT ( 'NONE',  ( 162.8034185388970343, 63.22443559329414597, 58.45892248144684089 ) ) ;
#6054=CARTESIAN_POINT ( 'NONE',  ( -54.08488990389049178, 15.46443908526321742, 57.20895787309505920 ) ) ;
#6057=CARTESIAN_POINT ( 'NONE',  ( -13.55164437043334402, 8.341947975718044361, 86.45009797131527307 ) ) ;
#6062=ORIENTED_EDGE ( 'NONE', *, *, #9927, .F. ) ;
#6065=CARTESIAN_POINT ( 'NONE',  ( -55.05276343752910151, -170.0000000000000000, -62.06087458892354647 ) ) ;
#6066=CARTESIAN_POINT ( 'NONE',  ( 102.7551177910568470, 25.56939188780864214, 36.61368049026674498 ) ) ;
#6068=CARTESIAN_POINT ( 'NONE',  ( 63.01563776193090405, 13.70579113808098271, 71.65751152968501003 ) ) ;
#6070=CARTESIAN_POINT ( 'NONE',  ( 37.46254810722765427, 8.164772623042710009, -23.53660314867922665 ) ) ;
#6071=CARTESIAN_POINT ( 'NONE',  ( 164.1338586910086406, 64.33646242148856231, 40.36181753565011121 ) ) ;
#6072=CARTESIAN_POINT ( 'NONE',  ( 109.7782172510783596, 29.77507867835876709, 2.766663615273646570 ) ) ;
#6075=CARTESIAN_POINT ( 'NONE',  ( -132.6811329440527061, 52.36246882380746115, 94.99999999999866418 ) ) ;
#6079=CARTESIAN_POINT ( 'NONE',  ( -51.34562532494749831, 14.75613283840037226, -36.17846625611093714 ) ) ;
#6080=B_SPLINE_CURVE_WITH_KNOTS ( 'NONE', 3,
 ( #39150, #34911, #24003, #12056, #2206, #23658, #6774, #29278, #60589, #55305, #2548, #45098, #13110, #18374, #28220, #49670, #1498, #8169, #39829, #44407, #61289, #22959, #7125, #50726, #40180, #56349, #28583, #1866, #23320, #52113, #3931, #4280, #68304, #41219, #40519, #62680, #8524, #19761, #41560, #19409, #20107, #25403, #63014, #3577 ),
 .UNSPECIFIED., .F., .F.,
 ( 4, 2, 2, 2, 2, 2, 2, 2, 2, 2, 2, 2, 1, 2, 2, 2, 2, 2, 2, 1, 2, 2, 4 ),
 ( 0.02381751147647563974, 0.02531129726520769604, 0.02605819015957372767, 0.02680508305393975582, 0.02829886884267181907, 0.02979265463140388231, 0.03053954752576990353, 0.03128644042013592474, 0.03278022620886795330, 0.03427401199759998879, 0.03576779778633201734, 0.03651469068069804202, 0.03726158357506405283, 0.03800847646943007058, 0.03875536936379608832, 0.04024915515252812381, 0.04174294094126016624, 0.04323672672999220867, 0.04398361962435821948, 0.04473051251872424416, 0.04547740541309025497, 0.04622429830745627966, 0.04771808409618832902 ),
 .UNSPECIFIED. ) ;
#6081=EDGE_CURVE ( 'NONE', #61817, #9471, #14712, .T. ) ;
#6084=DIRECTION ( 'NONE',  ( 0.000000000000000000, 0.000000000000000000, 1.000000000000000000 ) ) ;
#6086=CARTESIAN_POINT ( 'NONE',  ( -85.84807893108717280, 26.27917891747323864, 93.79365355873615329 ) ) ;
#6091=CARTESIAN_POINT ( 'NONE',  ( -15.31363169557738857, 7.494880774892000552, -16.56097040027614398 ) ) ;
#6092=CARTESIAN_POINT ( 'NONE',  ( -168.3977227042350364, 83.48347000932561457, 86.17750987296554399 ) ) ;
#6096=CARTESIAN_POINT ( 'NONE',  ( -38.80621507254813451, 11.94263265896520210, 66.02956010511333318 ) ) ;
#6099=CARTESIAN_POINT ( 'NONE',  ( 22.30016284075437127, 6.796348835713777348, -12.42137258383503173 ) ) ;
#6100=ORIENTED_EDGE ( 'NONE', *, *, #66117, .F. ) ;
#6110=CARTESIAN_POINT ( 'NONE',  ( -109.5025362253418706, 36.60371748273998094, 13.26117751266643197 ) ) ;
#6111=CARTESIAN_POINT ( 'NONE',  ( 18.89064107370903045, 6.619789970027398773, 44.34734594329952273 ) ) ;
#6112=CARTESIAN_POINT ( 'NONE',  ( 136.7690435008551049, 44.39743995805024923, -23.59407883755694257 ) ) ;
#6113=ORIENTED_EDGE ( 'NONE', *, *, #6819, .T. ) ;
#6116=VECTOR ( 'NONE', #38276, 1000.000000000000000 ) ;
#6118=CARTESIAN_POINT ( 'NONE',  ( -150.3850953947692517, 66.25368649589886161, -8.006832433699385021 ) ) ;
#6119=CARTESIAN_POINT ( 'NONE',  ( 31.95163392065795804, 8.568192436298499359, -44.11143406309549420 ) ) ;
#6121=DIRECTION ( 'NONE',  ( 0.000000000000000000, 0.000000000000000000, 1.000000000000000000 ) ) ;
#6123=AXIS2_PLACEMENT_3D ( 'NONE', #5017, #4669, #53879 ) ;
#6125=CARTESIAN_POINT ( 'NONE',  ( -155.1355020251929204, 69.10372769512068203, 60.08263860740119355 ) ) ;
#6127=CARTESIAN_POINT ( 'NONE',  ( 102.7435092758398127, 25.56449004647817702, 10.53745896246627467 ) ) ;
#6128=CARTESIAN_POINT ( 'NONE',  ( 86.62931800182293784, -170.0000000000000000, -97.01066537983908233 ) ) ;
#6134=CARTESIAN_POINT ( 'NONE',  ( 9.288975942802419894, 6.379608420846962780, -66.11257998586452800 ) ) ;
#6136=VECTOR ( 'NONE', #68467, 1000.000000000000000 ) ;
#6141=CARTESIAN_POINT ( 'NONE',  ( -133.3926783185152090, 51.63401075114365568, -42.11240704302350935 ) ) ;
#6153=CARTESIAN_POINT ( 'NONE',  ( 116.9197133427646804, 33.22079464767577406, 60.50180823940809915 ) ) ;
#6154=CARTESIAN_POINT ( 'NONE',  ( 136.7507824285648894, 44.38599729999916121, 70.77785851943963280 ) ) ;
#6155=CARTESIAN_POINT ( 'NONE',  ( -71.16584859396995455, 19.60484997908767113, -42.38048587538112599 ) ) ;
#6156=CARTESIAN_POINT ( 'NONE',  ( -100.4262673593280226, 31.84860241619272969, 45.30150371153577282 ) ) ;
#6157=EDGE_CURVE ( 'NONE', #35238, #63173, #22176, .T. ) ;
#6160=CARTESIAN_POINT ( 'NONE',  ( -53.38065169970959545, 15.27943072477081721, -8.556598799231236896 ) ) ;
#6161=B_SPLINE_CURVE_WITH_KNOTS ( 'NONE', 3,
 ( #13636, #46326, #35091, #23508, #35442, #2397, #40024, #29466, #23855, #2056, #3095, #56542, #66779, #3429, #61134, #24206, #44949, #41065, #51621, #2741, #8372, #24894, #62524, #18568, #56196, #61484, #67131, #13304, #8014, #24555, #45990, #50925, #66436, #39674, #67460, #19252, #62161, #67802, #14339, #35793, #57242, #9057, #30507, #53320, #42771, #42094, #68155, #16048 ),
 .UNSPECIFIED., .F., .F.,
 ( 4, 2, 2, 2, 2, 2, 2, 2, 2, 2, 2, 2, 2, 2, 2, 2, 2, 2, 2, 2, 2, 2, 2, 4 ),
 ( 6.938893903907228378E-18, 0.001591515129442212751, 0.003183030258884418564, 0.003978787823605516374, 0.004774545388326614619, 0.006366060517768862281, 0.007957575647211110811, 0.009549090776653357607, 0.01034484834137448794, 0.01114060590609561828, 0.01193636347081674862, 0.01273212103553787895, 0.01432363616498013963, 0.01591515129442239856, 0.01671090885914353064, 0.01750666642386466271, 0.01830242398858579131, 0.01909818155330691991, 0.02068969668274923610, 0.02148545424747039592, 0.02228121181219155922, 0.02387272694163382336, 0.02466848450635492421, 0.02546424207107602852 ),
 .UNSPECIFIED. ) ;
#6162=ADVANCED_FACE ( 'NONE', ( #5043 ), #19853, .F. ) ;
#6168=CARTESIAN_POINT ( 'NONE',  ( -144.2038301586456157, 61.09856042007389476, -47.63804030527379041 ) ) ;
#6169=CARTESIAN_POINT ( 'NONE',  ( -166.0031475600388831, 80.98114714564768235, -66.67602937550397257 ) ) ;
#6171=CARTESIAN_POINT ( 'NONE',  ( -133.3913294106239391, 51.63304446851032026, 91.41765249869638410 ) ) ;
#6172=ORIENTED_EDGE ( 'NONE', *, *, #10339, .T. ) ;
#6173=CARTESIAN_POINT ( 'NONE',  ( 58.46823952472683317, 12.69204591816734684, 16.45271400437258080 ) ) ;
#6175=VECTOR ( 'NONE', #41501, 1000.000000000000000 ) ;
#6177=ORIENTED_EDGE ( 'NONE', *, *, #34254, .T. ) ;
#6179=CARTESIAN_POINT ( 'NONE',  ( -56.02358673658416421, 14.94347049174936970, -23.32432881613157960 ) ) ;
#6183=CARTESIAN_POINT ( 'NONE',  ( 184.3941060377211727, 82.01604625189465025, -23.62510121971022414 ) ) ;
#6184=CARTESIAN_POINT ( 'NONE',  ( 80.73012746365749592, 17.49169339352364005, -11.81929625901135417 ) ) ;
#6185=CARTESIAN_POINT ( 'NONE',  ( 94.12811352634518869, 22.11743943276049507, -70.69009586073259754 ) ) ;
#6188=CARTESIAN_POINT ( 'NONE',  ( -99.98930671699734773, 31.63190627461931470, 4.017523108268790999 ) ) ;
#6194=B_SPLINE_CURVE_WITH_KNOTS ( 'NONE', 3,
 ( #22551, #33475, #32419, #12001, #392, #1448, #13397, #24308, #39775, #40466, #39426, #7071, #46087, #66529, #8467, #40812, #8114, #67556, #34166, #55604, #18675, #3195, #44710, #29564, #23948, #34859, #50673, #24652, #2495, #18320, #29226, #12351, #33808, #7434, #50337, #29919, #35192, #45397, #60877, #61585, #66877, #45750, #13060 ),
 .UNSPECIFIED., .F., .F.,
 ( 4, 2, 2, 2, 2, 2, 2, 2, 1, 2, 2, 2, 2, 2, 2, 2, 2, 2, 2, 2, 2, 4 ),
 ( 1.734723475976807094E-18, 0.001466540241398130986, 0.002199810362097197672, 0.002933080482796264141, 0.004399620724194394476, 0.005866160965592523945, 0.007332701206990653413, 0.008065971327689720749, 0.008799241448388787218, 0.009532511569087855421, 0.01026578168978692363, 0.01173232193118506177, 0.01319886217258319644, 0.01466540241398133111, 0.01539867253468040278, 0.01613194265537947619, 0.01759848289677760913, 0.01906502313817574901, 0.01979829325887481201, 0.02053156337957388194, 0.02199810362097201488, 0.02346464386237014782 ),
 .UNSPECIFIED. ) ;
#6196=CARTESIAN_POINT ( 'NONE',  ( 10.83418588031599583, 6.392467435475930770, 31.86208434653760335 ) ) ;
#6200=DIRECTION ( 'NONE',  ( -0.000000000000000000, 0.000000000000000000, -1.000000000000000000 ) ) ;
#6201=CARTESIAN_POINT ( 'NONE',  ( -7.825402957745087207, -170.0000000000000000, -42.91807073194382838 ) ) ;
#6202=CARTESIAN_POINT ( 'NONE',  ( 43.35536254672140188, 9.973606330917817786, -49.49790769984580407 ) ) ;
#6205=CARTESIAN_POINT ( 'NONE',  ( -26.88635117726413171, 9.904687797303028063, 16.85200533244904619 ) ) ;
#6207=CARTESIAN_POINT ( 'NONE',  ( -15.27748264047829885, 7.491388194171919146, -41.93772705272429846 ) ) ;
#6208=CARTESIAN_POINT ( 'NONE',  ( -85.35521056349260505, 24.98314685266450752, 94.99999999999866418 ) ) ;
#6209=CARTESIAN_POINT ( 'NONE',  ( 89.20981392318256553, 21.38519354635262459, 71.10286512656854541 ) ) ;
#6210=CARTESIAN_POINT ( 'NONE',  ( 153.4268936273268764, 54.57409659828382331, -23.10063676753390283 ) ) ;
#6213=CARTESIAN_POINT ( 'NONE',  ( 110.6336604720866035, 30.17285371011658057, -89.61153874658104712 ) ) ;
#6214=CYLINDRICAL_SURFACE ( 'NONE', #57367, 7.500000000000013323 ) ;
#6216=ORIENTED_EDGE ( 'NONE', *, *, #53042, .F. ) ;
#6218=CARTESIAN_POINT ( 'NONE',  ( -29.49620345460274606, 9.280093073089046740, 18.13254437223945459 ) ) ;
#6219=CARTESIAN_POINT ( 'NONE',  ( 46.80475532923159676, 10.50744084852537341, -71.19293443510808572 ) ) ;
#6223=CARTESIAN_POINT ( 'NONE',  ( 90.94525594974463445, 22.00941049511687098, 84.75862509362771391 ) ) ;
#6226=VECTOR ( 'NONE', #63406, 1000.000000000000000 ) ;
#6229=CARTESIAN_POINT ( 'NONE',  ( -132.8123438040339579, 51.22132183644640691, 14.18276217007199946 ) ) ;
#6230=CARTESIAN_POINT ( 'NONE',  ( -168.7329347389696181, 83.83901812802758968, -48.31275808947942352 ) ) ;
#6231=CARTESIAN_POINT ( 'NONE',  ( -180.1266724401835688, 95.28036793547788363, 89.30961988341643121 ) ) ;
#6238=CARTESIAN_POINT ( 'NONE',  ( 198.4059165548112560, 99.71594270191988585, -12.89058402406104342 ) ) ;
#6240=CARTESIAN_POINT ( 'NONE',  ( -4.072522659361693442, 7.683023425615343349, -76.26080512505431841 ) ) ;
#6246=CARTESIAN_POINT ( 'NONE',  ( -96.76336539645315327, 31.18045094643427362, 32.91415803190486855 ) ) ;
#6248=CARTESIAN_POINT ( 'NONE',  ( 113.4418023215250457, 31.50656691678298316, 3.466527937886946464 ) ) ;
#6252=EDGE_LOOP ( 'NONE', ( #19238, #2485, #27981, #3587 ) ) ;
#6256=CARTESIAN_POINT ( 'NONE',  ( -78.66644367742111399, -170.0000000000000000, -69.46000122218158879 ) ) ;
#6258=CARTESIAN_POINT ( 'NONE',  ( 162.7921669283191761, 61.91024532638673605, 31.61904728604499226 ) ) ;
#6265=CARTESIAN_POINT ( 'NONE',  ( 39.40195752203892710, 8.409560354027373563, 3.069283715499574683 ) ) ;
#6267=CARTESIAN_POINT ( 'NONE',  ( -37.92511097250854846, 10.74631978746600325, -65.88783957002343072 ) ) ;
#6268=CARTESIAN_POINT ( 'NONE',  ( 20.35964562795319566, 7.697260051881318788, 70.32522021214651886 ) ) ;
#6279=CARTESIAN_POINT ( 'NONE',  ( -38.69577193929646342, 10.89562623693160326, -44.77552114323132315 ) ) ;
#6280=CARTESIAN_POINT ( 'NONE',  ( -94.77322158248860262, 29.12812870088611561, 91.80393034221229698 ) ) ;
#6284=CARTESIAN_POINT ( 'NONE',  ( -47.56904557163428393, 13.83539285446097189, 90.91553801162412185 ) ) ;
#6286=CARTESIAN_POINT ( 'NONE',  ( 79.23200707685337818, 17.02828389812517784, 65.31902592513927175 ) ) ;
#6290=VERTEX_POINT ( 'NONE', #47592 ) ;
#6293=CARTESIAN_POINT ( 'NONE',  ( 210.1954643503415525, 114.1986276268024056, -65.56311968808857671 ) ) ;
#6295=CARTESIAN_POINT ( 'NONE',  ( -71.16770070143910232, 19.60548673929829988, 10.54887064238381456 ) ) ;
#6297=CARTESIAN_POINT ( 'NONE',  ( -53.38256734720888375, 14.24001356352780689, 3.657108157446994134 ) ) ;
#6299=CARTESIAN_POINT ( 'NONE',  ( 103.0463737467386665, 26.78595250599333255, -95.00000000000133582 ) ) ;
#6302=DIRECTION ( 'NONE',  ( -0.000000000000000000, 1.000000000000000000, -0.000000000000000000 ) ) ;
#6304=DIRECTION ( 'NONE',  ( -0.000000000000000000, 1.000000000000000000, -0.000000000000000000 ) ) ;
#6306=ORIENTED_EDGE ( 'NONE', *, *, #9062, .F. ) ;
#6307=CARTESIAN_POINT ( 'NONE',  ( -80.55742067659893735, 23.05042616197511762, 30.64490407056336707 ) ) ;
#6308=CARTESIAN_POINT ( 'NONE',  ( 155.7265855639938650, 57.57443315515121895, -77.77659484219802266 ) ) ;
#6310=CARTESIAN_POINT ( 'NONE',  ( -23.93880457192868860, 8.479983864459175180, 64.80067904941660117 ) ) ;
#6311=CARTESIAN_POINT ( 'NONE',  ( 127.2397149628677653, 37.56999625068102944, -13.11060947991069447 ) ) ;
#6313=ORIENTED_EDGE ( 'NONE', *, *, #24718, .F. ) ;
#6314=CARTESIAN_POINT ( 'NONE',  ( -31.43908319763709969, 9.591432048623765638, 3.371903815725488585 ) ) ;
#6318=CARTESIAN_POINT ( 'NONE',  ( 208.9781236209185522, 112.4006213943319352, 42.88291611263555581 ) ) ;
#6319=EDGE_CURVE ( 'NONE', #67501, #23678, #48190, .T. ) ;
#6320=CARTESIAN_POINT ( 'NONE',  ( -5.879983509979055611, 7.779504553499496211, 57.20031220924396820 ) ) ;
#6328=ORIENTED_EDGE ( 'NONE', *, *, #10795, .T. ) ;
#6329=CARTESIAN_POINT ( 'NONE',  ( 158.3595886390531575, 58.34525996025799799, -24.23990596987918877 ) ) ;
#6333=CARTESIAN_POINT ( 'NONE',  ( -132.5858388588929131, 52.29441124308996791, -92.68433720153500133 ) ) ;
#6339=CARTESIAN_POINT ( 'NONE',  ( 84.27368848767926579, 18.63026910897605859, 3.230755797320154610 ) ) ;
#6348=EDGE_CURVE ( 'NONE', #66136, #22496, #2466, .T. ) ;
#6349=CARTESIAN_POINT ( 'NONE',  ( 87.58098510096633049, 19.74745174099416190, 2.912695539183820514 ) ) ;
#6351=VERTEX_POINT ( 'NONE', #22521 ) ;
#6354=CARTESIAN_POINT ( 'NONE',  ( 38.91512155099544401, 9.360679678889633593, 29.91383430596324899 ) ) ;
#6356=CARTESIAN_POINT ( 'NONE',  ( -131.2803255164624829, 50.14412978403780841, -10.34452356867482870 ) ) ;
#6361=CARTESIAN_POINT ( 'NONE',  ( 133.8566784816069344, 42.60093787723652525, -77.86786152285937135 ) ) ;
#6366=FACE_BOUND ( 'NONE', #12452, .T. ) ;
#6367=CARTESIAN_POINT ( 'NONE',  ( -1.314022807222069877, 6.554273999800678929, -66.00870565782550159 ) ) ;
#6368=CARTESIAN_POINT ( 'NONE',  ( -179.5186635612084274, 96.12511541314945873, 69.11882369886130562 ) ) ;
#6371=CARTESIAN_POINT ( 'NONE',  ( -4.502148936856956496, 7.704491846230413721, 44.35705480072686413 ) ) ;
#6374=CARTESIAN_POINT ( 'NONE',  ( -125.8938041572051389, 47.69968343338778283, -76.75825448869764500 ) ) ;
#6375=CARTESIAN_POINT ( 'NONE',  ( -14.84452950307166041, 8.460866451887698148, 34.96186735029871073 ) ) ;
#6376=CARTESIAN_POINT ( 'NONE',  ( 160.5141379054754225, 60.05651755415394177, 16.93420630349488931 ) ) ;
#6377=CARTESIAN_POINT ( 'NONE',  ( 43.68116950786570385, 10.02170697302967461, -90.63548873402001504 ) ) ;
#6378=ORIENTED_EDGE ( 'NONE', *, *, #64654, .T. ) ;
#6381=EDGE_LOOP ( 'NONE', ( #3291, #63257 ) ) ;
#6384=CARTESIAN_POINT ( 'NONE',  ( 39.88971011078925955, 8.472992116645420069, 56.75838489642695350 ) ) ;
#6386=CARTESIAN_POINT ( 'NONE',  ( 70.50372867914782660, 14.53505678900966913, -15.88564835880266024 ) ) ;
#6387=CARTESIAN_POINT ( 'NONE',  ( -31.43908319763709969, 10.61114334766715928, -50.31719736520186359 ) ) ;
#6389=CARTESIAN_POINT ( 'NONE',  ( -53.13788504024113024, 15.21566150156365183, -76.82833932811897171 ) ) ;
#6390=ORIENTED_EDGE ( 'NONE', *, *, #36540, .T. ) ;
#6391=CARTESIAN_POINT ( 'NONE',  ( -75.76674366953606921, 22.30988704043531712, -89.37459560296670702 ) ) ;
#6393=CARTESIAN_POINT ( 'NONE',  ( -118.6302575928420424, 43.07263081214306055, -13.68204589171926244 ) ) ;
#6394=ORIENTED_EDGE ( 'NONE', *, *, #52016, .T. ) ;
#6396=CARTESIAN_POINT ( 'NONE',  ( 36.08914434112043779, 9.014684630517852071, 70.99154541230063842 ) ) ;
#6397=CARTESIAN_POINT ( 'NONE',  ( 180.6710448012268557, 78.18844465372404784, 56.15314469597509373 ) ) ;
#6400=CARTESIAN_POINT ( 'NONE',  ( -168.7329347389695897, 83.83901812802758968, -21.46820749901573677 ) ) ;
#6404=CARTESIAN_POINT ( 'NONE',  ( 92.53033045403535084, 22.59263332688196257, 5.712192295102347828 ) ) ;
#6405=CARTESIAN_POINT ( 'NONE',  ( -15.13254930056756464, 7.477527548005404867, 66.16798222535943808 ) ) ;
#6406=CARTESIAN_POINT ( 'NONE',  ( -83.69653436244857403, 24.30167057287991028, -10.20239559727127165 ) ) ;
#6408=CARTESIAN_POINT ( 'NONE',  ( 41.35041461497707616, 8.670465437677201237, -9.016052168402659106 ) ) ;
#6409=CARTESIAN_POINT ( 'NONE',  ( 208.6132326550593916, 111.8685719053116543, -10.57063359225124799 ) ) ;
#6411=FACE_BOUND ( 'NONE', #28187, .T. ) ;
#6412=CARTESIAN_POINT ( 'NONE',  ( -62.54085973597666026, 16.81797209566546414, -43.20757385135579653 ) ) ;
#6413=EDGE_CURVE ( 'NONE', #16646, #34225, #39401, .T. ) ;
#6415=PLANE ( 'NONE',  #61463 ) ;
#6416=CARTESIAN_POINT ( 'NONE',  ( 93.72687053612523300, 23.04134601640627977, -45.79658200368525911 ) ) ;
#6417=LINE ( 'NONE', #48954, #36381 ) ;
#6419=CARTESIAN_POINT ( 'NONE',  ( 212.1913428512247037, 119.0779339498137688, 63.19771715593021355 ) ) ;
#6433=CARTESIAN_POINT ( 'NONE',  ( 102.7435092758398127, 25.56449004647817702, 37.38200955292992944 ) ) ;
#6437=ORIENTED_EDGE ( 'NONE', *, *, #19264, .T. ) ;
#6438=DIRECTION ( 'NONE',  ( -0.000000000000000000, 1.000000000000000000, -0.000000000000000000 ) ) ;
#6440=AXIS2_PLACEMENT_3D ( 'NONE', #30238, #19673, #62600 ) ;
#6441=CARTESIAN_POINT ( 'NONE',  ( -156.0209085498132424, 71.27066046086521567, -72.91444613903827587 ) ) ;
#6442=CARTESIAN_POINT ( 'NONE',  ( 69.36287815987334682, 15.27486453472191741, 6.465547984870822162 ) ) ;
#6445=CARTESIAN_POINT ( 'NONE',  ( -47.65155309726505806, 13.85482731128120015, -43.95499868855683445 ) ) ;
#6446=CARTESIAN_POINT ( 'NONE',  ( -48.23766733091050440, 13.99378332280058679, 14.11372853788430426 ) ) ;
#6448=CARTESIAN_POINT ( 'NONE',  ( -154.7858533099351632, 70.14406136060938479, -90.65412252175239871 ) ) ;
#6449=CARTESIAN_POINT ( 'NONE',  ( 64.62779760674203544, 13.05212430187077288, -89.57393277581095958 ) ) ;
#6450=CARTESIAN_POINT ( 'NONE',  ( 80.45890692537896882, 17.40706746439065000, 86.62450930750821954 ) ) ;
#6454=EDGE_CURVE ( 'NONE', #47540, #5410, #43085, .T. ) ;
#6457=CARTESIAN_POINT ( 'NONE',  ( -14.76369745117753141, 7.442560531763926512, -13.19444848579071028 ) ) ;
#6458=CARTESIAN_POINT ( 'NONE',  ( -165.6311038533940234, 80.59874732648039242, 91.58102387426585267 ) ) ;
#6460=FACE_OUTER_BOUND ( 'NONE', #38844, .T. ) ;
#6462=CARTESIAN_POINT ( 'NONE',  ( -58.76099769480629220, 16.75353773354894216, -36.19268434689433889 ) ) ;
#6464=CARTESIAN_POINT ( 'NONE',  ( -76.78936026062119424, 21.61552955137053544, -76.72525579395438911 ) ) ;
#6466=ORIENTED_EDGE ( 'NONE', *, *, #31873, .F. ) ;
#6468=ORIENTED_EDGE ( 'NONE', *, *, #15494, .T. ) ;
#6471=CARTESIAN_POINT ( 'NONE',  ( -61.71208512347170938, 17.61895039024948417, -92.92744643277735861 ) ) ;
#6472=DIRECTION ( 'NONE',  ( -0.000000000000000000, 1.000000000000000000, -0.000000000000000000 ) ) ;
#6473=CARTESIAN_POINT ( 'NONE',  ( 117.7417271423230147, 33.63613196344606138, -16.04272938009505012 ) ) ;
#6475=CARTESIAN_POINT ( 'NONE',  ( -109.0297561673455817, 36.34391931706015555, 14.45457006512591036 ) ) ;
#6476=CARTESIAN_POINT ( 'NONE',  ( -7.825402957745087207, -170.0000000000000000, 37.61558103944720699 ) ) ;
#6477=CARTESIAN_POINT ( 'NONE',  ( 139.7883986595927581, 46.32091287009613723, -21.27522919412053071 ) ) ;
#6483=CARTESIAN_POINT ( 'NONE',  ( -12.78015296493257758, 7.264294661536300879, 16.42255799229593549 ) ) ;
#6484=CARTESIAN_POINT ( 'NONE',  ( 32.15641333221390141, 7.577415570152255420, -68.01178621890366571 ) ) ;
#6485=CARTESIAN_POINT ( 'NONE',  ( 61.10129719786242219, 12.23677173834304988, -9.120487640209377744 ) ) ;
#6487=CARTESIAN_POINT ( 'NONE',  ( -35.99432170610150195, 10.38324794858010236, 58.58295102095021178 ) ) ;
#6491=CARTESIAN_POINT ( 'NONE',  ( 188.2091813586561670, 87.61952156613882892, 66.01175409503154867 ) ) ;
#6492=CARTESIAN_POINT ( 'NONE',  ( -157.0077369422017739, 70.81157624963286423, 64.78427050012133748 ) ) ;
#6493=CARTESIAN_POINT ( 'NONE',  ( -2.177337698256109899, 7.595833446947582779, -37.95934834430985916 ) ) ;
#6494=CARTESIAN_POINT ( 'NONE',  ( 106.6228877857910788, 27.24245963308693419, 16.85254313621388533 ) ) ;
#6495=CARTESIAN_POINT ( 'NONE',  ( -168.9758607987575090, 82.62968668822608720, -89.63544783193323440 ) ) ;
#6496=CARTESIAN_POINT ( 'NONE',  ( -81.01337222286376516, 23.22902179892323460, -49.75485830830231038 ) ) ;
#6497=FACE_BOUND ( 'NONE', #30299, .T. ) ;
#6499=CARTESIAN_POINT ( 'NONE',  ( 8.683531412707431230, 6.377173148747124820, -67.44837463207127826 ) ) ;
#6500=CIRCLE ( 'NONE', #58164, 242.4895526022646379 ) ;
#6505=CARTESIAN_POINT ( 'NONE',  ( -130.5740389938243311, 49.65308610043483384, -36.53356454646863938 ) ) ;
#6506=CARTESIAN_POINT ( 'NONE',  ( 46.90222083990963853, 9.503928413859245694, -69.72417923928249195 ) ) ;
#6508=EDGE_LOOP ( 'NONE', ( #61200, #15158, #29974, #33 ) ) ;
#6510=CARTESIAN_POINT ( 'NONE',  ( -129.1194034443450107, 48.65405036159125984, -89.31855732894304367 ) ) ;
#6515=CARTESIAN_POINT ( 'NONE',  ( 173.6012773665503914, 71.36035397668605640, -44.31334785685113076 ) ) ;
#6518=ORIENTED_EDGE ( 'NONE', *, *, #67134, .F. ) ;
#6519=CARTESIAN_POINT ( 'NONE',  ( 112.1100957124161539, 30.86846953551570394, 56.67668910139203575 ) ) ;
#6525=CARTESIAN_POINT ( 'NONE',  ( -189.3111515777349894, 107.1887855376296699, 39.51096003599841566 ) ) ;
#6534=CARTESIAN_POINT ( 'NONE',  ( -126.5249622811510619, 46.90973041002839494, 84.31430626055380628 ) ) ;
#6539=CARTESIAN_POINT ( 'NONE',  ( -133.3392045760936924, 51.59583146030206535, 37.06569111768722280 ) ) ;
#6540=CARTESIAN_POINT ( 'NONE',  ( -173.1211646369891355, -170.0000000000000000, 38.32169460664103156 ) ) ;
#6542=EDGE_CURVE ( 'NONE', #45708, #47842, #22923, .T. ) ;
#6543=CARTESIAN_POINT ( 'NONE',  ( 90.30840373526896769, 21.77864858272154081, 30.67197374571127000 ) ) ;
#6544=CARTESIAN_POINT ( 'NONE',  ( 84.05098130332766004, 18.55728792516086756, -9.429979211940626271 ) ) ;
#6547=CARTESIAN_POINT ( 'NONE',  ( 89.21005684773501798, 20.31770592753386850, -77.21217177953165844 ) ) ;
#6550=EDGE_LOOP ( 'NONE', ( #10957, #9468 ) ) ;
#6553=DIRECTION ( 'NONE',  ( -0.000000000000000000, 1.000000000000000000, -0.000000000000000000 ) ) ;
#6556=CARTESIAN_POINT ( 'NONE',  ( 212.1913428512246469, 119.0779339498137688, -44.18048520592454054 ) ) ;
#6558=CARTESIAN_POINT ( 'NONE',  ( -103.2129897037410586, 33.25684593987698889, 72.31981736734853428 ) ) ;
#6562=CARTESIAN_POINT ( 'NONE',  ( -30.46358361599562414, 10.45190018822945177, 18.32402868574788712 ) ) ;
#6565=CARTESIAN_POINT ( 'NONE',  ( 110.2429982417149574, -170.0000000000000000, -97.11153874658106133 ) ) ;
#6567=DIRECTION ( 'NONE',  ( -0.000000000000000000, 1.000000000000000000, -0.000000000000000000 ) ) ;
#6568=CARTESIAN_POINT ( 'NONE',  ( 36.08914434112045200, 9.014684630517862729, 17.30244423137330045 ) ) ;
#6572=DIRECTION ( 'NONE',  ( 0.000000000000000000, 0.000000000000000000, 1.000000000000000000 ) ) ;
#6574=EDGE_LOOP ( 'NONE', ( #32144, #13566 ) ) ;
#6576=CARTESIAN_POINT ( 'NONE',  ( 86.62931800182293784, 20.48449268398422518, 29.71208757247930521 ) ) ;
#6582=VECTOR ( 'NONE', #12041, 1000.000000000000000 ) ;
#6583=CARTESIAN_POINT ( 'NONE',  ( 91.46693946628187177, 22.19998770144037437, 85.16047213861423870 ) ) ;
#6589=CARTESIAN_POINT ( 'NONE',  ( -133.1093894320206061, 51.43221067881451347, 9.158613437822465286 ) ) ;
#6592=CARTESIAN_POINT ( 'NONE',  ( -132.8257891167039872, 52.46553896898736724, -39.53870018935421626 ) ) ;
#6593=ORIENTED_EDGE ( 'NONE', *, *, #1514, .T. ) ;
#6595=CYLINDRICAL_SURFACE ( 'NONE', #32964, 7.500000000000013323 ) ;
#6596=CARTESIAN_POINT ( 'NONE',  ( -145.5261806899007127, 60.87473129144527917, -21.82853397724819544 ) ) ;
#6597=CARTESIAN_POINT ( 'NONE',  ( -1.095583923122883663, 7.553030873957008673, -66.44300051098797155 ) ) ;
#6601=CARTESIAN_POINT ( 'NONE',  ( -60.64199216239837398, 17.30050036439947547, 5.965679938627520329 ) ) ;
#6602=CARTESIAN_POINT ( 'NONE',  ( 200.8410151090926377, 101.2014854111317703, -37.37915825681574233 ) ) ;
#6605=CARTESIAN_POINT ( 'NONE',  ( 23.09784929786603058, 6.844738137842332648, -41.32192824243960416 ) ) ;
#6606=CARTESIAN_POINT ( 'NONE',  ( 116.5100763992442694, 33.01539745157280237, 14.39398281521365064 ) ) ;
#6609=ORIENTED_EDGE ( 'NONE', *, *, #51552, .T. ) ;
#6611=CARTESIAN_POINT ( 'NONE',  ( 180.6713229637342693, 79.61878926895388986, 29.30859410551139987 ) ) ;
#6612=CARTESIAN_POINT ( 'NONE',  ( -34.92258123724119656, 11.21139125453447072, -89.86097876557430197 ) ) ;
#6613=CARTESIAN_POINT ( 'NONE',  ( -13.47517652744368633, 8.334971000693560228, -64.80585601353286052 ) ) ;
#6620=CARTESIAN_POINT ( 'NONE',  ( -33.36721086971962080, 9.915747831546610769, -8.720602974680872421 ) ) ;
#6621=CARTESIAN_POINT ( 'NONE',  ( 152.9731052498706276, 54.23675565345623539, -91.29877024755251114 ) ) ;
#6622=CARTESIAN_POINT ( 'NONE',  ( -132.4776673493542489, 52.21763813822158085, 7.674206648579892764 ) ) ;
#6623=CARTESIAN_POINT ( 'NONE',  ( 19.75315861330098599, 7.667327050329334703, 57.98827929678517989 ) ) ;
#6626=VECTOR ( 'NONE', #7830, 1000.000000000000000 ) ;
#6628=ORIENTED_EDGE ( 'NONE', *, *, #65770, .F. ) ;
#6632=CARTESIAN_POINT ( 'NONE',  ( -38.54881010929333485, 10.86689971295294299, -40.37941364402734479 ) ) ;
#6633=CARTESIAN_POINT ( 'NONE',  ( 63.01563776193090405, 12.67277567978497643, 17.96841034875761878 ) ) ;
#6636=CARTESIAN_POINT ( 'NONE',  ( -72.78270026377323632, 21.23376443558119675, -11.09364622117974264 ) ) ;
#6642=CARTESIAN_POINT ( 'NONE',  ( 211.5175447467295839, 116.1901475271413631, -67.53534590373220681 ) ) ;
#6644=CARTESIAN_POINT ( 'NONE',  ( -75.43044859198181484, 21.11535168543637653, 17.84392632519180921 ) ) ;
#6646=CARTESIAN_POINT ( 'NONE',  ( -50.14771795543005339, 13.42081263859818385, 5.278126018137767161 ) ) ;
#6652=DIRECTION ( 'NONE',  ( -0.000000000000000000, 1.000000000000000000, -0.000000000000000000 ) ) ;
#6653=ORIENTED_EDGE ( 'NONE', *, *, #64872, .F. ) ;
#6655=DIRECTION ( 'NONE',  ( -0.000000000000000000, 1.000000000000000000, -0.000000000000000000 ) ) ;
#6658=CARTESIAN_POINT ( 'NONE',  ( -29.03891846981454705, 10.22741474064055822, -76.78417915649073677 ) ) ;
#6660=CARTESIAN_POINT ( 'NONE',  ( 45.76553115525426563, 10.34124506813255095, 33.43704435240822903 ) ) ;
#6663=VERTEX_POINT ( 'NONE', #63169 ) ;
#6666=VECTOR ( 'NONE', #17877, 1000.000000000000000 ) ;
#6669=CARTESIAN_POINT ( 'NONE',  ( 34.82939798935585429, 8.870855050008911391, -10.31006242790380512 ) ) ;
#6672=CARTESIAN_POINT ( 'NONE',  ( 139.5357843740262069, 46.15750388987612496, 85.78907572748585153 ) ) ;
#6673=CARTESIAN_POINT ( 'NONE',  ( 198.7583180600454966, 100.1639442742712589, -92.92991841917546481 ) ) ;
#6677=CARTESIAN_POINT ( 'NONE',  ( -118.9649285217356010, 42.09781191014327106, -72.14050056521936938 ) ) ;
#6681=CARTESIAN_POINT ( 'NONE',  ( 164.4728833318992542, 63.30716077995683833, -14.07991251278742695 ) ) ;
#6684=B_SPLINE_CURVE_WITH_KNOTS ( 'NONE', 3,
 ( #27698, #54416, #64299, #37563, #15429, #43523, #31600, #42157, #4864, #5213, #32639, #69225, #59015, #26671, #48107, #21054, #16794, #5889, #59697, #42501, #21384, #58665, #42827, #16108, #37214, #10831, #32300, #48786, #11509, #43176, #32982, #48434, #37915, #53730, #5553, #271, #631, #27006, #59360, #22082, #65001, #28762, #55477, #6946 ),
 .UNSPECIFIED., .F., .F.,
 ( 4, 2, 2, 2, 2, 2, 2, 2, 2, 2, 2, 2, 2, 2, 2, 2, 2, 2, 2, 2, 2, 4 ),
 ( 0.02416815208377491586, 0.02567033257376879346, 0.02642142281876572879, 0.02717251306376266759, 0.02867469355375654519, 0.02942578379875346664, 0.03017687404375039156, 0.03167905453374424141, 0.03318123502373808431, 0.03393232526873500576, 0.03468341551373193415, 0.03618559600372578400, 0.03693668624872270545, 0.03768777649371962690, 0.03918995698371346287, 0.04069213747370729883, 0.04219431796370114174, 0.04369649845369498464, 0.04444758869869190610, 0.04519867894368882061, 0.04670085943368269821, 0.04820303992367657581 ),
 .UNSPECIFIED. ) ;
#6685=CARTESIAN_POINT ( 'NONE',  ( 137.3861614007145704, 44.78548268714478553, 16.78755531203335138 ) ) ;
#6692=VERTEX_POINT ( 'NONE', #30812 ) ;
#6696=AXIS2_PLACEMENT_3D ( 'NONE', #35794, #24207, #57244 ) ;
#6697=CARTESIAN_POINT ( 'NONE',  ( 92.51858280840788495, 21.51505926344913533, 5.696835879890508991 ) ) ;
#6700=CARTESIAN_POINT ( 'NONE',  ( 8.000000000000007105, 249.8719672152120381, 94.99999999999866418 ) ) ;
#6701=CARTESIAN_POINT ( 'NONE',  ( 69.36122620657974380, 15.27447566922079858, 94.99999999999866418 ) ) ;
#6702=CARTESIAN_POINT ( 'NONE',  ( 32.30062460741315533, 8.603096374765343057, 34.98847621939621888 ) ) ;
#6703=CARTESIAN_POINT ( 'NONE',  ( 67.55199883153194662, 14.80832170058783070, 31.32067154591900504 ) ) ;
#6704=CARTESIAN_POINT ( 'NONE',  ( -180.4951058960675709, 97.32429862471644810, -94.40723590757134787 ) ) ;
#6709=CARTESIAN_POINT ( 'NONE',  ( 141.1220430186941996, 47.19066702031172866, -68.48793956740368571 ) ) ;
#6710=CARTESIAN_POINT ( 'NONE',  ( -146.1140637052940008, 62.65471088530804877, -75.86152977379298079 ) ) ;
#6712=FACE_BOUND ( 'NONE', #67341, .T. ) ;
#6713=CARTESIAN_POINT ( 'NONE',  ( -7.825402957745087207, 6.891034867348160731, -62.26262132240749736 ) ) ;
#6715=CARTESIAN_POINT ( 'NONE',  ( -143.7133518487516710, 60.70463114991426323, -10.69940592156271997 ) ) ;
#6718=CYLINDRICAL_SURFACE ( 'NONE', #15271, 7.500000000000013323 ) ;
#6721=CARTESIAN_POINT ( 'NONE',  ( -119.5404913382139966, 43.63271406506957817, -73.25228717473794404 ) ) ;
#6722=CARTESIAN_POINT ( 'NONE',  ( -13.79190010541703337, 8.363435739308565431, 42.18623782823312496 ) ) ;
#6723=CARTESIAN_POINT ( 'NONE',  ( 162.8142581494935541, 61.92799983924231100, 15.34889811814740490 ) ) ;
#6726=CARTESIAN_POINT ( 'NONE',  ( -38.93938005333174601, 11.96888249046460118, 11.11159176475013766 ) ) ;
#6729=CARTESIAN_POINT ( 'NONE',  ( 80.16761386260782274, 18.37011649821943848, -74.00622491332923403 ) ) ;
#6730=CARTESIAN_POINT ( 'NONE',  ( 117.7396772390111437, 33.63508787755782947, 90.38373562684182616 ) ) ;
#6732=CARTESIAN_POINT ( 'NONE',  ( -14.97251655505445633, 7.462297851175272889, 89.00806855038318588 ) ) ;
#6734=CARTESIAN_POINT ( 'NONE',  ( -25.80443741485378695, 9.749985135376004308, -37.84319293131525797 ) ) ;
#6736=CARTESIAN_POINT ( 'NONE',  ( 117.4396227366912626, -170.0000000000000000, -95.00000000000133582 ) ) ;
#6739=ORIENTED_EDGE ( 'NONE', *, *, #61159, .T. ) ;
#6740=CARTESIAN_POINT ( 'NONE',  ( 36.30999198706538778, 9.040534725358945423, 71.09571704279858295 ) ) ;
#6742=CARTESIAN_POINT ( 'NONE',  ( 174.6176230994777825, 72.30829341023250834, 67.49244533490978881 ) ) ;
#6744=CARTESIAN_POINT ( 'NONE',  ( -166.7050147108374460, 81.70694330787515014, -11.44399333260963303 ) ) ;
#6748=VERTEX_POINT ( 'NONE', #908 ) ;
#6749=CARTESIAN_POINT ( 'NONE',  ( 106.6181401479172308, 28.34160787025144046, -36.85221939481564135 ) ) ;
#6750=CARTESIAN_POINT ( 'NONE',  ( -12.39701069459754912, 7.231688578592716077, 58.49449396597306361 ) ) ;
#6754=CARTESIAN_POINT ( 'NONE',  ( 212.0739503583954217, 117.0412199804969617, -18.37996829939370613 ) ) ;
#6755=FACE_BOUND ( 'NONE', #26345, .T. ) ;
#6756=CARTESIAN_POINT ( 'NONE',  ( -56.97107423601134002, 15.20373812575556727, -49.98290253789251381 ) ) ;
#6762=CARTESIAN_POINT ( 'NONE',  ( -180.6215424137752166, 97.48070480470859422, 11.78308709916989550 ) ) ;
#6763=CARTESIAN_POINT ( 'NONE',  ( 155.2910738464914004, 55.97560547655808705, 2.874285109824962881 ) ) ;
#6765=ADVANCED_FACE ( 'NONE', ( #11104 ), #20978, .T. ) ;
#6769=CARTESIAN_POINT ( 'NONE',  ( 55.52750043885183828, 11.05966813607792254, 9.978530875651303589 ) ) ;
#6774=CARTESIAN_POINT ( 'NONE',  ( -57.65574514524055871, 16.43983577669856189, -22.90970587626445365 ) ) ;
#6775=CARTESIAN_POINT ( 'NONE',  ( 103.8317086685000135, 26.02720265156214197, 41.01109807538037444 ) ) ;
#6782=CARTESIAN_POINT ( 'NONE',  ( 67.93317348534930034, 14.90531593353391848, 16.15235655697943429 ) ) ;
#6784=CARTESIAN_POINT ( 'NONE',  ( -50.53243683205840853, 14.55237037207940709, -36.71190027716730242 ) ) ;
#6785=CARTESIAN_POINT ( 'NONE',  ( 15.78827728214693416, -170.0000000000000000, -69.86349468914949057 ) ) ;
#6792=VERTEX_POINT ( 'NONE', #47691 ) ;
#6795=LINE ( 'NONE', #22985, #3189 ) ;
#6796=CARTESIAN_POINT ( 'NONE',  ( -170.5404825127988033, 85.78476310886819078, 84.96378268994482141 ) ) ;
#6797=CARTESIAN_POINT ( 'NONE',  ( -48.56549579811110817, 13.03742088415615896, -12.07592667915758611 ) ) ;
#6799=CARTESIAN_POINT ( 'NONE',  ( 108.3819860115547300, 28.02992728837240932, -23.85848975555797580 ) ) ;
#6800=CARTESIAN_POINT ( 'NONE',  ( -62.06231780744544579, 17.72446026058424806, -40.03704603771073778 ) ) ;
#6802=CARTESIAN_POINT ( 'NONE',  ( -71.16584859396995455, 19.60484997908768179, -69.22503646584482340 ) ) ;
#6803=CARTESIAN_POINT ( 'NONE',  ( 21.44031696305385282, 6.747195267824409370, -11.22020411404090012 ) ) ;
#6811=CARTESIAN_POINT ( 'NONE',  ( -58.54432058204184841, 16.69162069828844253, -89.76429277260994866 ) ) ;
#6814=CARTESIAN_POINT ( 'NONE',  ( 116.0963032583227914, 32.80867113471307306, -21.29345617767813437 ) ) ;
#6817=CARTESIAN_POINT ( 'NONE',  ( 137.3861614007144851, 44.78548268714477132, -10.05699527843033181 ) ) ;
#6819=EDGE_CURVE ( 'NONE', #44163, #59279, #55688, .T. ) ;
#6820=ORIENTED_EDGE ( 'NONE', *, *, #36756, .T. ) ;
#6824=DIRECTION ( 'NONE',  ( 0.000000000000000000, 0.000000000000000000, 1.000000000000000000 ) ) ;
#6826=CARTESIAN_POINT ( 'NONE',  ( 61.09275639403235658, 12.23448398202909715, -23.64161583801792688 ) ) ;
#6828=EDGE_CURVE ( 'NONE', #58537, #67063, #12507, .T. ) ;
#6832=CARTESIAN_POINT ( 'NONE',  ( 186.2680729609084551, 85.48839327635664631, 58.21274974874516772 ) ) ;
#6833=CARTESIAN_POINT ( 'NONE',  ( 197.6341357773624736, 98.74251867088338486, -68.13172239288054755 ) ) ;
#6836=CARTESIAN_POINT ( 'NONE',  ( -165.6393662153604112, 79.16886183052817216, 12.08284213267020846 ) ) ;
#6838=FACE_BOUND ( 'NONE', #9492, .T. ) ;
#6844=CARTESIAN_POINT ( 'NONE',  ( -132.9109786433856755, 51.29129389542018913, -66.59759312975943146 ) ) ;
#6845=CARTESIAN_POINT ( 'NONE',  ( -103.8932886509197004, 34.74144483217663293, -76.68729370199592665 ) ) ;
#6849=CARTESIAN_POINT ( 'NONE',  ( 62.04382205963241148, 13.48099884269680793, -62.61244101702975939 ) ) ;
#6855=CARTESIAN_POINT ( 'NONE',  ( 183.4744593358819031, 81.05536227200067856, 83.38285715921820440 ) ) ;
#6856=VERTEX_POINT ( 'NONE', #18479 ) ;
#6859=CARTESIAN_POINT ( 'NONE',  ( 181.0840389613909736, 78.60582251573003987, -36.22505766587961062 ) ) ;
#6860=CARTESIAN_POINT ( 'NONE',  ( 157.4703587214989113, 58.92748579479261650, 29.40946747225336466 ) ) ;
#6863=CARTESIAN_POINT ( 'NONE',  ( 110.2429982417149432, 29.99119854320847267, 56.45576479620100940 ) ) ;
#6864=CARTESIAN_POINT ( 'NONE',  ( 138.2136629441929472, 45.30947856186676859, 57.73192867322060806 ) ) ;
#6865=CARTESIAN_POINT ( 'NONE',  ( -72.76696720809545127, 20.16136115364207626, -37.95795318151130004 ) ) ;
#6866=VECTOR ( 'NONE', #7852, 1000.000000000000000 ) ;
#6867=LINE ( 'NONE', #1958, #67456 ) ;
#6870=ORIENTED_EDGE ( 'NONE', *, *, #38442, .T. ) ;
#6871=CARTESIAN_POINT ( 'NONE',  ( 116.5096233816161941, 31.89062767870469273, -47.55059037069165129 ) ) ;
#6872=CARTESIAN_POINT ( 'NONE',  ( -72.21889834709580214, 21.03534256744168829, 14.93684858560963136 ) ) ;
#6873=CARTESIAN_POINT ( 'NONE',  ( -142.0227972901369071, 59.36121938936276621, -42.86931618990738713 ) ) ;
#6875=CARTESIAN_POINT ( 'NONE',  ( -128.1931195763440883, 48.02619254066235044, 84.66445025086169096 ) ) ;
#6876=ORIENTED_EDGE ( 'NONE', *, *, #42110, .F. ) ;
#6877=CARTESIAN_POINT ( 'NONE',  ( 62.52762183777208094, 13.59210632617624803, 17.96841034875761878 ) ) ;
#6879=CARTESIAN_POINT ( 'NONE',  ( -128.7810612886106298, 48.42424427998344783, 31.19417675835600434 ) ) ;
#6882=CARTESIAN_POINT ( 'NONE',  ( 182.7720841008444097, 80.32850885226591231, -24.19120961474466114 ) ) ;
#6883=CARTESIAN_POINT ( 'NONE',  ( 138.2204650371259049, 44.12203217345470563, -10.56042420382598834 ) ) ;
#6885=CARTESIAN_POINT ( 'NONE',  ( 91.13361825170458985, 21.00701373666981198, -64.14955825547987445 ) ) ;
#6886=EDGE_CURVE ( 'NONE', #52688, #18508, #29046, .T. ) ;
#6892=CARTESIAN_POINT ( 'NONE',  ( 44.35071890818839790, 9.104600422692273654, 43.07060720302936829 ) ) ;
#6895=CYLINDRICAL_SURFACE ( 'NONE', #34070, 7.500000000000013323 ) ;
#6896=CARTESIAN_POINT ( 'NONE',  ( 210.0122310839192039, 115.7355030290287488, -38.51083372022162621 ) ) ;
#6898=LINE ( 'NONE', #28354, #23633 ) ;
#6899=CARTESIAN_POINT ( 'NONE',  ( -125.8938041572051105, 46.49392987655494380, -34.91370389823391918 ) ) ;
#6900=CARTESIAN_POINT ( 'NONE',  ( -30.46060138092287062, 9.432375387772216513, -35.36506637325409486 ) ) ;
#6901=DIRECTION ( 'NONE',  ( -0.8118923937861950435, -0.5838071093367415143, 0.000000000000000000 ) ) ;
#6912=CARTESIAN_POINT ( 'NONE',  ( -84.96580414052105823, 24.82184094495580240, 68.84061359761649612 ) ) ;
#6913=CARTESIAN_POINT ( 'NONE',  ( 129.5225439633633755, 40.02995148249141266, 30.87120519579052313 ) ) ;
#6918=CARTESIAN_POINT ( 'NONE',  ( -102.2801239173131194, 33.91021738430207222, -23.17002667451225406 ) ) ;
#6919=B_SPLINE_CURVE_WITH_KNOTS ( 'NONE', 3,
 ( #19338, #14419, #3509, #24979, #3176, #40110, #8802, #46411, #56629, #34843, #29902, #40450, #35871, #13382, #61895, #30595, #40794, #62249 ),
 .UNSPECIFIED., .F., .F.,
 ( 4, 2, 2, 2, 2, 2, 2, 2, 4 ),
 ( 0.000000000000000000, 0.001360351328785557685, 0.002040526993178300424, 0.002720702657571043813, 0.004081053986356537530, 0.005441405315142032115, 0.006801756643927526699, 0.008162107972713021284, 0.01088281063028401045 ),
 .UNSPECIFIED. ) ;
#6926=CARTESIAN_POINT ( 'NONE',  ( -8.810383862755523765, 7.965311326754785703, 18.22247569387398158 ) ) ;
#6929=CARTESIAN_POINT ( 'NONE',  ( -95.07081908554464178, 29.26686063496962120, -94.08517559775140171 ) ) ;
#6933=CARTESIAN_POINT ( 'NONE',  ( -38.17232309348612773, 11.81874355808867705, -39.47676223961260433 ) ) ;
#6935=CARTESIAN_POINT ( 'NONE',  ( -168.0003605155415016, 83.06333427281273885, -47.69718177220133271 ) ) ;
#6936=CARTESIAN_POINT ( 'NONE',  ( -165.8118651643725059, 79.34448671302054379, 90.28955021999587416 ) ) ;
#6940=ADVANCED_FACE ( 'NONE', ( #8277 ), #14917, .T. ) ;
#6942=CARTESIAN_POINT ( 'NONE',  ( -2.172839205444465627, 7.595638683704374117, -74.71678878236892274 ) ) ;
#6946=CARTESIAN_POINT ( 'NONE',  ( 86.62931800182293784, 20.48449268398423584, 17.86753698201564688 ) ) ;
#6947=CARTESIAN_POINT ( 'NONE',  ( -96.02159028238557426, 30.82695531378848486, 42.15941767080024505 ) ) ;
#6949=LINE ( 'NONE', #18898, #5612 ) ;
#6950=CIRCLE ( 'NONE', #48438, 243.4957430088094839 ) ;
#6956=EDGE_LOOP ( 'NONE', ( #35684, #60493, #21224, #39983 ) ) ;
#6957=CARTESIAN_POINT ( 'NONE',  ( -118.5480034463614629, 41.84363520065495123, -94.51110357902348369 ) ) ;
#6959=CARTESIAN_POINT ( 'NONE',  ( -38.78626392836186909, 11.93872315530319916, -95.00000000000133582 ) ) ;
#6960=CARTESIAN_POINT ( 'NONE',  ( -7.825402957745087207, 7.899365992529248537, -62.26262132240749736 ) ) ;
#6962=CARTESIAN_POINT ( 'NONE',  ( 164.3577270662354408, 63.21061577643033758, 33.92876650929636639 ) ) ;
#6970=CARTESIAN_POINT ( 'NONE',  ( -34.06864996337442619, 10.03773626259442153, -8.944471349985661845 ) ) ;
#6973=CARTESIAN_POINT ( 'NONE',  ( -133.1640943168118554, 52.70734926280009347, 13.13691334606962613 ) ) ;
#6974=CARTESIAN_POINT ( 'NONE',  ( 23.28809538736929241, 7.864824219997537114, 64.85145018203481015 ) ) ;
#6975=ORIENTED_EDGE ( 'NONE', *, *, #42870, .T. ) ;
#6978=CARTESIAN_POINT ( 'NONE',  ( 86.62931800182293784, -170.0000000000000000, 44.71208757247933363 ) ) ;
#6979=CARTESIAN_POINT ( 'NONE',  ( 181.0840389613909736, 78.60582251573005408, -63.06960825634327961 ) ) ;
#6982=CARTESIAN_POINT ( 'NONE',  ( -100.8462079694196945, 32.05831806546150631, 84.34044455310514365 ) ) ;
#6984=CARTESIAN_POINT ( 'NONE',  ( -133.3958821919893012, 51.63629593114586669, 64.45030094466832793 ) ) ;
#6985=CARTESIAN_POINT ( 'NONE',  ( -75.00452312211126582, 22.03104735285382176, -22.32063719065431329 ) ) ;
#6988=CARTESIAN_POINT ( 'NONE',  ( 80.72161230109723817, 17.48902961068032980, 59.40974494857174193 ) ) ;
#6990=CARTESIAN_POINT ( 'NONE',  ( 32.90953848114693869, 7.653665824624196645, 33.65092423327369175 ) ) ;
#6991=EDGE_CURVE ( 'NONE', #27549, #62345, #36388, .T. ) ;
#6993=CARTESIAN_POINT ( 'NONE',  ( 185.1802655733641245, 82.84606286178494372, 43.10721277487510150 ) ) ;
#6994=CARTESIAN_POINT ( 'NONE',  ( 39.40195752203892710, 9.424259417798131366, -23.77526687496409608 ) ) ;
#6997=CARTESIAN_POINT ( 'NONE',  ( -118.8691191306315034, 43.21907118237572121, 67.60517970726668580 ) ) ;
#6998=CARTESIAN_POINT ( 'NONE',  ( -50.13771638889895144, 13.41835215703894235, 16.65896950491509898 ) ) ;
#7000=CARTESIAN_POINT ( 'NONE',  ( 150.0433793199863430, 52.09973307442955814, -44.70445035943132694 ) ) ;
#7006=ORIENTED_EDGE ( 'NONE', *, *, #51305, .T. ) ;
#7008=DIRECTION ( 'NONE',  ( -0.000000000000000000, 1.000000000000000000, -0.000000000000000000 ) ) ;
#7010=ORIENTED_EDGE ( 'NONE', *, *, #52782, .T. ) ;
#7012=CARTESIAN_POINT ( 'NONE',  ( 150.4722669492348643, 53.65054032737663192, -73.17996140608711642 ) ) ;
#7013=CARTESIAN_POINT ( 'NONE',  ( 44.34362023773823580, 10.12115849931653244, 31.75035674218548820 ) ) ;
#7015=CARTESIAN_POINT ( 'NONE',  ( -24.94151142167915935, 8.614613465433023975, 60.78288318456196038 ) ) ;
#7016=ORIENTED_EDGE ( 'NONE', *, *, #17879, .T. ) ;
#7018=LINE ( 'NONE', #12296, #51437 ) ;
#7020=CARTESIAN_POINT ( 'NONE',  ( 33.44035656425387515, 8.720466003183668491, -11.69816230808393875 ) ) ;
#7022=CARTESIAN_POINT ( 'NONE',  ( -31.43908319763709969, 9.591432048623765638, -77.16174795566554678 ) ) ;
#7024=CARTESIAN_POINT ( 'NONE',  ( -25.26048095167901053, 9.674257073897546633, -92.24941411008894931 ) ) ;
#7025=( LENGTH_UNIT ( ) NAMED_UNIT ( * ) SI_UNIT ( .MILLI., .METRE. ) );
#7028=EDGE_LOOP ( 'NONE', ( #6437, #50230, #48154, #1980 ) ) ;
#7033=CARTESIAN_POINT ( 'NONE',  ( -127.9466635691204033, 49.07377124385244826, -88.87715223634489803 ) ) ;
#7035=ORIENTED_EDGE ( 'NONE', *, *, #33293, .T. ) ;
#7040=ORIENTED_EDGE ( 'NONE', *, *, #43748, .F. ) ;
#7041=CARTESIAN_POINT ( 'NONE',  ( -125.6703656163501677, 47.55170550253211559, 3.775397282693374379 ) ) ;
#7042=CARTESIAN_POINT ( 'NONE',  ( 91.51282003084288874, 21.14522045960332619, 16.08068469543150059 ) ) ;
#7043=EDGE_CURVE ( 'NONE', #58885, #58406, #45602, .T. ) ;
#7045=ORIENTED_EDGE ( 'NONE', *, *, #49743, .F. ) ;
#7050=CARTESIAN_POINT ( 'NONE',  ( 70.36689301615740533, 15.53981654908576715, 92.52592592651693337 ) ) ;
#7051=CARTESIAN_POINT ( 'NONE',  ( 37.45439421541016856, 9.177432671831381228, 44.67329806592552899 ) ) ;
#7056=CARTESIAN_POINT ( 'NONE',  ( -148.7068999155605127, 63.50299517929035176, -88.53389495002838316 ) ) ;
#7057=CARTESIAN_POINT ( 'NONE',  ( 133.8566784816069628, 41.42467568809806977, -62.86786152285933582 ) ) ;
#7058=ORIENTED_EDGE ( 'NONE', *, *, #59330, .T. ) ;
#7059=CARTESIAN_POINT ( 'NONE',  ( 136.9822423813093053, 44.53121110416871886, -77.18959649595817041 ) ) ;
#7061=EDGE_LOOP ( 'NONE', ( #11577, #29186, #63939, #24140 ) ) ;
#7065=CARTESIAN_POINT ( 'NONE',  ( -37.39246151129640339, 11.66872370876246201, 42.30430913977911445 ) ) ;
#7066=CARTESIAN_POINT ( 'NONE',  ( -146.1140637052938303, 62.65471088530801325, -22.17242859286556822 ) ) ;
#7069=CARTESIAN_POINT ( 'NONE',  ( -9.503708068039186330, 7.005809988361353824, -89.28523705486915674 ) ) ;
#7070=CARTESIAN_POINT ( 'NONE',  ( -54.56693200831791302, 14.55131601960338728, -62.06087458892353226 ) ) ;
#7071=CARTESIAN_POINT ( 'NONE',  ( -2.177337698256113896, 7.595833446947585443, -11.11479775384615287 ) ) ;
#7072=CARTESIAN_POINT ( 'NONE',  ( -12.78319349481551015, 8.274445259016799170, 43.26445497206980662 ) ) ;
#7073=CARTESIAN_POINT ( 'NONE',  ( 112.7784411285248751, 30.07270878825235272, 3.204304144210361915 ) ) ;
#7074=CARTESIAN_POINT ( 'NONE',  ( -49.10775795518740949, 14.20291014622890913, -91.82781261574977805 ) ) ;
#7075=ORIENTED_EDGE ( 'NONE', *, *, #19264, .F. ) ;
#7076=CARTESIAN_POINT ( 'NONE',  ( -100.4440683050664518, 32.98184228837416043, -35.22808132192965758 ) ) ;
#7080=CARTESIAN_POINT ( 'NONE',  ( 79.18180043629686793, 18.06526831600452354, -71.18470387585151116 ) ) ;
#7081=B_SPLINE_CURVE_WITH_KNOTS ( 'NONE', 3,
 ( #52052, #20728, #9491, #67545, #14759, #29907, #63303, #19690, #52397, #40799, #41844, #47110, #57331, #24984, #58348, #46074, #67895, #62253, #68574, #15458, #9837, #51707, #30599, #36910, #51366, #3181, #42524, #38907, #33975, #23432, #55415, #43806, #12515, #11808, #38194, #1609, #65639, #6543, #33286, #28701, #17432, #4890, #27640, #64940, #65280 ),
 .UNSPECIFIED., .F., .F.,
 ( 4, 2, 2, 2, 2, 2, 2, 2, 2, 2, 2, 1, 2, 2, 2, 2, 2, 2, 2, 2, 2, 2, 4 ),
 ( 0.000000000000000000, 0.001510509505235996860, 0.002265764257853974690, 0.003021019010471952086, 0.004531528515707860909, 0.005286783268325837871, 0.006042038020943815702, 0.007552547526179744473, 0.009063057031415674980, 0.01057356653665160462, 0.01132882128926957117, 0.01208407604188753426, 0.01283933079450549734, 0.01359458554712346216, 0.01510509505235941782, 0.01586034980497739652, 0.01661560455759537175, 0.01812611406283131180, 0.01963662356806725184, 0.02039187832068520972, 0.02114713307330316414, 0.02265764257853903826, 0.02416815208377490892 ),
 .UNSPECIFIED. ) ;
#7082=CARTESIAN_POINT ( 'NONE',  ( 46.84183314611287585, 9.494161546644495075, 65.23765100148109752 ) ) ;
#7086=CARTESIAN_POINT ( 'NONE',  ( -73.27510762699375846, 21.40833250163870360, -91.07236566172743153 ) ) ;
#7090=FACE_OUTER_BOUND ( 'NONE', #27961, .T. ) ;
#7093=CARTESIAN_POINT ( 'NONE',  ( -167.4860113959264822, 82.52233889531186151, 70.12209724409757428 ) ) ;
#7095=CARTESIAN_POINT ( 'NONE',  ( -166.9992034932274976, 82.01285191063135471, -11.00469205210656476 ) ) ;
#7099=CARTESIAN_POINT ( 'NONE',  ( 94.02499804464930833, 23.15433260743127164, 11.63953833574553798 ) ) ;
#7101=CARTESIAN_POINT ( 'NONE',  ( -85.91089317961403538, 25.21459833389209848, -17.77817569153331334 ) ) ;
#7103=CARTESIAN_POINT ( 'NONE',  ( -102.2801239173131052, 32.78103895658057354, 30.51907450641510522 ) ) ;
#7105=FACE_BOUND ( 'NONE', #59118, .T. ) ;
#7107=CARTESIAN_POINT ( 'NONE',  ( 157.4703587214989113, 58.92748579479258808, 56.25401806271706562 ) ) ;
#7113=CARTESIAN_POINT ( 'NONE',  ( -52.00092620775819796, 14.92276858858357080, 57.80656622093086128 ) ) ;
#7121=ORIENTED_EDGE ( 'NONE', *, *, #22252, .F. ) ;
#7125=CARTESIAN_POINT ( 'NONE',  ( -62.54086041493278714, 17.86944394914986844, -15.38065428761472297 ) ) ;
#7126=CARTESIAN_POINT ( 'NONE',  ( 88.98820631332496589, 21.30618275724809507, -77.30172795873590985 ) ) ;
#7127=EDGE_LOOP ( 'NONE', ( #23271, #45642, #57596, #10332 ) ) ;
#7129=CARTESIAN_POINT ( 'NONE',  ( 42.03719354205840375, 9.783015072457470040, 71.28445026601322354 ) ) ;
#7130=CARTESIAN_POINT ( 'NONE',  ( 162.7963212667073378, 63.21900188423068556, 42.19573780102387417 ) ) ;
#7131=CARTESIAN_POINT ( 'NONE',  ( -156.6862310659955142, 71.88416263379568250, -66.91380956130490176 ) ) ;
#7132=CARTESIAN_POINT ( 'NONE',  ( 64.93224207568370332, 14.16036304753835751, 17.72345651798445232 ) ) ;
#7133=CARTESIAN_POINT ( 'NONE',  ( 88.30010642107259855, 19.99780058782973668, 44.52758616833133942 ) ) ;
#7135=B_SPLINE_CURVE_WITH_KNOTS ( 'NONE', 3,
 ( #38532, #11792, #2307, #23420, #45901, #45201, #49770, #66683, #18477, #13206, #61385, #1596, #29721, #23060, #39927, #6872, #18822, #35003, #33623, #12863, #34671, #55053, #28684, #56107, #33963, #51185, #7923, #44512, #17416, #39585, #65987, #28324, #61037, #29376, #18132, #50139, #12505, #50828, #34317, #1963, #56447, #2647, #24110, #17787, #67033 ),
 .UNSPECIFIED., .F., .F.,
 ( 4, 2, 2, 2, 2, 2, 2, 2, 2, 2, 2, 1, 2, 2, 2, 2, 2, 2, 2, 2, 2, 2, 4 ),
 ( 0.000000000000000000, 0.001512548138464662540, 0.002268822207696996520, 0.003025096276929330717, 0.004537644415393961815, 0.005293918484626292977, 0.006050192553858625005, 0.007562740692323284726, 0.009075288830787947916, 0.01058783696925261197, 0.01134411103848494314, 0.01210038510771727083, 0.01285665917694960199, 0.01361293324618192968, 0.01512548138464658333, 0.01588175545387890755, 0.01663802952311123351, 0.01815057766157588195, 0.01966312580004053387, 0.02041939986927285983, 0.02117567393850518578, 0.02268822207696979953, 0.02420077021543441328 ),
 .UNSPECIFIED. ) ;
#7136=ADVANCED_FACE ( 'NONE', ( #37403 ), #15619, .F. ) ;
#7139=CARTESIAN_POINT ( 'NONE',  ( -128.7724923851857284, 49.63576597317771899, -8.639783561551448443 ) ) ;
#7141=CARTESIAN_POINT ( 'NONE',  ( 116.8937673311173029, 32.08228998570054102, -20.05360614510496831 ) ) ;
#7142=CARTESIAN_POINT ( 'NONE',  ( 79.53586065807786554, 17.12142427614169549, 88.44133967985683853 ) ) ;
#7147=EDGE_CURVE ( 'NONE', #60092, #3228, #23810, .T. ) ;
#7150=CARTESIAN_POINT ( 'NONE',  ( -14.19493007850031674, 7.389842975086043708, -20.04074768020527486 ) ) ;
#7151=CARTESIAN_POINT ( 'NONE',  ( 175.8947993867357411, 74.90689716047910451, 4.528190670890809955 ) ) ;
#7152=CARTESIAN_POINT ( 'NONE',  ( -54.56693200831794144, 14.55131601960339260, -8.371773407996172978 ) ) ;
#7153=CARTESIAN_POINT ( 'NONE',  ( 103.1653143050726271, 25.74301230421574971, -14.04530181743896300 ) ) ;
#7155=CARTESIAN_POINT ( 'NONE',  ( -56.01329802674222691, 15.98369420723829215, -50.17033095554772615 ) ) ;
#7164=ORIENTED_EDGE ( 'NONE', *, *, #59844, .T. ) ;
#7166=CARTESIAN_POINT ( 'NONE',  ( -142.0227972901369071, 59.36121938936275910, 10.81978499101997926 ) ) ;
#7170=CARTESIAN_POINT ( 'NONE',  ( -166.7136514167008841, 81.71618216218793407, 34.41466395245560506 ) ) ;
#7171=CARTESIAN_POINT ( 'NONE',  ( 113.4418023215250741, 31.50656691678298316, -23.37802265257673184 ) ) ;
#7172=CARTESIAN_POINT ( 'NONE',  ( -104.5730787903383145, 33.96058035148152499, 18.33112389144127263 ) ) ;
#7173=CARTESIAN_POINT ( 'NONE',  ( 173.9832054143776077, -170.0000000000000000, -95.00000000000133582 ) ) ;
#7174=CARTESIAN_POINT ( 'NONE',  ( 134.0849965622594198, 42.73957449886182758, -24.17876034193199786 ) ) ;
#7179=CARTESIAN_POINT ( 'NONE',  ( -11.78792974237933322, 7.181513757308655599, 4.398590650106096511 ) ) ;
#7181=CARTESIAN_POINT ( 'NONE',  ( 93.74127541358416238, 23.04685498098406171, -94.59213288005628328 ) ) ;
#7184=CARTESIAN_POINT ( 'NONE',  ( 197.6341357773624736, 98.74251867088341328, 66.09103055943789684 ) ) ;
#7187=CARTESIAN_POINT ( 'NONE',  ( 197.8598785550297521, 99.02620879292950917, -73.76648511621989712 ) ) ;
#7188=CARTESIAN_POINT ( 'NONE',  ( -7.336630171688596214, 7.867399454768214895, -50.41807073194386390 ) ) ;
#7190=CARTESIAN_POINT ( 'NONE',  ( -165.9111709580270428, 79.44576090485632847, 13.56375512218778567 ) ) ;
#7191=CARTESIAN_POINT ( 'NONE',  ( 79.40386128751609363, 18.13359811229536689, -95.00000000000133582 ) ) ;
#7192=FACE_BOUND ( 'NONE', #64297, .T. ) ;
#7193=CARTESIAN_POINT ( 'NONE',  ( 45.80999061969644970, -170.0000000000000000, 94.99999999999866418 ) ) ;
#7199=CARTESIAN_POINT ( 'NONE',  ( -129.6001310305488801, 48.98284622040322489, -62.73388853355896089 ) ) ;
#7200=CARTESIAN_POINT ( 'NONE',  ( -105.4487797565984266, 35.55724615608639994, -76.17295365369301408 ) ) ;
#7203=VECTOR ( 'NONE', #69, 1000.000000000000000 ) ;
#7204=ADVANCED_FACE ( 'NONE', ( #29291 ), #18387, .F. ) ;
#7207=CARTESIAN_POINT ( 'NONE',  ( -132.5824930541232902, 51.05842456469446944, -92.67789068422645471 ) ) ;
#7209=CARTESIAN_POINT ( 'NONE',  ( 188.3847560247618276, 86.31304713945776541, 88.76876813952972611 ) ) ;
#7210=ORIENTED_EDGE ( 'NONE', *, *, #63302, .F. ) ;
#7213=DIRECTION ( 'NONE',  ( -0.000000000000000000, 1.000000000000000000, -0.000000000000000000 ) ) ;
#7214=CARTESIAN_POINT ( 'NONE',  ( 152.2924710224605462, 54.98503313872890175, 42.34074644621131966 ) ) ;
#7217=CARTESIAN_POINT ( 'NONE',  ( 63.01563776193091826, -170.0000000000000000, -43.22069083216975116 ) ) ;
#7218=CARTESIAN_POINT ( 'NONE',  ( -180.6209440844958181, 95.88392769199009535, 11.79712387883822267 ) ) ;
#7219=CARTESIAN_POINT ( 'NONE',  ( -73.81689110552362365, 20.53332132481501304, -48.34183327519426143 ) ) ;
#7223=CARTESIAN_POINT ( 'NONE',  ( -190.3074740493607067, 108.5764897054613272, 34.54018387887567343 ) ) ;
#7224=EDGE_CURVE ( 'NONE', #9825, #52425, #2564, .T. ) ;
#7230=CARTESIAN_POINT ( 'NONE',  ( -147.1538409485623049, 63.51600817366545471, -49.43746523392897529 ) ) ;
#7232=CARTESIAN_POINT ( 'NONE',  ( -133.4012376778782141, 51.64011534538437331, 91.75614716867997345 ) ) ;
#7233=EDGE_LOOP ( 'NONE', ( #68377, #7605 ) ) ;
#7234=CARTESIAN_POINT ( 'NONE',  ( 80.30232379693109124, 17.35837133860830761, -47.35644897165359168 ) ) ;
#7238=DIRECTION ( 'NONE',  ( -0.000000000000000000, 1.000000000000000000, -0.000000000000000000 ) ) ;
#7239=CARTESIAN_POINT ( 'NONE',  ( 79.63513233364426469, 18.20496177163924045, 34.49303652560662670 ) ) ;
#7242=CARTESIAN_POINT ( 'NONE',  ( 136.9934874058117771, 43.35050367224291534, -9.850568217420210715 ) ) ;
#7244=CARTESIAN_POINT ( 'NONE',  ( -176.3763474213711504, 92.36993073950279154, -22.13818532828629770 ) ) ;
#7245=AXIS2_PLACEMENT_3D ( 'NONE', #45288, #18914, #67453 ) ;
#7246=CARTESIAN_POINT ( 'NONE',  ( -53.38065169970958124, 15.27943072477081721, 45.13250238169609929 ) ) ;
#7250=CARTESIAN_POINT ( 'NONE',  ( 39.89571693415782505, 8.473773298340390170, 44.91383430596326320 ) ) ;
#7252=CARTESIAN_POINT ( 'NONE',  ( 159.2319614735956463, 59.03334608081209467, 56.45037870953245829 ) ) ;
#7253=FACE_OUTER_BOUND ( 'NONE', #26699, .T. ) ;
#7256=EDGE_CURVE ( 'NONE', #55692, #12765, #68319, .T. ) ;
#7258=CARTESIAN_POINT ( 'NONE',  ( 205.5130322755755117, 109.1888880665735257, -36.32593103262158252 ) ) ;
#7259=CARTESIAN_POINT ( 'NONE',  ( -74.18622060908360538, 21.73430079572374041, -75.49420155812906330 ) ) ;
#7260=LINE ( 'NONE', #23091, #57337 ) ;
#7262=CARTESIAN_POINT ( 'NONE',  ( -28.13266652174639049, 9.071935854491421480, -36.08090444528406238 ) ) ;
#7263=CARTESIAN_POINT ( 'NONE',  ( 164.6406716478538499, 63.44801348349339776, -72.68468498746710793 ) ) ;
#7266=ORIENTED_EDGE ( 'NONE', *, *, #23821, .T. ) ;
#7269=DIRECTION ( 'NONE',  ( -0.000000000000000000, 1.000000000000000000, -0.000000000000000000 ) ) ;
#7273=LINE ( 'NONE', #1639, #60353 ) ;
#7274=CARTESIAN_POINT ( 'NONE',  ( -94.78138776532237841, 30.24234841992713285, -15.13398054818980398 ) ) ;
#7276=CARTESIAN_POINT ( 'NONE',  ( 36.21730804119342650, 8.016524789962645059, 84.30459139221660791 ) ) ;
#7278=ORIENTED_EDGE ( 'NONE', *, *, #15260, .T. ) ;
#7281=CARTESIAN_POINT ( 'NONE',  ( -13.79190010541703160, 8.363435739308561878, 15.34168723776943821 ) ) ;
#7285=ORIENTED_EDGE ( 'NONE', *, *, #58832, .F. ) ;
#7288=CARTESIAN_POINT ( 'NONE',  ( -38.93938005333174601, 11.96888249046460651, -42.57750941617720741 ) ) ;
#7289=CARTESIAN_POINT ( 'NONE',  ( -172.3038663181179686, 87.72015621195183144, -34.71195716474998960 ) ) ;
#7292=CARTESIAN_POINT ( 'NONE',  ( -119.5267374018686581, 42.44190186039714519, -38.41742699949217155 ) ) ;
#7295=EDGE_CURVE ( 'NONE', #47869, #1332, #15453, .T. ) ;
#7299=CARTESIAN_POINT ( 'NONE',  ( -173.1211646369891355, 88.63826465341152527, 45.82169460664104577 ) ) ;
#7300=CARTESIAN_POINT ( 'NONE',  ( 197.1974290009105459, 96.59277840252784131, -44.14995505087879479 ) ) ;
#7303=CARTESIAN_POINT ( 'NONE',  ( 21.75684465274326129, 6.764994602232770049, -38.45100986864918013 ) ) ;
#7306=CARTESIAN_POINT ( 'NONE',  ( 112.5537757279407032, 31.07998172410696469, 17.41770588639016282 ) ) ;
#7307=VERTEX_POINT ( 'NONE', #14154 ) ;
#7309=EDGE_CURVE ( 'NONE', #16185, #25573, #56561, .T. ) ;
#7310=CARTESIAN_POINT ( 'NONE',  ( 59.29597493004737885, 11.84030339376941043, 43.84378064322283564 ) ) ;
#7316=CARTESIAN_POINT ( 'NONE',  ( -119.2006376716276037, 42.24203504200470860, -92.71035546800322891 ) ) ;
#7319=EDGE_CURVE ( 'NONE', #52964, #41204, #17945, .T. ) ;
#7322=CARTESIAN_POINT ( 'NONE',  ( -96.46475761760915191, 31.03789227780931981, 86.96133435859920269 ) ) ;
#7327=CARTESIAN_POINT ( 'NONE',  ( 207.4610690199662031, 111.9701171077052209, -63.68629331923244052 ) ) ;
#7328=CARTESIAN_POINT ( 'NONE',  ( -38.89042640463648581, 10.93374343663408865, -14.98468536607676960 ) ) ;
#7330=CARTESIAN_POINT ( 'NONE',  ( -126.3453033442920628, 47.99870040347945377, 3.775397282693373047 ) ) ;
#7331=CARTESIAN_POINT ( 'NONE',  ( 15.78827728214693416, 7.507518794609588042, 56.85925826316891829 ) ) ;
#7334=ORIENTED_EDGE ( 'NONE', *, *, #7996, .T. ) ;
#7339=CARTESIAN_POINT ( 'NONE',  ( -34.74740905761646559, 10.15745573515589228, -36.06853344480607149 ) ) ;
#7340=CARTESIAN_POINT ( 'NONE',  ( -96.46749073287921306, 29.92475971289336556, 86.95816172513350750 ) ) ;
#7341=ADVANCED_FACE ( 'NONE', ( #39766 ), #66178, .F. ) ;
#7342=CARTESIAN_POINT ( 'NONE',  ( -142.0902782307735208, 58.13494170555998863, 37.07437729448285779 ) ) ;
#7343=CARTESIAN_POINT ( 'NONE',  ( -132.6161619568759988, 51.08240647571220450, 61.62853753731319983 ) ) ;
#7344=CARTESIAN_POINT ( 'NONE',  ( -71.97658551692140350, 20.95070248419150261, -19.17076785925019777 ) ) ;
#7346=CARTESIAN_POINT ( 'NONE',  ( 80.16939877002756987, 17.31693935407226448, 67.89906232374367789 ) ) ;
#7349=CARTESIAN_POINT ( 'NONE',  ( 31.90217595456441302, 7.552213897210509508, 37.90790274029890128 ) ) ;
#7352=CARTESIAN_POINT ( 'NONE',  ( 181.0840389613909736, 78.60582251573003987, 44.30859410551141764 ) ) ;
#7354=VECTOR ( 'NONE', #23359, 1000.000000000000000 ) ;
#7356=CARTESIAN_POINT ( 'NONE',  ( -122.8011284400168250, 45.68452922414294193, 58.11634083775930293 ) ) ;
#7357=CARTESIAN_POINT ( 'NONE',  ( -53.13004807512037786, 14.17398740785108480, 18.23844739916169289 ) ) ;
#7358=CARTESIAN_POINT ( 'NONE',  ( 155.2910738464913152, 55.97560547655806573, -50.81481607110237775 ) ) ;
#7360=CARTESIAN_POINT ( 'NONE',  ( 160.5018603162735076, 61.33906090758085838, -77.34339245626459558 ) ) ;
#7364=CARTESIAN_POINT ( 'NONE',  ( -155.7433525314458791, 69.65452735858369238, -11.29319091142111375 ) ) ;
#7365=EDGE_LOOP ( 'NONE', ( #54260, #47878 ) ) ;
#7366=CARTESIAN_POINT ( 'NONE',  ( -7.825402957745087207, -170.0000000000000000, 37.61558103944720699 ) ) ;
#7371=CARTESIAN_POINT ( 'NONE',  ( -85.09761763353360209, 24.87634954265997678, 41.78514032919718346 ) ) ;
#7372=CARTESIAN_POINT ( 'NONE',  ( 151.3136733342016669, 54.26417151662143112, -66.17808903341922644 ) ) ;
#7373=CARTESIAN_POINT ( 'NONE',  ( 45.89232972084001005, 10.36128169546909916, 33.64739044171249560 ) ) ;
#7374=CARTESIAN_POINT ( 'NONE',  ( 141.3403471770512851, 46.13063628128488602, -44.08590368907992030 ) ) ;
#7381=CARTESIAN_POINT ( 'NONE',  ( -0.8863173716723049544, 7.545240407187534970, 13.64818108344007719 ) ) ;
#7382=CARTESIAN_POINT ( 'NONE',  ( -0.3740447803642787949, 7.527031846085009192, 63.47620538581821847 ) ) ;
#7384=FILL_AREA_STYLE ('',( #43944 ) ) ;
#7386=CARTESIAN_POINT ( 'NONE',  ( -125.8938041572051105, 46.49392987655492959, -76.75825448869764500 ) ) ;
#7388=CARTESIAN_POINT ( 'NONE',  ( 164.6499013411309420, 63.45576988183554334, -14.59376700924564219 ) ) ;
#7389=LINE ( 'NONE', #67188, #45152 ) ;
#7390=CARTESIAN_POINT ( 'NONE',  ( 63.49940197359693883, 12.78497925206076324, 56.65751152968497451 ) ) ;
#7393=ORIENTED_EDGE ( 'NONE', *, *, #11513, .F. ) ;
#7397=ORIENTED_EDGE ( 'NONE', *, *, #58407, .T. ) ;
#7399=CARTESIAN_POINT ( 'NONE',  ( 64.93224207568368911, 14.16036304753835218, 71.41255769891185423 ) ) ;
#7403=AXIS2_PLACEMENT_3D ( 'NONE', #41940, #22560, #12359 ) ;
#7404=VERTEX_POINT ( 'NONE', #35877 ) ;
#7406=CARTESIAN_POINT ( 'NONE',  ( 88.99522780200240391, 20.24180937454203999, 17.48863613379957371 ) ) ;
#7408=CARTESIAN_POINT ( 'NONE',  ( 164.6499013411307999, 63.45576988183551492, -41.43831759970928630 ) ) ;
#7415=CARTESIAN_POINT ( 'NONE',  ( 57.92895196976683536, 12.57818278445338755, 85.48064400023716303 ) ) ;
#7416=CARTESIAN_POINT ( 'NONE',  ( 36.99999522780156980, 9.122638774496635961, 30.30464867167598797 ) ) ;
#7417=VECTOR ( 'NONE', #60964, 1000.000000000000000 ) ;
#7419=CARTESIAN_POINT ( 'NONE',  ( -179.6145635655384183, 96.24253679848490606, -92.13970873418386986 ) ) ;
#7421=CARTESIAN_POINT ( 'NONE',  ( 132.0582325211145189, 40.34869848118184166, -63.07262740430937242 ) ) ;
#7422=VERTEX_POINT ( 'NONE', #34849 ) ;
#7423=CARTESIAN_POINT ( 'NONE',  ( 141.3586046882815594, 47.34625111366353423, -70.87675768225021500 ) ) ;
#7426=CARTESIAN_POINT ( 'NONE',  ( -156.4966862384868307, 71.70877417666511633, -39.54005476914262829 ) ) ;
#7428=CARTESIAN_POINT ( 'NONE',  ( -32.40928421737412179, 10.77259363352673383, 30.26336764027513482 ) ) ;
#7429=CARTESIAN_POINT ( 'NONE',  ( -168.7187482717113483, 82.35796501763486788, -48.30229039519385736 ) ) ;
#7430=CARTESIAN_POINT ( 'NONE',  ( -5.417282889646088506, 7.753782747238991746, 44.72272311776506371 ) ) ;
#7433=CARTESIAN_POINT ( 'NONE',  ( -52.45215874217874585, 13.99961488531758391, -76.59970130483547734 ) ) ;
#7434=CARTESIAN_POINT ( 'NONE',  ( -3.253130881186329759, 7.643323950922367160, -22.03867337319629627 ) ) ;
#7435=CARTESIAN_POINT ( 'NONE',  ( -14.56631729561072142, 8.434645566888205437, 40.94015154958498215 ) ) ;
#7436=CARTESIAN_POINT ( 'NONE',  ( 113.8748103246145433, 30.59837980920002209, 16.84643264326143708 ) ) ;
#7437=DIRECTION ( 'NONE',  ( 0.000000000000000000, -1.000000000000000000, 0.000000000000000000 ) ) ;
#7439=CARTESIAN_POINT ( 'NONE',  ( -95.86163447241557378, 30.75089131639703410, -46.42652761453075527 ) ) ;
#7441=CARTESIAN_POINT ( 'NONE',  ( 109.7724924842965777, 28.66436020578542099, -62.76698815611733551 ) ) ;
#7442=CARTESIAN_POINT ( 'NONE',  ( 45.89232972084000295, 10.36128169546909383, -20.04171073921484947 ) ) ;
#7443=CARTESIAN_POINT ( 'NONE',  ( 45.90693067088657386, 9.344800815249321602, 68.02348139506582925 ) ) ;
#7445=FACE_OUTER_BOUND ( 'NONE', #49043, .T. ) ;
#7448=CARTESIAN_POINT ( 'NONE',  ( -118.3918229753714968, 42.92682904595257298, -16.07878825854773552 ) ) ;
#7452=CARTESIAN_POINT ( 'NONE',  ( 181.0840389613909736, 78.60582251573006829, 71.15314469597512925 ) ) ;
#7455=CARTESIAN_POINT ( 'NONE',  ( 107.2614272668148914, 28.62909081796205868, 70.84170775330584036 ) ) ;
#7459=ORIENTED_EDGE ( 'NONE', *, *, #5767, .T. ) ;
#7460=CARTESIAN_POINT ( 'NONE',  ( 91.50468583833760761, 22.21368636549395958, 4.646999254352490283 ) ) ;
#7464=CARTESIAN_POINT ( 'NONE',  ( -14.32120159453989672, 7.401444311907543927, 60.70308768940526534 ) ) ;
#7465=CARTESIAN_POINT ( 'NONE',  ( -81.90020664963800812, 23.57971581008655804, -22.54224771583843534 ) ) ;
#7468=FACE_BOUND ( 'NONE', #43662, .T. ) ;
#7474=EDGE_CURVE ( 'NONE', #6290, #68152, #37550, .T. ) ;
#7476=CARTESIAN_POINT ( 'NONE',  ( 86.62931800182292363, 19.42108912189599224, -89.51066537983906812 ) ) ;
#7478=CARTESIAN_POINT ( 'NONE',  ( 32.90051628396145134, 8.664124555952431805, -73.73572960565718404 ) ) ;
#7479=FACE_OUTER_BOUND ( 'NONE', #46124, .T. ) ;
#7480=CARTESIAN_POINT ( 'NONE',  ( 156.5977259323289275, 56.97512126940429766, 2.602768280174560633 ) ) ;
#7483=CARTESIAN_POINT ( 'NONE',  ( 58.47673920847984164, 11.66523265296355483, 4.477951416689838204 ) ) ;
#7484=CARTESIAN_POINT ( 'NONE',  ( 198.7129816317745679, 100.1061386900355785, -39.29776229674419596 ) ) ;
#7490=CARTESIAN_POINT ( 'NONE',  ( 94.11733320392092139, 23.18939451097131155, -70.65979286123472036 ) ) ;
#7493=EDGE_CURVE ( 'NONE', #40620, #6748, #58952, .T. ) ;
#7496=CARTESIAN_POINT ( 'NONE',  ( 161.7031777507227162, 62.31724004902782355, 43.11786657228953601 ) ) ;
#7500=EDGE_LOOP ( 'NONE', ( #22265, #17521, #54700, #58872 ) ) ;
#7502=CARTESIAN_POINT ( 'NONE',  ( -52.00092620775819796, 14.92276858858357258, -49.57163614092388570 ) ) ;
#7504=CARTESIAN_POINT ( 'NONE',  ( -54.56685407443680447, 15.59259313022788440, 18.47277718246750311 ) ) ;
#7505=CARTESIAN_POINT ( 'NONE',  ( -15.15117926080556465, 8.490099586177995761, -95.00000000000133582 ) ) ;
#7506=CARTESIAN_POINT ( 'NONE',  ( -155.6741333259783460, 70.95299863499437265, -91.72665331470490457 ) ) ;
#7508=CARTESIAN_POINT ( 'NONE',  ( 84.09769155791593676, 18.57180883336368638, 83.81111254107904074 ) ) ;
#7511=VERTEX_POINT ( 'NONE', #11113 ) ;
#7514=CARTESIAN_POINT ( 'NONE',  ( 46.41758729921141935, 9.425975226414244901, 7.906304787334934581 ) ) ;
#7515=CARTESIAN_POINT ( 'NONE',  ( -177.7741424253921707, 94.02182498476740591, 86.12237327923784846 ) ) ;
#7516=CARTESIAN_POINT ( 'NONE',  ( -47.95193882091085413, 12.89180642785319542, -18.33614611382470017 ) ) ;
#7517=CARTESIAN_POINT ( 'NONE',  ( 106.0171289417044136, 26.97542621030655852, -10.37713856442654503 ) ) ;
#7518=CARTESIAN_POINT ( 'NONE',  ( -130.2071229607963119, 50.62285182196875866, 44.27336784337931164 ) ) ;
#7519=CARTESIAN_POINT ( 'NONE',  ( 200.4600337307565496, 100.7087439352121123, 16.06857715856459734 ) ) ;
#7520=CARTESIAN_POINT ( 'NONE',  ( 209.7104118037933347, 115.2827355935552873, 84.81015762066461150 ) ) ;
#7522=CARTESIAN_POINT ( 'NONE',  ( -73.63346300764936814, 20.46798018699518806, -75.02584359677265979 ) ) ;
#7524=EDGE_LOOP ( 'NONE', ( #62360, #26646, #4807, #34209 ) ) ;
#7526=CARTESIAN_POINT ( 'NONE',  ( 12.03162622199373288, 7.415834979634795765, -9.678397900994031744 ) ) ;
#7529=CARTESIAN_POINT ( 'NONE',  ( -146.7404675333697810, 63.17262273741977907, 18.35075481789837681 ) ) ;
#7534=DIRECTION ( 'NONE',  ( -0.000000000000000000, 1.000000000000000000, -0.000000000000000000 ) ) ;
#7535=CARTESIAN_POINT ( 'NONE',  ( 140.0820590176526252, 46.51134312115245706, -20.86892350826419573 ) ) ;
#7536=ORIENTED_EDGE ( 'NONE', *, *, #62668, .T. ) ;
#7539=CARTESIAN_POINT ( 'NONE',  ( -9.771516655894551207, 7.025139475821123192, 3.511394494525364784 ) ) ;
#7541=CARTESIAN_POINT ( 'NONE',  ( 58.47673920847984874, 11.66523265296357614, -22.36659917377383522 ) ) ;
#7542=CARTESIAN_POINT ( 'NONE',  ( -47.95193882091083992, 12.89180642785318653, 35.35295506710262714 ) ) ;
#7543=CARTESIAN_POINT ( 'NONE',  ( 203.9203998321607685, 106.9845510704142271, 71.02229316225890443 ) ) ;
#7546=LINE ( 'NONE', #39204, #27864 ) ;
#7547=CARTESIAN_POINT ( 'NONE',  ( 179.4207200232661137, 76.93724985992176357, -63.20564937983176890 ) ) ;
#7551=CARTESIAN_POINT ( 'NONE',  ( -167.0043730366751902, 80.56812533391482134, -91.53196777109012316 ) ) ;
#7554=CARTESIAN_POINT ( 'NONE',  ( -189.5883860598227670, 107.5728846252917066, 94.41119403186252157 ) ) ;
#7555=EDGE_CURVE ( 'NONE', #50199, #22455, #66118, .T. ) ;
#7556=CIRCLE ( 'NONE', #14274, 243.4957430088094839 ) ;
#7557=EDGE_CURVE ( 'NONE', #37405, #15400, #40924, .T. ) ;
#7563=CARTESIAN_POINT ( 'NONE',  ( -128.9786047358386440, 48.55852351614670681, -62.41807552428025474 ) ) ;
#7564=DIRECTION ( 'NONE',  ( 0.000000000000000000, 0.000000000000000000, 1.000000000000000000 ) ) ;
#7567=AXIS2_PLACEMENT_3D ( 'NONE', #3164, #56974, #8791 ) ;
#7570=CARTESIAN_POINT ( 'NONE',  ( -188.6739852773920347, 108.2139733222100517, 13.28364116741142809 ) ) ;
#7571=CARTESIAN_POINT ( 'NONE',  ( 175.7669052691647664, 73.39379665792895935, 85.19702012587089257 ) ) ;
#7575=CYLINDRICAL_SURFACE ( 'NONE', #3848, 7.500000000000013323 ) ;
#7576=CARTESIAN_POINT ( 'NONE',  ( 150.2805372522807090, 53.51147386362156055, 39.06112697484593355 ) ) ;
#7579=ORIENTED_EDGE ( 'NONE', *, *, #40483, .F. ) ;
#7581=CARTESIAN_POINT ( 'NONE',  ( -177.1540936177023298, 91.73126115633627364, 5.138615071113800781 ) ) ;
#7582=CARTESIAN_POINT ( 'NONE',  ( -55.05276343752910151, -170.0000000000000000, 10.97277718246748890 ) ) ;
#7583=CARTESIAN_POINT ( 'NONE',  ( -78.66644367742111399, 23.39876645725287219, 30.41820113967310490 ) ) ;
#7584=CARTESIAN_POINT ( 'NONE',  ( -26.88635117726413526, 9.904687797303056485, -9.992545258014629894 ) ) ;
#7585=CARTESIAN_POINT ( 'NONE',  ( -54.08488990389050599, 15.46443908526321565, -23.32469389829597617 ) ) ;
#7588=DIRECTION ( 'NONE',  ( -0.000000000000000000, 1.000000000000000000, -0.000000000000000000 ) ) ;
#7591=CARTESIAN_POINT ( 'NONE',  ( -127.9171280854046699, 47.84023031960693118, 84.58149700715385677 ) ) ;
#7593=CARTESIAN_POINT ( 'NONE',  ( 82.13067365723604496, 17.93447087949267527, -49.34213147692616275 ) ) ;
#7595=CARTESIAN_POINT ( 'NONE',  ( -148.4259959918497884, 63.26767374754764717, 72.49016198256882149 ) ) ;
#7596=VECTOR ( 'NONE', #28483, 1000.000000000000000 ) ;
#7597=CARTESIAN_POINT ( 'NONE',  ( 84.27937148876357298, 19.69225537006224513, 30.08568434253633228 ) ) ;
#7598=CARTESIAN_POINT ( 'NONE',  ( -38.02163356681019479, 10.76490728754187032, 94.99999999999866418 ) ) ;
#7599=CARTESIAN_POINT ( 'NONE',  ( 188.4904153916304779, 86.42965364612511792, -18.09992457417106237 ) ) ;
#7600=CARTESIAN_POINT ( 'NONE',  ( 141.3403471770513420, 46.13063628128487892, -17.24135309861619803 ) ) ;
#7602=CYLINDRICAL_SURFACE ( 'NONE', #44338, 7.500000000000027534 ) ;
#7603=CARTESIAN_POINT ( 'NONE',  ( 19.03725708678846118, 7.633457022989709628, -89.93545773326505355 ) ) ;
#7604=CARTESIAN_POINT ( 'NONE',  ( -155.6759163077703363, 69.59305396324219828, -91.70819391566057277 ) ) ;
#7605=ORIENTED_EDGE ( 'NONE', *, *, #31141, .F. ) ;
#7608=CARTESIAN_POINT ( 'NONE',  ( 105.8022841538863901, 26.88074187880707910, 57.89262865156256055 ) ) ;
#7616=CARTESIAN_POINT ( 'NONE',  ( -108.1144194775597498, 35.84457139767600609, 60.12441792465978807 ) ) ;
#7624=FACE_OUTER_BOUND ( 'NONE', #448, .T. ) ;
#7625=CARTESIAN_POINT ( 'NONE',  ( -83.12901536265223967, 24.07178615860086168, 70.79554670785140047 ) ) ;
#7626=CARTESIAN_POINT ( 'NONE',  ( 126.7877523219522971, 38.47018873135922945, 39.57023082146568527 ) ) ;
#7628=CARTESIAN_POINT ( 'NONE',  ( 181.0840389613909736, 80.03940679743416808, 29.30859410551139277 ) ) ;
#7630=CARTESIAN_POINT ( 'NONE',  ( 34.84173759613682364, 7.859847277726514925, 70.23282494151600019 ) ) ;
#7633=CARTESIAN_POINT ( 'NONE',  ( -6.851003965218993130, 6.829052369041588300, -50.37077420520065374 ) ) ;
#7636=EDGE_CURVE ( 'NONE', #54401, #31358, #61841, .T. ) ;
#7637=CARTESIAN_POINT ( 'NONE',  ( -142.8450945664715164, 58.72815783657286914, 14.83098911521528862 ) ) ;
#7639=CARTESIAN_POINT ( 'NONE',  ( -109.7647482398635503, 36.74843029291201901, -68.81159568595916198 ) ) ;
#7641=CARTESIAN_POINT ( 'NONE',  ( 128.0540543950622521, 39.18660671946769014, -11.90031528999368504 ) ) ;
#7642=ORIENTED_EDGE ( 'NONE', *, *, #62280, .F. ) ;
#7646=CARTESIAN_POINT ( 'NONE',  ( -32.40928421737412890, 10.77259363352673205, -50.27028413111590055 ) ) ;
#7648=CARTESIAN_POINT ( 'NONE',  ( -171.2728242145607283, 85.09337373898185319, 84.72424543254817308 ) ) ;
#7650=CARTESIAN_POINT ( 'NONE',  ( -118.9649285217356010, 42.09781191014327817, -45.29594997475566487 ) ) ;
#7651=CARTESIAN_POINT ( 'NONE',  ( -144.2188519266540254, 59.82027639618912929, -20.79196203645875940 ) ) ;
#7655=CARTESIAN_POINT ( 'NONE',  ( 151.5196126176748805, 54.41511917384920594, 86.02076705022442127 ) ) ;
#7656=EDGE_CURVE ( 'NONE', #50694, #18800, #36054, .T. ) ;
#7663=CARTESIAN_POINT ( 'NONE',  ( 18.89064107370902690, 6.619789970027398773, -36.18630582809151264 ) ) ;
#7666=CARTESIAN_POINT ( 'NONE',  ( 57.39674746172461539, 11.43903079040058834, 42.30479512360005856 ) ) ;
#7668=VERTEX_POINT ( 'NONE', #57850 ) ;
#7670=CARTESIAN_POINT ( 'NONE',  ( 174.1422537179815038, 73.24254491731254291, 33.95503749249008507 ) ) ;
#7671=CARTESIAN_POINT ( 'NONE',  ( 23.09784929786603414, 6.844738137842331760, -68.16647883290328025 ) ) ;
#7672=CARTESIAN_POINT ( 'NONE',  ( -12.77550690612892659, 8.273784096785062658, -75.41817604663297914 ) ) ;
#7673=ORIENTED_EDGE ( 'NONE', *, *, #59054, .T. ) ;
#7677=EDGE_LOOP ( 'NONE', ( #51285, #13075 ) ) ;
#7678=CARTESIAN_POINT ( 'NONE',  ( 210.9631450001601252, 117.1791136960929265, -74.83007442223710370 ) ) ;
#7680=CARTESIAN_POINT ( 'NONE',  ( 153.9530329262830435, 54.96668088430648424, -90.67854091719155463 ) ) ;
#7681=CARTESIAN_POINT ( 'NONE',  ( -127.6881387055492922, 48.89937523111242967, 3.989620345208920504 ) ) ;
#7690=LINE ( 'NONE', #23520, #39296 ) ;
#7691=CARTESIAN_POINT ( 'NONE',  ( -142.8450945664714880, 58.72815783657286204, 41.67553970567896471 ) ) ;
#7692=CARTESIAN_POINT ( 'NONE',  ( 86.62931800182293784, 19.42108912189599579, -62.66611478937537782 ) ) ;
#7693=CARTESIAN_POINT ( 'NONE',  ( -75.43271753227887189, 22.18711452892410918, -8.986709910220804787 ) ) ;
#7696=ORIENTED_EDGE ( 'NONE', *, *, #35097, .F. ) ;
#7698=ADVANCED_FACE ( 'NONE', ( #31464 ), #4389, .F. ) ;
#7699=CARTESIAN_POINT ( 'NONE',  ( 31.95008798096001712, 7.556925044648907352, 38.39634584779201987 ) ) ;
#7704=CARTESIAN_POINT ( 'NONE',  ( -102.2801239173131052, 32.78103895658058065, 72.36362509687883460 ) ) ;
#7705=CARTESIAN_POINT ( 'NONE',  ( -120.4666325602656087, 44.20829586446608772, 59.78203764639147266 ) ) ;
#7706=CARTESIAN_POINT ( 'NONE',  ( -7.825402957745081878, 7.899365992529270741, -50.41807073194384259 ) ) ;
#7713=CARTESIAN_POINT ( 'NONE',  ( -58.32502757340552080, 16.62877055630751499, 57.89620646628114287 ) ) ;
#7714=CARTESIAN_POINT ( 'NONE',  ( 39.40195752203892710, -170.0000000000000000, 91.10293548689062959 ) ) ;
#7718=CARTESIAN_POINT ( 'NONE',  ( 150.0278556977734752, 53.32860603304212077, -69.39036461173597559 ) ) ;
#7719=CARTESIAN_POINT ( 'NONE',  ( -36.37371824399144060, 10.45334302951138739, 32.04685305616742852 ) ) ;
#7720=EDGE_CURVE ( 'NONE', #52493, #3111, #52900, .T. ) ;
#7721=CARTESIAN_POINT ( 'NONE',  ( 141.2366329129480675, 46.06278879703612006, -44.88589907137630064 ) ) ;
#7722=EDGE_CURVE ( 'NONE', #5837, #45785, #53480, .T. ) ;
#7723=EDGE_LOOP ( 'NONE', ( #48333, #42067, #60467, #8377 ) ) ;
#7726=CARTESIAN_POINT ( 'NONE',  ( 32.15613847490628530, 8.588587416860168133, -18.22703462462936486 ) ) ;
#7728=CARTESIAN_POINT ( 'NONE',  ( -156.9402586331177361, -170.0000000000000000, -95.00000000000133582 ) ) ;
#7729=CARTESIAN_POINT ( 'NONE',  ( 88.98408042523108463, 20.23787745328938215, 56.93183881311599492 ) ) ;
#7730=DIRECTION ( 'NONE',  ( -0.000000000000000000, 1.000000000000000000, -0.000000000000000000 ) ) ;
#7735=CARTESIAN_POINT ( 'NONE',  ( 159.2389084450350083, 59.03884018680377466, -9.477483402660668688 ) ) ;
#7737=CARTESIAN_POINT ( 'NONE',  ( 70.26722489419888973, 14.47234958177329389, 62.17998598294791890 ) ) ;
#7738=CARTESIAN_POINT ( 'NONE',  ( 139.1353280997809634, 44.70436000187871883, -65.03450818519148413 ) ) ;
#7742=ORIENTED_EDGE ( 'NONE', *, *, #31957, .T. ) ;
#7745=CARTESIAN_POINT ( 'NONE',  ( 162.0812592823604916, 62.62783216273700049, -10.84498442540020413 ) ) ;
#7746=CARTESIAN_POINT ( 'NONE',  ( 8.540853903193188046, 6.376814430361483765, 39.46023411190206787 ) ) ;
#7748=CARTESIAN_POINT ( 'NONE',  ( 63.99027454648602031, 13.93445177372598742, 56.70534288924221755 ) ) ;
#7749=CARTESIAN_POINT ( 'NONE',  ( 128.9313283535441599, 38.52887643767397918, -91.54200002570384243 ) ) ;
#7752=CARTESIAN_POINT ( 'NONE',  ( 158.3636111008086687, 59.62671916656142201, -36.12418429913763163 ) ) ;
#7753=CARTESIAN_POINT ( 'NONE',  ( -149.5074843970971017, 65.50121172469319220, -22.96827994102830317 ) ) ;
#7760=CARTESIAN_POINT ( 'NONE',  ( 33.31166872005966439, 8.707041209322246900, 33.02990241366695301 ) ) ;
#7761=CARTESIAN_POINT ( 'NONE',  ( 84.27937148876361562, 19.69225537006224869, -23.60341683839102345 ) ) ;
#7762=CARTESIAN_POINT ( 'NONE',  ( -130.5740389938243027, 49.65308610043482673, -9.689013956004959738 ) ) ;
#7763=CARTESIAN_POINT ( 'NONE',  ( 35.45122521384750058, 8.940329117834592054, -90.37916076915726649 ) ) ;
#7764=CARTESIAN_POINT ( 'NONE',  ( 131.6005058089755266, 40.07838125795769457, -77.53578642827864087 ) ) ;
#7769=CARTESIAN_POINT ( 'NONE',  ( -155.2836587093739524, 70.59655508952971559, -47.10335330728528902 ) ) ;
#7771=CARTESIAN_POINT ( 'NONE',  ( -38.16652041892307778, 11.81761816422916311, 34.36470182406579710 ) ) ;
#7772=CARTESIAN_POINT ( 'NONE',  ( -0.8863172752569277169, 7.545240277686256825, 40.49273171542998284 ) ) ;
#7774=CARTESIAN_POINT ( 'NONE',  ( -55.05276343752909440, 14.68156374112638929, -77.06087458892358200 ) ) ;
#7776=CARTESIAN_POINT ( 'NONE',  ( -15.32495246574475267, 8.506829480038510027, 37.11362200784080301 ) ) ;
#7777=CARTESIAN_POINT ( 'NONE',  ( -62.49130718206700408, 16.80297926264071151, 9.982333063200602652 ) ) ;
#7780=CARTESIAN_POINT ( 'NONE',  ( -94.78138776532242105, 30.24234841992715417, -41.97853113865350139 ) ) ;
#7781=ORIENTED_EDGE ( 'NONE', *, *, #17137, .T. ) ;
#7783=CARTESIAN_POINT ( 'NONE',  ( 46.51679720856117228, 10.46086439153924097, -18.69848944342430030 ) ) ;
#7784=CARTESIAN_POINT ( 'NONE',  ( 46.89006465517228861, 9.501960077668741178, 64.74722328374446079 ) ) ;
#7786=CARTESIAN_POINT ( 'NONE',  ( -15.30839993758081263, 7.494375438621725394, 91.90590778965562890 ) ) ;
#7788=DIRECTION ( 'NONE',  ( 0.000000000000000000, 0.000000000000000000, 1.000000000000000000 ) ) ;
#7789=CARTESIAN_POINT ( 'NONE',  ( 63.01563776193090405, 13.70579113808096672, -89.40979201309708913 ) ) ;
#7792=ORIENTED_EDGE ( 'NONE', *, *, #33532, .T. ) ;
#7802=CARTESIAN_POINT ( 'NONE',  ( 59.94652978725889625, 13.01168383647462790, -9.528566960319547974 ) ) ;
#7805=CARTESIAN_POINT ( 'NONE',  ( 105.2529848321548229, 27.73895015262024089, -49.02683151908587433 ) ) ;
#7806=CARTESIAN_POINT ( 'NONE',  ( -14.94265033805045917, 7.459411036484910440, 62.04421683837972523 ) ) ;
#7807=CARTESIAN_POINT ( 'NONE',  ( 11.21312910819262321, 7.403355431336986037, 58.39587251282808467 ) ) ;
#7809=CARTESIAN_POINT ( 'NONE',  ( 211.8476521439973794, 116.6941316755177525, -14.69380237910506715 ) ) ;
#7810=FACE_BOUND ( 'NONE', #28442, .T. ) ;
#7815=CARTESIAN_POINT ( 'NONE',  ( -178.5750994113944614, 94.98114813978524751, 6.304711435512811768 ) ) ;
#7816=CARTESIAN_POINT ( 'NONE',  ( 210.0055645826033697, 115.7254585628714096, 58.23048686943388219 ) ) ;
#7820=ORIENTED_EDGE ( 'NONE', *, *, #55941, .T. ) ;
#7823=CARTESIAN_POINT ( 'NONE',  ( 199.3764173596862577, 100.9540560740992277, -49.13558951988117229 ) ) ;
#7828=CARTESIAN_POINT ( 'NONE',  ( -83.69653436244854561, 24.30167057287989962, -63.89149677819863626 ) ) ;
#7830=DIRECTION ( 'NONE',  ( -0.000000000000000000, 1.000000000000000000, -0.000000000000000000 ) ) ;
#7833=CARTESIAN_POINT ( 'NONE',  ( 46.23113030541875901, 10.41513832761375546, 67.36843900475240332 ) ) ;
#7835=CARTESIAN_POINT ( 'NONE',  ( -105.5471966583786099, 35.60982465102040351, -89.44928979052285456 ) ) ;
#7836=CARTESIAN_POINT ( 'NONE',  ( 110.2429982417149574, 29.99119854320843714, 17.76666361527367499 ) ) ;
#7839=CARTESIAN_POINT ( 'NONE',  ( 59.72647370436681769, 12.96353798836694615, -36.47598787309180324 ) ) ;
#7840=CARTESIAN_POINT ( 'NONE',  ( -13.74877239730504286, 8.359278534280710105, -91.92798095535714253 ) ) ;
#7841=CARTESIAN_POINT ( 'NONE',  ( 111.1868021579656869, 29.32055685204858619, -9.122472411873387088 ) ) ;
#7842=B_SPLINE_CURVE_WITH_KNOTS ( 'NONE', 3,
 ( #10268, #31730, #3284, #52500, #24742, #25783, #46177, #67651, #19447, #47210, #62365, #14180, #57093, #8906, #51810, #25088, #46525, #43654, #21862, #53165, #405, #6022, #49276, #38391, #16587, #48570, #69364, #59141, #5674, #33127, #22217, #42629, #10611, #21183, #48923, #43305, #15898, #64086, #32430, #64429, #54199, #42958, #27137, #4997, #763, #53857 ),
 .UNSPECIFIED., .F., .F.,
 ( 4, 2, 2, 2, 2, 2, 2, 2, 2, 2, 2, 2, 2, 2, 2, 2, 2, 2, 2, 2, 2, 2, 4 ),
 ( 0.000000000000000000, 0.003373244802897216229, 0.004216556003621520395, 0.005059867204345824994, 0.006746489605794432458, 0.007589800806518737057, 0.008433112007243040789, 0.009276423207967343654, 0.01011973440869164999, 0.01180635681014026439, 0.01349297921158888053, 0.01433629041231318686, 0.01517960161303749493, 0.01686622401448609199, 0.01770953521521038618, 0.01855284641593467690, 0.02023946881738333120, 0.02108278001810763233, 0.02192609121883193346, 0.02361271362028053572, 0.02445602482100480909, 0.02529933602172908594, 0.02698595842317762922 ),
 .UNSPECIFIED. ) ;
#7844=CARTESIAN_POINT ( 'NONE',  ( 92.81079987519940744, 21.62352428699447771, 86.64070398657467820 ) ) ;
#7847=EDGE_LOOP ( 'NONE', ( #39035, #6466 ) ) ;
#7851=CARTESIAN_POINT ( 'NONE',  ( 46.76970795284344717, 9.482505412758841956, 12.03441307903643498 ) ) ;
#7852=DIRECTION ( 'NONE',  ( -0.000000000000000000, 1.000000000000000000, -0.000000000000000000 ) ) ;
#7853=CARTESIAN_POINT ( 'NONE',  ( -47.68742944762958302, 12.82957801017946409, -14.39326825997502901 ) ) ;
#7855=CARTESIAN_POINT ( 'NONE',  ( 198.7084915431530874, 98.47675983942194478, 5.340935046836625233 ) ) ;
#7856=CARTESIAN_POINT ( 'NONE',  ( 212.1850009103741570, 119.0680341029749485, 91.03128498463323126 ) ) ;
#7858=FACE_OUTER_BOUND ( 'NONE', #56705, .T. ) ;
#7859=CARTESIAN_POINT ( 'NONE',  ( -85.10909119100207931, 25.97025675005452072, 60.89070622084423690 ) ) ;
#7860=CARTESIAN_POINT ( 'NONE',  ( -14.76369756425703805, 7.442560416198674034, 40.49465273683735234 ) ) ;
#7861=EDGE_LOOP ( 'NONE', ( #16126, #1375 ) ) ;
#7863=CARTESIAN_POINT ( 'NONE',  ( 9.819093282782491272, 7.389085782749407194, -11.60726699437242715 ) ) ;
#7865=EDGE_LOOP ( 'NONE', ( #21923, #11913, #4394 ) ) ;
#7867=CARTESIAN_POINT ( 'NONE',  ( 188.0094179620990928, 87.39792407168457089, -73.46270491724961005 ) ) ;
#7868=CARTESIAN_POINT ( 'NONE',  ( -30.80792614961258380, 10.50774217500252483, 83.92525404607846440 ) ) ;
#7871=CARTESIAN_POINT ( 'NONE',  ( -31.43908319763710679, -170.0000000000000000, 64.56100499665288339 ) ) ;
#7872=CARTESIAN_POINT ( 'NONE',  ( 13.84704553156521456, 7.452804552247569880, -50.26752412725904406 ) ) ;
#7873=CARTESIAN_POINT ( 'NONE',  ( 132.0582325211144905, 40.34869848118183455, -36.22807681384569634 ) ) ;
#7876=CARTESIAN_POINT ( 'NONE',  ( 188.5503229283306439, 87.99928427996027835, 89.75865996300565541 ) ) ;
#7879=CARTESIAN_POINT ( 'NONE',  ( 59.08638499266954369, 11.79550614876704095, -22.76912641790571712 ) ) ;
#7880=ADVANCED_FACE ( 'NONE', ( #45130 ), #61315, .F. ) ;
#7888=CARTESIAN_POINT ( 'NONE',  ( -57.89360549284272395, 16.50663738101750511, -62.60719078153508121 ) ) ;
#7889=CARTESIAN_POINT ( 'NONE',  ( 198.7123879174244507, 100.1053816708572270, -75.19790834202754581 ) ) ;
#7892=CARTESIAN_POINT ( 'NONE',  ( -166.9969673948021693, 80.56076768517785069, 15.81477353917873785 ) ) ;
#7894=FACE_BOUND ( 'NONE', #26965, .T. ) ;
#7895=LINE ( 'NONE', #7193, #51248 ) ;
#7896=CARTESIAN_POINT ( 'NONE',  ( -6.840981040171499217, 6.828436339979226055, 71.91165652771135797 ) ) ;
#7899=CARTESIAN_POINT ( 'NONE',  ( 150.4722669492348359, 53.65054032737662482, 61.04279154623130665 ) ) ;
#7909=DIRECTION ( 'NONE',  ( 0.000000000000000000, 0.000000000000000000, 1.000000000000000000 ) ) ;
#7910=CARTESIAN_POINT ( 'NONE',  ( 149.9883446984744921, 53.30011109831374938, 36.32171926678490337 ) ) ;
#7914=CARTESIAN_POINT ( 'NONE',  ( -177.1539090641758207, 91.73101548694631902, 17.81618785780625558 ) ) ;
#7915=CARTESIAN_POINT ( 'NONE',  ( -0.3734056954813061990, 6.520221844775924147, 11.74911637933309372 ) ) ;
#7917=CARTESIAN_POINT ( 'NONE',  ( 55.64941011647476898, 12.11006142851271328, -41.74712242361913894 ) ) ;
#7918=CARTESIAN_POINT ( 'NONE',  ( -79.14094329813315198, 23.58034730000057877, 30.41820113967311201 ) ) ;
#7919=CARTESIAN_POINT ( 'NONE',  ( -26.88234027341226096, 9.904106450608203716, -21.94961641608552227 ) ) ;
#7920=CARTESIAN_POINT ( 'NONE',  ( 139.6359093656973300, 45.02518919224739591, 14.95245080739227994 ) ) ;
#7922=CARTESIAN_POINT ( 'NONE',  ( 117.7447573007802646, 32.50990724960316669, -42.93223025960289618 ) ) ;
#7923=CARTESIAN_POINT ( 'NONE',  ( -71.42007367207963853, 20.75704712149298814, 9.074083910195316349 ) ) ;
#7924=CARTESIAN_POINT ( 'NONE',  ( 41.35041461497704773, 8.670465437677199461, -35.86060275886635651 ) ) ;
#7926=CARTESIAN_POINT ( 'NONE',  ( -118.3864707679337016, 41.74547427441078895, 91.72959842008201292 ) ) ;
#7928=CARTESIAN_POINT ( 'NONE',  ( 83.37786665291103816, 18.33670623396829313, -36.54571592794794554 ) ) ;
#7929=EDGE_CURVE ( 'NONE', #3613, #32490, #29306, .T. ) ;
#7932=CARTESIAN_POINT ( 'NONE',  ( 79.18180043629686793, 18.06526831600444893, 36.19349848600327846 ) ) ;
#7934=CARTESIAN_POINT ( 'NONE',  ( 188.2133404574782958, 86.12414067617879709, -14.53428918749921017 ) ) ;
#7938=CARTESIAN_POINT ( 'NONE',  ( -173.5422248620772621, 89.11126078969417108, -7.867406574286299303 ) ) ;
#7944=CARTESIAN_POINT ( 'NONE',  ( 103.0103829243729052, 25.67737053862328978, 66.00548782892786903 ) ) ;
#7946=DIRECTION ( 'NONE',  ( 0.000000000000000000, 0.000000000000000000, 1.000000000000000000 ) ) ;
#7947=EDGE_CURVE ( 'NONE', #10403, #44678, #50066, .T. ) ;
#7948=CARTESIAN_POINT ( 'NONE',  ( 188.4359598230020367, 86.36951380984527304, -45.23692044763556197 ) ) ;
#7951=CARTESIAN_POINT ( 'NONE',  ( 157.9130201331580849, 57.99550255803047349, -77.96873488960136456 ) ) ;
#7954=ORIENTED_EDGE ( 'NONE', *, *, #20668, .F. ) ;
#7955=CARTESIAN_POINT ( 'NONE',  ( -78.66644367742111399, -170.0000000000000000, -50.11545063171791270 ) ) ;
#7956=CARTESIAN_POINT ( 'NONE',  ( -80.81202825120918476, 23.15032834068050249, 84.41426225767527569 ) ) ;
#7958=ADVANCED_FACE ( 'NONE', ( #7858 ), #50757, .F. ) ;
#7961=CARTESIAN_POINT ( 'NONE',  ( -60.64199216239839529, 17.30050036439947903, 32.81023052909118576 ) ) ;
#7964=CARTESIAN_POINT ( 'NONE',  ( 61.08522853873727598, 13.26388801693371455, 44.57671891123612795 ) ) ;
#7967=CARTESIAN_POINT ( 'NONE',  ( -1.857619870843145948, 6.575690665396235701, -38.34909718101288689 ) ) ;
#7969=CARTESIAN_POINT ( 'NONE',  ( -15.32584732649904247, 8.506915958926390076, 11.25943598086905872 ) ) ;
#7970=CARTESIAN_POINT ( 'NONE',  ( -148.4259959918497316, 63.26767374754767559, 18.80106080164143378 ) ) ;
#7972=CARTESIAN_POINT ( 'NONE',  ( 197.6145711261844724, 97.10888456119688783, 61.00577141233620182 ) ) ;
#7973=VECTOR ( 'NONE', #8628, 1000.000000000000000 ) ;
#7974=CARTESIAN_POINT ( 'NONE',  ( 130.3281282802763315, 40.49854652972194913, -23.31374654723702378 ) ) ;
#7975=B_SPLINE_CURVE_WITH_KNOTS ( 'NONE', 3,
 ( #11381, #42708, #32849, #21597, #38837, #37428, #49708, #43044, #15978, #28262, #32505, #38121, #16668, #64516, #60285, #846, #27218, #54286, #49009, #27920, #49358, #22298, #1191, #17358, #33568, #1539, #58879, #7868, #40220, #61669, #60629, #23696, #12445, #66969, #45487, #50077, #39868, #13827, #13487, #50766, #61326, #2249, #30014, #24047, #1907, #66619, #13151, #2587, #67317, #44806, #62009, #8563, #56745, #34948, #55700, #33905 ),
 .UNSPECIFIED., .F., .F.,
 ( 4, 2, 2, 2, 2, 2, 2, 2, 2, 2, 2, 2, 2, 2, 2, 2, 2, 2, 2, 1, 2, 2, 2, 2, 2, 2, 1, 2, 4 ),
 ( 0.000000000000000000, 0.001942337377849021095, 0.002913506066773531751, 0.003884674755698042190, 0.004855843444622553497, 0.005827012133547063502, 0.006798180822471573508, 0.007769349511396084380, 0.009711686889245072299, 0.01068285557816955368, 0.01165402426709403680, 0.01262519295601851992, 0.01359636164494300303, 0.01456753033386748615, 0.01553869902279196927, 0.01748103640064091469, 0.01845220508956538566, 0.01942337377848985316, 0.02039454246741432067, 0.02136571115633879164, 0.02233687984526325915, 0.02330804853418772665, 0.02525038591203665472, 0.02622155460096109794, 0.02719272328988554463, 0.02816389197880998785, 0.02913506066773443454, 0.03010622935665888122, 0.03107739804558332444 ),
 .UNSPECIFIED. ) ;
#7982=CARTESIAN_POINT ( 'NONE',  ( -172.0255068454375476, 85.91730236827989131, 84.58687643171798243 ) ) ;
#7984=CARTESIAN_POINT ( 'NONE',  ( 128.0882145863933772, 39.20607399008170546, 5.346544642291981120 ) ) ;
#7986=CARTESIAN_POINT ( 'NONE',  ( 201.5987353083856135, 103.8544727311227547, 3.019891354123939831 ) ) ;
#7987=CARTESIAN_POINT ( 'NONE',  ( 160.4971326318155604, 61.33565791516289778, 83.72971345548070587 ) ) ;
#7992=CARTESIAN_POINT ( 'NONE',  ( -102.2801239173131194, -170.0000000000000000, 57.36362509687880618 ) ) ;
#7993=CARTESIAN_POINT ( 'NONE',  ( 82.74007713545067588, 18.13042311233562742, 3.950172779682598723 ) ) ;
#7994=LINE ( 'NONE', #67442, #11765 ) ;
#7996=EDGE_CURVE ( 'NONE', #57426, #65931, #13813, .T. ) ;
#7999=ORIENTED_EDGE ( 'NONE', *, *, #11286, .F. ) ;
#8000=CARTESIAN_POINT ( 'NONE',  ( -168.1839487819771080, 83.25723186408066567, 17.12777191623586859 ) ) ;
#8002=CYLINDRICAL_SURFACE ( 'NONE', #10702, 7.500000000000013323 ) ;
#8004=CARTESIAN_POINT ( 'NONE',  ( -94.77617431038508755, 30.23990705277885382, 91.48307754187669616 ) ) ;
#8006=CARTESIAN_POINT ( 'NONE',  ( -25.79929641484369185, 9.749255553662436569, 32.74771463646250425 ) ) ;
#8008=ORIENTED_EDGE ( 'NONE', *, *, #15902, .T. ) ;
#8010=CARTESIAN_POINT ( 'NONE',  ( 212.1978255065450583, 119.0880569674902603, -70.32159165902619691 ) ) ;
#8011=EDGE_CURVE ( 'NONE', #4848, #60490, #46866, .T. ) ;
#8014=CARTESIAN_POINT ( 'NONE',  ( 140.4769819293527462, 46.76840769395177944, 33.47658864813747925 ) ) ;
#8015=CARTESIAN_POINT ( 'NONE',  ( 116.0963032583227772, 32.80867113471310148, 32.39564500324919294 ) ) ;
#8016=CARTESIAN_POINT ( 'NONE',  ( -132.5976199670998881, 52.30296609017644727, 7.902498531389648306 ) ) ;
#8017=CARTESIAN_POINT ( 'NONE',  ( 67.93154431625914924, 14.90489441944787785, -75.75106977084269033 ) ) ;
#8018=VERTEX_POINT ( 'NONE', #51800 ) ;
#8027=CARTESIAN_POINT ( 'NONE',  ( -133.1093894320205209, 51.43221067881453479, 62.84771461874985476 ) ) ;
#8028=CARTESIAN_POINT ( 'NONE',  ( -73.10086105983762650, 21.34631349770504016, -10.71955127705281896 ) ) ;
#8030=DIRECTION ( 'NONE',  ( -0.000000000000000000, 1.000000000000000000, -0.000000000000000000 ) ) ;
#8032=CARTESIAN_POINT ( 'NONE',  ( 37.70762885381311946, 8.195134395012281914, 44.72399686281225684 ) ) ;
#8034=VERTEX_POINT ( 'NONE', #20468 ) ;
#8035=CARTESIAN_POINT ( 'NONE',  ( 182.7789203043889756, 80.33475476315290109, 44.12694607665732605 ) ) ;
#8041=EDGE_CURVE ( 'NONE', #52276, #25055, #57623, .T. ) ;
#8042=CARTESIAN_POINT ( 'NONE',  ( 157.4703587214989113, 57.65129005721576760, -51.12418429913766005 ) ) ;
#8045=CARTESIAN_POINT ( 'NONE',  ( -154.6171773099879658, 68.63761944777706958, -9.973008346805338320 ) ) ;
#8048=CARTESIAN_POINT ( 'NONE',  ( -55.05276343752909440, 15.72344139423348430, 57.16187836339483397 ) ) ;
#8049=CYLINDRICAL_SURFACE ( 'NONE', #49921, 7.500000000000020428 ) ;
#8052=CARTESIAN_POINT ( 'NONE',  ( 39.40195752203891999, 9.424259417798145577, 18.06928371549960133 ) ) ;
#8053=CARTESIAN_POINT ( 'NONE',  ( -35.99019277275120743, 10.38248800679342132, 43.69771462296589704 ) ) ;
#8054=CARTESIAN_POINT ( 'NONE',  ( 139.1353280997809634, 44.70436000187871173, -38.18995759472777252 ) ) ;
#8057=CARTESIAN_POINT ( 'NONE',  ( -150.3831389294225858, 66.25266777263978213, 57.61345155406902308 ) ) ;
#8060=FACE_OUTER_BOUND ( 'NONE', #47092, .T. ) ;
#8061=CARTESIAN_POINT ( 'NONE',  ( 182.7789203043889756, 80.33475476315292951, 17.28239548619366062 ) ) ;
#8063=CARTESIAN_POINT ( 'NONE',  ( 87.58098510096635891, 19.74745174099416545, 56.60179672011121710 ) ) ;
#8071=CARTESIAN_POINT ( 'NONE',  ( -149.5074843970971017, 65.50121172469319220, 30.72082123989904545 ) ) ;
#8073=CARTESIAN_POINT ( 'NONE',  ( 70.46452034227868921, 14.52462608639673292, 63.15238888589277622 ) ) ;
#8074=CARTESIAN_POINT ( 'NONE',  ( 139.1306635769909690, 45.89653412152166823, 4.827772763954556901 ) ) ;
#8079=CARTESIAN_POINT ( 'NONE',  ( 163.1370549780984049, 63.50181104276887822, -21.71851364603849532 ) ) ;
#8080=CARTESIAN_POINT ( 'NONE',  ( 8.336031647119270360, 6.376437040857335425, 38.49332896737825394 ) ) ;
#8083=CARTESIAN_POINT ( 'NONE',  ( 65.40383840050411379, 14.27443447873227278, 57.03128338250952112 ) ) ;
#8084=CARTESIAN_POINT ( 'NONE',  ( 126.3606262338561379, 37.07877897843705028, 90.26304925273296931 ) ) ;
#8086=CARTESIAN_POINT ( 'NONE',  ( -146.5268141329886760, 61.69196909035589726, -62.27134214804291901 ) ) ;
#8089=CARTESIAN_POINT ( 'NONE',  ( 175.0857681883884140, -170.0000000000000000, 94.99999999999866418 ) ) ;
#8091=CARTESIAN_POINT ( 'NONE',  ( -96.77705718164448001, 31.18700926299571563, 16.29415678444673787 ) ) ;
#8092=EDGE_CURVE ( 'NONE', #16646, #35238, #29964, .T. ) ;
#8094=CARTESIAN_POINT ( 'NONE',  ( 58.70125406583569827, 12.74196547173361616, 84.85832636372359161 ) ) ;
#8096=CARTESIAN_POINT ( 'NONE',  ( 85.68197636629476222, 20.16141071296263121, -23.93233960346654143 ) ) ;
#8097=CARTESIAN_POINT ( 'NONE',  ( -171.4867114763004849, 85.32693843184998173, 30.99019746422447241 ) ) ;
#8098=CARTESIAN_POINT ( 'NONE',  ( -142.0747101610765242, 58.12276061064464017, -95.00000000000133582 ) ) ;
#8099=CARTESIAN_POINT ( 'NONE',  ( 127.1040286383415321, 37.49395136275127527, -73.64177352694797207 ) ) ;
#8100=ADVANCED_FACE ( 'NONE', ( #15550 ), #58440, .F. ) ;
#8103=CARTESIAN_POINT ( 'NONE',  ( -15.27733754929849752, 8.502213909106947298, 65.43888028898012976 ) ) ;
#8107=CARTESIAN_POINT ( 'NONE',  ( -156.0209085498131856, 71.27066046086520146, -46.06989554857462110 ) ) ;
#8109=CARTESIAN_POINT ( 'NONE',  ( -33.12994257348896809, 10.89587983539684934, 30.40543924679923293 ) ) ;
#8111=CARTESIAN_POINT ( 'NONE',  ( -2.873329055852806402, 7.626065826870668474, 31.96118308163061528 ) ) ;
#8113=CARTESIAN_POINT ( 'NONE',  ( -53.14475157111026249, 14.17819596930906734, -76.81816462347461538 ) ) ;
#8114=CARTESIAN_POINT ( 'NONE',  ( -0.8863172752569271617, 7.545240277686256825, -13.19636946549736045 ) ) ;
#8116=CARTESIAN_POINT ( 'NONE',  ( 174.1251613516844543, 71.84747073139210727, 12.81514609272755045 ) ) ;
#8118=CARTESIAN_POINT ( 'NONE',  ( 110.2429982417149432, 28.88204397445229432, 17.76666361527367499 ) ) ;
#8120=CARTESIAN_POINT ( 'NONE',  ( -94.77890319529974761, 30.24118571794804566, -43.01465426540235626 ) ) ;
#8122=CARTESIAN_POINT ( 'NONE',  ( 110.2429982417149290, 28.88204397445231209, -77.76698815611739235 ) ) ;
#8125=CARTESIAN_POINT ( 'NONE',  ( 41.09671232177016265, 8.635892912882342287, 56.94825200755940386 ) ) ;
#8127=CARTESIAN_POINT ( 'NONE',  ( -15.32317988097521066, 7.495800589904738409, 90.93220421695207278 ) ) ;
#8136=ORIENTED_EDGE ( 'NONE', *, *, #40268, .T. ) ;
#8139=CARTESIAN_POINT ( 'NONE',  ( 41.44400078756287797, 8.683588207969460626, -89.58023771676421632 ) ) ;
#8142=CARTESIAN_POINT ( 'NONE',  ( 62.52762183777210936, 13.59210632617625691, -8.876140241706057310 ) ) ;
#8144=CARTESIAN_POINT ( 'NONE',  ( 108.3753929817421522, 29.13179266688723956, -36.14330376477542472 ) ) ;
#8145=CARTESIAN_POINT ( 'NONE',  ( -9.771516655894554759, 7.025139475821123192, 57.20049567545273561 ) ) ;
#8146=CARTESIAN_POINT ( 'NONE',  ( -83.52505811737952968, 24.23179517241435121, -21.50563568346970200 ) ) ;
#8148=CARTESIAN_POINT ( 'NONE',  ( 13.72076016085272165, 6.443109411582633506, -89.48629928841640435 ) ) ;
#8150=ORIENTED_EDGE ( 'NONE', *, *, #52893, .F. ) ;
#8156=CARTESIAN_POINT ( 'NONE',  ( 63.98009977735162579, 12.89803120691696137, 29.85932659275067280 ) ) ;
#8157=B_SPLINE_CURVE_WITH_KNOTS ( 'NONE', 3,
 ( #1101, #60879, #17983, #44349, #23264, #23609, #34521, #33809, #22552, #66531, #54548, #17628, #27829, #39777, #43995, #18321, #12702, #65474, #6375, #61238, #28886, #38739, #60183, #7776, #34167, #12002, #49618, #44712, #33476, #54898, #7435, #29228, #6722, #66190, #7072, #28167, #1449, #28530, #39427, #55964, #16918, #50338, #50674, #38381, #2497 ),
 .UNSPECIFIED., .F., .F.,
 ( 4, 2, 2, 1, 2, 2, 2, 2, 2, 2, 2, 2, 2, 2, 2, 2, 2, 2, 2, 2, 2, 2, 4 ),
 ( 0.02346464386237015476, 0.02493212228186625704, 0.02566586149161431338, 0.02639960070136236625, 0.02713333991111042259, 0.02786707912085847547, 0.02933455754035457080, 0.03006829675010262715, 0.03080203595985068349, 0.03226951437934681005, 0.03300325358909486639, 0.03373699279884292274, 0.03520447121833903542, 0.03667194963783514117, 0.03740568884758319751, 0.03813942805733125385, 0.03960690647682735960, 0.04107438489632346534, 0.04254186331581957803, 0.04327560252556764131, 0.04400934173531570459, 0.04547682015481182422, 0.04694429857430795078 ),
 .UNSPECIFIED. ) ;
#8159=AXIS2_PLACEMENT_3D ( 'NONE', #1440, #2488, #55239 ) ;
#8166=VERTEX_POINT ( 'NONE', #17265 ) ;
#8167=EDGE_CURVE ( 'NONE', #60768, #21955, #8157, .T. ) ;
#8168=CARTESIAN_POINT ( 'NONE',  ( -81.23297981660239486, 23.31577157498399444, -62.40870875688570862 ) ) ;
#8169=CARTESIAN_POINT ( 'NONE',  ( -62.15063206372445848, 17.75106610013994413, -18.34472482884989120 ) ) ;
#8170=CARTESIAN_POINT ( 'NONE',  ( 94.06416612695404922, 23.16920323269610549, -69.14766088501639274 ) ) ;
#8174=EDGE_LOOP ( 'NONE', ( #10388, #33885, #65037, #5269 ) ) ;
#8175=CARTESIAN_POINT ( 'NONE',  ( 13.84937401517046673, 6.446378549072246500, -35.76972009710845413 ) ) ;
#8176=CARTESIAN_POINT ( 'NONE',  ( -107.6612349940556328, 36.74343276704001937, -90.96034172286037744 ) ) ;
#8180=ADVANCED_FACE ( 'NONE', ( #14087 ), #35546, .F. ) ;
#8184=CARTESIAN_POINT ( 'NONE',  ( -102.2801239173131194, 32.78103895658057354, 18.67452391595144334 ) ) ;
#8186=ADVANCED_FACE ( 'NONE', ( #30616 ), #62628, .F. ) ;
#8187=CARTESIAN_POINT ( 'NONE',  ( 79.19119222799088220, 18.06817527909835164, -42.32747752434355704 ) ) ;
#8188=CARTESIAN_POINT ( 'NONE',  ( -167.3106824190689110, 82.33819578244379045, -91.13552483532193094 ) ) ;
#8191=EDGE_CURVE ( 'NONE', #48198, #41404, #48356, .T. ) ;
#8193=CARTESIAN_POINT ( 'NONE',  ( 46.65037935242575884, 9.463293687292228640, 12.51126093126612027 ) ) ;
#8194=CARTESIAN_POINT ( 'NONE',  ( -31.43908319763710679, -170.0000000000000000, -89.00629854612920155 ) ) ;
#8196=CARTESIAN_POINT ( 'NONE',  ( 102.8111940033034415, 25.59308899183601937, -15.53619449273017494 ) ) ;
#8197=CARTESIAN_POINT ( 'NONE',  ( 197.9847015768255574, 97.56951352050457160, 13.21957474342690553 ) ) ;
#8198=CARTESIAN_POINT ( 'NONE',  ( -29.75098818128877198, 9.320063824353118420, -89.18649209667817956 ) ) ;
#8199=CARTESIAN_POINT ( 'NONE',  ( 210.5761663949224101, 116.5895149528252404, 85.72674437253323276 ) ) ;
#8200=CARTESIAN_POINT ( 'NONE',  ( 212.1978255065450583, 119.0880569674902461, 37.05661070282843639 ) ) ;
#8201=CARTESIAN_POINT ( 'NONE',  ( -83.69370847062542396, 25.38703975185373807, 59.19179572676554102 ) ) ;
#8202=CARTESIAN_POINT ( 'NONE',  ( -12.39701069459753846, 7.231688578592714300, 31.64994337550934489 ) ) ;
#8208=CARTESIAN_POINT ( 'NONE',  ( -143.2498117110515352, 60.33382252735061257, 7.233766551320602645 ) ) ;
#8211=CARTESIAN_POINT ( 'NONE',  ( -168.0052514572427071, 83.06849406765624622, 43.81149462059376276 ) ) ;
#8212=CARTESIAN_POINT ( 'NONE',  ( -95.04120270830171080, 29.25306318840326725, -40.48597676605763951 ) ) ;
#8214=CARTESIAN_POINT ( 'NONE',  ( -23.95089599695170079, 9.496585844566176604, 10.38338860445121625 ) ) ;
#8219=CARTESIAN_POINT ( 'NONE',  ( 128.3856248084844651, 38.21741401878866640, -48.67688400636009760 ) ) ;
#8220=EDGE_LOOP ( 'NONE', ( #22699, #19585, #50468, #64923 ) ) ;
#8223=CARTESIAN_POINT ( 'NONE',  ( 188.4752958934330707, 87.91563303859531686, 91.78575244328496296 ) ) ;
#8226=AXIS2_PLACEMENT_3D ( 'NONE', #27507, #21882, #63776 ) ;
#8227=CARTESIAN_POINT ( 'NONE',  ( -24.70354720400821691, 8.582324684301861240, -66.32597363807256841 ) ) ;
#8231=CARTESIAN_POINT ( 'NONE',  ( -62.55320287144887459, 17.87319849854531029, -69.32330422822633409 ) ) ;
#8232=CARTESIAN_POINT ( 'NONE',  ( 198.2581645178919132, 99.52881771501682806, -66.81519542867474115 ) ) ;
#8236=CARTESIAN_POINT ( 'NONE',  ( -24.32776401346968598, 9.546905915310563984, 66.99408005789631204 ) ) ;
#8238=CARTESIAN_POINT ( 'NONE',  ( -54.09522495088362604, 14.42642983673692036, 57.20752439395842259 ) ) ;
#8239=CARTESIAN_POINT ( 'NONE',  ( -101.8637373947396014, 32.56989439519480101, -88.71231002810291955 ) ) ;
#8242=CARTESIAN_POINT ( 'NONE',  ( -126.7989199172159545, 47.09198523267863834, -76.71749280709809682 ) ) ;
#8244=CARTESIAN_POINT ( 'NONE',  ( -78.66644367742109978, 23.39876645725290061, -35.11545063171788428 ) ) ;
#8245=CYLINDRICAL_SURFACE ( 'NONE', #31109, 7.500000000000013323 ) ;
#8247=CARTESIAN_POINT ( 'NONE',  ( 204.6977192012829789, -170.0000000000000000, 36.70772073876943153 ) ) ;
#8248=EDGE_CURVE ( 'NONE', #26499, #65633, #22009, .T. ) ;
#8259=CARTESIAN_POINT ( 'NONE',  ( -179.2262621278717916, 94.19039042964669761, 15.86246328341808365 ) ) ;
#8260=DIRECTION ( 'NONE',  ( -0.000000000000000000, 1.000000000000000000, -0.000000000000000000 ) ) ;
#8262=CARTESIAN_POINT ( 'NONE',  ( 57.39233401791016576, 12.46575990788837629, -38.23382626024586983 ) ) ;
#8263=CARTESIAN_POINT ( 'NONE',  ( -83.69370847062540975, 25.38703975185372030, 32.34724513630185783 ) ) ;
#8264=CARTESIAN_POINT ( 'NONE',  ( 151.2978913959096019, 53.00666906180277493, 86.32333572920605036 ) ) ;
#8265=VECTOR ( 'NONE', #39964, 1000.000000000000000 ) ;
#8266=CARTESIAN_POINT ( 'NONE',  ( 134.7697261969508986, 41.97802808873668567, 2.707623648563555196 ) ) ;
#8272=AXIS2_PLACEMENT_3D ( 'NONE', #43345, #20865, #32458 ) ;
#8275=CARTESIAN_POINT ( 'NONE',  ( -78.66644367742111399, -170.0000000000000000, -88.80455181264524356 ) ) ;
#8276=ADVANCED_FACE ( 'NONE', ( #15470 ), #307, .F. ) ;
#8277=FACE_OUTER_BOUND ( 'NONE', #19680, .T. ) ;
#8278=CARTESIAN_POINT ( 'NONE',  ( -118.6398180864478746, 41.89949912940330279, 93.74388258701110033 ) ) ;
#8280=CARTESIAN_POINT ( 'NONE',  ( 86.62931800182293784, 20.48449268398422518, 2.867536982015617575 ) ) ;
#8285=CARTESIAN_POINT ( 'NONE',  ( 85.68197636629477643, 20.16141071296262766, 29.75676157746082140 ) ) ;
#8287=LINE ( 'NONE', #61396, #33935 ) ;
#8288=CARTESIAN_POINT ( 'NONE',  ( -122.3963566076408398, 44.23346594671848209, 58.31322267358287803 ) ) ;
#8289=CARTESIAN_POINT ( 'NONE',  ( -85.73740570227380431, 26.23277384689411917, -18.28398584103688407 ) ) ;
#8290=CARTESIAN_POINT ( 'NONE',  ( -173.9526029538035914, 89.57590038685107459, -22.83302484729744464 ) ) ;
#8296=CARTESIAN_POINT ( 'NONE',  ( 157.4703587214989113, 57.65129005721575339, 56.25401806271706562 ) ) ;
#8297=CARTESIAN_POINT ( 'NONE',  ( -190.6985136298602015, 109.1272424661243434, 69.71826505393651985 ) ) ;
#8301=CARTESIAN_POINT ( 'NONE',  ( -142.0376140313400413, 59.37288070770861736, 92.66934662550120549 ) ) ;
#8309=CARTESIAN_POINT ( 'NONE',  ( 65.62848231372477414, 13.29388722724785232, -50.25499563657418634 ) ) ;
#8311=B_SPLINE_CURVE_WITH_KNOTS ( 'NONE', 3,
 ( #58401, #32032, #41892, #10215, #62666, #31681, #53116, #4949, #52449, #30652, #4266, #15846, #14474, #57731, #9542, #31344, #26411, #21139, #47847, #20095, #35929, #41207, #69313, #15162, #42581, #52103, #64037, #52772, #4599, #14805, #3917, #25390, #37291, #46823, #58741, #26753, #68290, #41549, #65790, #5972, #59782, #16190, #32379, #27788, #22860, #11593 ),
 .UNSPECIFIED., .F., .F.,
 ( 4, 2, 2, 2, 2, 2, 2, 2, 2, 2, 2, 2, 2, 2, 2, 2, 2, 2, 2, 2, 2, 2, 4 ),
 ( 0.02989107162308295151, 0.03170280136394039439, 0.03351453110479783726, 0.03532626084565527319, 0.03713799058651271606, 0.03894972032737015893, 0.03985558519779885955, 0.04076145006822755323, 0.04166731493865626079, 0.04257317980908495447, 0.04347904467951365509, 0.04438490954994235571, 0.04529077442037104245, 0.04619663929079972919, 0.04710250416122842287, 0.04800836903165710268, 0.04891423390208579636, 0.04982009877251449004, 0.05163182851337179413, 0.05344355825422911210, 0.05525528799508642314, 0.05706701773594373417, 0.05887874747680104520 ),
 .UNSPECIFIED. ) ;
#8312=CARTESIAN_POINT ( 'NONE',  ( -59.57462349605616225, 16.98779896904798292, 31.81369624524355544 ) ) ;
#8314=B_SPLINE_CURVE_WITH_KNOTS ( 'NONE', 3,
 ( #36284, #68630, #52111, #30317, #25400, #20435, #57390, #4957, #63363, #46481, #40865, #63012, #67957, #51769, #14813, #15170, #41558, #46831, #35938, #9900, #57740, #68302, #62317, #20105, #58083, #19757, #20786, #68963, #47504, #53126, #36636, #4277, #42253, #52457, #9202, #63711, #31354, #9551, #41902, #36976, #31690, #25740, #52784, #4609, #31016, #47169, #26075 ),
 .UNSPECIFIED., .F., .F.,
 ( 4, 2, 2, 2, 2, 2, 2, 2, 2, 2, 2, 2, 1, 2, 2, 2, 2, 2, 2, 2, 2, 2, 2, 4 ),
 ( 1.471961680016038988E-17, 0.001520400357568961946, 0.002280600536353415489, 0.003040800715137868381, 0.004561201072706815365, 0.005321401251491302518, 0.006081601430275788804, 0.007602001787844744896, 0.008362201966629227712, 0.009122402145413712263, 0.01064280250298268136, 0.01140300268176716592, 0.01216320286055165047, 0.01292340303933613502, 0.01368360321812061957, 0.01520400357568959041, 0.01596420375447407322, 0.01672440393325855951, 0.01824480429082752514, 0.01976520464839649077, 0.02052540482718097359, 0.02128560500596545640, 0.02280600536353444979, 0.02432640572110344318 ),
 .UNSPECIFIED. ) ;
#8315=CARTESIAN_POINT ( 'NONE',  ( -101.3537077702550988, 33.43904726487055257, -8.213091884549116983 ) ) ;
#8317=CARTESIAN_POINT ( 'NONE',  ( 36.08729376665095856, 8.001156100723207487, 71.00402338158136217 ) ) ;
#8318=CARTESIAN_POINT ( 'NONE',  ( 31.93506723555891114, 7.555455508788918806, 91.88129699972643039 ) ) ;
#8319=DIRECTION ( 'NONE',  ( 1.000000000000000000, 0.000000000000000000, 0.000000000000000000 ) ) ;
#8321=CARTESIAN_POINT ( 'NONE',  ( -4.081377963939786468, 6.676029627840588176, -49.42132635526748885 ) ) ;
#8323=CARTESIAN_POINT ( 'NONE',  ( -15.13211202216341000, 8.488266782358818929, 9.061675589273599840 ) ) ;
#8324=CIRCLE ( 'NONE', #17284, 242.4895526022646379 ) ;
#8326=CARTESIAN_POINT ( 'NONE',  ( 19.54326199789021601, 7.657220834818548205, -22.67136140125942134 ) ) ;
#8327=CARTESIAN_POINT ( 'NONE',  ( -108.1144194775597356, 35.84457139767599898, -74.09833502765862079 ) ) ;
#8328=AXIS2_PLACEMENT_3D ( 'NONE', #36270, #15512, #20427 ) ;
#8333=CARTESIAN_POINT ( 'NONE',  ( 126.7877523219523539, 38.47018873135924366, -40.96342094992535721 ) ) ;
#8336=CARTESIAN_POINT ( 'NONE',  ( -166.2727198696243249, 79.81537471512569937, 88.93420674593960484 ) ) ;
#8337=ORIENTED_EDGE ( 'NONE', *, *, #14857, .T. ) ;
#8338=CARTESIAN_POINT ( 'NONE',  ( 126.3580464630938707, 38.22944795020836040, 9.865174046250384521 ) ) ;
#8340=CARTESIAN_POINT ( 'NONE',  ( -146.1142527948576912, 61.35394402951023096, -8.775903138490287247 ) ) ;
#8343=ORIENTED_EDGE ( 'NONE', *, *, #18653, .F. ) ;
#8345=CARTESIAN_POINT ( 'NONE',  ( 149.9615052160180824, 53.28073030175414004, 90.47490059719181943 ) ) ;
#8347=CARTESIAN_POINT ( 'NONE',  ( -62.55184817504198946, 17.87278652436697257, 10.45716724043575852 ) ) ;
#8350=CARTESIAN_POINT ( 'NONE',  ( -156.4797890011541881, 71.69341087347115149, 35.44366185432402006 ) ) ;
#8354=ORIENTED_EDGE ( 'NONE', *, *, #64624, .F. ) ;
#8355=CARTESIAN_POINT ( 'NONE',  ( 61.10129719786243641, 12.23677173834304988, 44.56861354071796910 ) ) ;
#8358=CARTESIAN_POINT ( 'NONE',  ( -166.0031475600388546, 80.98114714564768235, 13.85762239588704503 ) ) ;
#8360=CARTESIAN_POINT ( 'NONE',  ( 19.10216788411014122, 6.629360741291162817, -76.59611760968499539 ) ) ;
#8363=CARTESIAN_POINT ( 'NONE',  ( -130.5904357464318082, 50.88938808445630002, 70.83209939336214234 ) ) ;
#8366=CARTESIAN_POINT ( 'NONE',  ( -71.17846906053298994, 20.67346400882179225, -43.10994888763725186 ) ) ;
#8369=CARTESIAN_POINT ( 'NONE',  ( 211.3710169359754616, 117.8057917113659983, -74.10472688487821813 ) ) ;
#8372=CARTESIAN_POINT ( 'NONE',  ( 141.2801018238827169, 47.29457739955283557, 38.11267848623182175 ) ) ;
#8375=CARTESIAN_POINT ( 'NONE',  ( -132.0870433264403232, 51.94057326482882786, 15.51298448247340644 ) ) ;
#8377=ORIENTED_EDGE ( 'NONE', *, *, #43724, .F. ) ;
#8379=CARTESIAN_POINT ( 'NONE',  ( 15.78827728214693416, 7.507518794609596924, -89.20804527961313113 ) ) ;
#8385=CARTESIAN_POINT ( 'NONE',  ( -168.7150276173047416, 82.35404041280327192, -62.96885486901207685 ) ) ;
#8386=VERTEX_POINT ( 'NONE', #48142 ) ;
#8387=CARTESIAN_POINT ( 'NONE',  ( -107.2385267828037740, 36.51474259889403129, 32.38677383163555135 ) ) ;
#8389=CARTESIAN_POINT ( 'NONE',  ( -38.89042640463648581, 10.93374343663408688, 11.85986522438690471 ) ) ;
#8390=CARTESIAN_POINT ( 'NONE',  ( 82.95856197793165165, 19.25847567427441120, 57.49813389157625210 ) ) ;
#8391=ORIENTED_EDGE ( 'NONE', *, *, #66240, .T. ) ;
#8392=CARTESIAN_POINT ( 'NONE',  ( 188.4389256074244372, 86.37278721358585187, 38.30605937947389350 ) ) ;
#8393=CARTESIAN_POINT ( 'NONE',  ( -189.3111515777350178, 107.1887855376296983, -67.86724232585632421 ) ) ;
#8397=CARTESIAN_POINT ( 'NONE',  ( -14.33060720034884206, 8.412649192293185862, -46.68279329759894125 ) ) ;
#8399=VERTEX_POINT ( 'NONE', #49529 ) ;
#8402=CARTESIAN_POINT ( 'NONE',  ( -58.96922974609609014, 15.76655591015168056, 31.41653672068953185 ) ) ;
#8407=CARTESIAN_POINT ( 'NONE',  ( 149.9883446984744637, 53.30011109831374938, -71.05648309506976545 ) ) ;
#8408=CARTESIAN_POINT ( 'NONE',  ( -38.84150381976579780, 10.92416363971239157, 36.48547519786994542 ) ) ;
#8409=CARTESIAN_POINT ( 'NONE',  ( 134.7697261969508702, 41.97802808873665725, -50.98147753236381874 ) ) ;
#8413=CARTESIAN_POINT ( 'NONE',  ( -154.0716379918897303, 69.49957566103793738, 59.09515286422640656 ) ) ;
#8414=CARTESIAN_POINT ( 'NONE',  ( -120.1259246007803370, 42.81147313035990010, 42.94087449994837868 ) ) ;
#8415=CARTESIAN_POINT ( 'NONE',  ( -58.96922974609608303, 15.76655591015168056, -49.11711505070150707 ) ) ;
#8417=CARTESIAN_POINT ( 'NONE',  ( -180.0154536325056824, 96.73346874014742980, -66.08948715273702135 ) ) ;
#8419=CARTESIAN_POINT ( 'NONE',  ( 88.28780346671264567, 19.99350429399658324, 56.73837274249751772 ) ) ;
#8421=CARTESIAN_POINT ( 'NONE',  ( 113.4493678088378488, 30.39339414805073147, 43.90767737034025231 ) ) ;
#8428=FACE_OUTER_BOUND ( 'NONE', #5436, .T. ) ;
#8429=LINE ( 'NONE', #19664, #35071 ) ;
#8430=CARTESIAN_POINT ( 'NONE',  ( 70.11438327604402332, 14.43198353181102433, 66.59053383333947806 ) ) ;
#8431=CARTESIAN_POINT ( 'NONE',  ( 188.1848725084043110, 86.09288252323347024, -95.00000000000133582 ) ) ;
#8436=CARTESIAN_POINT ( 'NONE',  ( 162.7963212667073662, 63.21900188423071398, -11.49336337990347268 ) ) ;
#8437=ORIENTED_EDGE ( 'NONE', *, *, #55316, .T. ) ;
#8438=FACE_OUTER_BOUND ( 'NONE', #36799, .T. ) ;
#8439=CARTESIAN_POINT ( 'NONE',  ( 136.0716339513249409, 42.77788611838532518, 83.52721415416694128 ) ) ;
#8440=EDGE_CURVE ( 'NONE', #46743, #10004, #50092, .T. ) ;
#8441=B_SPLINE_CURVE_WITH_KNOTS ( 'NONE', 3,
 ( #35078, #56527, #23838, #3416, #8355, #24875, #12585, #50910, #7310, #29804, #8705, #7666, #29448, #13965, #45977, #56891, #51268, #28768, #55482, #35427, #3078, #66761, #24191, #45636, #40006, #46313, #60762, #67790, #67445, #55845, #24541, #30159, #34402, #34745, #45280, #39319, #44933, #29112, #50562, #66418, #34043, #18904, #50217, #2041 ),
 .UNSPECIFIED., .F., .F.,
 ( 4, 2, 2, 2, 2, 2, 2, 2, 2, 2, 2, 2, 2, 2, 2, 2, 2, 2, 2, 2, 2, 4 ),
 ( 1.430489624538199204E-17, 0.001482469635030031312, 0.002223704452545036993, 0.002964939270060043108, 0.004447408905090028015, 0.005929878540120013357, 0.007412348175149999566, 0.008153582992664998308, 0.008894817810179993581, 0.01037728744520999280, 0.01185975708023999028, 0.01260099189775499770, 0.01334222671527000685, 0.01482469635030002689, 0.01556593116781503257, 0.01630716598533003825, 0.01778963562036003573, 0.01927210525539003322, 0.02001334007290503716, 0.02075457489042003417, 0.02223704452545005941, 0.02371951416048008118 ),
 .UNSPECIFIED. ) ;
#8442=ORIENTED_EDGE ( 'NONE', *, *, #48484, .F. ) ;
#8443=CARTESIAN_POINT ( 'NONE',  ( -143.2464978228199470, 59.04559547356110016, -65.01991048928078953 ) ) ;
#8445=CARTESIAN_POINT ( 'NONE',  ( 164.8407099662995563, 63.61629583487395223, -45.03983226934109751 ) ) ;
#8446=ORIENTED_EDGE ( 'NONE', *, *, #10463, .F. ) ;
#8447=CARTESIAN_POINT ( 'NONE',  ( -100.4440683050664802, 32.98184228837415333, 18.46101985899770881 ) ) ;
#8448=DIRECTION ( 'NONE',  ( 1.000000000000000000, 0.000000000000000000, -0.000000000000000000 ) ) ;
#8449=CARTESIAN_POINT ( 'NONE',  ( 39.40195752203891999, 9.424259417798149130, 44.91383430596327742 ) ) ;
#8451=CARTESIAN_POINT ( 'NONE',  ( 79.63513233364427890, 18.20496177163924045, -19.19606465532076101 ) ) ;
#8452=CARTESIAN_POINT ( 'NONE',  ( -173.5164030641130921, 89.08225398748109569, -88.40105834567732757 ) ) ;
#8456=CARTESIAN_POINT ( 'NONE',  ( -97.88021438939452423, 31.71889184683104901, 70.95604366137317243 ) ) ;
#8457=CARTESIAN_POINT ( 'NONE',  ( -13.92109095214680181, 8.375243258322935702, 60.08374128700357630 ) ) ;
#8460=CARTESIAN_POINT ( 'NONE',  ( 153.2208437558771834, 55.67531116261155688, -10.58205773850701092 ) ) ;
#8463=CARTESIAN_POINT ( 'NONE',  ( -38.54237244144231056, 11.89088379031759857, 40.13604733081889719 ) ) ;
#8464=CARTESIAN_POINT ( 'NONE',  ( -156.9406434201983700, 70.74968524571474404, -68.00748788645172738 ) ) ;
#8466=CARTESIAN_POINT ( 'NONE',  ( -50.51700111023806983, 13.51182830536853707, -63.56779930169986415 ) ) ;
#8467=CARTESIAN_POINT ( 'NONE',  ( -1.327237339234998759, 7.561837009978233048, -12.32062923382155795 ) ) ;
#8470=CARTESIAN_POINT ( 'NONE',  ( -60.13226458141419783, 16.10241298991027392, 16.49623137758026203 ) ) ;
#8480=CARTESIAN_POINT ( 'NONE',  ( 17.48988570800757714, 7.568061572928497682, 44.82321039106459182 ) ) ;
#8484=CARTESIAN_POINT ( 'NONE',  ( 57.24431143549729484, 12.43480675010534142, -92.04784424611891325 ) ) ;
#8485=CARTESIAN_POINT ( 'NONE',  ( -165.9111709580270713, 79.44576090485635689, 67.25285630311519469 ) ) ;
#8488=CARTESIAN_POINT ( 'NONE',  ( -102.2801239173131194, -170.0000000000000000, -42.51457726497592660 ) ) ;
#8490=CARTESIAN_POINT ( 'NONE',  ( 180.2473887773227830, 77.76029175826235473, -9.380507075415927432 ) ) ;
#8491=EDGE_CURVE ( 'NONE', #51274, #63292, #38285, .T. ) ;
#8497=CARTESIAN_POINT ( 'NONE',  ( 208.9781236209185522, 112.4006213943319494, 16.03836552217190103 ) ) ;
#8498=CARTESIAN_POINT ( 'NONE',  ( 8.480977594057444335, 7.382886909400594000, 62.65247559583071535 ) ) ;
#8499=CARTESIAN_POINT ( 'NONE',  ( 205.0999694062793708, 106.8955893716604777, 29.20772073876941732 ) ) ;
#8500=FACE_BOUND ( 'NONE', #39990, .T. ) ;
#8501=ADVANCED_FACE ( 'NONE', ( #35811 ), #9076, .F. ) ;
#8505=ORIENTED_EDGE ( 'NONE', *, *, #60104, .T. ) ;
#8507=CARTESIAN_POINT ( 'NONE',  ( -131.7919109508896440, 51.73197705097236820, 87.16560392311338035 ) ) ;
#8509=CARTESIAN_POINT ( 'NONE',  ( 35.66087318222938052, 8.964867769223229033, -76.48343667692702752 ) ) ;
#8510=CARTESIAN_POINT ( 'NONE',  ( -177.1514380519393228, 93.28180884530866024, 17.81740703023968209 ) ) ;
#8512=CARTESIAN_POINT ( 'NONE',  ( 10.70182286329413657, 6.391103395496205763, 85.68233535448860039 ) ) ;
#8519=CARTESIAN_POINT ( 'NONE',  ( 204.3129818922372749, 107.5244029525887726, -51.32593103262158962 ) ) ;
#8523=CARTESIAN_POINT ( 'NONE',  ( -84.54326985437106146, 24.64760594531648863, -64.77422351691623703 ) ) ;
#8524=CARTESIAN_POINT ( 'NONE',  ( -58.33157376762797242, 16.63098604184963847, -9.122086124161532084 ) ) ;
#8525=CARTESIAN_POINT ( 'NONE',  ( 93.72059824125558691, 23.03897520779757357, -67.67350929168541995 ) ) ;
#8529=CARTESIAN_POINT ( 'NONE',  ( 12.03194517566455879, 6.409266703743583982, -36.50893166399959711 ) ) ;
#8533=ADVANCED_FACE ( 'NONE', ( #52997 ), #15385, .F. ) ;
#8534=CARTESIAN_POINT ( 'NONE',  ( 103.5589117581614573, 27.00490790413960696, 13.70687759248179383 ) ) ;
#8536=CARTESIAN_POINT ( 'NONE',  ( -55.05276343752909440, 15.72344139423348430, -50.21632399845989170 ) ) ;
#8537=CARTESIAN_POINT ( 'NONE',  ( 177.7886308167536527, 76.74396398590876345, -63.81728127495517100 ) ) ;
#8540=CARTESIAN_POINT ( 'NONE',  ( 82.14396250120411480, 18.99560174459422868, -49.33747787473168245 ) ) ;
#8541=CYLINDRICAL_SURFACE ( 'NONE', #14191, 7.500000000000020428 ) ;
#8548=CARTESIAN_POINT ( 'NONE',  ( 132.9485794245231318, 40.87843215479637138, 17.62435611736938768 ) ) ;
#8549=CARTESIAN_POINT ( 'NONE',  ( -30.37684067568228485, 9.419394800775835463, -89.07888657189737103 ) ) ;
#8550=CARTESIAN_POINT ( 'NONE',  ( 212.0244789595925852, 118.8177636388541742, 88.78004848219350720 ) ) ;
#8551=CARTESIAN_POINT ( 'NONE',  ( 210.9631450001600683, 117.1791136960928981, 32.54812793961757933 ) ) ;
#8553=CARTESIAN_POINT ( 'NONE',  ( -7.825402957745087207, 6.891034867348158954, 45.11558103944722120 ) ) ;
#8558=CARTESIAN_POINT ( 'NONE',  ( 198.4017331595409246, 98.09114638179340773, -21.06574306269706653 ) ) ;
#8562=CARTESIAN_POINT ( 'NONE',  ( 188.2086267457325448, 87.61890531228286250, -72.92993270353426283 ) ) ;
#8563=CARTESIAN_POINT ( 'NONE',  ( -38.74552978434543604, 11.93068052085773445, 93.18845920815178374 ) ) ;
#8564=CARTESIAN_POINT ( 'NONE',  ( -99.10260179032847816, 31.19580119595417855, -35.71676853837713139 ) ) ;
#8567=CARTESIAN_POINT ( 'NONE',  ( 38.42020198992003799, 8.283430712587435352, -50.57129177816508303 ) ) ;
#8572=CARTESIAN_POINT ( 'NONE',  ( 129.1137093889807943, 38.63348691920619871, -49.33819672148214863 ) ) ;
#8573=VERTEX_POINT ( 'NONE', #21342 ) ;
#8576=ADVANCED_FACE ( 'NONE', ( #31911 ), #15041, .F. ) ;
#8582=CARTESIAN_POINT ( 'NONE',  ( 12.03317402819681980, 6.409531826169462931, 4.173255377313227044 ) ) ;
#8585=CARTESIAN_POINT ( 'NONE',  ( -58.97243502469714826, 16.81420332340173829, -63.16196468205944115 ) ) ;
#8588=CARTESIAN_POINT ( 'NONE',  ( 181.0840389613909736, 78.60582251573003987, 2.464043515047718458 ) ) ;
#8589=CARTESIAN_POINT ( 'NONE',  ( -29.74902699556087171, 10.33856194202125600, 71.87213699941901268 ) ) ;
#8592=CARTESIAN_POINT ( 'NONE',  ( -53.14475157111026959, 14.17819596930906378, 57.40458832884380058 ) ) ;
#8594=CARTESIAN_POINT ( 'NONE',  ( -1.088326810997878091, 6.545818265928950552, 61.12801010162523596 ) ) ;
#8595=EDGE_CURVE ( 'NONE', #41030, #3067, #14746, .T. ) ;
#8598=CARTESIAN_POINT ( 'NONE',  ( 154.4617654203036068, 56.60942201271838314, 56.86943609086132057 ) ) ;
#8599=CARTESIAN_POINT ( 'NONE',  ( -107.0544991134679833, 36.41543129049377114, -75.14825369610649375 ) ) ;
#8600=CARTESIAN_POINT ( 'NONE',  ( -55.05276343752910151, 14.68156374112636264, -50.21632399845989170 ) ) ;
#8607=ORIENTED_EDGE ( 'NONE', *, *, #35262, .F. ) ;
#8609=CARTESIAN_POINT ( 'NONE',  ( 151.1827182658834658, 54.16800928478853194, 32.78911015225024528 ) ) ;
#8612=CARTESIAN_POINT ( 'NONE',  ( -173.1211646369891355, -170.0000000000000000, 45.82169460664104577 ) ) ;
#8614=CARTESIAN_POINT ( 'NONE',  ( -179.5178913137216341, 94.54206947403385186, 15.43129202131554756 ) ) ;
#8615=CARTESIAN_POINT ( 'NONE',  ( -4.955782654901484285, 6.720825733572401539, 3.828862293532663053 ) ) ;
#8618=CARTESIAN_POINT ( 'NONE',  ( -79.14638003838381053, 23.58242782405879723, 45.41820113967313688 ) ) ;
#8620=VECTOR ( 'NONE', #44395, 1000.000000000000000 ) ;
#8621=CARTESIAN_POINT ( 'NONE',  ( 151.5037942372329383, 53.15665752640120445, 86.04130639192804608 ) ) ;
#8622=CARTESIAN_POINT ( 'NONE',  ( 140.4897729434290738, 45.57634363643750675, 13.70496928957165750 ) ) ;
#8626=CARTESIAN_POINT ( 'NONE',  ( 117.7411475730015553, 32.50808475802732289, -43.96506892200977035 ) ) ;
#8627=CARTESIAN_POINT ( 'NONE',  ( 15.78827728214693416, 6.500811158483284835, 56.85925826316891829 ) ) ;
#8628=DIRECTION ( 'NONE',  ( -0.000000000000000000, 1.000000000000000000, -0.000000000000000000 ) ) ;
#8631=VERTEX_POINT ( 'NONE', #60377 ) ;
#8632=CARTESIAN_POINT ( 'NONE',  ( 80.72161230109728081, 17.48902961068030848, -47.96845741328300505 ) ) ;
#8636=CARTESIAN_POINT ( 'NONE',  ( 80.15818551272217007, 18.36718314243334049, 41.03562789125641785 ) ) ;
#8638=CARTESIAN_POINT ( 'NONE',  ( 183.1910712700538113, 80.76073941711165105, -9.669732058764036964 ) ) ;
#8640=CARTESIAN_POINT ( 'NONE',  ( -83.53167274806554587, 25.32068190668983831, -10.04220442384894341 ) ) ;
#8642=CARTESIAN_POINT ( 'NONE',  ( -150.3898662070192529, 64.92828409760433317, -34.81283053149196149 ) ) ;
#8644=VERTEX_POINT ( 'NONE', #43827 ) ;
#8645=CARTESIAN_POINT ( 'NONE',  ( -105.8879245385188170, 35.79035667534147791, 17.76733064874386514 ) ) ;
#8646=CARTESIAN_POINT ( 'NONE',  ( 102.8518012651273921, 25.61025413220827573, 65.25412124308606110 ) ) ;
#8648=CARTESIAN_POINT ( 'NONE',  ( -189.5325095384513645, 107.4952257375067575, 67.39672208484692817 ) ) ;
#8650=CYLINDRICAL_SURFACE ( 'NONE', #60693, 7.500000000000013323 ) ;
#8651=CARTESIAN_POINT ( 'NONE',  ( -142.7670279077608768, 59.94957184373900816, 88.60369296171910491 ) ) ;
#8656=AXIS2_PLACEMENT_3D ( 'NONE', #35470, #57275, #9087 ) ;
#8660=CARTESIAN_POINT ( 'NONE',  ( 70.11438327604403753, 14.43198353181102433, -40.78766852851526892 ) ) ;
#8663=CARTESIAN_POINT ( 'NONE',  ( -62.54086041493278714, 17.86944394914988976, 38.30844689331261321 ) ) ;
#8664=CARTESIAN_POINT ( 'NONE',  ( -31.43908319763709969, 10.61114334766716638, -77.16174795566554678 ) ) ;
#8666=CARTESIAN_POINT ( 'NONE',  ( 59.72647370436681769, 12.96353798836696392, 44.05766389829923213 ) ) ;
#8667=CARTESIAN_POINT ( 'NONE',  ( 44.96493392236942555, 9.198276979102484319, 86.06197627692814933 ) ) ;
#8671=CARTESIAN_POINT ( 'NONE',  ( -0.3249717932738294679, 6.518578686837486202, -42.42990240311857519 ) ) ;
#8673=CARTESIAN_POINT ( 'NONE',  ( -120.1497954511983437, 42.82624472369558788, 6.426331581351773181 ) ) ;
#8675=CARTESIAN_POINT ( 'NONE',  ( 130.3019683985925781, 39.31883119822050787, -23.29995166167127252 ) ) ;
#8677=CARTESIAN_POINT ( 'NONE',  ( -125.8938041572051389, -170.0000000000000000, 11.27539728269340280 ) ) ;
#8678=CARTESIAN_POINT ( 'NONE',  ( 198.7029050523552485, 98.46895521196215384, 68.08812002989884604 ) ) ;
#8679=CIRCLE ( 'NONE', #58116, 242.4895526022646379 ) ;
#8680=EDGE_CURVE ( 'NONE', #59735, #47754, #8909, .T. ) ;
#8684=CARTESIAN_POINT ( 'NONE',  ( 126.4219470349615904, 38.26519385429183728, -42.50070869923012395 ) ) ;
#8685=CYLINDRICAL_SURFACE ( 'NONE', #45508, 7.500000000000013323 ) ;
#8687=CARTESIAN_POINT ( 'NONE',  ( 188.4374648754671568, 87.87346242052443301, -45.22988680152230501 ) ) ;
#8690=CARTESIAN_POINT ( 'NONE',  ( -142.8450945664714880, 58.72815783657285493, -12.01356147524839102 ) ) ;
#8692=ORIENTED_EDGE ( 'NONE', *, *, #46795, .F. ) ;
#8693=B_SPLINE_CURVE_WITH_KNOTS ( 'NONE', 3,
 ( #63374, #53135, #30675, #68973, #31027, #9218, #63722, #26084, #36297, #9567, #4292, #52467, #52122, #68639, #20117, #25410, #20450, #20801, #4965, #3942, #47514, #31703, #46149, #67623, #15532, #15185, #14492, #36646, #67972, #40875, #57066, #36984, #14149, #14828, #3591, #58423, #58091, #9911, #62337, #31367, #10237, #46490, #19418, #52796, #35611, #8879, #30329, #19772, #41230, #35949, #46845, #68313, #41568, #37311, #25 ),
 .UNSPECIFIED., .F., .F.,
 ( 4, 2, 2, 2, 2, 2, 2, 2, 2, 2, 2, 2, 2, 2, 2, 2, 2, 2, 2, 1, 2, 2, 2, 2, 2, 2, 2, 4 ),
 ( 0.000000000000000000, 0.001942359098140214761, 0.002913538647210304252, 0.003884718196280394394, 0.004855897745350484102, 0.005827077294420574677, 0.006798256843490665252, 0.007769436392560754960, 0.009711795490700933509, 0.01068297503977101715, 0.01165415458884109731, 0.01262533413791117921, 0.01359651368698126112, 0.01456769323605134128, 0.01553887278512142318, 0.01748123188326161995, 0.01845241143233171399, 0.01942359098140180457, 0.02039477053047190208, 0.02136595007954199613, 0.02233712962861208670, 0.02330830917768218075, 0.02525066827582240700, 0.02719302737396263325, 0.02816420692303274118, 0.02913538647210285257, 0.03010656602117296396, 0.03107774557024307188 ),
 .UNSPECIFIED. ) ;
#8694=CARTESIAN_POINT ( 'NONE',  ( 164.6573696294227886, 64.77826598361185972, 92.77428207146242300 ) ) ;
#8696=CARTESIAN_POINT ( 'NONE',  ( 126.4318266066172214, 38.27072266789465971, -71.45960955399186787 ) ) ;
#8697=CARTESIAN_POINT ( 'NONE',  ( 127.4953815656695042, 37.71366486045443622, 41.01473559900087906 ) ) ;
#8698=CARTESIAN_POINT ( 'NONE',  ( -156.9900125991010498, 72.16580261738673130, 37.63415873823330315 ) ) ;
#8699=CARTESIAN_POINT ( 'NONE',  ( -102.2801239173131194, -170.0000000000000000, -50.01457726497594081 ) ) ;
#8704=EDGE_CURVE ( 'NONE', #41997, #60761, #46643, .T. ) ;
#8705=CARTESIAN_POINT ( 'NONE',  ( 58.09436971064711486, 11.58462396079456802, 42.99375819818929045 ) ) ;
#8709=CARTESIAN_POINT ( 'NONE',  ( -165.7690020878298469, 80.74028011998679233, 9.965654948806628610 ) ) ;
#8710=CARTESIAN_POINT ( 'NONE',  ( 23.03864809957654103, 6.841061756139155570, -67.92891564569549701 ) ) ;
#8712=CARTESIAN_POINT ( 'NONE',  ( -130.2071229607963119, 50.62285182196877997, 71.11791843384300194 ) ) ;
#8713=ORIENTED_EDGE ( 'NONE', *, *, #5490, .F. ) ;
#8714=CARTESIAN_POINT ( 'NONE',  ( -149.5074843970971301, -170.0000000000000000, -15.46827994102828541 ) ) ;
#8715=CARTESIAN_POINT ( 'NONE',  ( -73.09214866197369531, 21.34321757515763451, -47.65756488281920156 ) ) ;
#8719=CARTESIAN_POINT ( 'NONE',  ( 208.9583973663597760, 114.1615900753670729, -76.85894075021298022 ) ) ;
#8722=CARTESIAN_POINT ( 'NONE',  ( 116.0822834687217124, 32.80169113915573575, 41.84374816554769438 ) ) ;
#8726=VERTEX_POINT ( 'NONE', #31060 ) ;
#8734=CARTESIAN_POINT ( 'NONE',  ( 66.30636076182547356, 14.49616748423541779, -36.46357697616834770 ) ) ;
#8736=CARTESIAN_POINT ( 'NONE',  ( -118.8691191306315034, 43.21907118237574252, 40.76062911680295286 ) ) ;
#8737=CARTESIAN_POINT ( 'NONE',  ( -172.7154982671752634, 86.67743928531946551, -76.55650775521371543 ) ) ;
#8738=EDGE_CURVE ( 'NONE', #64426, #55324, #56747, .T. ) ;
#8740=CARTESIAN_POINT ( 'NONE',  ( -103.8932886509197004, 34.74144483217663293, 30.69090865985877414 ) ) ;
#8742=CARTESIAN_POINT ( 'NONE',  ( -179.7494535813537482, 94.82199694967370363, -92.35590895999905570 ) ) ;
#8743=EDGE_CURVE ( 'NONE', #18334, #16719, #30785, .T. ) ;
#8744=CARTESIAN_POINT ( 'NONE',  ( 80.16761386260786537, 18.37011649821944559, 60.21652803898918904 ) ) ;
#8747=CARTESIAN_POINT ( 'NONE',  ( -189.7987719395348734, 107.8653664616570467, -66.07470785493005394 ) ) ;
#8748=DIRECTION ( 'NONE',  ( 0.000000000000000000, 1.000000000000000000, 0.000000000000000000 ) ) ;
#8751=CARTESIAN_POINT ( 'NONE',  ( -33.12994257348896099, 10.89587983539684934, -23.28366193412811214 ) ) ;
#8759=PLANE ( 'NONE',  #53313 ) ;
#8760=EDGE_LOOP ( 'NONE', ( #37980, #44653, #19269, #29519 ) ) ;
#8763=CARTESIAN_POINT ( 'NONE',  ( -57.96611496808679220, 15.48164310774731511, -89.48114299131638916 ) ) ;
#8771=CARTESIAN_POINT ( 'NONE',  ( -149.9471644042847061, 65.87751327280741975, 57.57507356156872191 ) ) ;
#8772=CARTESIAN_POINT ( 'NONE',  ( -190.6985136298602015, 109.1272424661243434, 69.71826505393651985 ) ) ;
#8777=CARTESIAN_POINT ( 'NONE',  ( 126.6884460900547253, 38.41453276189364630, 88.46451693205000311 ) ) ;
#8778=CARTESIAN_POINT ( 'NONE',  ( 202.1047637245956707, 104.5251427319220880, -90.44580026730181999 ) ) ;
#8782=VERTEX_POINT ( 'NONE', #45058 ) ;
#8783=CARTESIAN_POINT ( 'NONE',  ( 133.8566784816069344, -170.0000000000000000, -9.178760341931969435 ) ) ;
#8784=CARTESIAN_POINT ( 'NONE',  ( 110.2429982417149290, 28.88204397445231209, -77.76698815611739235 ) ) ;
#8785=CARTESIAN_POINT ( 'NONE',  ( 64.94794467308301478, 13.12874966082104500, 71.42075418314232138 ) ) ;
#8786=CARTESIAN_POINT ( 'NONE',  ( 134.0849965622592777, 42.73957449886180626, 2.665790248531672457 ) ) ;
#8789=CARTESIAN_POINT ( 'NONE',  ( 164.0105905242218967, 64.23277447906897919, -20.45969130717543294 ) ) ;
#8791=DIRECTION ( 'NONE',  ( 0.000000000000000000, 0.000000000000000000, 1.000000000000000000 ) ) ;
#8792=CARTESIAN_POINT ( 'NONE',  ( 131.4605497067148576, 39.99540099990633735, 83.56475536640037660 ) ) ;
#8795=CARTESIAN_POINT ( 'NONE',  ( 163.5944155533005642, 63.88379440759436534, -47.96116750131039908 ) ) ;
#8796=CARTESIAN_POINT ( 'NONE',  ( -142.0747101610765242, 58.12276061064464017, -95.00000000000133582 ) ) ;
#8797=CARTESIAN_POINT ( 'NONE',  ( 164.0298848570287191, 62.93631132702880393, -39.94902995324983408 ) ) ;
#8799=CARTESIAN_POINT ( 'NONE',  ( -101.3537077702551130, 33.43904726487055257, 18.63145870591456088 ) ) ;
#8800=PLANE ( 'NONE',  #29004 ) ;
#8801=AXIS2_PLACEMENT_3D ( 'NONE', #53545, #65159, #11682 ) ;
#8802=CARTESIAN_POINT ( 'NONE',  ( 151.4107046593863970, 54.33532586763775640, -92.88899967025768944 ) ) ;
#8803=CARTESIAN_POINT ( 'NONE',  ( 84.97658021689284169, 19.92447159015900127, -23.79656231590709226 ) ) ;
#8804=CARTESIAN_POINT ( 'NONE',  ( -177.4531271036652811, 93.64011491047624247, -89.77488431374720790 ) ) ;
#8805=CARTESIAN_POINT ( 'NONE',  ( -35.17686701826946205, 10.23452050416468317, -63.14123844676133501 ) ) ;
#8808=CARTESIAN_POINT ( 'NONE',  ( -100.4347360276018719, 32.97716872911836106, 57.57929195606707395 ) ) ;
#8809=CARTESIAN_POINT ( 'NONE',  ( -15.32584732649904069, 8.506915958926390076, 64.94853716179643754 ) ) ;
#8811=CARTESIAN_POINT ( 'NONE',  ( 150.7770046255793090, 53.87214803240242134, -13.38559856645425938 ) ) ;
#8818=CARTESIAN_POINT ( 'NONE',  ( 186.7642514597452816, 86.02880938169741398, 14.86798059005289119 ) ) ;
#8820=ADVANCED_FACE ( 'NONE', ( #1821 ), #33488, .F. ) ;
#8821=CARTESIAN_POINT ( 'NONE',  ( 181.0840389613909736, 78.60582251573002566, 17.46404351504774510 ) ) ;
#8822=CARTESIAN_POINT ( 'NONE',  ( -62.30463872474478393, 16.74658165105248031, 8.995110152397721492 ) ) ;
#8826=ORIENTED_EDGE ( 'NONE', *, *, #44878, .F. ) ;
#8827=CARTESIAN_POINT ( 'NONE',  ( 103.8093541423579325, 26.01745837747065337, -74.15374262448062836 ) ) ;
#8829=CARTESIAN_POINT ( 'NONE',  ( -76.10397364431022993, 21.36211154336730189, 4.020946145479624256 ) ) ;
#8832=CARTESIAN_POINT ( 'NONE',  ( -1.041619319073134209, 6.544118473861825436, 88.08972450370782781 ) ) ;
#8833=CARTESIAN_POINT ( 'NONE',  ( -103.2061297292849673, 34.38496953192505856, -23.12722278067304771 ) ) ;
#8834=ORIENTED_EDGE ( 'NONE', *, *, #55645, .F. ) ;
#8835=CARTESIAN_POINT ( 'NONE',  ( -73.09185868250600038, 20.27574131633382848, 69.80405428110501020 ) ) ;
#8836=CARTESIAN_POINT ( 'NONE',  ( -167.9853834315979668, 81.58767916550898747, 70.65234695604632975 ) ) ;
#8839=CARTESIAN_POINT ( 'NONE',  ( -156.8764584803562343, 70.69066846313525332, 36.79685793462269316 ) ) ;
#8841=CARTESIAN_POINT ( 'NONE',  ( 173.9288990958750105, 71.66475105971929338, -14.55843106041742629 ) ) ;
#8842=CARTESIAN_POINT ( 'NONE',  ( 105.4376736768159049, 27.81988511842609668, 58.19221132259757212 ) ) ;
#8844=EDGE_CURVE ( 'NONE', #3228, #2336, #27679, .T. ) ;
#8845=CARTESIAN_POINT ( 'NONE',  ( 56.28782924480459116, 12.23883190161851786, -13.02440547745225707 ) ) ;
#8848=ORIENTED_EDGE ( 'NONE', *, *, #7474, .T. ) ;
#8851=CARTESIAN_POINT ( 'NONE',  ( 206.2980740120524672, 108.5619562183279641, 29.36932263840130375 ) ) ;
#8852=FACE_BOUND ( 'NONE', #64846, .T. ) ;
#8853=ORIENTED_EDGE ( 'NONE', *, *, #16274, .T. ) ;
#8857=CARTESIAN_POINT ( 'NONE',  ( -131.1743031487010285, 51.29764465557688879, 86.47423539255719049 ) ) ;
#8858=CARTESIAN_POINT ( 'NONE',  ( 31.90247004928963648, 8.563336936370813390, -70.46775824028989632 ) ) ;
#8860=CARTESIAN_POINT ( 'NONE',  ( 9.319975126229035567, 6.379801983805998944, 94.99999999999866418 ) ) ;
#8861=CARTESIAN_POINT ( 'NONE',  ( 23.27050824778650551, 7.863710279203344200, 90.59102996714455003 ) ) ;
#8865=CARTESIAN_POINT ( 'NONE',  ( 200.8383807319521281, 102.8517715783673481, -50.27105883604635039 ) ) ;
#8866=VERTEX_POINT ( 'NONE', #1117 ) ;
#8867=CYLINDRICAL_SURFACE ( 'NONE', #58691, 7.500000000000013323 ) ;
#8870=CARTESIAN_POINT ( 'NONE',  ( -94.87734348028330089, 30.28727895192195874, -95.00000000000133582 ) ) ;
#8873=CARTESIAN_POINT ( 'NONE',  ( 46.80475532923156834, 10.50744084852536986, 63.02981851721033024 ) ) ;
#8874=CARTESIAN_POINT ( 'NONE',  ( -103.1197975032058878, 34.34092642966945874, -88.74784833587132482 ) ) ;
#8878=B_SPLINE_CURVE_WITH_KNOTS ( 'NONE', 3,
 ( #59101, #56178, #27436, #32728, #64381, #59787, #40003, #721, #48873, #22172, #32387, #29445, #11257, #38345, #37647, #1410, #16545, #10913, #11966, #33078, #43613, #48525, #43257, #34742, #22517, #16883, #50907, #22867, #61460, #17594, #44313, #358, #64740, #65084, #28135, #11602, #7993, #43958, #37999, #54506, #6339, #2722, #27793, #54155, #16196 ),
 .UNSPECIFIED., .F., .F.,
 ( 4, 2, 2, 2, 2, 2, 2, 2, 2, 2, 2, 1, 2, 2, 2, 2, 2, 2, 2, 2, 2, 2, 4 ),
 ( 1.430489624538199204E-17, 0.001502898956853370750, 0.002254348435280047452, 0.003005797913706724153, 0.004508696870560113118, 0.005260146348986827550, 0.006011595827413541114, 0.007514494784267002070, 0.009017393741120462158, 0.01052029269797392398, 0.01127174217640064882, 0.01202319165482737540, 0.01277464113325410371, 0.01352609061168082681, 0.01502898956853427649, 0.01578043904696100133, 0.01653188852538772097, 0.01803478748224116718, 0.01953768643909460992, 0.02028913591752133302, 0.02104058539594805613, 0.02254348435280153704, 0.02404638330965502141 ),
 .UNSPECIFIED. ) ;
#8879=CARTESIAN_POINT ( 'NONE',  ( -23.95473360498494131, 8.482091576176225445, 90.59507644628696710 ) ) ;
#8880=CARTESIAN_POINT ( 'NONE',  ( -54.08488990389049889, 15.46443908526321209, 3.519856692167697254 ) ) ;
#8881=CARTESIAN_POINT ( 'NONE',  ( -125.8938041572051389, 47.69968343338780414, -8.069153307770243089 ) ) ;
#8882=CARTESIAN_POINT ( 'NONE',  ( 104.3931729003986959, 26.26823401847090267, -38.70273746882388366 ) ) ;
#8883=CARTESIAN_POINT ( 'NONE',  ( -30.47069031368415537, 9.433993659086574723, 30.26315491089761167 ) ) ;
#8884=CARTESIAN_POINT ( 'NONE',  ( -167.9527981889698651, 83.01270690821465337, -90.44578552921110770 ) ) ;
#8889=LINE ( 'NONE', #67635, #35685 ) ;
#8891=CARTESIAN_POINT ( 'NONE',  ( 130.3245512970360664, 39.33195360491887271, 16.79886750242043902 ) ) ;
#8893=CARTESIAN_POINT ( 'NONE',  ( 198.3763953778758093, 99.67840569793540340, 86.34231611871854284 ) ) ;
#8895=CARTESIAN_POINT ( 'NONE',  ( 211.3710169359753479, 117.8057917113659130, 33.27347547697646490 ) ) ;
#8896=CARTESIAN_POINT ( 'NONE',  ( -83.51110947562233378, 25.31252704029285638, 59.03229609086976382 ) ) ;
#8897=DIRECTION ( 'NONE',  ( -0.8118923937861950435, -0.5838071093367415143, 0.000000000000000000 ) ) ;
#8901=CARTESIAN_POINT ( 'NONE',  ( 200.8298320869469933, 101.1869877914232916, -23.42140642344036650 ) ) ;
#8905=CARTESIAN_POINT ( 'NONE',  ( 187.0788993276711949, 86.37277723143235164, -75.08339630570569057 ) ) ;
#8906=CARTESIAN_POINT ( 'NONE',  ( -143.4048679855201271, 60.45763799613828127, 69.43254532525401146 ) ) ;
#8908=CARTESIAN_POINT ( 'NONE',  ( -125.8938041572051389, -170.0000000000000000, 64.96449846362078517 ) ) ;
#8909=B_SPLINE_CURVE_WITH_KNOTS ( 'NONE', 3,
 ( #5850, #33655, #6562, #587, #48750, #60010, #938, #38929, #22038, #6205, #51124, #28359, #44174, #49805, #1631, #65663, #49451, #2939, #43484, #56394, #33307, #37875, #8214, #12192, #29664, #17451, #11831, #24402, #64961, #59321, #11133, #32597, #54022, #59655, #27657, #22386, #51476, #68672, #35293, #46527, #30016, #36328, #52503, #30361 ),
 .UNSPECIFIED., .F., .F.,
 ( 4, 2, 2, 2, 2, 2, 2, 2, 2, 2, 2, 2, 2, 2, 2, 2, 2, 2, 2, 2, 2, 4 ),
 ( 7.949501638480626889E-18, 0.001473754749730506707, 0.002210632124595751820, 0.002947509499460997367, 0.004421264249191475017, 0.005895018998921953100, 0.007368773748652430317, 0.008105651123517666756, 0.008842528498382903196, 0.01031628324811337781, 0.01179003799784384895, 0.01252691537270908366, 0.01326379274757431663, 0.01473754749730477737, 0.01547442487217000860, 0.01621130224703523984, 0.01768505699676569884, 0.01915881174649616478, 0.01989568912136139428, 0.02063256649622662725, 0.02210632124595709666, 0.02358007599568756260 ),
 .UNSPECIFIED. ) ;
#8911=CARTESIAN_POINT ( 'NONE',  ( 39.40195752203892710, 8.409560354027394879, -50.61981746542779348 ) ) ;
#8912=CARTESIAN_POINT ( 'NONE',  ( -105.4589068214113894, 34.42476264325675572, 4.365203437741908665 ) ) ;
#8913=CARTESIAN_POINT ( 'NONE',  ( 12.04188192036245297, 7.416006018508746855, -49.52083859284432776 ) ) ;
#8914=CARTESIAN_POINT ( 'NONE',  ( 126.3580543567275356, 37.07735301062816546, -43.21940575724328681 ) ) ;
#8917=CARTESIAN_POINT ( 'NONE',  ( 187.1611749077166564, 86.46285392389889068, 86.08845492538941357 ) ) ;
#8919=CARTESIAN_POINT ( 'NONE',  ( -23.98903001682803193, 8.486614814224626713, -70.65595771900279942 ) ) ;
#8922=ADVANCED_FACE ( 'NONE', ( #49633 ), #65845, .T. ) ;
#8927=CARTESIAN_POINT ( 'NONE',  ( 173.7227242028391458, 71.47307702680409136, -72.03415706586312695 ) ) ;
#8930=CARTESIAN_POINT ( 'NONE',  ( 88.98408042523107042, 20.23787745328939636, -23.60181295827505110 ) ) ;
#8931=CARTESIAN_POINT ( 'NONE',  ( -24.95010104166214049, 9.631487977190598571, 68.32982050694094767 ) ) ;
#8934=CARTESIAN_POINT ( 'NONE',  ( -101.4457769059400931, 32.35908584109303376, -88.74728229414131420 ) ) ;
#8937=CARTESIAN_POINT ( 'NONE',  ( 149.9883446984744921, 53.30011109831377070, 63.16626985724861498 ) ) ;
#8938=FACE_OUTER_BOUND ( 'NONE', #37569, .T. ) ;
#8939=CARTESIAN_POINT ( 'NONE',  ( -50.51700111023805562, 13.51182830536853352, -36.72324871123618806 ) ) ;
#8948=LINE ( 'NONE', #25823, #51250 ) ;
#8950=B_SPLINE_CURVE_WITH_KNOTS ( 'NONE', 3,
 ( #52359, #25642, #47073, #68537, #15069, #57982, #9799, #68862, #20686, #32628, #38598, #26659, #258, #28039, #31942, #53370, #60040, #5205, #27338, #17122, #16451, #54762, #11858, #37204, #22418, #21375, #33337, #48426, #48096, #59685, #6592, #37552, #32287, #49479, #48776, #58651, #11497, #10472, #1312, #64991, #63946, #65334, #22764, #615, #11162, #53721, #43512, #54054 ),
 .UNSPECIFIED., .F., .F.,
 ( 4, 2, 2, 2, 2, 2, 2, 2, 2, 2, 2, 2, 2, 2, 2, 2, 2, 2, 2, 2, 2, 2, 2, 4 ),
 ( 0.02554216173022672010, 0.02715505844859240903, 0.02796150680777522574, 0.02876795516695804245, 0.03038085188532362729, 0.03199374860368921214, 0.03360664532205479699, 0.03441309368123757900, 0.03521954204042036102, 0.03602599039960314303, 0.03683243875878592505, 0.03844533547715150990, 0.03925178383633430579, 0.04005823219551710862, 0.04086468055469991145, 0.04167112891388270735, 0.04247757727306551712, 0.04328402563224831301, 0.04489692235061395337, 0.04650981906897959373, 0.04731626742816241737, 0.04812271578734524102, 0.04973561250571082587, 0.05134850922407641072 ),
 .UNSPECIFIED. ) ;
#8953=VECTOR ( 'NONE', #7588, 1000.000000000000000 ) ;
#8956=CARTESIAN_POINT ( 'NONE',  ( 62.53356220515463093, 13.59349015304564823, -50.72069083216976537 ) ) ;
#8959=CARTESIAN_POINT ( 'NONE',  ( -28.35957743809534648, 10.12373109553627692, -22.81564308554694165 ) ) ;
#8960=CARTESIAN_POINT ( 'NONE',  ( 138.6020257460769187, 44.36414356192209851, 15.99390124636234845 ) ) ;
#8964=CARTESIAN_POINT ( 'NONE',  ( -7.825402957745083654, 6.891034867348166948, -77.26262132240753999 ) ) ;
#8969=B_SPLINE_CURVE_WITH_KNOTS ( 'NONE', 3,
 ( #30483, #62846, #52617, #62502, #19226, #24531, #4104, #45969, #40681, #35771, #67434, #68464, #41730, #41392, #62140, #36452, #13957, #56883, #8696, #3407, #57566, #25221, #14648, #25566, #36111, #9376, #42068, #32214, #26925, #10060, #69483, #59609, #5121, #15684, #58925, #37132, #21302, #59271 ),
 .UNSPECIFIED., .F., .F.,
 ( 4, 2, 2, 2, 2, 2, 2, 2, 2, 2, 2, 2, 2, 2, 2, 2, 2, 2, 4 ),
 ( 0.02546424207107601118, 0.02703543426729225485, 0.02782103036540034199, 0.02860662646350842914, 0.03017781865972465893, 0.03174901085594088873, 0.03332020305215711159, 0.03489139524837334139, 0.03646258744458957118, 0.03724818354269765486, 0.03803377964080574547, 0.03881937573891382914, 0.03960497183702191282, 0.04117616403323804547, 0.04274735622945417812, 0.04431854842567031078, 0.04588974062188644343, 0.04746093281810256914, 0.05060331721053484832 ),
 .UNSPECIFIED. ) ;
#8971=ORIENTED_EDGE ( 'NONE', *, *, #29550, .F. ) ;
#8976=CARTESIAN_POINT ( 'NONE',  ( 200.4600337307566349, 100.7087439352121265, -64.46507461282644158 ) ) ;
#8983=CARTESIAN_POINT ( 'NONE',  ( -155.1302201283145905, 69.09929365814134883, -37.34342092834704374 ) ) ;
#8988=CARTESIAN_POINT ( 'NONE',  ( -108.5248383251030049, 37.21456094989613916, 7.013330406097838754 ) ) ;
#8989=CARTESIAN_POINT ( 'NONE',  ( 102.7425154123292685, 25.56407025871218863, 63.71405795841012321 ) ) ;
#8990=CARTESIAN_POINT ( 'NONE',  ( 110.9409838438198932, 29.20603643730970944, 83.32602672627702134 ) ) ;
#8993=DIRECTION ( 'NONE',  ( 0.000000000000000000, 0.000000000000000000, 1.000000000000000000 ) ) ;
#8996=CARTESIAN_POINT ( 'NONE',  ( -143.4445817893553112, 60.48932258267372220, 87.48363363319201369 ) ) ;
#8999=EDGE_LOOP ( 'NONE', ( #25995, #54804, #2071, #22165 ) ) ;
#9002=CARTESIAN_POINT ( 'NONE',  ( -81.90020664963797969, 23.57971581008655804, 57.99140405555259292 ) ) ;
#9003=CARTESIAN_POINT ( 'NONE',  ( 70.50372867914784081, 14.53505678900967446, -42.73019894926635232 ) ) ;
#9004=CARTESIAN_POINT ( 'NONE',  ( 105.5292268913834448, 26.76134294421019177, -91.26444993491544722 ) ) ;
#9005=EDGE_CURVE ( 'NONE', #41100, #30857, #37489, .T. ) ;
#9006=CARTESIAN_POINT ( 'NONE',  ( -59.58556642339447507, 16.99097764963621771, 43.81259177720935583 ) ) ;
#9007=CARTESIAN_POINT ( 'NONE',  ( -34.74023699876256899, 11.17830703027883388, -76.41366003997089251 ) ) ;
#9012=CARTESIAN_POINT ( 'NONE',  ( 38.91493890549799062, 8.346224043800608783, 56.75838489642698192 ) ) ;
#9013=CARTESIAN_POINT ( 'NONE',  ( 13.84120792123768773, 6.445822122644895735, -23.43379455737267136 ) ) ;
#9015=CARTESIAN_POINT ( 'NONE',  ( -4.070918861171934466, 6.675509947362631813, -36.42082469883077067 ) ) ;
#9017=CARTESIAN_POINT ( 'NONE',  ( -118.7011677090246735, 41.93687969120206560, 9.134074366734774131 ) ) ;
#9020=CARTESIAN_POINT ( 'NONE',  ( 22.28700331106867694, 7.803633676228380445, -12.42248016224392693 ) ) ;
#9021=CARTESIAN_POINT ( 'NONE',  ( 12.04188192036245120, 7.416006018508747744, 4.168262588083034181 ) ) ;
#9028=DIRECTION ( 'NONE',  ( 0.000000000000000000, 0.000000000000000000, 1.000000000000000000 ) ) ;
#9029=VERTEX_POINT ( 'NONE', #10880 ) ;
#9031=CARTESIAN_POINT ( 'NONE',  ( -148.6409722988649946, 63.44808865916660778, -8.015346559020745332 ) ) ;
#9033=VERTEX_POINT ( 'NONE', #58713 ) ;
#9034=CARTESIAN_POINT ( 'NONE',  ( 153.4899842167529869, 55.87722776145639614, 84.23368635199832966 ) ) ;
#9036=CARTESIAN_POINT ( 'NONE',  ( -56.73868929054668797, 16.18382781951277138, 18.28487575996624415 ) ) ;
#9038=CARTESIAN_POINT ( 'NONE',  ( -155.7457403566965297, 71.01814553754118720, 34.02709316248113680 ) ) ;
#9040=CARTESIAN_POINT ( 'NONE',  ( -96.02415295709703003, 29.71480036090584775, 33.87477838304790367 ) ) ;
#9043=ORIENTED_EDGE ( 'NONE', *, *, #56787, .F. ) ;
#9047=CARTESIAN_POINT ( 'NONE',  ( 174.6307688320643194, 73.70327352127000609, 32.97779385060549373 ) ) ;
#9049=CARTESIAN_POINT ( 'NONE',  ( 17.74393407086869701, 6.570779001277776921, -62.60608148900111303 ) ) ;
#9050=CARTESIAN_POINT ( 'NONE',  ( -126.3495878770405909, 48.00153794568855403, 72.46449846362078517 ) ) ;
#9051=ORIENTED_EDGE ( 'NONE', *, *, #61156, .T. ) ;
#9057=CARTESIAN_POINT ( 'NONE',  ( 136.1215428813736708, 43.99260314811116501, 29.84553875828433078 ) ) ;
#9059=CARTESIAN_POINT ( 'NONE',  ( -129.4036885357273547, 50.06837984316182855, 17.90749390567040678 ) ) ;
#9060=CARTESIAN_POINT ( 'NONE',  ( 68.94309019697858787, 15.16533147648752156, -65.44371665737369881 ) ) ;
#9062=EDGE_CURVE ( 'NONE', #45314, #39145, #32351, .T. ) ;
#9063=ORIENTED_EDGE ( 'NONE', *, *, #50367, .F. ) ;
#9065=CARTESIAN_POINT ( 'NONE',  ( -142.9756886485677398, 60.11539876121631920, -19.16347302773874262 ) ) ;
#9067=DIRECTION ( 'NONE',  ( -0.8160245890732938934, -0.5780171883497599028, 0.000000000000000000 ) ) ;
#9068=CARTESIAN_POINT ( 'NONE',  ( -54.84008385043469502, 14.62454595683343150, -88.90542517938720835 ) ) ;
#9071=CARTESIAN_POINT ( 'NONE',  ( 70.12389542974193546, 15.47520081968151651, -45.66377706524675517 ) ) ;
#9073=CARTESIAN_POINT ( 'NONE',  ( -166.7049310409072405, 80.25944422923579680, -65.16385208324180667 ) ) ;
#9076=CYLINDRICAL_SURFACE ( 'NONE', #5198, 7.500000000000020428 ) ;
#9079=CARTESIAN_POINT ( 'NONE',  ( 81.49482595366482940, 18.78720120198666166, -91.48285567191722123 ) ) ;
#9080=CARTESIAN_POINT ( 'NONE',  ( 82.12277968641508608, 18.98848723477814460, 70.07157773562504133 ) ) ;
#9084=CARTESIAN_POINT ( 'NONE',  ( 39.40195752203892710, 9.424259417798131366, 3.069283715499574239 ) ) ;
#9086=CARTESIAN_POINT ( 'NONE',  ( 32.29989959354728768, 7.591763852038297067, 12.99235193929992072 ) ) ;
#9087=DIRECTION ( 'NONE',  ( 0.000000000000000000, 0.000000000000000000, 1.000000000000000000 ) ) ;
#9090=ADVANCED_FACE ( 'NONE', ( #32004 ), #53776, .F. ) ;
#9092=CARTESIAN_POINT ( 'NONE',  ( -119.1961424429667034, 43.42002938933726597, -92.69538835324019033 ) ) ;
#9095=CARTESIAN_POINT ( 'NONE',  ( -59.95412189755932530, 17.09836075175410031, 58.96417071872249238 ) ) ;
#9096=CARTESIAN_POINT ( 'NONE',  ( -26.50364027666003963, 8.832969329054176200, 5.203539351318217321 ) ) ;
#9098=DIRECTION ( 'NONE',  ( 0.000000000000000000, 0.000000000000000000, 1.000000000000000000 ) ) ;
#9099=CARTESIAN_POINT ( 'NONE',  ( -13.47680110791658414, 7.324966777230640602, -74.71809665986256732 ) ) ;
#9101=CARTESIAN_POINT ( 'NONE',  ( 153.8224167330182013, 56.12711234192238408, -37.06696685681204428 ) ) ;
#9102=ORIENTED_EDGE ( 'NONE', *, *, #7493, .T. ) ;
#9105=CARTESIAN_POINT ( 'NONE',  ( 177.7886308167536242, 76.74396398590877766, -10.12818009402780461 ) ) ;
#9107=CARTESIAN_POINT ( 'NONE',  ( 39.40195752203892710, 8.409560354027394879, -50.61981746542779348 ) ) ;
#9110=CARTESIAN_POINT ( 'NONE',  ( 126.3484241331027675, 38.22406654827073424, 90.61007899326968129 ) ) ;
#9111=CARTESIAN_POINT ( 'NONE',  ( 204.3129818922373602, 107.5244029525888720, -24.48138044215792419 ) ) ;
#9112=CARTESIAN_POINT ( 'NONE',  ( -122.3745688183166465, 44.21964839958061333, -62.61830058063351601 ) ) ;
#9113=ORIENTED_EDGE ( 'NONE', *, *, #12074, .F. ) ;
#9115=CARTESIAN_POINT ( 'NONE',  ( 117.4696399285658686, 32.37118663718648293, -72.33972432310571321 ) ) ;
#9116=CARTESIAN_POINT ( 'NONE',  ( 188.2962140587029864, 87.71627202537840162, 34.72967280661650591 ) ) ;
#9117=CARTESIAN_POINT ( 'NONE',  ( 136.1215428813736992, 43.99260314811115791, 3.000988167820665353 ) ) ;
#9122=EDGE_CURVE ( 'NONE', #65219, #2040, #28198, .T. ) ;
#9123=CARTESIAN_POINT ( 'NONE',  ( 181.0840389613909736, 80.03940679743416808, 56.15314469597509373 ) ) ;
#9127=CARTESIAN_POINT ( 'NONE',  ( 69.35866309798979046, 15.27376159675660716, 68.16710321307755294 ) ) ;
#9129=CARTESIAN_POINT ( 'NONE',  ( 141.1600430683898537, 46.01273571695310949, 92.44402370497088839 ) ) ;
#9131=EDGE_LOOP ( 'NONE', ( #33787, #14223, #56092, #40351 ) ) ;
#9132=DIRECTION ( 'NONE',  ( 0.000000000000000000, 0.000000000000000000, 1.000000000000000000 ) ) ;
#9133=VECTOR ( 'NONE', #2916, 1000.000000000000000 ) ;
#9135=CARTESIAN_POINT ( 'NONE',  ( 113.8626313173125766, 31.71036178495293001, -36.83649234522183491 ) ) ;
#9140=CARTESIAN_POINT ( 'NONE',  ( 79.91920957766410538, 18.29292522273511068, -13.08905856853260019 ) ) ;
#9141=CARTESIAN_POINT ( 'NONE',  ( -166.2028193222419077, 79.74385139484274987, 35.41135073535578215 ) ) ;
#9142=CARTESIAN_POINT ( 'NONE',  ( 151.3309484205705076, 53.03078371058069962, 68.06927186267586194 ) ) ;
#9147=CARTESIAN_POINT ( 'NONE',  ( -7.825402957745085430, 7.899365992529246761, 71.96013162991091860 ) ) ;
#9150=CARTESIAN_POINT ( 'NONE',  ( 150.0278556977734468, 53.32860603304212077, -15.70126343080858611 ) ) ;
#9151=CARTESIAN_POINT ( 'NONE',  ( -62.02002361825626053, 16.66092005917081664, 88.71144110712529596 ) ) ;
#9152=CARTESIAN_POINT ( 'NONE',  ( 108.3942953861066343, 29.14039925067522674, 29.82753592392950992 ) ) ;
#9154=CARTESIAN_POINT ( 'NONE',  ( 56.64858667248266499, 11.28546282538443357, 87.02427806644405450 ) ) ;
#9155=CARTESIAN_POINT ( 'NONE',  ( 187.5246323291927126, 86.86207184872516507, 13.84593183401972460 ) ) ;
#9157=CARTESIAN_POINT ( 'NONE',  ( -173.1211646369891355, -170.0000000000000000, -15.36740657428631351 ) ) ;
#9158=ORIENTED_EDGE ( 'NONE', *, *, #46685, .F. ) ;
#9161=CARTESIAN_POINT ( 'NONE',  ( 107.0471828278920725, 27.43080724084231647, -63.46514271234853055 ) ) ;
#9162=CARTESIAN_POINT ( 'NONE',  ( 56.66438910147189034, 11.28870326331392526, -74.06174710983880516 ) ) ;
#9164=CARTESIAN_POINT ( 'NONE',  ( -0.4198266561544487518, 6.521779739161982725, 89.94873814021600822 ) ) ;
#9166=CARTESIAN_POINT ( 'NONE',  ( -109.4995148930278646, 37.75156937139181679, -17.76878308378839932 ) ) ;
#9170=CARTESIAN_POINT ( 'NONE',  ( -166.9969673948021978, 80.56076768517787912, 69.50387472010612555 ) ) ;
#9175=CARTESIAN_POINT ( 'NONE',  ( -118.4753258120605324, 41.79945864152914936, -95.00000000000133582 ) ) ;
#9177=CARTESIAN_POINT ( 'NONE',  ( 177.0075766083213011, 74.58167636505953624, -23.18021568563761292 ) ) ;
#9182=CARTESIAN_POINT ( 'NONE',  ( 39.40195752203892710, -170.0000000000000000, 29.91383430596324899 ) ) ;
#9184=CARTESIAN_POINT ( 'NONE',  ( 212.0739503583953933, 117.0412199804969759, 8.464582291069975284 ) ) ;
#9185=CARTESIAN_POINT ( 'NONE',  ( 15.78827728214693771, 7.507518794609574719, 71.85925826316895382 ) ) ;
#9186=CARTESIAN_POINT ( 'NONE',  ( 210.5178985598940073, 114.6803933586780886, 41.44437144286931840 ) ) ;
#9187=FACE_BOUND ( 'NONE', #17403, .T. ) ;
#9190=LINE ( 'NONE', #30649, #5313 ) ;
#9191=CARTESIAN_POINT ( 'NONE',  ( -118.6212148433689464, 43.06705977238695482, 93.76419461760292506 ) ) ;
#9192=CARTESIAN_POINT ( 'NONE',  ( 36.98541457540710553, 9.120571655722411464, -62.84764358573202969 ) ) ;
#9193=LINE ( 'NONE', #30653, #69140 ) ;
#9194=CARTESIAN_POINT ( 'NONE',  ( 204.6977192012829505, 108.0580384837234931, 56.05227132923312183 ) ) ;
#9201=VERTEX_POINT ( 'NONE', #6299 ) ;
#9202=CARTESIAN_POINT ( 'NONE',  ( -84.55373779407986490, 24.65190748253136377, 6.400853874559598644 ) ) ;
#9203=EDGE_LOOP ( 'NONE', ( #17271, #26273 ) ) ;
#9204=B_SPLINE_CURVE_WITH_KNOTS ( 'NONE', 3,
 ( #54483, #33755, #54125, #49912, #39032, #34105, #1040, #12290, #49204, #60476, #28109, #54838, #27761, #65409, #64708, #22491, #17918, #48847, #11937, #331, #692, #17199, #55189, #66131, #43587, #16516, #38671, #33409, #60117, #7373, #6660, #65058, #49552, #7013, #1742, #23202, #16857, #60816, #12642, #55540, #37974, #21784, #43233, #59418 ),
 .UNSPECIFIED., .F., .F.,
 ( 4, 2, 2, 2, 2, 2, 2, 2, 2, 2, 2, 2, 2, 2, 2, 2, 2, 2, 2, 2, 2, 4 ),
 ( 0.000000000000000000, 0.001472974678681649233, 0.002209462018022473849, 0.002945949357363298465, 0.004418924036044928616, 0.005891898714726559634, 0.007364873393408188050, 0.008101360732749002258, 0.008837848072089817333, 0.01031082275077144575, 0.01178379742945307763, 0.01252028476879390138, 0.01325677210813472687, 0.01472974678681635528, 0.01546623412615717209, 0.01620272146549798370, 0.01767569614417961732, 0.01914867082286124747, 0.01988515816220205734, 0.02062164550154286374, 0.02209462018022448695, 0.02356759485890610670 ),
 .UNSPECIFIED. ) ;
#9211=CARTESIAN_POINT ( 'NONE',  ( 45.89232972083999584, 10.36128169546909561, 60.49194103217620011 ) ) ;
#9213=CARTESIAN_POINT ( 'NONE',  ( 15.78827728214693416, 6.500811158483284835, 3.170157082241545687 ) ) ;
#9218=CARTESIAN_POINT ( 'NONE',  ( -38.92952675655186567, 10.94143817563081100, 91.90481984702363150 ) ) ;
#9219=CARTESIAN_POINT ( 'NONE',  ( 175.0696098417092230, 74.11936424544846602, -75.05761745562652720 ) ) ;
#9221=EDGE_CURVE ( 'NONE', #29497, #12427, #56627, .T. ) ;
#9224=CARTESIAN_POINT ( 'NONE',  ( 79.92842440418706929, 18.29578799637232933, -46.72678255005806136 ) ) ;
#9225=DIRECTION ( 'NONE',  ( -0.8118923937861950435, -0.5838071093367415143, 0.000000000000000000 ) ) ;
#9226=ORIENTED_EDGE ( 'NONE', *, *, #66169, .T. ) ;
#9227=VERTEX_POINT ( 'NONE', #62609 ) ;
#9229=CARTESIAN_POINT ( 'NONE',  ( -84.55783695959765112, 25.74181993349143482, -64.79229219887942293 ) ) ;
#9230=CARTESIAN_POINT ( 'NONE',  ( 181.0840389613909736, 80.03940679743415387, 17.46404351504774866 ) ) ;
#9233=DIRECTION ( 'NONE',  ( -0.000000000000000000, 1.000000000000000000, -0.000000000000000000 ) ) ;
#9234=CARTESIAN_POINT ( 'NONE',  ( -156.0171627975467459, 69.90368824761763733, 15.11010338763517069 ) ) ;
#9235=CARTESIAN_POINT ( 'NONE',  ( -119.2949674747224833, 43.48097822533566870, -65.65536687615315259 ) ) ;
#9237=CARTESIAN_POINT ( 'NONE',  ( -73.79615177260653525, 20.52570924097572203, -63.73540638605312836 ) ) ;
#9238=CARTESIAN_POINT ( 'NONE',  ( -108.1144194775597214, 35.84457139767598477, 33.27986733419606225 ) ) ;
#9241=CARTESIAN_POINT ( 'NONE',  ( -62.55959671100190178, 17.87514270266995808, 91.55944001517654840 ) ) ;
#9243=CARTESIAN_POINT ( 'NONE',  ( 198.3926538463959162, 98.07933330386025261, -12.88060239399294638 ) ) ;
#9245=CARTESIAN_POINT ( 'NONE',  ( -144.2038301586456726, 61.09856042007388055, 6.051060875653559989 ) ) ;
#9249=CARTESIAN_POINT ( 'NONE',  ( 141.3400002717723112, 47.33399859146518196, -42.95563374243955934 ) ) ;
#9250=CARTESIAN_POINT ( 'NONE',  ( 37.00112095025829717, 8.109340230899354296, -36.01023555749208072 ) ) ;
#9252=CARTESIAN_POINT ( 'NONE',  ( 9.050324533885213185, 7.384616180193962265, -46.34927038791500564 ) ) ;
#9253=CARTESIAN_POINT ( 'NONE',  ( 132.9485794245231318, 40.87843215479637138, -36.06474506355797160 ) ) ;
#9256=CARTESIAN_POINT ( 'NONE',  ( 176.7865369010601739, 75.76733092971367967, 84.34302050498311587 ) ) ;
#9257=CARTESIAN_POINT ( 'NONE',  ( -190.6985136298601731, 109.1272424661242582, -95.00000000000133582 ) ) ;
#9266=CARTESIAN_POINT ( 'NONE',  ( -175.1920326508032986, 89.46239303019291356, -49.43298755416176249 ) ) ;
#9267=CARTESIAN_POINT ( 'NONE',  ( 93.61951000632932107, 21.92572933971852223, -19.20632885156578240 ) ) ;
#9268=CARTESIAN_POINT ( 'NONE',  ( -27.49195330402088544, 9.993776132065303131, 58.17902382732258104 ) ) ;
#9275=CARTESIAN_POINT ( 'NONE',  ( -105.4642082819536455, 35.56541171990219397, -62.55240665351630014 ) ) ;
#9276=CARTESIAN_POINT ( 'NONE',  ( -51.34325167237333432, 13.71819364263222418, -36.19337418838312459 ) ) ;
#9283=ORIENTED_EDGE ( 'NONE', *, *, #20333, .F. ) ;
#9287=DIRECTION ( 'NONE',  ( 0.000000000000000000, 0.000000000000000000, 1.000000000000000000 ) ) ;
#9293=CARTESIAN_POINT ( 'NONE',  ( 59.30258796551118650, 12.87111270082601422, -49.75570897052192976 ) ) ;
#9294=CARTESIAN_POINT ( 'NONE',  ( -81.89510452344293867, 24.66033552777454929, 31.13203741669646263 ) ) ;
#9295=CARTESIAN_POINT ( 'NONE',  ( -23.95089599695169014, 9.496585844566173051, -16.46116198601244918 ) ) ;
#9297=ORIENTED_EDGE ( 'NONE', *, *, #59308, .T. ) ;
#9298=CARTESIAN_POINT ( 'NONE',  ( 133.8566784816069344, -170.0000000000000000, 29.51034083899533300 ) ) ;
#9300=CARTESIAN_POINT ( 'NONE',  ( -24.95010104166215470, 9.631487977190602123, 41.48526991647725737 ) ) ;
#9302=CARTESIAN_POINT ( 'NONE',  ( 200.8303160266298732, 102.8412051751308667, 43.14791935769463294 ) ) ;
#9303=B_SPLINE_CURVE_WITH_KNOTS ( 'NONE', 3,
 ( #9123, #25314, #64305, #15773, #25658, #4869, #58671, #47091, #31276, #52702, #46745, #57658, #68554, #20356, #9470, #47773, #42163, #4531, #20706, #26337, #63626, #15440, #68218, #41481, #31958, #36892, #69230, #58328, #63960, #21062, #53386, #26679, #32642, #277, #49147, #28404, #987, #21730, #5893, #22783, #22435, #66070, #16799, #12238 ),
 .UNSPECIFIED., .F., .F.,
 ( 4, 2, 2, 2, 2, 2, 2, 2, 2, 2, 2, 2, 2, 2, 2, 2, 2, 2, 2, 2, 2, 4 ),
 ( 0.02895403260893137515, 0.03071603688922225697, 0.03247804116951313880, 0.03424004544980401715, 0.03600204973009489551, 0.03776405401038578080, 0.03864505615053121651, 0.03952605829067665222, 0.04040706043082208793, 0.04128806257096752363, 0.04216906471111296628, 0.04305006685125840199, 0.04393106899140383770, 0.04481207113154928035, 0.04569307327169470911, 0.04657407541184015176, 0.04745507755198558747, 0.04833607969213102318, 0.05009808397242189459, 0.05186008825271277295, 0.05362209253300365130, 0.05714610109358542189 ),
 .UNSPECIFIED. ) ;
#9305=LINE ( 'NONE', #30079, #63541 ) ;
#9310=ORIENTED_EDGE ( 'NONE', *, *, #68306, .F. ) ;
#9312=CARTESIAN_POINT ( 'NONE',  ( 115.0485321076020853, 32.28990710985444679, -64.48787662897211703 ) ) ;
#9313=CARTESIAN_POINT ( 'NONE',  ( 8.000000000000007105, 249.8719672152120381, 94.99999999999866418 ) ) ;
#9321=CARTESIAN_POINT ( 'NONE',  ( -51.13576748034040520, 14.70354244225167406, 31.41683688099750071 ) ) ;
#9325=CARTESIAN_POINT ( 'NONE',  ( -86.15466590221103615, 26.40813842494317498, -42.12330144728298364 ) ) ;
#9326=AXIS2_PLACEMENT_3D ( 'NONE', #59218, #21252, #42363 ) ;
#9327=CARTESIAN_POINT ( 'NONE',  ( 103.3371571523556014, 25.81603694048630615, 93.80874747008428471 ) ) ;
#9329=CARTESIAN_POINT ( 'NONE',  ( 188.0081045302011091, 85.89855126821616693, -46.62130388048676366 ) ) ;
#9336=CARTESIAN_POINT ( 'NONE',  ( 179.7182127114821810, 77.23376928426336008, -90.00569010101817469 ) ) ;
#9337=CARTESIAN_POINT ( 'NONE',  ( 70.46452034227871764, 14.52462608639673647, -44.22581347596196366 ) ) ;
#9338=CARTESIAN_POINT ( 'NONE',  ( 107.2180420114370492, 27.50716259871310143, -90.23723215542567289 ) ) ;
#9342=CARTESIAN_POINT ( 'NONE',  ( 8.951900209438536038, 6.378066731449592908, -19.26863345807493388 ) ) ;
#9345=CARTESIAN_POINT ( 'NONE',  ( 15.78827728214693416, 7.507518794609588042, 3.170157082241545687 ) ) ;
#9346=CARTESIAN_POINT ( 'NONE',  ( 181.0840389613909736, 78.60582251573006829, 71.15314469597512925 ) ) ;
#9347=CARTESIAN_POINT ( 'NONE',  ( -125.8938041572051105, 46.49392987655492959, 3.775397282693376599 ) ) ;
#9350=B_SPLINE_CURVE_WITH_KNOTS ( 'NONE', 3,
 ( #58036, #36930, #20746, #40911, #15477, #4911, #61327, #66971, #61670, #51123, #37603, #54460, #58706, #16839, #37955, #53427, #10523, #312, #32343, #22122, #27045, #31062, #21427, #38299, #43569, #59739, #60096, #43911, #42869, #65394, #11213, #6642, #64693, #31995, #676, #53770, #1024, #6293, #5591, #17182, #65040, #27389, #11553, #37254, #33392, #48478, #10873, #42544, #59402, #38655 ),
 .UNSPECIFIED., .F., .F.,
 ( 4, 2, 2, 2, 2, 2, 2, 2, 2, 2, 2, 2, 2, 2, 2, 2, 2, 2, 2, 2, 2, 2, 2, 2, 4 ),
 ( 0.03126542424884326543, 0.03330676804260261636, 0.03534811183636196730, 0.03738945563012131823, 0.03943079942388067610, 0.04045147132076034463, 0.04147214321764001316, 0.04249281511451968862, 0.04351348701139935715, 0.04555483080515874972, 0.04657550270203845988, 0.04759617459891818392, 0.04810651054735805981, 0.04861684649579793571, 0.04963751839267768751, 0.05065819028955745318, 0.05167886218643720497, 0.05269953408331695677, 0.05372020598019670856, 0.05474087787707647423, 0.05576154977395622603, 0.05780289356771575737, 0.05984423736147530259, 0.06188558115523483394, 0.06392692494899437916 ),
 .UNSPECIFIED. ) ;
#9351=CARTESIAN_POINT ( 'NONE',  ( 19.75315861330098244, 7.667327050329332927, -22.54537247460588034 ) ) ;
#9352=CARTESIAN_POINT ( 'NONE',  ( 10.13563904803030979, 7.391572367417560407, 15.62368066821783685 ) ) ;
#9357=CARTESIAN_POINT ( 'NONE',  ( -125.8938041572051105, 46.49392987655493670, -88.60280507916129977 ) ) ;
#9360=CARTESIAN_POINT ( 'NONE',  ( -129.6001310305488516, 48.98284622040320357, -35.88933794309529901 ) ) ;
#9361=CARTESIAN_POINT ( 'NONE',  ( -109.5157885508426432, 37.76058765671429995, -40.47346829093316956 ) ) ;
#9362=CARTESIAN_POINT ( 'NONE',  ( 183.9887307715836755, 83.05100282186906213, -36.80690435289106688 ) ) ;
#9367=EDGE_CURVE ( 'NONE', #59065, #64204, #49184, .T. ) ;
#9368=CARTESIAN_POINT ( 'NONE',  ( -29.75049355503752579, 9.320234381800311496, -23.28418078306753003 ) ) ;
#9374=FACE_OUTER_BOUND ( 'NONE', #3949, .T. ) ;
#9375=EDGE_LOOP ( 'NONE', ( #40008, #23303, #63264, #43200 ) ) ;
#9376=CARTESIAN_POINT ( 'NONE',  ( 126.6266894765173987, 38.37986986668740741, -68.30481562020717945 ) ) ;
#9381=CARTESIAN_POINT ( 'NONE',  ( -94.85061234775062644, 29.16417548023186157, 36.96106783413039665 ) ) ;
#9382=DIRECTION ( 'NONE',  ( 0.000000000000000000, 0.000000000000000000, 1.000000000000000000 ) ) ;
#9388=CARTESIAN_POINT ( 'NONE',  ( -172.7173255566597447, 88.18461381371098184, 3.977144016177347030 ) ) ;
#9392=CARTESIAN_POINT ( 'NONE',  ( -178.0633751203918678, 92.80295726428050784, -9.721336043951847472 ) ) ;
#9393=CARTESIAN_POINT ( 'NONE',  ( -126.7944042662569046, 48.29830493043732531, 57.50493334633024745 ) ) ;
#9395=CARTESIAN_POINT ( 'NONE',  ( -109.1372336806175554, 37.55118937703328186, 88.60118964784474827 ) ) ;
#9397=EDGE_CURVE ( 'NONE', #6351, #49086, #37826, .T. ) ;
#9401=CARTESIAN_POINT ( 'NONE',  ( -58.76006735892197952, 15.70681061434692971, -22.39598332331549102 ) ) ;
#9403=VECTOR ( 'NONE', #36955, 1000.000000000000000 ) ;
#9405=CARTESIAN_POINT ( 'NONE',  ( -126.8016613879753578, 48.30316697011513583, 18.73391331175302810 ) ) ;
#9406=CARTESIAN_POINT ( 'NONE',  ( 70.12389542974193546, 15.47520081968152006, -72.50832765571044547 ) ) ;
#9410=CARTESIAN_POINT ( 'NONE',  ( 10.46559741370271723, 7.394044226375385165, -91.35694110006950552 ) ) ;
#9411=CARTESIAN_POINT ( 'NONE',  ( -167.1540252468941787, 80.72321878831098729, -46.76267734215787186 ) ) ;
#9415=CARTESIAN_POINT ( 'NONE',  ( -77.02112161466367013, 22.77583432622785509, 45.23932557689580847 ) ) ;
#9417=CARTESIAN_POINT ( 'NONE',  ( -143.3925773749112977, 59.16144459815141943, 42.57086191493854699 ) ) ;
#9419=CARTESIAN_POINT ( 'NONE',  ( 93.85477471612979627, 23.08982334209078147, -95.00000000000133582 ) ) ;
#9420=CARTESIAN_POINT ( 'NONE',  ( -166.2028657618940599, 79.74389853943286255, -66.14595115942351811 ) ) ;
#9424=ORIENTED_EDGE ( 'NONE', *, *, #67510, .F. ) ;
#9425=CARTESIAN_POINT ( 'NONE',  ( -33.83558513595455253, 9.996963989836510578, 17.98292301535087034 ) ) ;
#9431=CARTESIAN_POINT ( 'NONE',  ( 8.000000000000007105, 249.8719672152120381, -95.00000000000133582 ) ) ;
#9433=CIRCLE ( 'NONE', #28502, 242.4895526022646379 ) ;
#9434=CARTESIAN_POINT ( 'NONE',  ( -37.93379515072632557, 11.77251734620211465, -19.75563545715445457 ) ) ;
#9436=CARTESIAN_POINT ( 'NONE',  ( -118.4753258120605466, 42.97785158603420541, -95.00000000000133582 ) ) ;
#9441=CARTESIAN_POINT ( 'NONE',  ( -10.91976120871578004, 7.112268444252505262, -76.59894436445749477 ) ) ;
#9442=CARTESIAN_POINT ( 'NONE',  ( -95.21430597939263407, 29.33390900154316583, -18.23546955400044212 ) ) ;
#9443=CARTESIAN_POINT ( 'NONE',  ( 150.2193536046551685, 53.46717047532151668, -45.55991080038433694 ) ) ;
#9447=CARTESIAN_POINT ( 'NONE',  ( -156.3734885497380844, 71.59531449004281001, 62.03543042666215968 ) ) ;
#9448=CARTESIAN_POINT ( 'NONE',  ( 180.2494929075578227, 79.18888319146952881, -9.380507075415932761 ) ) ;
#9449=CARTESIAN_POINT ( 'NONE',  ( -103.8932886509197004, 34.74144483217664003, 57.53545925032246799 ) ) ;
#9452=CARTESIAN_POINT ( 'NONE',  ( -180.0094637318087223, 96.72611451757710199, -72.03732202628357584 ) ) ;
#9453=CARTESIAN_POINT ( 'NONE',  ( 93.61951000632933528, 21.92572933971851157, 61.32732291982528494 ) ) ;
#9455=CARTESIAN_POINT ( 'NONE',  ( 116.1021807117072058, 31.68810634233425816, 41.81952508025639048 ) ) ;
#9456=ADVANCED_FACE ( 'NONE', ( #20039 ), #10160, .F. ) ;
#9459=CARTESIAN_POINT ( 'NONE',  ( -118.8504142000306132, 42.02789424825281372, -66.66768671471533025 ) ) ;
#9462=CARTESIAN_POINT ( 'NONE',  ( 199.3671895066314335, 99.30947926630329903, 31.40750943429757669 ) ) ;
#9463=CARTESIAN_POINT ( 'NONE',  ( 116.8937673311173029, 32.08228998570056234, -73.74270732603237377 ) ) ;
#9464=CARTESIAN_POINT ( 'NONE',  ( 183.9887307715835902, 83.05100282186904792, 43.72674741849996849 ) ) ;
#9468=ORIENTED_EDGE ( 'NONE', *, *, #45418, .F. ) ;
#9470=CARTESIAN_POINT ( 'NONE',  ( 174.4978817191264682, 73.57770570413208588, 60.05495216553277515 ) ) ;
#9471=VERTEX_POINT ( 'NONE', #58683 ) ;
#9472=CARTESIAN_POINT ( 'NONE',  ( -102.7502407665687798, 33.01985383847078026, -35.01457726497592660 ) ) ;
#9473=CARTESIAN_POINT ( 'NONE',  ( 141.3536823173203913, 46.13936215296858734, 90.27715462940014390 ) ) ;
#9475=CARTESIAN_POINT ( 'NONE',  ( -62.15324028806256962, 16.70091357159899914, 40.28273643365055534 ) ) ;
#9478=CARTESIAN_POINT ( 'NONE',  ( -178.7458319892713519, 93.61502008198021940, 43.28923195309091199 ) ) ;
#9482=CARTESIAN_POINT ( 'NONE',  ( 115.7612476187723729, 32.64200929566222698, -38.31947670043274456 ) ) ;
#9488=CARTESIAN_POINT ( 'NONE',  ( 138.1919700334460117, 44.10401742531045954, 57.71697704383397820 ) ) ;
#9489=CARTESIAN_POINT ( 'NONE',  ( -175.0670687835823003, 90.85007209570210307, -88.64706874488653909 ) ) ;
#9490=CYLINDRICAL_SURFACE ( 'NONE', #43700, 7.500000000000020428 ) ;
#9491=CARTESIAN_POINT ( 'NONE',  ( 87.58754341703159696, 20.81465688423119786, 44.66585312417346643 ) ) ;
#9492=EDGE_LOOP ( 'NONE', ( #68981, #35356 ) ) ;
#9493=CARTESIAN_POINT ( 'NONE',  ( 41.09759788073309750, 9.651672055033847286, 17.87914307703790229 ) ) ;
#9495=CARTESIAN_POINT ( 'NONE',  ( 155.2992895652387801, 57.24699634758577815, -23.97237736446589196 ) ) ;
#9496=CARTESIAN_POINT ( 'NONE',  ( 208.5936709733499015, 113.6229123546138453, -23.40417240335101923 ) ) ;
#9498=CARTESIAN_POINT ( 'NONE',  ( -153.7005182577088931, 67.81869626254724892, -62.92235873534134072 ) ) ;
#9499=CARTESIAN_POINT ( 'NONE',  ( 55.65828023224232624, 11.08571960351219765, 89.50825515078493311 ) ) ;
#9500=CARTESIAN_POINT ( 'NONE',  ( 188.0103583326377077, 87.39896620268119420, 12.85485524293919468 ) ) ;
#9501=CARTESIAN_POINT ( 'NONE',  ( 211.5175447467296692, 116.1901475271414057, -40.69079531326852361 ) ) ;
#9502=CARTESIAN_POINT ( 'NONE',  ( 173.9413349464226997, 71.67637800842356910, 7.659110634810657459 ) ) ;
#9503=ORIENTED_EDGE ( 'NONE', *, *, #22947, .F. ) ;
#9505=DIRECTION ( 'NONE',  ( -0.000000000000000000, 1.000000000000000000, -0.000000000000000000 ) ) ;
#9507=CARTESIAN_POINT ( 'NONE',  ( -71.86568654225716557, 20.91200104397924164, 61.59056581666523300 ) ) ;
#9508=CARTESIAN_POINT ( 'NONE',  ( 58.09607305250593612, 11.58497620657515803, -75.74799500400911256 ) ) ;
#9511=CARTESIAN_POINT ( 'NONE',  ( -1.298947065946362001, 6.553849421084473548, 94.99999999999866418 ) ) ;
#9515=CARTESIAN_POINT ( 'NONE',  ( -77.71448999903259391, 21.96089801565739208, 72.21751608881839957 ) ) ;
#9521=CARTESIAN_POINT ( 'NONE',  ( -152.5067928559255677, 66.76529500553621688, 31.33228448026122237 ) ) ;
#9523=CARTESIAN_POINT ( 'NONE',  ( 174.2469308602415481, 71.96142024047682639, -19.97548777397644670 ) ) ;
#9525=EDGE_CURVE ( 'NONE', #13412, #51562, #55950, .T. ) ;
#9527=CARTESIAN_POINT ( 'NONE',  ( -142.0081215801270105, 58.07066293384866640, 11.07645372095419489 ) ) ;
#9530=ORIENTED_EDGE ( 'NONE', *, *, #36855, .F. ) ;
#9531=CARTESIAN_POINT ( 'NONE',  ( 210.6741002223296562, 114.9147155784837793, 14.40197977070410751 ) ) ;
#9532=CARTESIAN_POINT ( 'NONE',  ( 12.46490660984525789, 7.423426948220649635, 71.08722924195309645 ) ) ;
#9533=CARTESIAN_POINT ( 'NONE',  ( 212.1535111375854683, 117.1635556319084657, 37.53863579503308046 ) ) ;
#9534=FACE_BOUND ( 'NONE', #47207, .T. ) ;
#9538=EDGE_CURVE ( 'NONE', #15521, #63292, #16478, .T. ) ;
#9541=CARTESIAN_POINT ( 'NONE',  ( -118.3971226877368537, 42.93006216270222808, 91.40225232301679625 ) ) ;
#9542=CARTESIAN_POINT ( 'NONE',  ( -166.5704851812740799, 80.12110537694668722, -19.03004029801454422 ) ) ;
#9544=CARTESIAN_POINT ( 'NONE',  ( 20.87035195714981484, 6.716493875830939153, 85.67848478272195223 ) ) ;
#9545=CARTESIAN_POINT ( 'NONE',  ( 22.95772980082745462, 7.844166310250415108, 88.97759199307637346 ) ) ;
#9548=DIRECTION ( 'NONE',  ( 0.000000000000000000, -1.000000000000000000, 0.000000000000000000 ) ) ;
#9551=CARTESIAN_POINT ( 'NONE',  ( -83.14462298835726983, 24.07775853418027623, 5.038079082316872181 ) ) ;
#9558=CARTESIAN_POINT ( 'NONE',  ( 9.823983574062872037, 6.382904402091121199, -47.59236116552792595 ) ) ;
#9559=CARTESIAN_POINT ( 'NONE',  ( -178.0633751203918962, 92.80295726428049363, 70.81231572743919855 ) ) ;
#9560=CARTESIAN_POINT ( 'NONE',  ( 132.7179291807800610, 40.74118679001687582, 56.43832664394951593 ) ) ;
#9566=AXIS2_PLACEMENT_3D ( 'NONE', #5129, #21307, #48708 ) ;
#9567=CARTESIAN_POINT ( 'NONE',  ( -38.80623589257147898, 10.91725262622218828, 89.96254966543166631 ) ) ;
#9568=CARTESIAN_POINT ( 'NONE',  ( 173.5844030397475990, 72.71952271766126330, -70.87456350105938441 ) ) ;
#9571=CARTESIAN_POINT ( 'NONE',  ( 107.9301116202191935, 27.82606182274594886, -50.57270492925939465 ) ) ;
#9572=CARTESIAN_POINT ( 'NONE',  ( 79.33384730094452664, 18.11203072455029073, -45.07922390903824805 ) ) ;
#9574=ORIENTED_EDGE ( 'NONE', *, *, #68829, .F. ) ;
#9576=CARTESIAN_POINT ( 'NONE',  ( -82.93126516400698733, 25.07709093823495294, -75.63414270348664559 ) ) ;
#9577=CARTESIAN_POINT ( 'NONE',  ( 180.2494929075577659, 79.18888319146950039, 17.46404351504774866 ) ) ;
#9579=FACE_OUTER_BOUND ( 'NONE', #33902, .T. ) ;
#9580=CARTESIAN_POINT ( 'NONE',  ( 126.8237978310704221, 37.33705012421152247, 12.78451399988137105 ) ) ;
#9581=CARTESIAN_POINT ( 'NONE',  ( -155.7433525314458791, 69.65452735858370659, 15.55135967904255168 ) ) ;
#9583=CARTESIAN_POINT ( 'NONE',  ( 205.5130322755755685, 109.1888880665735826, 44.20772073876945285 ) ) ;
#9584=CARTESIAN_POINT ( 'NONE',  ( -81.01931326044685022, 24.31309346877658584, 71.88812866901480447 ) ) ;
#9585=CARTESIAN_POINT ( 'NONE',  ( -102.7456062648101778, 33.01749955571778372, 30.51907450641510877 ) ) ;
#9588=CARTESIAN_POINT ( 'NONE',  ( -48.08829070713510134, 13.95819972868300418, 88.70444353358108458 ) ) ;
#9596=CARTESIAN_POINT ( 'NONE',  ( 136.1215428813736708, 43.99260314811117212, -50.68811301310670103 ) ) ;
#9598=CARTESIAN_POINT ( 'NONE',  ( 32.67604596315972287, 7.629767358313822356, -46.44744588816674735 ) ) ;
#9600=CARTESIAN_POINT ( 'NONE',  ( 86.62931800182293784, 20.48449268398423229, 44.71208757247933363 ) ) ;
#9602=ORIENTED_EDGE ( 'NONE', *, *, #17786, .T. ) ;
#9609=B_SPLINE_CURVE_WITH_KNOTS ( 'NONE', 3,
 ( #55826, #23120, #7646, #35403, #62126, #18881, #61777, #2363, #61445, #23815, #13946, #29097, #28384, #23476, #45257, #2706, #13600, #40330, #55464, #13263, #24167, #7288, #50195, #35058, #34724, #45609, #18534, #44571, #6933, #49831, #66047, #56162, #60743, #67093, #56503, #17841, #39298, #28743, #44915, #66398, #61098, #26228, #9712 ),
 .UNSPECIFIED., .F., .F.,
 ( 4, 2, 2, 2, 2, 2, 2, 2, 2, 2, 2, 2, 1, 2, 2, 2, 2, 2, 2, 2, 2, 4 ),
 ( 0.02358007599568756954, 0.02505677178601666000, 0.02579511968118118961, 0.02653346757634572270, 0.02801016336667479581, 0.02948685915700387239, 0.03022520705216839507, 0.03096355494733291774, 0.03244025073766196310, 0.03391694652799101539, 0.03539364231832005381, 0.03613199021348457995, 0.03687033810864910610, 0.03760868600381363225, 0.03834703389897815146, 0.03982372968930719681, 0.04130042547963624910, 0.04277712126996529446, 0.04351546916512981367, 0.04425381706029432594, 0.04573051285062335047, 0.04720720864095236113 ),
 .UNSPECIFIED. ) ;
#9613=CARTESIAN_POINT ( 'NONE',  ( 15.29899606819416569, 6.485153354884286792, 3.170157082241544799 ) ) ;
#9614=CARTESIAN_POINT ( 'NONE',  ( 41.80869235728138023, 9.750404582811610155, -77.08460388544597208 ) ) ;
#9617=CARTESIAN_POINT ( 'NONE',  ( 210.6592759200688079, 116.7161312026394171, 14.42140922515896584 ) ) ;
#9619=CARTESIAN_POINT ( 'NONE',  ( 93.92910382125423041, 22.04227458821882379, -14.73737663557316857 ) ) ;
#9620=CARTESIAN_POINT ( 'NONE',  ( -30.46002654261638298, 10.45132580906816067, 57.10924613618367118 ) ) ;
#9622=CARTESIAN_POINT ( 'NONE',  ( -49.14234466229833487, 13.17605306081208205, 60.03827907641571215 ) ) ;
#9623=AXIS2_PLACEMENT_3D ( 'NONE', #40283, #24462, #20205 ) ;
#9627=EDGE_CURVE ( 'NONE', #2888, #52414, #27391, .T. ) ;
#9628=CARTESIAN_POINT ( 'NONE',  ( 131.3924949472282435, 41.12442122814098155, 3.078401348124321757 ) ) ;
#9630=CARTESIAN_POINT ( 'NONE',  ( -55.05276343752908730, 15.72344139423348430, 72.16187836339486239 ) ) ;
#9631=CARTESIAN_POINT ( 'NONE',  ( -107.7886332494339996, 36.81249801143972178, -64.24604545677848932 ) ) ;
#9632=CARTESIAN_POINT ( 'NONE',  ( -53.38256734720888375, 14.24001356352780867, -50.03199302348036781 ) ) ;
#9636=CARTESIAN_POINT ( 'NONE',  ( -31.43908319763710679, -170.0000000000000000, 30.21645440618916112 ) ) ;
#9640=CARTESIAN_POINT ( 'NONE',  ( 34.55626349558410482, 8.840813453039558567, 85.36898312980444814 ) ) ;
#9646=CARTESIAN_POINT ( 'NONE',  ( 31.99894129856764025, 7.561773404408291377, -17.50242361378957412 ) ) ;
#9647=CARTESIAN_POINT ( 'NONE',  ( -80.56139928459657540, 24.13290941644246956, 45.17878892873373076 ) ) ;
#9648=CARTESIAN_POINT ( 'NONE',  ( 161.3124398469970231, 60.70116285586392024, 84.15009968631400739 ) ) ;
#9649=CARTESIAN_POINT ( 'NONE',  ( 92.51858280840789917, 21.51505926344916020, 32.54138647035420462 ) ) ;
#9651=CARTESIAN_POINT ( 'NONE',  ( 104.7227067006896704, 27.50728936118536438, -21.67830293406160891 ) ) ;
#9653=CARTESIAN_POINT ( 'NONE',  ( 12.46277766093406569, 6.416700641561363661, 71.09963920718769259 ) ) ;
#9654=CARTESIAN_POINT ( 'NONE',  ( -190.6985136298601731, 109.1272424661242582, 94.99999999999866418 ) ) ;
#9655=CARTESIAN_POINT ( 'NONE',  ( 197.5344630110112689, 98.61758706718750034, 34.46336747874654094 ) ) ;
#9658=CARTESIAN_POINT ( 'NONE',  ( 157.4703587214989398, -170.0000000000000000, 10.06491688178970456 ) ) ;
#9665=CARTESIAN_POINT ( 'NONE',  ( 112.1009898303695564, 30.86414810229298311, -62.98576819390486037 ) ) ;
#9667=CARTESIAN_POINT ( 'NONE',  ( 201.5903370237274999, 102.1785392640257726, -77.50997439458886618 ) ) ;
#9669=CARTESIAN_POINT ( 'NONE',  ( -36.37229078872272936, 11.47648211215765102, 58.89076057092043470 ) ) ;
#9671=CARTESIAN_POINT ( 'NONE',  ( -118.5043919384111462, 41.81711884544881030, 66.27494688493422359 ) ) ;
#9672=CARTESIAN_POINT ( 'NONE',  ( -86.16504208171679124, 26.41251233979377133, -16.30058366687843829 ) ) ;
#9673=CARTESIAN_POINT ( 'NONE',  ( 17.72992212664810197, 6.570588738776103277, -23.42286153992951725 ) ) ;
#9676=ORIENTED_EDGE ( 'NONE', *, *, #21898, .F. ) ;
#9679=CARTESIAN_POINT ( 'NONE',  ( -79.62207341875657107, 23.76621716825512465, -35.16117203328388285 ) ) ;
#9680=CARTESIAN_POINT ( 'NONE',  ( 163.7607557204680120, 62.71181783708026813, 67.86960462155784057 ) ) ;
#9681=CARTESIAN_POINT ( 'NONE',  ( 113.8626313173126334, 31.71036178495293711, -9.991941754758171257 ) ) ;
#9682=CARTESIAN_POINT ( 'NONE',  ( 186.2722199822850655, 84.01218714714251234, -38.28895599514326875 ) ) ;
#9683=FACE_OUTER_BOUND ( 'NONE', #56398, .T. ) ;
#9684=CARTESIAN_POINT ( 'NONE',  ( -153.7013249156687777, 69.16788179302882611, 85.68575647905826997 ) ) ;
#9688=ORIENTED_EDGE ( 'NONE', *, *, #60121, .F. ) ;
#9690=EDGE_CURVE ( 'NONE', #17040, #51087, #4727, .T. ) ;
#9692=CARTESIAN_POINT ( 'NONE',  ( 108.7042516502346814, 28.17621584866460438, -89.76095026914288155 ) ) ;
#9694=CARTESIAN_POINT ( 'NONE',  ( -34.06637338149494099, 11.05895377318623574, -76.69071157721195675 ) ) ;
#9696=CARTESIAN_POINT ( 'NONE',  ( 185.1710994180822638, 84.30654632312740659, 69.95762266168335941 ) ) ;
#9697=CARTESIAN_POINT ( 'NONE',  ( 46.13705514479446634, 9.381301642376868699, 94.41946954417569771 ) ) ;
#9700=CARTESIAN_POINT ( 'NONE',  ( 187.2465631085774476, 85.06582225041687195, 67.95777364192932168 ) ) ;
#9701=CARTESIAN_POINT ( 'NONE',  ( -119.1795380580999932, 42.22910606512927956, 7.923488756519734721 ) ) ;
#9703=CARTESIAN_POINT ( 'NONE',  ( 127.4750938923429828, 37.70245908594343121, -20.62732788491080527 ) ) ;
#9704=CARTESIAN_POINT ( 'NONE',  ( 16.77104078056616743, 7.540619757007628543, -8.723023917128227112 ) ) ;
#9705=CARTESIAN_POINT ( 'NONE',  ( 12.46490660984525611, 7.423426948220646970, 17.39812806102571230 ) ) ;
#9708=ORIENTED_EDGE ( 'NONE', *, *, #43789, .F. ) ;
#9709=CARTESIAN_POINT ( 'NONE',  ( 188.0081045302010807, 85.89855126821616693, 7.067797300440569863 ) ) ;
#9711=CARTESIAN_POINT ( 'NONE',  ( -132.6811329440527061, 51.12842468617797920, 94.99999999999866418 ) ) ;
#9712=CARTESIAN_POINT ( 'NONE',  ( -31.43908319763710679, 10.61114334766715928, -35.31719736520183517 ) ) ;
#9713=CARTESIAN_POINT ( 'NONE',  ( -109.7156874346698316, 37.87149323084328500, -41.49882581585664099 ) ) ;
#9715=CARTESIAN_POINT ( 'NONE',  ( 185.1660960081724170, 84.30194217633010112, -50.02099752507488262 ) ) ;
#9716=VERTEX_POINT ( 'NONE', #57241 ) ;
#9721=CARTESIAN_POINT ( 'NONE',  ( 197.6341357773624452, 98.74251867088341328, 12.40192937851051624 ) ) ;
#9724=CARTESIAN_POINT ( 'NONE',  ( 115.0454575488273719, 31.16784721673997893, 58.18990905230850785 ) ) ;
#9726=ORIENTED_EDGE ( 'NONE', *, *, #33020, .T. ) ;
#9727=CARTESIAN_POINT ( 'NONE',  ( -57.89360549284268131, 16.50663738101750511, 17.92646098985595771 ) ) ;
#9728=CARTESIAN_POINT ( 'NONE',  ( 133.3990214534117342, 41.14886683286417934, 29.52083177294308669 ) ) ;
#9730=CARTESIAN_POINT ( 'NONE',  ( -100.4466073551322722, 31.85873123265079698, 30.73181422168544685 ) ) ;
#9731=FACE_OUTER_BOUND ( 'NONE', #41243, .T. ) ;
#9737=CARTESIAN_POINT ( 'NONE',  ( -120.1497954511983721, 42.82624472369560209, -20.41821900911190113 ) ) ;
#9739=CARTESIAN_POINT ( 'NONE',  ( -174.7869898116916545, 88.99756909636809610, -8.005991368106910144 ) ) ;
#9740=CARTESIAN_POINT ( 'NONE',  ( -128.3448054685827628, 49.34430406923178225, 57.87263026190729676 ) ) ;
#9742=CARTESIAN_POINT ( 'NONE',  ( -109.6883992247426818, 37.85633120528618178, 90.49244489616368980 ) ) ;
#9747=B_SPLINE_CURVE_WITH_KNOTS ( 'NONE', 3,
 ( #29168, #18960, #8409, #35484, #56946, #18615, #39373, #23204, #28468, #60818, #56238, #45694, #12644, #34106, #34463, #61176, #55541, #40069, #46032, #7721, #50617, #7374, #28826, #67173, #50278, #13343, #2100, #23552, #2435, #61525, #44990, #67498, #66471, #8054, #29506, #19295, #50970, #2782, #40406, #56588, #61854, #13677, #29860 ),
 .UNSPECIFIED., .F., .F.,
 ( 4, 2, 2, 2, 2, 2, 2, 2, 2, 2, 2, 1, 2, 2, 2, 2, 2, 2, 2, 2, 2, 4 ),
 ( 0.02515559250233023042, 0.02674001423437968178, 0.02753222510040440746, 0.02832443596642913314, 0.02990885769847851511, 0.03149327943052789708, 0.03307770116257727905, 0.03386991202860197003, 0.03466212289462666796, 0.03624654462667600829, 0.03703875549270066458, 0.03783096635872532781, 0.03862317722474998410, 0.03941538809077464733, 0.04099980982282398767, 0.04258423155487332801, 0.04337644242089799818, 0.04416865328692266834, 0.04575307501897196011, 0.04733749675102125187, 0.04892191848307054364, 0.05050634021511983540 ),
 .UNSPECIFIED. ) ;
#9749=CARTESIAN_POINT ( 'NONE',  ( -127.6894679065405143, 48.89973668460848444, -61.96241609914127935 ) ) ;
#9750=FACE_OUTER_BOUND ( 'NONE', #64777, .T. ) ;
#9751=CARTESIAN_POINT ( 'NONE',  ( -132.2286325684322605, 52.04087929935081291, 15.29861258695694914 ) ) ;
#9756=DIRECTION ( 'NONE',  ( 0.000000000000000000, 0.000000000000000000, 1.000000000000000000 ) ) ;
#9761=CARTESIAN_POINT ( 'NONE',  ( -72.78270026377323632, 21.23376443558121451, 42.59545495974758467 ) ) ;
#9762=CARTESIAN_POINT ( 'NONE',  ( 83.60262962804348774, 18.41036205028015615, 30.34569721731013558 ) ) ;
#9763=CARTESIAN_POINT ( 'NONE',  ( -148.6409722988650230, 63.44808865916660778, 45.67375462190659618 ) ) ;
#9764=LINE ( 'NONE', #40721, #40692 ) ;
#9765=CARTESIAN_POINT ( 'NONE',  ( -166.3175803736862122, 79.86140754556168986, -65.88834115860622376 ) ) ;
#9767=CARTESIAN_POINT ( 'NONE',  ( -109.7816385129979153, 36.75776661907243437, -16.17071436857322908 ) ) ;
#9768=ADVANCED_FACE ( 'NONE', ( #25924 ), #5147, .F. ) ;
#9769=ORIENTED_EDGE ( 'NONE', *, *, #11261, .T. ) ;
#9776=CARTESIAN_POINT ( 'NONE',  ( 36.31593203568479566, 8.028139509847026289, 3.729209276822607944 ) ) ;
#9777=CARTESIAN_POINT ( 'NONE',  ( -101.8140949286062664, 33.67224128592401655, -61.85912785543960268 ) ) ;
#9778=EDGE_CURVE ( 'NONE', #42183, #52004, #57564, .T. ) ;
#9779=CARTESIAN_POINT ( 'NONE',  ( -38.17232309348611352, 11.81874355808867882, -12.63221164914891226 ) ) ;
#9783=CYLINDRICAL_SURFACE ( 'NONE', #49717, 7.500000000000013323 ) ;
#9785=CARTESIAN_POINT ( 'NONE',  ( -189.5329886872042948, 107.4958891766010538, 9.446604222255606587 ) ) ;
#9787=CARTESIAN_POINT ( 'NONE',  ( -15.08468253268400616, 7.472949889606721463, -71.71047699793288643 ) ) ;
#9789=CARTESIAN_POINT ( 'NONE',  ( 150.5744176759382640, 53.72473166688030233, -46.58491299805970698 ) ) ;
#9791=ORIENTED_EDGE ( 'NONE', *, *, #40759, .T. ) ;
#9792=B_SPLINE_CURVE_WITH_KNOTS ( 'NONE', 3,
 ( #47738, #15058, #20673, #58637, #37536, #69202, #58987, #21027, #42471, #46717, #3811, #63932, #31928, #15743, #10454, #5191, #64273, #53356, #19996, #10807, #21359, #42806, #25279, #31246, #36168, #52676, #41792, #68191, #52343, #25962, #25628, #42130, #47062, #28023, #17109, #38948, #65678, #49821, #5529, #54040, #54751, #49467, #26981, #17467, #59336 ),
 .UNSPECIFIED., .F., .F.,
 ( 4, 2, 2, 1, 2, 2, 2, 2, 2, 2, 2, 2, 2, 2, 2, 2, 2, 2, 2, 2, 2, 2, 4 ),
 ( 0.02346057189573570734, 0.02492590417315489540, 0.02565857031186449116, 0.02639123645057409040, 0.02712390258928368963, 0.02785656872799328540, 0.02932190100541250469, 0.03005456714412212821, 0.03078723328283175520, 0.03225256556025103694, 0.03298523169896067087, 0.03371789783767031173, 0.03518323011508959347, 0.03664856239250887521, 0.03738122853121851608, 0.03811389466992815694, 0.03957922694734743174, 0.04104455922476671348, 0.04250989150218599522, 0.04324255764089562221, 0.04397522377960524920, 0.04544055605702451706, 0.04690588833444379185 ),
 .UNSPECIFIED. ) ;
#9795=CARTESIAN_POINT ( 'NONE',  ( 173.6007744016332310, 72.73482010729016167, -16.29864277669430450 ) ) ;
#9796=ADVANCED_FACE ( 'NONE', ( #58949 ), #44154, .F. ) ;
#9798=CARTESIAN_POINT ( 'NONE',  ( -108.6622665321722963, 37.28993738537004532, 60.91613424318486381 ) ) ;
#9799=CARTESIAN_POINT ( 'NONE',  ( -128.3448054685827913, 49.34430406923178225, -49.50557209994745733 ) ) ;
#9801=CARTESIAN_POINT ( 'NONE',  ( -180.6021503146988891, 97.45669259943414886, -68.43622221639195402 ) ) ;
#9802=CARTESIAN_POINT ( 'NONE',  ( -0.3734056954813043117, 6.520221844775925923, -15.09543421113058592 ) ) ;
#9804=CARTESIAN_POINT ( 'NONE',  ( 203.1423857108908351, 105.9238244286949708, -24.32896508841773908 ) ) ;
#9805=CARTESIAN_POINT ( 'NONE',  ( 93.62778197569794258, 21.92873160988601811, -94.18428683514613908 ) ) ;
#9807=CARTESIAN_POINT ( 'NONE',  ( 141.0645618855930650, 45.95036951196544095, 34.87073521758011907 ) ) ;
#9809=CARTESIAN_POINT ( 'NONE',  ( 198.3926538463959162, 98.07933330386030946, 40.80849878693443600 ) ) ;
#9810=CARTESIAN_POINT ( 'NONE',  ( 117.3110050642448527, 32.29133253383015756, -72.82576982094163043 ) ) ;
#9812=CARTESIAN_POINT ( 'NONE',  ( 188.2950976467627129, 87.71503060978554345, 38.89136225366228672 ) ) ;
#9814=CARTESIAN_POINT ( 'NONE',  ( 46.68054346512387554, -170.0000000000000000, -95.00000000000133582 ) ) ;
#9816=ORIENTED_EDGE ( 'NONE', *, *, #50367, .T. ) ;
#9818=CARTESIAN_POINT ( 'NONE',  ( 8.000000000000007105, 249.8719672152120381, 94.99999999999866418 ) ) ;
#9821=CARTESIAN_POINT ( 'NONE',  ( -77.02372450489325217, 21.70271995013164457, -23.09265542052123976 ) ) ;
#9822=CARTESIAN_POINT ( 'NONE',  ( 70.38121440378671423, 14.50253793787157619, -68.58809608872070385 ) ) ;
#9823=CARTESIAN_POINT ( 'NONE',  ( -62.15799747763097827, 16.70234469631019181, 35.36517553705993322 ) ) ;
#9824=CARTESIAN_POINT ( 'NONE',  ( 153.4509883044095773, 55.84811350575042610, 3.728611983228252491 ) ) ;
#9825=VERTEX_POINT ( 'NONE', #16730 ) ;
#9826=CARTESIAN_POINT ( 'NONE',  ( -180.3158531669106708, 95.51092859788505507, 36.18186780709032746 ) ) ;
#9827=CARTESIAN_POINT ( 'NONE',  ( -55.05276343752909440, 14.68156374112638751, 30.31732777293113301 ) ) ;
#9828=CARTESIAN_POINT ( 'NONE',  ( 110.2429982417149574, 29.99119854320846201, -50.92243756565370916 ) ) ;
#9829=VERTEX_POINT ( 'NONE', #26946 ) ;
#9831=DIRECTION ( 'NONE',  ( -0.8118923937861950435, -0.5838071093367415143, 0.000000000000000000 ) ) ;
#9834=CARTESIAN_POINT ( 'NONE',  ( 138.2204650371258765, 44.12203217345471984, 69.97322756756503281 ) ) ;
#9835=FACE_OUTER_BOUND ( 'NONE', #136, .T. ) ;
#9836=CARTESIAN_POINT ( 'NONE',  ( 149.9838583332408177, 52.05699766415860097, 63.22552044860083242 ) ) ;
#9837=CARTESIAN_POINT ( 'NONE',  ( 94.06416612695406343, 23.16920323269611970, 38.23054147683830450 ) ) ;
#9839=CARTESIAN_POINT ( 'NONE',  ( 46.85361596800669304, 10.51535167202353982, 11.55398794432161047 ) ) ;
#9841=CARTESIAN_POINT ( 'NONE',  ( 150.2805372522807374, 53.51147386362153924, -14.62797420608141685 ) ) ;
#9842=CARTESIAN_POINT ( 'NONE',  ( -60.68849253689218415, 16.26481095007954636, 86.51621802059693778 ) ) ;
#9843=CARTESIAN_POINT ( 'NONE',  ( 105.2529848321548513, 27.73895015262024089, 31.50682025230513972 ) ) ;
#9845=CARTESIAN_POINT ( 'NONE',  ( 55.55684455929184651, 11.06550510321506309, 91.85626868916205012 ) ) ;
#9846=CARTESIAN_POINT ( 'NONE',  ( 181.9411407973024950, 80.91291802046384873, 17.46404351504775221 ) ) ;
#9848=CARTESIAN_POINT ( 'NONE',  ( 210.4897348480409107, 114.6382060222044856, -48.59704500875022148 ) ) ;
#9849=B_SPLINE_CURVE_WITH_KNOTS ( 'NONE', 3,
 ( #46714, #52673, #47735, #41789, #53009, #46357, #4498, #19636, #14704, #31243, #51992, #63245, #36165, #25276, #62558, #35826, #57625, #9092, #3808, #68188, #15055, #9436 ),
 .UNSPECIFIED., .F., .F.,
 ( 4, 2, 2, 2, 2, 2, 2, 2, 2, 2, 4 ),
 ( 0.01188903298721832522, 0.01335733661179801766, 0.01409148842408784741, 0.01482564023637767715, 0.01629394386095731409, 0.01702809567324713863, 0.01776224748553696664, 0.01923055111011659490, 0.02069885473469623011, 0.02216715835927585837, 0.02363546198385549010 ),
 .UNSPECIFIED. ) ;
#9852=ORIENTED_EDGE ( 'NONE', *, *, #40876, .T. ) ;
#9858=CARTESIAN_POINT ( 'NONE',  ( 55.52750043885183828, 11.05966813607792609, -70.55512089573974777 ) ) ;
#9862=CARTESIAN_POINT ( 'NONE',  ( -5.276390875695798677, 6.738249428566100541, 84.24366927175032060 ) ) ;
#9865=ORIENTED_EDGE ( 'NONE', *, *, #29593, .T. ) ;
#9867=CARTESIAN_POINT ( 'NONE',  ( 204.6977192012829789, 106.3443248447423315, -90.01503221354893469 ) ) ;
#9871=CARTESIAN_POINT ( 'NONE',  ( 60.63507185982732040, 12.13307030573224310, -36.10436450079728843 ) ) ;
#9876=CARTESIAN_POINT ( 'NONE',  ( -142.6264002846224059, 58.55577336362197371, 8.380890507460796002 ) ) ;
#9877=EDGE_LOOP ( 'NONE', ( #22982, #24362, #53064, #14384 ) ) ;
#9878=ADVANCED_FACE ( 'NONE', ( #27283 ), #37849, .F. ) ;
#9880=CARTESIAN_POINT ( 'NONE',  ( -132.2286325684321753, 52.04087929935079160, 42.14316317742062523 ) ) ;
#9882=CARTESIAN_POINT ( 'NONE',  ( 17.73567516211396011, 7.577454475141603751, -50.27825812027533914 ) ) ;
#9883=CARTESIAN_POINT ( 'NONE',  ( -145.3233446620410518, 62.00659513626053609, 44.46214151374382340 ) ) ;
#9884=CARTESIAN_POINT ( 'NONE',  ( 207.8484262634767958, 110.7633525054914685, 29.88871051959747049 ) ) ;
#9885=CARTESIAN_POINT ( 'NONE',  ( -5.417282889646090283, 7.753782747238992634, 71.56727370822876821 ) ) ;
#9886=ADVANCED_FACE ( 'NONE', ( #5827 ), #43459, .F. ) ;
#9890=CARTESIAN_POINT ( 'NONE',  ( -132.9421279255324180, 52.54859020878311782, 94.39416510571184915 ) ) ;
#9891=CARTESIAN_POINT ( 'NONE',  ( 33.44035656425387515, 8.720466003183664938, -65.38726348901131757 ) ) ;
#9894=CARTESIAN_POINT ( 'NONE',  ( 8.312979081382955826, 7.382612536522051627, 91.89463208679092077 ) ) ;
#9898=EDGE_LOOP ( 'NONE', ( #63134, #43456, #20793, #28046 ) ) ;
#9899=AXIS2_PLACEMENT_3D ( 'NONE', #1840, #23637, #61610 ) ;
#9900=CARTESIAN_POINT ( 'NONE',  ( -85.75222301046100881, 25.14826148333819233, 13.58240162667133433 ) ) ;
#9901=ORIENTED_EDGE ( 'NONE', *, *, #50361, .F. ) ;
#9904=AXIS2_PLACEMENT_3D ( 'NONE', #1, #63088, #57129 ) ;
#9906=CARTESIAN_POINT ( 'NONE',  ( 11.21387192505586583, 6.397095920409658909, -48.98246565900599592 ) ) ;
#9907=CARTESIAN_POINT ( 'NONE',  ( -173.1211646369891355, 87.12891641440857882, 72.66624519710475738 ) ) ;
#9909=CARTESIAN_POINT ( 'NONE',  ( 129.4987365823222376, 38.85470922756775991, 57.74612764648421859 ) ) ;
#9911=CARTESIAN_POINT ( 'NONE',  ( -26.69041786375498759, 8.859891017920633161, 85.59129543098580939 ) ) ;
#9913=ADVANCED_FACE ( 'NONE', ( #38905 ), #12170, .F. ) ;
#9914=FACE_OUTER_BOUND ( 'NONE', #45544, .T. ) ;
#9916=DIRECTION ( 'NONE',  ( -0.000000000000000000, 1.000000000000000000, -0.000000000000000000 ) ) ;
#9918=CARTESIAN_POINT ( 'NONE',  ( -142.0729208125266325, 59.40063722436773475, -68.01976547901179515 ) ) ;
#9921=CARTESIAN_POINT ( 'NONE',  ( -86.10360257264201778, 26.38663017581291115, -68.45782834547087248 ) ) ;
#9925=CARTESIAN_POINT ( 'NONE',  ( 126.3541873520043737, 37.07520218256171063, 9.666275146592695933 ) ) ;
#9927=EDGE_CURVE ( 'NONE', #41004, #68538, #45854, .T. ) ;
#9930=CARTESIAN_POINT ( 'NONE',  ( 164.4615316623334991, 63.29763980349835606, 7.335938463145385668 ) ) ;
#9933=CARTESIAN_POINT ( 'NONE',  ( -53.82112958582657569, 15.39502561506177436, 84.10151456793303737 ) ) ;
#9939=CARTESIAN_POINT ( 'NONE',  ( 18.19858669090299585, 7.596860100017450712, -62.75709018195347966 ) ) ;
#9941=CARTESIAN_POINT ( 'NONE',  ( -167.6524579626394882, 82.69702609844095775, 33.18325406944033062 ) ) ;
#9943=CARTESIAN_POINT ( 'NONE',  ( 136.7507824285648894, 44.38599729999916121, -36.60034384241509997 ) ) ;
#9944=CARTESIAN_POINT ( 'NONE',  ( 38.42384008295178432, 8.283891555743467805, -35.66795922405820818 ) ) ;
#9945=CARTESIAN_POINT ( 'NONE',  ( 154.0401952541423327, 55.03227529428315279, -36.95059798010156271 ) ) ;
#9951=CARTESIAN_POINT ( 'NONE',  ( 174.4872540107491830, 73.56684916581080813, 86.85688443472005815 ) ) ;
#9961=CARTESIAN_POINT ( 'NONE',  ( 175.5406524085946671, 73.17873692326780599, -75.64701513590247828 ) ) ;
#9963=CARTESIAN_POINT ( 'NONE',  ( 91.49345572560146422, 21.13836538408680354, -22.19096141595985827 ) ) ;
#9964=FACE_OUTER_BOUND ( 'NONE', #66239, .T. ) ;
#9966=EDGE_CURVE ( 'NONE', #52761, #36484, #3008, .T. ) ;
#9967=CARTESIAN_POINT ( 'NONE',  ( 158.3636111008086402, 59.62671916656142912, 71.25401806271710825 ) ) ;
#9969=CARTESIAN_POINT ( 'NONE',  ( 127.2107679985236501, 38.70844091144999055, 13.68070527223361665 ) ) ;
#9971=B_SPLINE_CURVE_WITH_KNOTS ( 'NONE', 3,
 ( #1297, #39285, #18521, #18175, #60727, #61761, #29419, #39625, #62110, #50179, #13249, #34007, #29762, #23462, #45242, #12547, #29082, #3380, #61081, #67077, #51573, #50528, #56849, #13928, #50868, #12908, #40315, #45939, #23800, #35390, #61429, #34364, #51224, #45592, #56146, #34709, #8666, #18867, #28728, #7964, #55446, #66723, #56488 ),
 .UNSPECIFIED., .F., .F.,
 ( 4, 2, 2, 2, 2, 2, 2, 2, 2, 2, 2, 2, 1, 2, 2, 2, 2, 2, 2, 2, 2, 4 ),
 ( 0.02379577142314828753, 0.02527778373276530488, 0.02601878988757380315, 0.02675979604238230489, 0.02824180835199932571, 0.02972382066161635347, 0.03046482681642485868, 0.03120583297123336736, 0.03268784528085037777, 0.03416985759046738125, 0.03565186990008439166, 0.03639287605489288646, 0.03713388220970138126, 0.03787488836450987606, 0.03861589451931837086, 0.04009790682893536046, 0.04157991913855234312, 0.04306193144816933271, 0.04380293760297783445, 0.04454394375778632231, 0.04602595606740331191, 0.04750796837702030151 ),
 .UNSPECIFIED. ) ;
#9973=CARTESIAN_POINT ( 'NONE',  ( -106.6711220790662935, 36.20923238211248929, -75.44417277361526430 ) ) ;
#9974=CARTESIAN_POINT ( 'NONE',  ( -47.80193682758674356, 12.85650137125658077, -44.69689073443416305 ) ) ;
#9975=CARTESIAN_POINT ( 'NONE',  ( -7.504072346567051355, 7.878344583761114350, 83.80449388539848599 ) ) ;
#9976=B_SPLINE_CURVE_WITH_KNOTS ( 'NONE', 3,
 ( #30837, #25222, #13958, #30484, #25567, #41731, #50901, #35417, #46655, #24867, #56884, #8697, #52281, #63189, #51600, #3408, #36453, #57906, #41038, #35772, #24180, #68133, #62847, #36112, #47005, #40345, #68465, #67104, #61792, #35069, #10393, #21303, #25905, #16022, #10744, #63529, #53296, #69135, #37133, #20964, #36803, #5122, #63876, #9728, #4443, #47677 ),
 .UNSPECIFIED., .F., .F.,
 ( 4, 2, 2, 2, 2, 2, 2, 2, 2, 2, 2, 2, 2, 2, 2, 2, 2, 2, 2, 2, 2, 2, 4 ),
 ( 3.179800655392250756E-17, 0.001572224531395685155, 0.003144449062791338217, 0.004716673594186991496, 0.006288898125582645209, 0.007861122656978298054, 0.009433347188373950032, 0.01021945945407176301, 0.01100557171976957599, 0.01179168398546738897, 0.01257779625116520195, 0.01415002078256084699, 0.01493613304825866690, 0.01572224531395648855, 0.01650835757965430847, 0.01729446984535213186, 0.01886669437674773700, 0.01965280664244555345, 0.02043891890814336990, 0.02201114343953899585, 0.02358336797093462528, 0.02436948023663244867, 0.02515559250233026511 ),
 .UNSPECIFIED. ) ;
#9979=CARTESIAN_POINT ( 'NONE',  ( -60.13226458141419073, 16.10241298991027037, 70.18533255850762487 ) ) ;
#9982=CARTESIAN_POINT ( 'NONE',  ( 46.23891277379962617, 10.41636740230860525, 88.00200862900838672 ) ) ;
#9983=CARTESIAN_POINT ( 'NONE',  ( -174.7800083645696532, 88.99302808536934606, -76.38271240644930060 ) ) ;
#9985=EDGE_LOOP ( 'NONE', ( #38162, #68083 ) ) ;
#9988=CARTESIAN_POINT ( 'NONE',  ( 33.76124497394584978, 7.742545529019359662, -11.30815924838790743 ) ) ;
#9989=CARTESIAN_POINT ( 'NONE',  ( 175.0634607207819329, 74.11351956991634893, -39.24529874372897353 ) ) ;
#9992=CARTESIAN_POINT ( 'NONE',  ( 204.6977192012829789, 106.3443248447423599, -24.48138044215792419 ) ) ;
#9995=CARTESIAN_POINT ( 'NONE',  ( 109.3154830994003390, 29.56170298203817381, -24.03505716380648138 ) ) ;
#9998=CARTESIAN_POINT ( 'NONE',  ( 8.540564391411908929, 7.383006541823029067, 35.57011664530912753 ) ) ;
#9999=CARTESIAN_POINT ( 'NONE',  ( 200.4574930424075205, 102.3536505870638251, 42.91127342808825063 ) ) ;
#10004=VERTEX_POINT ( 'NONE', #47278 ) ;
#10010=EDGE_CURVE ( 'NONE', #964, #21211, #8679, .T. ) ;
#10013=CARTESIAN_POINT ( 'NONE',  ( 151.6192474229130198, 53.24103268919213860, -75.16762133081471120 ) ) ;
#10015=CARTESIAN_POINT ( 'NONE',  ( -153.5002794404625490, 67.64160439471096709, -48.66572705198576188 ) ) ;
#10016=EDGE_LOOP ( 'NONE', ( #950, #60613 ) ) ;
#10018=EDGE_LOOP ( 'NONE', ( #13039, #38080, #26577, #24138 ) ) ;
#10021=CARTESIAN_POINT ( 'NONE',  ( -81.24432217070638274, 24.40203426192924852, -35.56837079089353182 ) ) ;
#10022=CARTESIAN_POINT ( 'NONE',  ( 163.1495034066983862, 62.20479872133083887, 68.67890006866612396 ) ) ;
#10023=CARTESIAN_POINT ( 'NONE',  ( -156.7435307435794130, 71.93726016406968427, 9.383933217110650205 ) ) ;
#10027=VERTEX_POINT ( 'NONE', #25162 ) ;
#10028=ORIENTED_EDGE ( 'NONE', *, *, #60738, .T. ) ;
#10030=CARTESIAN_POINT ( 'NONE',  ( 32.90051628396145134, 8.664124555952449569, -46.89117901519352927 ) ) ;
#10032=CARTESIAN_POINT ( 'NONE',  ( -33.83721310978700814, 11.01869210665939569, -76.77220433069990690 ) ) ;
#10033=CARTESIAN_POINT ( 'NONE',  ( 197.5344630110112973, 98.61758706718748613, 61.30791806921028808 ) ) ;
#10035=CARTESIAN_POINT ( 'NONE',  ( 35.65775178405256440, 7.951994368745589625, 57.75521004793950652 ) ) ;
#10036=CARTESIAN_POINT ( 'NONE',  ( -173.1211646369891355, -170.0000000000000000, -69.05650775521368701 ) ) ;
#10037=CARTESIAN_POINT ( 'NONE',  ( -6.840981040171508099, 6.828436339979229608, -35.46654583414340323 ) ) ;
#10043=CARTESIAN_POINT ( 'NONE',  ( 10.83521140779424385, 7.398743030771590234, 5.017172746912176962 ) ) ;
#10046=CARTESIAN_POINT ( 'NONE',  ( 181.5127080940606845, 79.03904173130086974, 17.46404351504774510 ) ) ;
#10048=CARTESIAN_POINT ( 'NONE',  ( 175.8855729601531834, 73.50624012737691260, 31.38118644907393673 ) ) ;
#10052=CARTESIAN_POINT ( 'NONE',  ( 188.2950976467627129, 87.71503060978560029, -41.64228951772874154 ) ) ;
#10053=ORIENTED_EDGE ( 'NONE', *, *, #15518, .T. ) ;
#10056=CARTESIAN_POINT ( 'NONE',  ( 173.6797811602132811, 71.43321480276107138, 89.28613363591487939 ) ) ;
#10058=CARTESIAN_POINT ( 'NONE',  ( 112.7784411285249035, 30.07270878825233140, 56.89340532513772786 ) ) ;
#10060=CARTESIAN_POINT ( 'NONE',  ( 128.0540543950622521, 39.18660671946769014, -65.58941647092106564 ) ) ;
#10061=CARTESIAN_POINT ( 'NONE',  ( 8.000000000000007105, 249.8719672152120381, 94.99999999999866418 ) ) ;
#10064=CARTESIAN_POINT ( 'NONE',  ( 160.3358006062388199, 59.91363101085903509, -90.37214895256691705 ) ) ;
#10065=EDGE_CURVE ( 'NONE', #16002, #47540, #27781, .T. ) ;
#10066=CARTESIAN_POINT ( 'NONE',  ( 94.12811352634518869, 22.11743943276050217, -43.84554527026892146 ) ) ;
#10071=ORIENTED_EDGE ( 'NONE', *, *, #19714, .T. ) ;
#10073=CARTESIAN_POINT ( 'NONE',  ( -119.5576859660651365, 42.46117483543969939, -19.59024322217818792 ) ) ;
#10076=CARTESIAN_POINT ( 'NONE',  ( -180.5230320745700681, 95.76406004447549947, -16.61624996634525786 ) ) ;
#10079=CARTESIAN_POINT ( 'NONE',  ( -109.2878468539942816, 37.63446276172139449, 94.40069165669748941 ) ) ;
#10082=ORIENTED_EDGE ( 'NONE', *, *, #1936, .F. ) ;
#10083=CARTESIAN_POINT ( 'NONE',  ( -60.97727891098333686, 16.35024395194893287, -20.49696293675446412 ) ) ;
#10086=CARTESIAN_POINT ( 'NONE',  ( -94.85061234775062644, 29.16417548023187223, 10.11651724366670457 ) ) ;
#10087=CARTESIAN_POINT ( 'NONE',  ( -98.69283175933883001, 30.99524616306738523, -75.96291905404460465 ) ) ;
#10090=ORIENTED_EDGE ( 'NONE', *, *, #39111, .T. ) ;
#10093=CARTESIAN_POINT ( 'NONE',  ( -166.3188283541502699, 79.86268666707378827, -45.38284161879311540 ) ) ;
#10098=CARTESIAN_POINT ( 'NONE',  ( -71.27103490383372275, 20.70545763375144332, 39.19188336387009741 ) ) ;
#10099=CARTESIAN_POINT ( 'NONE',  ( 84.05098130332766004, 18.55728792516086756, 44.25912196898673301 ) ) ;
#10101=CARTESIAN_POINT ( 'NONE',  ( -119.2949674747224833, 43.48097822533565449, 41.72283548570154466 ) ) ;
#10105=ORIENTED_EDGE ( 'NONE', *, *, #59946, .F. ) ;
#10106=CARTESIAN_POINT ( 'NONE',  ( -14.55425570676092129, 7.423011834016145727, -39.59648726401223229 ) ) ;
#10107=CARTESIAN_POINT ( 'NONE',  ( 86.14890207173843351, 20.31981596387580424, 71.55663816294304524 ) ) ;
#10108=CARTESIAN_POINT ( 'NONE',  ( -80.34986779050261418, 22.96961150679207719, -88.98360521546140944 ) ) ;
#10110=CARTESIAN_POINT ( 'NONE',  ( 32.66883187925819243, 8.640402022338113497, 7.229089490855268529 ) ) ;
#10112=CARTESIAN_POINT ( 'NONE',  ( 33.03621582719334526, 7.666716336587111158, -73.93768929495423947 ) ) ;
#10113=CARTESIAN_POINT ( 'NONE',  ( -96.43817545481738307, 31.02509717589733640, -74.08903276496864976 ) ) ;
#10114=DIRECTION ( 'NONE',  ( -0.000000000000000000, 1.000000000000000000, -0.000000000000000000 ) ) ;
#10116=CYLINDRICAL_SURFACE ( 'NONE', #40999, 7.500000000000020428 ) ;
#10120=CARTESIAN_POINT ( 'NONE',  ( -189.3111515777349894, 107.1887855376296699, 12.66640944553473069 ) ) ;
#10122=CARTESIAN_POINT ( 'NONE',  ( -15.07200981767290493, 7.471751903425211339, -67.81403541448362660 ) ) ;
#10124=CARTESIAN_POINT ( 'NONE',  ( 150.0278556977734468, 53.32860603304212788, -42.54581402127228529 ) ) ;
#10129=CARTESIAN_POINT ( 'NONE',  ( 173.9457771591584390, 73.05793967547533896, -19.19921062527386368 ) ) ;
#10131=DIRECTION ( 'NONE',  ( -0.000000000000000000, 1.000000000000000000, -0.000000000000000000 ) ) ;
#10133=DIRECTION ( 'NONE',  ( -0.000000000000000000, 1.000000000000000000, -0.000000000000000000 ) ) ;
#10135=CARTESIAN_POINT ( 'NONE',  ( -1.857619870843141952, 6.575690665396231260, -11.50454659054918949 ) ) ;
#10136=CARTESIAN_POINT ( 'NONE',  ( 197.2847860006354779, 98.30530166401517533, -18.13261055250281473 ) ) ;
#10137=CARTESIAN_POINT ( 'NONE',  ( -152.2442544045799480, 66.53514540059047988, 84.90555898563886217 ) ) ;
#10138=CARTESIAN_POINT ( 'NONE',  ( 139.2921620648436942, 44.80435067172504660, 31.81952079417536083 ) ) ;
#10141=FACE_OUTER_BOUND ( 'NONE', #59352, .T. ) ;
#10142=CARTESIAN_POINT ( 'NONE',  ( 153.4509883044095773, 55.84811350575044031, 30.57316257369191703 ) ) ;
#10147=ADVANCED_FACE ( 'NONE', ( #26180 ), #31461, .F. ) ;
#10149=CARTESIAN_POINT ( 'NONE',  ( -109.7647482398635361, 36.74843029291201191, -41.96704509549551432 ) ) ;
#10150=CARTESIAN_POINT ( 'NONE',  ( 69.49862690228275142, 14.27023134440512386, -73.86852559465907575 ) ) ;
#10154=CARTESIAN_POINT ( 'NONE',  ( -179.2262621278718200, 94.19039042964671182, 42.70701387388177750 ) ) ;
#10156=VECTOR ( 'NONE', #2409, 1000.000000000000000 ) ;
#10158=CARTESIAN_POINT ( 'NONE',  ( 113.4402889550712530, 31.50582881646776912, -36.62137660074326106 ) ) ;
#10160=CYLINDRICAL_SURFACE ( 'NONE', #45720, 7.500000000000020428 ) ;
#10161=CARTESIAN_POINT ( 'NONE',  ( 137.3958226571046453, 43.60243650158411555, 57.22592436439141039 ) ) ;
#10162=CARTESIAN_POINT ( 'NONE',  ( 63.01563776193091826, 13.70579113808095073, 2.968410348757589468 ) ) ;
#10164=CARTESIAN_POINT ( 'NONE',  ( 186.6054783416232112, 84.37128553200975034, -21.98102405639298595 ) ) ;
#10167=CARTESIAN_POINT ( 'NONE',  ( 46.23304607317101045, 10.41544405387737982, 7.463327010731485522 ) ) ;
#10172=CARTESIAN_POINT ( 'NONE',  ( -62.41607942644581897, 16.78015853244291478, 89.94130366719888059 ) ) ;
#10175=CARTESIAN_POINT ( 'NONE',  ( 70.37328515878277813, 14.50043699572714040, 89.50955696056523436 ) ) ;
#10177=CARTESIAN_POINT ( 'NONE',  ( 212.1707951106655514, 117.1901534358505899, -43.16799237652320187 ) ) ;
#10179=VERTEX_POINT ( 'NONE', #14589 ) ;
#10181=ORIENTED_EDGE ( 'NONE', *, *, #13431, .T. ) ;
#10182=CARTESIAN_POINT ( 'NONE',  ( 181.0840389613909736, -170.0000000000000000, 29.30859410551139277 ) ) ;
#10183=CARTESIAN_POINT ( 'NONE',  ( 60.40277045393652600, 12.08176563382370183, -63.03086484206352225 ) ) ;
#10184=CARTESIAN_POINT ( 'NONE',  ( -122.3994536713185255, 45.42826354555015911, 71.60485157671216427 ) ) ;
#10186=CARTESIAN_POINT ( 'NONE',  ( 164.0073343966822392, 64.23003864582459244, -66.78297849933632335 ) ) ;
#10188=CARTESIAN_POINT ( 'NONE',  ( -72.20490592113146988, 19.96451062593607872, 68.60262606855620504 ) ) ;
#10189=CARTESIAN_POINT ( 'NONE',  ( 199.3110346421775603, 99.23841336744848718, -92.27908572396052023 ) ) ;
#10192=CARTESIAN_POINT ( 'NONE',  ( -156.9252506979473196, 70.73559306219777909, 37.07661470075439070 ) ) ;
#10195=DIRECTION ( 'NONE',  ( -0.000000000000000000, 1.000000000000000000, -0.000000000000000000 ) ) ;
#10199=CARTESIAN_POINT ( 'NONE',  ( -132.8150886319752146, 52.45790550853838852, 35.21935937789461235 ) ) ;
#10201=CARTESIAN_POINT ( 'NONE',  ( 206.3125232506202735, 108.5822159704961933, 17.19853195675947788 ) ) ;
#10202=CARTESIAN_POINT ( 'NONE',  ( -143.2498117110515068, 60.33382252735059126, 34.07831714178427518 ) ) ;
#10204=CARTESIAN_POINT ( 'NONE',  ( 208.6132326550593916, 111.8685719053116543, 43.11846758867611129 ) ) ;
#10206=CARTESIAN_POINT ( 'NONE',  ( -1.455067768715155196, 7.566780179921179794, 68.42619738054045797 ) ) ;
#10211=ORIENTED_EDGE ( 'NONE', *, *, #25898, .T. ) ;
#10212=ORIENTED_EDGE ( 'NONE', *, *, #43336, .T. ) ;
#10214=CARTESIAN_POINT ( 'NONE',  ( -190.6985136298601731, 109.1272424661242582, -95.00000000000133582 ) ) ;
#10215=CARTESIAN_POINT ( 'NONE',  ( -171.4867114763003997, 85.32693843184996751, -22.69890371670287266 ) ) ;
#10219=CARTESIAN_POINT ( 'NONE',  ( 8.747314885369917192, 7.383532170996436328, 93.80849556495012109 ) ) ;
#10220=B_SPLINE_CURVE_WITH_KNOTS ( 'NONE', 3,
 ( #16061, #27301, #58966, #54017, #48743, #11128, #582, #58278, #10780, #64602, #47717, #16410, #25938, #32253, #5507, #21004, #15722, #59650, #44537, #50162, #28001, #66018, #22735, #54731, #17089, #60713, #38923, #44169, #50511, #17814, #54373, #1625, #38212, #11465, #12529, #7259, #39610, #44885, #23447, #18157, #49445, #1990, #39269, #33301, #23090 ),
 .UNSPECIFIED., .F., .F.,
 ( 4, 2, 2, 2, 2, 2, 2, 2, 2, 2, 2, 1, 2, 2, 2, 2, 2, 2, 2, 2, 2, 2, 4 ),
 ( 0.000000000000000000, 0.001512548138464782236, 0.002268822207697173462, 0.003025096276929564471, 0.004537644415394318301, 0.005293918484626675483, 0.006050192553859033533, 0.007562740692323722744, 0.009075288830788411087, 0.01058783696925309943, 0.01134411103848542365, 0.01210038510771774788, 0.01285665917695007210, 0.01361293324618239459, 0.01512548138464699446, 0.01588175545387929613, 0.01663802952311159433, 0.01815057766157616645, 0.01966312580004073510, 0.02041939986927301942, 0.02117567393850530028, 0.02268822207696985158, 0.02420077021543439941 ),
 .UNSPECIFIED. ) ;
#10221=VERTEX_POINT ( 'NONE', #37764 ) ;
#10232=CARTESIAN_POINT ( 'NONE',  ( -119.2804658695888094, 43.47213805166352785, 7.728477835248403593 ) ) ;
#10234=CARTESIAN_POINT ( 'NONE',  ( -175.9852529046322331, 90.37283472601130541, 72.11072863597617300 ) ) ;
#10235=CARTESIAN_POINT ( 'NONE',  ( 126.8237978310705358, 37.33705012421154379, 66.47361518080877829 ) ) ;
#10236=EDGE_LOOP ( 'NONE', ( #13576, #37625, #11876, #47673 ) ) ;
#10237=CARTESIAN_POINT ( 'NONE',  ( -25.36310660490340396, 8.672627506263530961, 86.99672183978204032 ) ) ;
#10240=CARTESIAN_POINT ( 'NONE',  ( 109.7724924842965919, 28.66436020578543520, -35.92243756565368784 ) ) ;
#10242=CARTESIAN_POINT ( 'NONE',  ( -24.41864932425148993, 8.543938959778817122, 40.36687269096346853 ) ) ;
#10245=AXIS2_PLACEMENT_3D ( 'NONE', #21288, #41713, #63174 ) ;
#10247=ADVANCED_FACE ( 'NONE', ( #27202 ), #53584, .F. ) ;
#10250=CARTESIAN_POINT ( 'NONE',  ( -79.61235761536667610, 23.76245710489569518, -76.91537820575416617 ) ) ;
#10251=CARTESIAN_POINT ( 'NONE',  ( 173.9457771591584105, 73.05793967547531054, 7.645339965189813292 ) ) ;
#10253=CARTESIAN_POINT ( 'NONE',  ( 8.000000000000007105, 249.8719672152120381, -95.00000000000133582 ) ) ;
#10255=CARTESIAN_POINT ( 'NONE',  ( 36.77263075747509902, 8.082075437684869357, -89.78184162056548701 ) ) ;
#10256=CARTESIAN_POINT ( 'NONE',  ( 197.2450958997033865, 98.25574850261155291, 91.26861472641076034 ) ) ;
#10258=CARTESIAN_POINT ( 'NONE',  ( 70.51484748609223630, 14.53801151001411363, 9.956432264353654915 ) ) ;
#10260=CARTESIAN_POINT ( 'NONE',  ( 157.4703587214989113, 57.65129005721576760, 2.564916881789689018 ) ) ;
#10263=CARTESIAN_POINT ( 'NONE',  ( -49.42889165003705187, 14.28050133789322018, 86.50253100448308885 ) ) ;
#10264=VERTEX_POINT ( 'NONE', #26869 ) ;
#10267=CARTESIAN_POINT ( 'NONE',  ( 22.15943197741200521, 7.796127622097903220, -73.82810297161255164 ) ) ;
#10268=CARTESIAN_POINT ( 'NONE',  ( -149.5074843970971017, 65.50121172469319220, 72.56537183036277838 ) ) ;
#10269=DIRECTION ( 'NONE',  ( -0.000000000000000000, 1.000000000000000000, -0.000000000000000000 ) ) ;
#10271=CARTESIAN_POINT ( 'NONE',  ( 139.3041645503688528, 46.00819478311334620, -48.68433813850839442 ) ) ;
#10272=CARTESIAN_POINT ( 'NONE',  ( 207.3574376820450595, 111.8208281420536707, -90.49371098840704519 ) ) ;
#10279=CARTESIAN_POINT ( 'NONE',  ( 128.3483068049043538, 39.35455865146280274, -92.10653312658361358 ) ) ;
#10280=CARTESIAN_POINT ( 'NONE',  ( 66.89344749234535925, 14.64254390099354985, -90.47725094589908679 ) ) ;
#10281=CARTESIAN_POINT ( 'NONE',  ( 92.52113039222221857, 22.58921125235803018, 15.03444035171357740 ) ) ;
#10282=CARTESIAN_POINT ( 'NONE',  ( 185.5457097283154724, 84.70846743303873438, -10.83386876099697282 ) ) ;
#10283=CARTESIAN_POINT ( 'NONE',  ( -86.06016868996614733, 25.27707703029502539, -14.48738519166817440 ) ) ;
#10285=CARTESIAN_POINT ( 'NONE',  ( -179.5082312244189495, 94.53075638132058600, -46.15200650400738169 ) ) ;
#10286=CARTESIAN_POINT ( 'NONE',  ( 92.53566308513171634, 21.52138666710686721, -11.82835652178502706 ) ) ;
#10296=CARTESIAN_POINT ( 'NONE',  ( 151.3136733342017237, 54.26417151662144533, 68.04466391889920374 ) ) ;
#10299=CARTESIAN_POINT ( 'NONE',  ( -6.210370628187416919, 7.798947244808402957, 83.97346081649014593 ) ) ;
#10309=EDGE_CURVE ( 'NONE', #52004, #42183, #31519, .T. ) ;
#10310=VERTEX_POINT ( 'NONE', #40206 ) ;
#10311=CARTESIAN_POINT ( 'NONE',  ( 32.57244506765509584, 8.630607406489110289, 87.98557846726629350 ) ) ;
#10313=CARTESIAN_POINT ( 'NONE',  ( 39.40195752203892710, 9.424259417798133143, -77.46436805589148378 ) ) ;
#10319=CARTESIAN_POINT ( 'NONE',  ( -3.253130881186330647, 7.643323950922364496, 4.805877217267385149 ) ) ;
#10320=CARTESIAN_POINT ( 'NONE',  ( 173.8623159076319951, 72.97967239795019623, -45.76964742264968322 ) ) ;
#10321=CARTESIAN_POINT ( 'NONE',  ( 160.5022159022404367, 60.04643339566187876, 83.71124699655744905 ) ) ;
#10323=ORIENTED_EDGE ( 'NONE', *, *, #53799, .F. ) ;
#10325=B_SPLINE_CURVE_WITH_KNOTS ( 'NONE', 3,
 ( #69314, #27086, #43610, #43253, #21140, #42582, #64733, #32724, #64038, #37996, #54148, #15847, #58742, #65080, #10565, #5973, #48869, #52773, #58074, #49228, #55214, #44310, #23226, #45005, #39392, #65791, #50298, #28847, #55925, #12663, #55563, #66843, #33775, #7738, #22513, #2456, #23910, #44675, #34125, #54502, #50632, #60143, #29190 ),
 .UNSPECIFIED., .F., .F.,
 ( 4, 2, 2, 2, 2, 2, 2, 2, 2, 2, 2, 1, 2, 2, 2, 2, 2, 2, 2, 2, 2, 4 ),
 ( 0.02515559250233022348, 0.02674001423437951525, 0.02753222510040416460, 0.02832443596642881742, 0.02990885769847818204, 0.03149327943052755013, 0.03307770116257691129, 0.03386991202860161615, 0.03466212289462632101, 0.03624654462667572380, 0.03703875549270041478, 0.03783096635872511271, 0.03862317722474981063, 0.03941538809077450162, 0.04099980982282387665, 0.04258423155487325168, 0.04337644242089793573, 0.04416865328692261977, 0.04575307501897192541, 0.04733749675102122412, 0.04892191848307052976, 0.05050634021511983540 ),
 .UNSPECIFIED. ) ;
#10328=CARTESIAN_POINT ( 'NONE',  ( 197.1979149960397990, 98.19687999752002838, 36.37236663005180759 ) ) ;
#10331=ORIENTED_EDGE ( 'NONE', *, *, #138, .T. ) ;
#10332=ORIENTED_EDGE ( 'NONE', *, *, #27544, .F. ) ;
#10339=EDGE_CURVE ( 'NONE', #56789, #54495, #34243, .T. ) ;
#10340=CARTESIAN_POINT ( 'NONE',  ( -32.40928421737412179, 10.77259363352673205, 57.10791823073882512 ) ) ;
#10342=CARTESIAN_POINT ( 'NONE',  ( 152.1190604254710479, 53.60705199010334354, -75.72949298238010840 ) ) ;
#10349=CARTESIAN_POINT ( 'NONE',  ( -81.00768240531208164, 24.30850321514433432, -49.74466447296814664 ) ) ;
#10350=CARTESIAN_POINT ( 'NONE',  ( 159.6725804802005371, 59.38339663535509771, 70.93746766617782384 ) ) ;
#10351=CARTESIAN_POINT ( 'NONE',  ( -150.3850953947692517, 66.25368649589887582, 18.83771815676428574 ) ) ;
#10354=CARTESIAN_POINT ( 'NONE',  ( 15.78827728214693416, 6.500811158483329244, 45.01470767270524931 ) ) ;
#10355=CARTESIAN_POINT ( 'NONE',  ( -156.9757241921502953, 72.15252929097994183, 92.68305819821679847 ) ) ;
#10360=CARTESIAN_POINT ( 'NONE',  ( 35.65622260226239604, 8.964590916200315007, -36.61753697201972813 ) ) ;
#10363=CARTESIAN_POINT ( 'NONE',  ( -37.92542950990691963, 10.74638084523342130, 60.78760712818166212 ) ) ;
#10366=CARTESIAN_POINT ( 'NONE',  ( 186.0827296088607170, 85.28826835108064586, 69.24936458491407620 ) ) ;
#10367=CARTESIAN_POINT ( 'NONE',  ( 8.336031647119270360, 6.376437040857336314, -15.19577221354909824 ) ) ;
#10371=CARTESIAN_POINT ( 'NONE',  ( -83.12901536265221125, 24.07178615860086168, -36.58265565400330388 ) ) ;
#10372=CARTESIAN_POINT ( 'NONE',  ( 15.78827728214693060, 6.500811158483329244, 71.85925826316895382 ) ) ;
#10374=CARTESIAN_POINT ( 'NONE',  ( 8.540564391411908929, 7.383006541823030844, 8.725566054845465658 ) ) ;
#10380=LINE ( 'NONE', #48338, #10695 ) ;
#10381=CARTESIAN_POINT ( 'NONE',  ( -108.9444157621018547, 37.44493815491211564, -39.03547156667866602 ) ) ;
#10385=CARTESIAN_POINT ( 'NONE',  ( -26.49516976694650339, 8.831756547364850718, -10.31156455694099883 ) ) ;
#10387=CARTESIAN_POINT ( 'NONE',  ( 197.3064269725219333, 98.33232022113057269, 11.17706977006253766 ) ) ;
#10388=ORIENTED_EDGE ( 'NONE', *, *, #12502, .F. ) ;
#10390=CARTESIAN_POINT ( 'NONE',  ( 112.5554747942046134, 29.96654954475022237, 56.81725345967257113 ) ) ;
#10392=CARTESIAN_POINT ( 'NONE',  ( 86.62931800182293784, 19.42108912189600645, -8.977013608448025650 ) ) ;
#10393=CARTESIAN_POINT ( 'NONE',  ( 127.6144785300460143, 37.78099129859914740, 32.84513397848537153 ) ) ;
#10403=VERTEX_POINT ( 'NONE', #56729 ) ;
#10404=VECTOR ( 'NONE', #35125, 1000.000000000000000 ) ;
#10406=CARTESIAN_POINT ( 'NONE',  ( -125.4481990864046423, 46.20056605584957055, -23.06915330777029993 ) ) ;
#10409=CARTESIAN_POINT ( 'NONE',  ( -180.4643341113398378, 95.69224917234933514, -13.81201931865484589 ) ) ;
#10411=CARTESIAN_POINT ( 'NONE',  ( -142.4991775570125299, 58.45550857435406300, -39.58818248682278096 ) ) ;
#10413=CYLINDRICAL_SURFACE ( 'NONE', #25232, 7.500000000000013323 ) ;
#10416=CARTESIAN_POINT ( 'NONE',  ( -133.3149301983942507, 51.57857650535022032, 39.23854680323682231 ) ) ;
#10417=CARTESIAN_POINT ( 'NONE',  ( -62.45356936877016807, 16.79156452995241366, -17.11305785722446160 ) ) ;
#10419=CARTESIAN_POINT ( 'NONE',  ( 79.23200707685333555, 17.02828389812517074, -15.21462584625181691 ) ) ;
#10420=CARTESIAN_POINT ( 'NONE',  ( -125.8938041572051389, 47.69968343338778283, -76.75825448869764500 ) ) ;
#10423=CARTESIAN_POINT ( 'NONE',  ( -99.10260179032844974, 31.19580119595417855, -62.56131912884078616 ) ) ;
#10426=B_SPLINE_CURVE_WITH_KNOTS ( 'NONE', 3,
 ( #69353, #31382, #35966, #4308, #51798, #15548, #31041, #31718, #57420, #4982, #20466, #52486, #46865, #3607, #9235, #68331, #30690, #36660, #26450, #47887, #21172, #64073, #58782, #52141, #3958, #20131, #25075, #54897, #44347, #6721, #21500, #27828, #6010, #38033, #32758, #43643, #28165, #22206, #53504, #43993, #37681, #42947, #49266, #64417, #33112, #6374 ),
 .UNSPECIFIED., .F., .F.,
 ( 4, 2, 2, 2, 2, 2, 2, 2, 2, 2, 2, 2, 2, 2, 2, 2, 2, 2, 2, 2, 2, 2, 4 ),
 ( 6.938893903907228378E-18, 0.003192770216278258480, 0.003990962770347825268, 0.004789155324417392924, 0.006385540432556518695, 0.007183732986626099361, 0.007981925540695681762, 0.009578310648834874319, 0.01037650320290446106, 0.01117469575697404606, 0.01197288831104363106, 0.01277108086511321607, 0.01436746597325242771, 0.01596385108139163761, 0.01676204363546123649, 0.01756023618953083190, 0.01835842874360043078, 0.01915662129767002619, 0.02075300640580920661, 0.02234939151394838355, 0.02394577662208756397, 0.02474396917615715244, 0.02554216173022674438 ),
 .UNSPECIFIED. ) ;
#10427=CARTESIAN_POINT ( 'NONE',  ( 188.4359598230020651, 86.36951380984525883, -72.08147103809925227 ) ) ;
#10428=CARTESIAN_POINT ( 'NONE',  ( 14.80205238535217127, 6.470775952815775334, 30.06371155530308670 ) ) ;
#10429=DIRECTION ( 'NONE',  ( -0.8118923937861950435, -0.5838071093367415143, 0.000000000000000000 ) ) ;
#10431=FACE_OUTER_BOUND ( 'NONE', #61194, .T. ) ;
#10432=CARTESIAN_POINT ( 'NONE',  ( -74.79539698934961223, 21.95498232236883851, 31.48986615712328430 ) ) ;
#10433=CARTESIAN_POINT ( 'NONE',  ( 84.97343609940688225, 18.86260005312943377, 44.53087885251839140 ) ) ;
#10434=CARTESIAN_POINT ( 'NONE',  ( 68.94948716683070700, 15.16699441119057923, -47.83381367184613708 ) ) ;
#10435=CARTESIAN_POINT ( 'NONE',  ( -118.6727642982647239, 43.09863379477474865, 36.02294872542282889 ) ) ;
#10436=CARTESIAN_POINT ( 'NONE',  ( 212.0739503583954217, 117.0412199804969617, 62.15368347199733279 ) ) ;
#10437=ORIENTED_EDGE ( 'NONE', *, *, #35607, .T. ) ;
#10438=CARTESIAN_POINT ( 'NONE',  ( -108.5289085648060734, 36.07014995015116909, -11.51505029103895517 ) ) ;
#10440=CARTESIAN_POINT ( 'NONE',  ( -15.07200981767291204, 7.471751903425211339, -40.96948482401995761 ) ) ;
#10443=CARTESIAN_POINT ( 'NONE',  ( 87.11239765416380010, 20.65008247340817960, 71.55663816294303103 ) ) ;
#10444=CARTESIAN_POINT ( 'NONE',  ( 151.7956716830626647, 53.36999433148314154, -11.86948592691346605 ) ) ;
#10446=CARTESIAN_POINT ( 'NONE',  ( 31.99894129856762603, 7.561773404408291377, -71.19152479471692629 ) ) ;
#10448=VECTOR ( 'NONE', #21509, 1000.000000000000000 ) ;
#10453=CARTESIAN_POINT ( 'NONE',  ( 60.40531521312254171, 13.11276739283242421, 57.12225848735855038 ) ) ;
#10454=CARTESIAN_POINT ( 'NONE',  ( 9.837735240994025077, 7.389327806910503504, -74.43536120031389203 ) ) ;
#10460=CARTESIAN_POINT ( 'NONE',  ( -99.10260179032840711, 31.19580119595418211, -8.872217947913421554 ) ) ;
#10462=CARTESIAN_POINT ( 'NONE',  ( 79.94135235523673089, 18.29982848521581928, 87.49016971473862725 ) ) ;
#10463=EDGE_CURVE ( 'NONE', #22089, #47869, #8889, .T. ) ;
#10465=ORIENTED_EDGE ( 'NONE', *, *, #41864, .F. ) ;
#10471=CARTESIAN_POINT ( 'NONE',  ( -109.7811201291769834, 37.90784085457603680, 65.09395327358092231 ) ) ;
#10472=CARTESIAN_POINT ( 'NONE',  ( -130.5904357464318366, 50.88938808445631423, -36.54610296849261886 ) ) ;
#10475=CARTESIAN_POINT ( 'NONE',  ( -5.416136198635864041, 6.745992685878658079, -23.18025356100167045 ) ) ;
#10476=CARTESIAN_POINT ( 'NONE',  ( 197.1975259970232059, 98.19639476549650681, -16.65484193907906629 ) ) ;
#10479=CARTESIAN_POINT ( 'NONE',  ( 140.2332932573541484, 45.41010019581507606, 40.99038388568915536 ) ) ;
#10484=CARTESIAN_POINT ( 'NONE',  ( 160.5018603162734792, 61.33906090758087259, 3.190259315126446449 ) ) ;
#10489=CARTESIAN_POINT ( 'NONE',  ( -108.5289085648060308, 36.07014995015116199, -38.35960088150262237 ) ) ;
#10492=CARTESIAN_POINT ( 'NONE',  ( -60.97011009284708649, 16.34812508431679490, 42.45179124754056943 ) ) ;
#10494=CARTESIAN_POINT ( 'NONE',  ( 156.5890478960376981, 58.24007662587946754, 17.52612138860288837 ) ) ;
#10496=CARTESIAN_POINT ( 'NONE',  ( -180.4654253355437277, 95.69358270527506249, 36.77113452514563363 ) ) ;
#10498=LINE ( 'NONE', #42518, #62031 ) ;
#10504=CARTESIAN_POINT ( 'NONE',  ( -169.8791831685529985, 83.59058982490282119, 45.09941841846899990 ) ) ;
#10506=CARTESIAN_POINT ( 'NONE',  ( -31.92580063159128301, 9.671320706097199960, -77.16174795566554678 ) ) ;
#10512=CARTESIAN_POINT ( 'NONE',  ( 212.0803491126037557, 118.9047894217573571, -15.61684406194017960 ) ) ;
#10514=CARTESIAN_POINT ( 'NONE',  ( -156.3790798118594410, 70.23422112803311279, -72.17447922398677917 ) ) ;
#10515=CARTESIAN_POINT ( 'NONE',  ( -108.6669825835168268, 36.14542924967227577, 87.76374826371203142 ) ) ;
#10520=CARTESIAN_POINT ( 'NONE',  ( -102.2801239173131052, 33.91021738430208643, -88.70367844590326456 ) ) ;
#10522=CARTESIAN_POINT ( 'NONE',  ( -71.42546113164833343, 20.75891408601220078, 66.78154372501096248 ) ) ;
#10523=CARTESIAN_POINT ( 'NONE',  ( 211.0967808702091588, 115.5516932918877018, -74.59216173768591318 ) ) ;
#10525=CARTESIAN_POINT ( 'NONE',  ( -71.56718866013694935, 19.74312628447964002, 13.54490632388451843 ) ) ;
#10526=CARTESIAN_POINT ( 'NONE',  ( -120.5002574492099114, 44.22930148497322023, 70.18197274062502800 ) ) ;
#10527=CARTESIAN_POINT ( 'NONE',  ( 15.78827728214693416, 7.507518794609589818, 30.01470767270522089 ) ) ;
#10528=CARTESIAN_POINT ( 'NONE',  ( 197.3953739035038950, 96.83737926879658175, 92.16504039591205810 ) ) ;
#10530=ORIENTED_EDGE ( 'NONE', *, *, #63696, .T. ) ;
#10532=DIRECTION ( 'NONE',  ( 0.000000000000000000, 0.000000000000000000, 1.000000000000000000 ) ) ;
#10533=ORIENTED_EDGE ( 'NONE', *, *, #41476, .T. ) ;
#10535=CARTESIAN_POINT ( 'NONE',  ( -24.32471770265757982, 9.546495606312149107, -72.08645900122067474 ) ) ;
#10541=CARTESIAN_POINT ( 'NONE',  ( -148.6426981422628444, 63.44891673852537650, 3.913616068001397164 ) ) ;
#10546=CARTESIAN_POINT ( 'NONE',  ( -128.1267916618074878, 49.19573276651589566, 45.29461237954313191 ) ) ;
#10547=ORIENTED_EDGE ( 'NONE', *, *, #39694, .F. ) ;
#10549=CARTESIAN_POINT ( 'NONE',  ( -147.7925265216585444, 64.04960911618974251, 30.91620572533726374 ) ) ;
#10551=CARTESIAN_POINT ( 'NONE',  ( 181.0840389613909736, -170.0000000000000000, 71.15314469597512925 ) ) ;
#10564=CARTESIAN_POINT ( 'NONE',  ( 32.89501968360929851, 8.663558833820815153, -66.20267533015858419 ) ) ;
#10565=CARTESIAN_POINT ( 'NONE',  ( 140.1999945597798671, 45.38880890490931108, -74.37758294665758285 ) ) ;
#10566=CARTESIAN_POINT ( 'NONE',  ( 70.50372867914784081, 14.53505678900967268, 37.80345282212471858 ) ) ;
#10567=CARTESIAN_POINT ( 'NONE',  ( 8.289642123990038414, 7.382587591294829998, 91.56333915467209295 ) ) ;
#10568=ORIENTED_EDGE ( 'NONE', *, *, #63330, .F. ) ;
#10572=CARTESIAN_POINT ( 'NONE',  ( -73.10694748374054086, 20.28107308417882848, 32.86053516446196454 ) ) ;
#10576=CARTESIAN_POINT ( 'NONE',  ( -180.4643341113398094, 95.69224917234933514, 66.72163245273618770 ) ) ;
#10577=CARTESIAN_POINT ( 'NONE',  ( 127.2202105166096118, 37.55913282978153944, 60.35159291791857328 ) ) ;
#10579=CARTESIAN_POINT ( 'NONE',  ( 150.2809931605061990, 52.27058242113233888, 34.75635080141699262 ) ) ;
#10580=AXIS2_PLACEMENT_3D ( 'NONE', #59794, #33783, #32733 ) ;
#10583=CARTESIAN_POINT ( 'NONE',  ( -190.6985136298601731, 109.1272424661242582, -95.00000000000133582 ) ) ;
#10584=CARTESIAN_POINT ( 'NONE',  ( 137.5911612413395630, 44.91497189902067078, -63.85950958629689467 ) ) ;
#10585=CARTESIAN_POINT ( 'NONE',  ( -148.6426892915312408, 64.76241938621078020, -61.65738112195565890 ) ) ;
#10586=VERTEX_POINT ( 'NONE', #46860 ) ;
#10588=CARTESIAN_POINT ( 'NONE',  ( 8.000000000000007105, 249.8719672152120381, 0.000000000000000000 ) ) ;
#10590=CARTESIAN_POINT ( 'NONE',  ( -180.5801285865471755, 97.42945596116099694, 64.36713565232477663 ) ) ;
#10591=CARTESIAN_POINT ( 'NONE',  ( 114.9635499210459670, 31.12758084072142140, -91.26968024238497890 ) ) ;
#10594=CARTESIAN_POINT ( 'NONE',  ( -84.21836162213170951, 25.60181819557224259, 6.007885502826089130 ) ) ;
#10598=CARTESIAN_POINT ( 'NONE',  ( 197.1966017667921278, 98.19524189129653280, 90.58426338797916344 ) ) ;
#10601=CARTESIAN_POINT ( 'NONE',  ( -80.56139928459658961, 24.13290941644245535, 72.02333951919742105 ) ) ;
#10602=CARTESIAN_POINT ( 'NONE',  ( 43.33582519206056816, 9.970536411945046140, -90.41014636795507897 ) ) ;
#10603=VERTEX_POINT ( 'NONE', #39 ) ;
#10604=CARTESIAN_POINT ( 'NONE',  ( -37.37206033059240440, 11.66494618096612612, 6.277285149997919866 ) ) ;
#10608=ORIENTED_EDGE ( 'NONE', *, *, #53288, .T. ) ;
#10611=CARTESIAN_POINT ( 'NONE',  ( -144.2038301586456157, 61.09856042007388055, 59.74016205658093526 ) ) ;
#10612=DIRECTION ( 'NONE',  ( -0.8160245890732938934, -0.5780171883497599028, 0.000000000000000000 ) ) ;
#10613=CARTESIAN_POINT ( 'NONE',  ( 138.2136629441928619, 45.30947856186674727, -49.64627368863411050 ) ) ;
#10614=CARTESIAN_POINT ( 'NONE',  ( 211.6758053788387883, 118.2764674294293457, -94.75375889897657089 ) ) ;
#10616=FACE_OUTER_BOUND ( 'NONE', #7524, .T. ) ;
#10623=CARTESIAN_POINT ( 'NONE',  ( -169.1116812882276292, 84.24296059722695418, -9.013269524975111580 ) ) ;
#10628=CARTESIAN_POINT ( 'NONE',  ( -12.78015296493257225, 7.264294661536299991, 70.11165917322330188 ) ) ;
#10631=CARTESIAN_POINT ( 'NONE',  ( 43.14356474118745410, 8.925336319666904217, -22.79396403428114937 ) ) ;
#10634=CARTESIAN_POINT ( 'NONE',  ( 164.8433205901839074, 64.93586312665797777, 65.15668412550157029 ) ) ;
#10635=AXIS2_PLACEMENT_3D ( 'NONE', #54358, #22721, #27642 ) ;
#10638=CARTESIAN_POINT ( 'NONE',  ( 129.4887940973039804, 40.01039828304094215, 16.28148538411281976 ) ) ;
#10641=CARTESIAN_POINT ( 'NONE',  ( 152.2924710224605462, 54.98503313872889464, 69.18529703667503838 ) ) ;
#10642=CYLINDRICAL_SURFACE ( 'NONE', #28750, 7.500000000000020428 ) ;
#10643=FACE_OUTER_BOUND ( 'NONE', #42422, .T. ) ;
#10646=CARTESIAN_POINT ( 'NONE',  ( -14.35185884954381308, 8.414771159230838293, 94.99999999999866418 ) ) ;
#10653=VERTEX_POINT ( 'NONE', #37676 ) ;
#10655=CARTESIAN_POINT ( 'NONE',  ( 46.81205265836391050, 10.50862573052651072, 89.89773165160593749 ) ) ;
#10657=CARTESIAN_POINT ( 'NONE',  ( 141.0229350107040887, 47.12561858623062960, -95.00000000000133582 ) ) ;
#10658=VERTEX_POINT ( 'NONE', #49261 ) ;
#10659=CARTESIAN_POINT ( 'NONE',  ( -56.97107423601133291, 15.20373812575555306, -76.82745312835619700 ) ) ;
#10660=CARTESIAN_POINT ( 'NONE',  ( 31.90217595456442012, 7.552213897210509508, -15.78119844062844734 ) ) ;
#10661=CARTESIAN_POINT ( 'NONE',  ( 173.7263186949343776, 72.85225335320951956, -45.20748257772405765 ) ) ;
#10663=CARTESIAN_POINT ( 'NONE',  ( 87.58098510096635891, 19.74745174099416900, 29.75724612964751259 ) ) ;
#10665=CARTESIAN_POINT ( 'NONE',  ( -54.56685407443680447, 15.59259313022788085, -35.21632399845987038 ) ) ;
#10667=CARTESIAN_POINT ( 'NONE',  ( 12.91653430408660697, 7.431946598423015971, 30.57340478084518764 ) ) ;
#10668=CARTESIAN_POINT ( 'NONE',  ( 68.78485849535977081, 14.08475838183477080, -92.04534818299838150 ) ) ;
#10669=B_SPLINE_CURVE_WITH_KNOTS ( 'NONE', 3,
 ( #61756, #3035, #40311, #30115, #52248, #46622, #8309, #56484, #29758, #35042, #30449, #24498, #18863, #45935, #47908, #57533, #42639, #4069, #2680, #9337, #51220, #64095, #9003, #19191, #40650, #62106, #8660, #69372, #67068, #15910, #13580, #30800, #13922, #29413, #35386, #56844, #26470, #37350, #35738, #46270, #51566, #41008, #58808 ),
 .UNSPECIFIED., .F., .F.,
 ( 4, 2, 2, 2, 2, 2, 2, 2, 2, 2, 2, 2, 1, 2, 2, 2, 2, 2, 2, 2, 2, 4 ),
 ( 0.02371951416048008465, 0.02520633211177543062, 0.02594974108742308105, 0.02669315006307073496, 0.02817996801436603582, 0.02966678596566133322, 0.03041019494130899059, 0.03115360391695664796, 0.03264042186825195924, 0.03412723981954727398, 0.03561405777084258872, 0.03635746674649023569, 0.03710087572213788265, 0.03784428469778552961, 0.03858769367343317658, 0.04007451162472847050, 0.04156132957602376443, 0.04304814752731905836, 0.04379155650296670532, 0.04453496547861433841, 0.04602178342990957682, 0.04750860138120482218 ),
 .UNSPECIFIED. ) ;
#10670=CARTESIAN_POINT ( 'NONE',  ( -85.97950457423550574, 26.33440868064809237, 89.91133426644037741 ) ) ;
#10677=EDGE_CURVE ( 'NONE', #31197, #19164, #49944, .T. ) ;
#10680=CARTESIAN_POINT ( 'NONE',  ( -13.29455179262033226, 8.319166883236663423, -21.21143003818049166 ) ) ;
#10684=ORIENTED_EDGE ( 'NONE', *, *, #33364, .T. ) ;
#10686=CARTESIAN_POINT ( 'NONE',  ( -156.8764584803561206, 70.69066846313522490, -43.73679383676832799 ) ) ;
#10691=CARTESIAN_POINT ( 'NONE',  ( -85.73740570227384694, 26.23277384689413694, -45.12853643150059924 ) ) ;
#10692=CARTESIAN_POINT ( 'NONE',  ( 117.6855018526752161, 32.47998843907879518, 91.79128257728453377 ) ) ;
#10693=CARTESIAN_POINT ( 'NONE',  ( -156.3734885497381413, 71.59531449004289527, 8.346329245734816382 ) ) ;
#10695=VECTOR ( 'NONE', #21629, 1000.000000000000000 ) ;
#10697=CARTESIAN_POINT ( 'NONE',  ( 22.81270948571149404, 6.827178363529885274, 40.15439324559184087 ) ) ;
#10701=ORIENTED_EDGE ( 'NONE', *, *, #47877, .F. ) ;
#10702=AXIS2_PLACEMENT_3D ( 'NONE', #66076, #29117, #44594 ) ;
#10706=CARTESIAN_POINT ( 'NONE',  ( 36.08914434112044489, 9.014684630517859176, -36.38665694955406593 ) ) ;
#10710=CARTESIAN_POINT ( 'NONE',  ( 198.2588776805010866, 99.52972231602377917, 59.69594739211307655 ) ) ;
#10713=CARTESIAN_POINT ( 'NONE',  ( -149.5074843970971017, 64.17983161892348676, 57.56537183036274996 ) ) ;
#10714=CARTESIAN_POINT ( 'NONE',  ( 23.09590709048885060, 7.852755081912512480, 12.37589148572721953 ) ) ;
#10717=CARTESIAN_POINT ( 'NONE',  ( -82.93267503967652488, 23.99263498936122474, -36.44237337058958559 ) ) ;
#10718=CARTESIAN_POINT ( 'NONE',  ( 23.24028701062093560, 6.853614888934260740, 65.33720227182544704 ) ) ;
#10720=CARTESIAN_POINT ( 'NONE',  ( 10.13405324523498585, 6.385324379632245417, -74.81575908290277255 ) ) ;
#10721=B_SPLINE_CURVE_WITH_KNOTS ( 'NONE', 3,
 ( #61167, #31160, #40059, #46974, #23543, #60807, #4411, #55531, #56229, #8045, #12634, #29496, #12991, #61515, #7364, #44981, #25874, #41361, #29158, #39712, #50608, #23883, #13334, #2772, #45685, #67162, #62815, #14618, #52252, #25537, #37105, #5776, #16683, #63848, #11393, #43407, #5440, #53264, #26555, #59240, #15991, #154, #59577, #32868 ),
 .UNSPECIFIED., .F., .F.,
 ( 4, 2, 2, 2, 2, 2, 2, 2, 2, 2, 2, 2, 2, 2, 2, 2, 2, 2, 2, 2, 2, 4 ),
 ( 1.398578778534940505E-17, 0.003433139681083792211, 0.004291424601354686813, 0.005149709521625580981, 0.006866279362167290387, 0.007724564282438155065, 0.008582849202709021477, 0.009441134122979885288, 0.01029941904325075083, 0.01201598888379252529, 0.01373255872433429801, 0.01459084364460517917, 0.01544912856487606553, 0.01630741348514694669, 0.01716569840541783132, 0.01888226824595960751, 0.02059883808650138370, 0.02145712300677229956, 0.02231540792704321888, 0.02403197776758502283, 0.02574854760812682677, 0.02746511744866863072 ),
 .UNSPECIFIED. ) ;
#10726=CARTESIAN_POINT ( 'NONE',  ( 175.8963338753314360, 73.51705463274397800, 42.23070144013426130 ) ) ;
#10727=CARTESIAN_POINT ( 'NONE',  ( -130.2196570250629293, 49.40815211106347959, -48.55858868297418240 ) ) ;
#10729=CARTESIAN_POINT ( 'NONE',  ( -104.5916564445180796, 35.10571011602409186, -35.36428607247657396 ) ) ;
#10730=ADVANCED_FACE ( 'NONE', ( #60176 ), #22897, .F. ) ;
#10731=CARTESIAN_POINT ( 'NONE',  ( 55.52751777340356654, 12.08567914268658683, -69.57556231829563842 ) ) ;
#10734=ORIENTED_EDGE ( 'NONE', *, *, #22542, .F. ) ;
#10736=CARTESIAN_POINT ( 'NONE',  ( -24.19091603582231897, 8.513464105188678133, -14.02971085878847823 ) ) ;
#10737=CARTESIAN_POINT ( 'NONE',  ( 175.0836463967652605, 72.74684624755143147, 85.98398430601433517 ) ) ;
#10741=CARTESIAN_POINT ( 'NONE',  ( 110.7114632166111790, 29.09878355652112703, 56.45576479620100940 ) ) ;
#10744=CARTESIAN_POINT ( 'NONE',  ( 129.1137093889808511, 38.63348691920622713, 31.19545504990886897 ) ) ;
#10746=CARTESIAN_POINT ( 'NONE',  ( 140.0820590176526537, 46.51134312115247837, 59.66472826312686095 ) ) ;
#10748=CARTESIAN_POINT ( 'NONE',  ( 81.52811112547603045, 17.74308114851538676, -91.50889126552081621 ) ) ;
#10750=LINE ( 'NONE', #21306, #5780 ) ;
#10756=CARTESIAN_POINT ( 'NONE',  ( -166.3205068063722081, 81.30869308872871670, 8.302501522647505183 ) ) ;
#10759=CARTESIAN_POINT ( 'NONE',  ( -174.7800083645696532, 88.99302808536933185, -22.69361122552189869 ) ) ;
#10760=CARTESIAN_POINT ( 'NONE',  ( -190.6985136298601731, 109.1272424661242582, 94.99999999999866418 ) ) ;
#10761=CARTESIAN_POINT ( 'NONE',  ( -149.5074843970971301, 64.17983161892345834, -49.81283053149198992 ) ) ;
#10762=ORIENTED_EDGE ( 'NONE', *, *, #45896, .F. ) ;
#10764=ORIENTED_EDGE ( 'NONE', *, *, #62967, .T. ) ;
#10765=CARTESIAN_POINT ( 'NONE',  ( -126.3508039230933377, 46.79479538767116509, 45.61994787315712330 ) ) ;
#10767=CARTESIAN_POINT ( 'NONE',  ( 86.14852828165528820, 19.25704475759651402, -8.977013608448029203 ) ) ;
#10771=CARTESIAN_POINT ( 'NONE',  ( -95.19652294162975181, 29.32558722310178823, 13.69184615439291619 ) ) ;
#10772=CARTESIAN_POINT ( 'NONE',  ( -152.6866856590304735, 66.92104572559831865, -89.15920658215685535 ) ) ;
#10775=CARTESIAN_POINT ( 'NONE',  ( 186.6054783416232112, 84.37128553200975034, -75.67012523732033458 ) ) ;
#10777=CARTESIAN_POINT ( 'NONE',  ( -165.9986675144416211, 79.53506019208359135, -39.84463087508462564 ) ) ;
#10779=CARTESIAN_POINT ( 'NONE',  ( 106.4072861358878299, 28.24787347451998798, -63.81749795290593852 ) ) ;
#10780=CARTESIAN_POINT ( 'NONE',  ( -75.00636493611888511, 22.03142602679957207, -62.89598738381337029 ) ) ;
#10782=CARTESIAN_POINT ( 'NONE',  ( 46.65860211212413589, 10.48377752989034128, -41.16074490250159812 ) ) ;
#10783=CARTESIAN_POINT ( 'NONE',  ( 211.7451286015360949, 116.5372661580811666, 66.13550906399829898 ) ) ;
#10786=CARTESIAN_POINT ( 'NONE',  ( -108.9136445001390001, 36.28030794288192595, -12.16150055407688058 ) ) ;
#10787=EDGE_LOOP ( 'NONE', ( #50395, #54175, #55009, #26614 ) ) ;
#10791=CARTESIAN_POINT ( 'NONE',  ( -85.00384554948603011, 24.83757696374530965, -92.28742627645222285 ) ) ;
#10792=B_SPLINE_CURVE_WITH_KNOTS ( 'NONE', 3,
 ( #8664, #63159, #41697, #67751, #36078, #10032, #9694, #9007, #14955, #52251, #68431, #47645, #19195, #36420, #31159, #35389, #31487, #3713, #30453, #40656, #57537, #46625, #4409, #56847, #24833, #41011, #52590, #62109, #4073, #30120, #62465, #68100, #19904, #14281, #58216, #25873, #47301, #35741, #41360, #15311, #13926, #62813, #57192 ),
 .UNSPECIFIED., .F., .F.,
 ( 4, 2, 2, 2, 2, 2, 2, 2, 2, 2, 2, 2, 1, 2, 2, 2, 2, 2, 2, 2, 2, 4 ),
 ( 0.02358007599568757648, 0.02505677178601659061, 0.02579511968118109247, 0.02653346757634559433, 0.02801016336667459805, 0.02948685915700360524, 0.03022520705216810710, 0.03096355494733261243, 0.03244025073766165779, 0.03391694652799069620, 0.03539364231831973462, 0.03613199021348427464, 0.03687033810864881467, 0.03760868600381335469, 0.03834703389897789472, 0.03982372968930697477, 0.04130042547963604788, 0.04277712126996512099, 0.04351546916512966101, 0.04425381706029420104, 0.04573051285062328802, 0.04720720864095238195 ),
 .UNSPECIFIED. ) ;
#10793=CARTESIAN_POINT ( 'NONE',  ( 112.1100957124161539, 30.86846953551571104, 2.987587920464681357 ) ) ;
#10794=CARTESIAN_POINT ( 'NONE',  ( -78.66644367742109978, 23.39876645725288640, -23.27090004125422595 ) ) ;
#10795=EDGE_CURVE ( 'NONE', #68783, #31812, #35640, .T. ) ;
#10796=AXIS2_PLACEMENT_3D ( 'NONE', #44896, #56485, #29414 ) ;
#10797=CARTESIAN_POINT ( 'NONE',  ( -101.3537077702550562, 33.43904726487055967, -61.90219306547648159 ) ) ;
#10798=CARTESIAN_POINT ( 'NONE',  ( -101.8140949286062238, 33.67224128592401655, -8.170026674512227416 ) ) ;
#10799=AXIS2_PLACEMENT_3D ( 'NONE', #2708, #31508, #9028 ) ;
#10802=CARTESIAN_POINT ( 'NONE',  ( 211.9471657255442949, 116.8466227750260344, 92.33050231943069264 ) ) ;
#10807=CARTESIAN_POINT ( 'NONE',  ( 8.683910719548892487, 7.383368463746304400, -72.27984568902408569 ) ) ;
#10809=CARTESIAN_POINT ( 'NONE',  ( 46.85361596800670725, 10.51535167202354515, -68.97966382706947286 ) ) ;
#10813=CARTESIAN_POINT ( 'NONE',  ( 79.97476514061575870, 18.30994623469640104, 94.42742991237855676 ) ) ;
#10818=CARTESIAN_POINT ( 'NONE',  ( -131.7724154034330297, 50.48821165954358037, 15.93959937002138716 ) ) ;
#10819=CARTESIAN_POINT ( 'NONE',  ( -107.7886332494339570, 36.81249801143972888, 69.97670749553998348 ) ) ;
#10820=CARTESIAN_POINT ( 'NONE',  ( -180.6010819689385301, 95.85959870121170923, 91.43127333083813824 ) ) ;
#10823=CARTESIAN_POINT ( 'NONE',  ( -6.126800896373028493, 6.786243985899684361, -23.38278218708607525 ) ) ;
#10825=B_SPLINE_CURVE_WITH_KNOTS ( 'NONE', 3,
 ( #48413, #601, #22056, #245, #64977, #43153, #16437, #32957, #38231, #49114, #59673, #22406, #54752, #43845, #1302, #22754, #34714, #12914, #44192, #61087, #12207, #8323, #34370, #50534, #7969, #23806, #13255, #2013, #28734, #61436, #17468, #50874, #7281, #23108, #66040, #28375, #55100, #66729, #17833, #39290, #66390, #38949, #6926, #49822, #55816 ),
 .UNSPECIFIED., .F., .F.,
 ( 4, 2, 2, 1, 2, 2, 2, 2, 2, 2, 2, 2, 2, 2, 2, 2, 2, 2, 2, 2, 2, 2, 4 ),
 ( 0.02346464386237014782, 0.02493212228186625704, 0.02566586149161431685, 0.02639960070136237319, 0.02713333991111042953, 0.02786707912085848587, 0.02933455754035460203, 0.03006829675010265837, 0.03080203595985071124, 0.03226951437934682393, 0.03300325358909487333, 0.03373699279884292968, 0.03520447121833904236, 0.03667194963783515504, 0.03740568884758320445, 0.03813942805733125385, 0.03960690647682736654, 0.04107438489632347228, 0.04254186331581957803, 0.04327560252556764131, 0.04400934173531569071, 0.04547682015481180340, 0.04694429857430792302 ),
 .UNSPECIFIED. ) ;
#10826=CARTESIAN_POINT ( 'NONE',  ( 197.5344433744249386, 98.61756151884681287, -14.73665922601220757 ) ) ;
#10827=CARTESIAN_POINT ( 'NONE',  ( -155.6121305361943143, 69.53530207094544835, 87.54207503471559448 ) ) ;
#10828=CARTESIAN_POINT ( 'NONE',  ( 141.3707934840545022, 46.15056991286790122, 36.98067333115320565 ) ) ;
#10831=CARTESIAN_POINT ( 'NONE',  ( 79.19119222799092483, 18.06817527909834098, 11.36162365658382356 ) ) ;
#10832=CARTESIAN_POINT ( 'NONE',  ( 161.7006237583813402, 62.31514460450498660, 3.854726898469810425 ) ) ;
#10837=AXIS2_PLACEMENT_3D ( 'NONE', #5248, #302, #48818 ) ;
#10838=CARTESIAN_POINT ( 'NONE',  ( -75.43953471071002070, 21.11829282998124668, -22.55799270516261146 ) ) ;
#10839=CARTESIAN_POINT ( 'NONE',  ( 69.73342236697681074, 14.33173522011653311, -73.43652197196315967 ) ) ;
#10840=CARTESIAN_POINT ( 'NONE',  ( -61.86403937395564157, 16.61416349803656090, 40.96657735976691583 ) ) ;
#10842=CARTESIAN_POINT ( 'NONE',  ( 149.9683128897950155, 53.28564708287390772, 10.59517325904875662 ) ) ;
#10844=CARTESIAN_POINT ( 'NONE',  ( 159.6593397521790791, 59.37286298965128850, 29.72214504742798624 ) ) ;
#10848=ORIENTED_EDGE ( 'NONE', *, *, #20333, .T. ) ;
#10855=CARTESIAN_POINT ( 'NONE',  ( -180.0094637318086370, 96.72611451757710199, 35.34088033557112851 ) ) ;
#10856=CARTESIAN_POINT ( 'NONE',  ( 126.6266894765173419, 38.37986986668738609, 65.91793733211123651 ) ) ;
#10857=ORIENTED_EDGE ( 'NONE', *, *, #13025, .T. ) ;
#10858=ORIENTED_EDGE ( 'NONE', *, *, #7947, .F. ) ;
#10861=CARTESIAN_POINT ( 'NONE',  ( -102.7447593990059289, 34.14748189312170723, 3.674523915951409148 ) ) ;
#10866=CARTESIAN_POINT ( 'NONE',  ( -132.9109786433856186, 51.29129389542018203, 67.62515982255897029 ) ) ;
#10868=ORIENTED_EDGE ( 'NONE', *, *, #51245, .F. ) ;
#10873=CARTESIAN_POINT ( 'NONE',  ( 206.3125232506203872, 108.5822159704962075, -63.33511981463161078 ) ) ;
#10875=EDGE_CURVE ( 'NONE', #27866, #57040, #6500, .T. ) ;
#10877=CARTESIAN_POINT ( 'NONE',  ( -37.36232632813460697, 10.63891575123902200, -91.90072181533541595 ) ) ;
#10878=CARTESIAN_POINT ( 'NONE',  ( 22.90619343622340054, 7.840927939412484449, 35.10082476785152039 ) ) ;
#10879=CARTESIAN_POINT ( 'NONE',  ( 198.3689982626052313, 98.05019997562733636, 86.36795352984687213 ) ) ;
#10880=CARTESIAN_POINT ( 'NONE',  ( -125.8938041572051105, 46.49392987655492959, -76.75825448869764500 ) ) ;
#10881=B_SPLINE_CURVE_WITH_KNOTS ( 'NONE', 3,
 ( #3888, #30974, #26035, #8480, #14780, #3208, #24662, #36244, #52420, #47130, #68594, #21106, #63670, #33034, #53432, #65045, #42548, #36935, #54109, #32348, #64004, #32001, #59743, #31647, #16505, #10878, #318, #37608, #11557, #59062, #5261, #16155, #68926, #27747, #15815, #37258, #16843, #22127, #53774, #26381, #48483, #58372, #10527 ),
 .UNSPECIFIED., .F., .F.,
 ( 4, 2, 2, 2, 2, 2, 2, 2, 1, 2, 2, 2, 2, 2, 2, 2, 2, 2, 2, 2, 2, 4 ),
 ( 0.000000000000000000, 0.001466285743483475203, 0.002199428615225213022, 0.002932571486966950407, 0.004398857230450435585, 0.005865142973933920763, 0.007331428717417405073, 0.008064571589159148096, 0.008797714460900890251, 0.009530857332642634142, 0.01026400020438437630, 0.01173028594786783806, 0.01319657169135130155, 0.01466285743483476331, 0.01539600030657650546, 0.01612914317831825109, 0.01759542892180173193, 0.01906171466528521971, 0.01979485753702697054, 0.02052800040876871790, 0.02199428615225220915, 0.02346057189573570387 ),
 .UNSPECIFIED. ) ;
#10882=ORIENTED_EDGE ( 'NONE', *, *, #14912, .T. ) ;
#10887=CARTESIAN_POINT ( 'NONE',  ( -26.88234027341226096, 9.904106450608207268, -75.63871759701287090 ) ) ;
#10888=CARTESIAN_POINT ( 'NONE',  ( 55.57657751403269941, 11.06944050856661832, -44.20687798256333423 ) ) ;
#10894=CARTESIAN_POINT ( 'NONE',  ( -130.5904357464317798, 50.88938808445630713, 43.98754880289844493 ) ) ;
#10896=ORIENTED_EDGE ( 'NONE', *, *, #63842, .F. ) ;
#10899=CARTESIAN_POINT ( 'NONE',  ( 62.04326772936976653, 12.44884401098615534, 56.70505522888109340 ) ) ;
#10904=ORIENTED_EDGE ( 'NONE', *, *, #42697, .F. ) ;
#10907=PLANE ( 'NONE',  #36177 ) ;
#10909=CARTESIAN_POINT ( 'NONE',  ( 181.0840389613909736, -170.0000000000000000, 36.80859410551140343 ) ) ;
#10910=CARTESIAN_POINT ( 'NONE',  ( 70.02892116572940040, 14.40944430928137088, 39.98237600456136676 ) ) ;
#10911=CARTESIAN_POINT ( 'NONE',  ( 9.628853386404982118, 7.387802178417762100, 86.91185589324661009 ) ) ;
#10913=CARTESIAN_POINT ( 'NONE',  ( 79.53408731553408018, 17.12082763744059832, 12.84865754040789732 ) ) ;
#10914=EDGE_LOOP ( 'NONE', ( #57946, #30950 ) ) ;
#10915=DIRECTION ( 'NONE',  ( -0.000000000000000000, 1.000000000000000000, -0.000000000000000000 ) ) ;
#10919=CARTESIAN_POINT ( 'NONE',  ( -118.3948752128398496, 42.92869324237092599, 11.57276413738803456 ) ) ;
#10922=CARTESIAN_POINT ( 'NONE',  ( 131.6189313563687620, 40.08924984825279125, 71.02825006529253926 ) ) ;
#10923=ORIENTED_EDGE ( 'NONE', *, *, #14255, .T. ) ;
#10928=CARTESIAN_POINT ( 'NONE',  ( 150.4550062612852628, 52.39582885725848627, 39.61425003142517198 ) ) ;
#10929=CARTESIAN_POINT ( 'NONE',  ( 69.72789637502502558, 15.37065610545704253, 33.95776896090188757 ) ) ;
#10936=CARTESIAN_POINT ( 'NONE',  ( -143.8756912989387047, 60.83492035645716811, -64.19810953127340269 ) ) ;
#10941=CARTESIAN_POINT ( 'NONE',  ( -7.825402957745083654, 6.891034867348166948, -77.26262132240753999 ) ) ;
#10942=CARTESIAN_POINT ( 'NONE',  ( -175.1895962157337010, 90.99110972060685754, 57.94477835241939090 ) ) ;
#10944=CARTESIAN_POINT ( 'NONE',  ( -118.8691191306315034, 43.21907118237573542, -39.77302265458806119 ) ) ;
#10945=CARTESIAN_POINT ( 'NONE',  ( -86.16710354151693707, 26.41338104675948628, 11.30814425100590981 ) ) ;
#10948=B_SPLINE_CURVE_WITH_KNOTS ( 'NONE', 3,
 ( #36946, #64018, #10541, #37623, #15147, #53785, #32017, #63683, #68938, #64354, #47143, #68606, #58056, #53445, #14793, #16168, #41879, #9876, #27064, #333, #4583, #21787, #36257, #57713, #9527, #26051, #13256, #60119, #61437, #7637, #29088, #13593, #66731, #18527, #61767, #34715, #11939, #43236, #33411, #11231, #38674, #55817, #50535, #7970, #23807, #56153, #1042, #27765 ),
 .UNSPECIFIED., .F., .F.,
 ( 4, 2, 2, 2, 2, 2, 2, 2, 2, 2, 2, 2, 2, 2, 2, 2, 2, 2, 2, 2, 2, 2, 2, 4 ),
 ( 0.02746511744866864113, 0.02914922134997090242, 0.03083332525127316370, 0.03251742915257542499, 0.03335948110322658339, 0.03420153305387774179, 0.03504358500452890712, 0.03588563695518006552, 0.03756974085648233375, 0.03841179280713347827, 0.03925384475778461585, 0.04009589670843575343, 0.04093794865908689795, 0.04262205256038916618, 0.04430615646169144134, 0.04514820841234259974, 0.04599026036299375120, 0.04767436426429605412, 0.04935846816559835704, 0.05020052011624950850, 0.05104257206690067383, 0.05272667596820304614, 0.05356872791885423923, 0.05441077986950544620 ),
 .UNSPECIFIED. ) ;
#10950=CARTESIAN_POINT ( 'NONE',  ( -71.79801807585624829, 19.82313861722078485, -93.28382037184846354 ) ) ;
#10951=CARTESIAN_POINT ( 'NONE',  ( 70.46452034227871764, 14.52462608639675601, 9.463287704965392066 ) ) ;
#10953=CARTESIAN_POINT ( 'NONE',  ( 42.60735219095521131, 9.864569470531383999, -90.02523864352265548 ) ) ;
#10956=CARTESIAN_POINT ( 'NONE',  ( -35.38962320578855980, 11.29584325137388134, 17.25183784669100362 ) ) ;
#10957=ORIENTED_EDGE ( 'NONE', *, *, #33293, .F. ) ;
#10961=CARTESIAN_POINT ( 'NONE',  ( 20.74561700410410836, 7.717362891868937425, -64.21423502926538163 ) ) ;
#10962=CARTESIAN_POINT ( 'NONE',  ( 117.1441767749777227, 33.33376675874068695, 93.81895193412631784 ) ) ;
#10967=B_SPLINE_CURVE_WITH_KNOTS ( 'NONE', 3,
 ( #18782, #12823, #7547, #29680, #13846, #55011, #49728, #29007, #28286, #41277, #4666, #68687, #19825, #19468, #26132, #30726, #14201, #68361, #47229, #14877, #62738, #35659, #63425, #69023, #8927, #57452, #42310, #20850, #52173, #3993, #30033, #9961, #3299, #63771, #35308, #68020, #20499, #46193, #25460, #14542, #36002, #52844, #41964, #47567 ),
 .UNSPECIFIED., .F., .F.,
 ( 4, 2, 2, 2, 2, 2, 2, 2, 2, 2, 2, 2, 2, 2, 2, 2, 2, 2, 2, 2, 2, 4 ),
 ( 0.000000000000000000, 0.003518733725596323494, 0.004398417156995387996, 0.005278100588394452931, 0.007037467451192651324, 0.007917150882591747485, 0.008796834313990845380, 0.01055620117678908107, 0.01231556803958732023, 0.01319525147098642159, 0.01407493490238551775, 0.01495461833378461738, 0.01583430176518371701, 0.01671398519658281664, 0.01759366862798191627, 0.01935303549078009819, 0.02111240235357827663, 0.02199208578497733116, 0.02287176921637638222, 0.02463113607917447739, 0.02639050294197257604, 0.02814986980477066775 ),
 .UNSPECIFIED. ) ;
#10969=CARTESIAN_POINT ( 'NONE',  ( -125.8938041572051389, 47.69968343338780414, -8.069153307770243089 ) ) ;
#10972=CARTESIAN_POINT ( 'NONE',  ( 34.45972925205163051, 8.830088223935240066, 58.59592793524065257 ) ) ;
#10973=CARTESIAN_POINT ( 'NONE',  ( -166.2053056899074761, 81.18967388993337408, 62.24998455618286641 ) ) ;
#10977=CARTESIAN_POINT ( 'NONE',  ( 93.72059824125561533, 23.03897520779758423, 12.86014247970559410 ) ) ;
#10978=CARTESIAN_POINT ( 'NONE',  ( 188.5838389098762775, 88.03667982118680868, -16.57130179220268573 ) ) ;
#10979=CARTESIAN_POINT ( 'NONE',  ( 212.1976655298229275, 119.0878071902807562, 9.685308493262699159 ) ) ;
#10981=CARTESIAN_POINT ( 'NONE',  ( -84.89017518714956623, 25.87942398301715130, -92.09563210729065474 ) ) ;
#10982=CARTESIAN_POINT ( 'NONE',  ( 46.50704915687941821, 9.440294391580033917, -13.86102426116064557 ) ) ;
#10984=FACE_BOUND ( 'NONE', #48313, .T. ) ;
#10986=B_SPLINE_CURVE_WITH_KNOTS ( 'NONE', 3,
 ( #57170, #8642, #30094, #66698, #51549, #18493, #24814, #61400, #13225, #34687, #46249, #8983, #56122, #63823, #47284, #4724, #5754, #46953, #21588, #48300, #41675, #64511, #26536, #25856, #10686, #15635, #37084, #43038, #52569, #68738, #36749, #47970, #134, #31467, #20554, #5422, #10015, #52903, #31136, #4392, #20218, #32162, #42018, #26190 ),
 .UNSPECIFIED., .F., .F.,
 ( 4, 2, 2, 2, 2, 2, 2, 2, 2, 2, 2, 2, 2, 2, 2, 2, 2, 2, 2, 2, 2, 4 ),
 ( 1.387778780781445676E-17, 0.003433139681083829942, 0.004291424601354737987, 0.005149709521625646033, 0.006866279362167389266, 0.007724564282438267822, 0.008582849202709144643, 0.009441134122980024065, 0.01029941904325090002, 0.01201598888379267101, 0.01373255872433444200, 0.01459084364460533703, 0.01544912856487623380, 0.01630741348514713057, 0.01716569840541802561, 0.01888226824595980180, 0.02059883808650157105, 0.02145712300677249038, 0.02231540792704340623, 0.02403197776758515466, 0.02574854760812689963, 0.02746511744866864460 ),
 .UNSPECIFIED. ) ;
#10990=CARTESIAN_POINT ( 'NONE',  ( -95.54114085644955878, 29.48728305236672398, 94.99999999999866418 ) ) ;
#10992=CARTESIAN_POINT ( 'NONE',  ( -47.94960849910473399, 13.92522873833625852, 67.11944450877264501 ) ) ;
#10999=CARTESIAN_POINT ( 'NONE',  ( 62.52742438962776106, 12.55954017561947822, 17.96841034875761878 ) ) ;
#11000=CARTESIAN_POINT ( 'NONE',  ( -57.42615654242918311, 15.33060010148602537, 71.78055872622512368 ) ) ;
#11001=ORIENTED_EDGE ( 'NONE', *, *, #47714, .F. ) ;
#11004=CARTESIAN_POINT ( 'NONE',  ( 32.66637210955355641, 8.640188015362515017, 94.41850791232543827 ) ) ;
#11005=CARTESIAN_POINT ( 'NONE',  ( 39.40195752203892710, 8.409560354027375340, -77.46436805589148378 ) ) ;
#11006=CARTESIAN_POINT ( 'NONE',  ( 107.9362503323352769, 27.82881837607801856, 44.26364398048654181 ) ) ;
#11007=ORIENTED_EDGE ( 'NONE', *, *, #19603, .F. ) ;
#11008=CARTESIAN_POINT ( 'NONE',  ( -62.30100056228381078, 16.74548393487071607, -67.56937781552855427 ) ) ;
#11009=CARTESIAN_POINT ( 'NONE',  ( 31.91375106836930797, 7.553354707452895944, -16.76326003512198781 ) ) ;
#11010=CARTESIAN_POINT ( 'NONE',  ( -78.66644367742109978, 23.39876645725289706, -88.80455181264524356 ) ) ;
#11011=CARTESIAN_POINT ( 'NONE',  ( 164.8818489117101365, 63.65095510281860669, 89.38953086370848666 ) ) ;
#11012=CARTESIAN_POINT ( 'NONE',  ( 90.30166390191405412, 20.70652093100729019, 30.65456310424210784 ) ) ;
#11013=B_SPLINE_CURVE_WITH_KNOTS ( 'NONE', 3,
 ( #58779, #43640, #20815, #64069, #15881, #5660, #48215, #65118, #32416, #63737, #42944, #26097, #59474, #10594, #48554, #36996, #38030, #64414, #32065, #21169, #54544, #42614, #58436, #10945, #748, #11284, #16223, #38375, #5333, #37678, #389, #21845, #26788, #43290, #11634, #32754, #59124, #64766, #33108, #54185, #6006, #27466, #47526, #48910, #42274, #15545 ),
 .UNSPECIFIED., .F., .F.,
 ( 4, 2, 2, 2, 2, 2, 2, 2, 2, 2, 2, 2, 2, 2, 2, 2, 2, 2, 2, 2, 2, 2, 4 ),
 ( 0.02420077021543441328, 0.02572112563160186202, 0.02648130333968560374, 0.02724148104776934545, 0.02876183646393683582, 0.02952201417202058101, 0.03028219188010432619, 0.03180254729627181309, 0.03332290271243929652, 0.03408308042052303477, 0.03484325812860676608, 0.03636361354477423563, 0.03712379125285796694, 0.03788396896094169825, 0.03864414666902542955, 0.03940432437710916086, 0.04092467979327661654, 0.04244503520944406527, 0.04396539062561151401, 0.04548574604177896274, 0.04624592374986269405, 0.04700610145794641148, 0.04852645687411390879 ),
 .UNSPECIFIED. ) ;
#11017=CARTESIAN_POINT ( 'NONE',  ( 8.000000000000007105, 249.8719672152120381, -95.00000000000133582 ) ) ;
#11018=CARTESIAN_POINT ( 'NONE',  ( 10.82760985890677574, 7.398654328676807168, 43.16107762503957446 ) ) ;
#11019=CARTESIAN_POINT ( 'NONE',  ( 63.82878426028240426, 12.86248996312277804, -89.44302009434157696 ) ) ;
#11021=CARTESIAN_POINT ( 'NONE',  ( -85.63158118751694303, 26.18843205417604025, 94.40781586612253307 ) ) ;
#11025=EDGE_CURVE ( 'NONE', #805, #29948, #22729, .T. ) ;
#11026=ORIENTED_EDGE ( 'NONE', *, *, #27865, .T. ) ;
#11027=CARTESIAN_POINT ( 'NONE',  ( -14.94265033805046095, 7.459411036484907775, -18.48943493301132435 ) ) ;
#11028=CARTESIAN_POINT ( 'NONE',  ( -170.7899427064031386, 86.05659250431358487, 84.87755278391203717 ) ) ;
#11031=CARTESIAN_POINT ( 'NONE',  ( -59.95412189755936794, 17.09836075175412873, -48.41403164313221907 ) ) ;
#11033=CIRCLE ( 'NONE', #35768, 242.4895526022646379 ) ;
#11034=CARTESIAN_POINT ( 'NONE',  ( 153.2282895792480417, 54.42637815496165388, -76.65839619712716058 ) ) ;
#11035=CARTESIAN_POINT ( 'NONE',  ( 18.89064107370902335, 6.619789970027396997, -9.341755237627822339 ) ) ;
#11038=ORIENTED_EDGE ( 'NONE', *, *, #69516, .T. ) ;
#11041=CARTESIAN_POINT ( 'NONE',  ( 68.94948716683070700, 15.16699441119058100, -20.98926308138244679 ) ) ;
#11043=CARTESIAN_POINT ( 'NONE',  ( -152.5101325120252795, 68.10842280990928543, 18.26319916783852904 ) ) ;
#11047=CARTESIAN_POINT ( 'NONE',  ( 187.5325688887159572, 85.37769363979907666, -39.85688821852441777 ) ) ;
#11049=CARTESIAN_POINT ( 'NONE',  ( -153.9360907722259242, 69.37825751209838643, 85.85008364023016725 ) ) ;
#11053=CARTESIAN_POINT ( 'NONE',  ( -151.6797345123119101, 67.37848486615945376, -8.276130779850848995 ) ) ;
#11055=B_SPLINE_CURVE_WITH_KNOTS ( 'NONE', 3,
 ( #20726, #31625, #3180, #30948, #52396, #67544, #19341, #35533, #8805, #43891, #27372, #26696, #16481, #38634, #6267, #15792, #48811, #65374, #63978, #37936, #54441, #59381, #11193, #22453, #5909, #652, #1001, #43545, #21751, #53060, #292, #21080, #49162, #47791, #60076, #37235, #4889, #17160, #48128, #48458, #27029, #42523, #10506, #58686 ),
 .UNSPECIFIED., .F., .F.,
 ( 4, 2, 2, 2, 2, 2, 2, 2, 2, 2, 2, 2, 2, 2, 2, 2, 2, 2, 2, 2, 2, 4 ),
 ( 0.000000000000000000, 0.001476829494128818624, 0.002215244241193236718, 0.002953658988257660233, 0.004430488482386508997, 0.005907317976515357762, 0.007384147470644206526, 0.008122562217708613128, 0.008860976964773019729, 0.01033780645890184161, 0.01181463595303066175, 0.01255305070009507355, 0.01329146544715948536, 0.01476829494128835060, 0.01550670968835276588, 0.01624512443541718462, 0.01772195392954600476, 0.01919878342367482491, 0.01993719817073923845, 0.02067561291780365199, 0.02215244241193248947, 0.02362927190606133043 ),
 .UNSPECIFIED. ) ;
#11056=CARTESIAN_POINT ( 'NONE',  ( -32.41982179707235900, 9.753975577087189208, 57.10945888221309730 ) ) ;
#11057=DIRECTION ( 'NONE',  ( 0.000000000000000000, 0.000000000000000000, 1.000000000000000000 ) ) ;
#11065=CARTESIAN_POINT ( 'NONE',  ( 23.09541709302173018, 6.844586979481589673, 62.65178007441200947 ) ) ;
#11071=LINE ( 'NONE', #53631, #43086 ) ;
#11072=CARTESIAN_POINT ( 'NONE',  ( -126.3458714439411068, 46.79154809309477514, -49.91370389823397602 ) ) ;
#11073=CARTESIAN_POINT ( 'NONE',  ( 41.81982603358024875, 8.735900550613184379, -62.84812721213725695 ) ) ;
#11074=CARTESIAN_POINT ( 'NONE',  ( 56.52885800925554349, 12.28784885070978738, -73.86213855357162572 ) ) ;
#11080=CARTESIAN_POINT ( 'NONE',  ( 197.2847860006354210, 98.30530166401518954, 8.711940037960845373 ) ) ;
#11082=ADVANCED_FACE ( 'NONE', ( #65292 ), #65651, .F. ) ;
#11084=CARTESIAN_POINT ( 'NONE',  ( 181.5079096844946775, 80.47139261082472217, 29.30859410551139277 ) ) ;
#11087=CARTESIAN_POINT ( 'NONE',  ( 115.7612476187724013, 32.64200929566222698, 69.05872566142198821 ) ) ;
#11090=CARTESIAN_POINT ( 'NONE',  ( 139.3041645503688244, 46.00819478311335331, 58.69386422334632414 ) ) ;
#11091=CARTESIAN_POINT ( 'NONE',  ( -74.19961951691013269, 20.67022044985854023, -48.64513555268851519 ) ) ;
#11092=CARTESIAN_POINT ( 'NONE',  ( 161.9809705076523301, 61.24480272096906930, -91.30888859218912046 ) ) ;
#11094=CARTESIAN_POINT ( 'NONE',  ( 92.51858280840787074, 21.51505926344915309, -47.99226530103682364 ) ) ;
#11104=FACE_OUTER_BOUND ( 'NONE', #30669, .T. ) ;
#11105=CARTESIAN_POINT ( 'NONE',  ( -144.7571537022063808, 60.25265659240449878, -48.12163853905629907 ) ) ;
#11107=FACE_OUTER_BOUND ( 'NONE', #9131, .T. ) ;
#11108=ADVANCED_FACE ( 'NONE', ( #66014 ), #39265, .F. ) ;
#11110=CARTESIAN_POINT ( 'NONE',  ( -143.2471548081022945, 59.04577938365766698, 60.90355539476639990 ) ) ;
#11113=CARTESIAN_POINT ( 'NONE',  ( 63.01563776193090405, 13.70579113808098093, -8.876140241706053757 ) ) ;
#11115=CARTESIAN_POINT ( 'NONE',  ( 197.3685896092615906, 96.80423329231983587, 8.239818201410752607 ) ) ;
#11121=CARTESIAN_POINT ( 'NONE',  ( 188.5662303205147055, 86.51341602961784361, -69.97109685562328707 ) ) ;
#11122=FACE_OUTER_BOUND ( 'NONE', #37349, .T. ) ;
#11127=DIRECTION ( 'NONE',  ( 1.000000000000000000, 0.000000000000000000, -0.000000000000000000 ) ) ;
#11128=CARTESIAN_POINT ( 'NONE',  ( -76.33235143960692426, 22.51916353135074544, -62.32845455250863154 ) ) ;
#11129=CARTESIAN_POINT ( 'NONE',  ( 66.94365390260637128, 14.65531706601759865, -49.61441550408923007 ) ) ;
#11130=CARTESIAN_POINT ( 'NONE',  ( -122.3759299995709284, 45.41285412136510757, 31.47923061853353488 ) ) ;
#11133=CARTESIAN_POINT ( 'NONE',  ( -25.07735481787161191, 9.648965052008787069, 6.892143237745487205 ) ) ;
#11135=CARTESIAN_POINT ( 'NONE',  ( -13.78709718204647494, 7.352743657744182926, -47.49489084203693068 ) ) ;
#11137=CARTESIAN_POINT ( 'NONE',  ( -149.5074843970971301, -170.0000000000000000, 30.72082123989904900 ) ) ;
#11138=CARTESIAN_POINT ( 'NONE',  ( 111.1865443042261603, 30.43181341527237649, 2.811416016180984023 ) ) ;
#11141=CARTESIAN_POINT ( 'NONE',  ( -99.10904156412041743, 32.31949011661294691, -62.54589874766276836 ) ) ;
#11144=ORIENTED_EDGE ( 'NONE', *, *, #55497, .F. ) ;
#11145=CARTESIAN_POINT ( 'NONE',  ( 133.8566784816069344, -170.0000000000000000, 10.16579024853168889 ) ) ;
#11148=CARTESIAN_POINT ( 'NONE',  ( 56.52885800925551507, 12.28784885070979449, 60.36061439874682577 ) ) ;
#11150=CARTESIAN_POINT ( 'NONE',  ( -28.13266652174640114, 9.071935854491421480, 17.60819673564329335 ) ) ;
#11152=CARTESIAN_POINT ( 'NONE',  ( -1.876547441458561227, 6.576559737910138814, 33.04152043553114027 ) ) ;
#11153=CARTESIAN_POINT ( 'NONE',  ( -104.5730787903383145, 33.96058035148152499, -62.20252787994973431 ) ) ;
#11154=CARTESIAN_POINT ( 'NONE',  ( 82.33194843254320006, 19.05534674436356113, 84.71864657193529524 ) ) ;
#11159=CARTESIAN_POINT ( 'NONE',  ( -128.9925397612933011, 48.56800623462828526, 4.441519302985077466 ) ) ;
#11160=CARTESIAN_POINT ( 'NONE',  ( -167.4844853368928455, 82.52074065752739784, -47.16599507922662582 ) ) ;
#11162=CARTESIAN_POINT ( 'NONE',  ( -127.6894679065405143, 48.89973668460849865, -35.11786550867761036 ) ) ;
#11166=CARTESIAN_POINT ( 'NONE',  ( 204.6977192012829789, 108.0580384837234931, -9.481380442157895772 ) ) ;
#11172=CARTESIAN_POINT ( 'NONE',  ( 110.2429982417149432, 28.88204397445228722, -62.76698815611734972 ) ) ;
#11173=CARTESIAN_POINT ( 'NONE',  ( 110.2429982417149290, 28.88204397445231209, -50.92243756565370916 ) ) ;
#11178=ORIENTED_EDGE ( 'NONE', *, *, #42162, .F. ) ;
#11179=CARTESIAN_POINT ( 'NONE',  ( -119.3119126656025770, 42.31023367294505988, -92.49952378818520060 ) ) ;
#11184=ORIENTED_EDGE ( 'NONE', *, *, #19229, .T. ) ;
#11185=CARTESIAN_POINT ( 'NONE',  ( 164.3702714028688092, 63.22112480708617710, 39.86111796590435574 ) ) ;
#11186=DIRECTION ( 'NONE',  ( -0.000000000000000000, 1.000000000000000000, -0.000000000000000000 ) ) ;
#11188=CARTESIAN_POINT ( 'NONE',  ( -77.71801202538874520, 23.03755222122951096, -35.16063552580117602 ) ) ;
#11189=ORIENTED_EDGE ( 'NONE', *, *, #33754, .F. ) ;
#11193=CARTESIAN_POINT ( 'NONE',  ( -38.92726670956011503, 10.94099576009806007, -70.15049777360351868 ) ) ;
#11196=EDGE_LOOP ( 'NONE', ( #8971, #27558 ) ) ;
#11198=CARTESIAN_POINT ( 'NONE',  ( -190.6985136298601731, 109.1272424661242582, 94.99999999999866418 ) ) ;
#11200=CARTESIAN_POINT ( 'NONE',  ( -48.41612563322100016, 13.00196567016870297, 94.99999999999866418 ) ) ;
#11202=CARTESIAN_POINT ( 'NONE',  ( -156.7487895666416193, 70.57327586518564999, -71.13043712117229234 ) ) ;
#11203=CARTESIAN_POINT ( 'NONE',  ( 65.61520826398337647, 13.28986957332403840, 83.93644943505340450 ) ) ;
#11206=CARTESIAN_POINT ( 'NONE',  ( 181.0840389613909736, 80.03940679743415387, -89.91415884680696990 ) ) ;
#11210=ORIENTED_EDGE ( 'NONE', *, *, #50771, .F. ) ;
#11213=CARTESIAN_POINT ( 'NONE',  ( 211.7451286015360381, 116.5372661580811240, -68.08724388832010277 ) ) ;
#11215=CARTESIAN_POINT ( 'NONE',  ( -74.19961951691011848, 20.67022044985851181, 5.043965628238842314 ) ) ;
#11218=CARTESIAN_POINT ( 'NONE',  ( 198.5547391818673191, 98.28306391574493261, 94.71473285867655534 ) ) ;
#11220=CARTESIAN_POINT ( 'NONE',  ( 150.4550062612852912, 52.39582885725846495, -40.91940173996584917 ) ) ;
#11221=CARTESIAN_POINT ( 'NONE',  ( 163.2911130186310515, 63.63047778106597718, -65.73252438383109109 ) ) ;
#11224=DIRECTION ( 'NONE',  ( -0.000000000000000000, 1.000000000000000000, -0.000000000000000000 ) ) ;
#11227=CARTESIAN_POINT ( 'NONE',  ( -85.75222301046102302, 25.14826148333820299, 40.42695221713501041 ) ) ;
#11228=CARTESIAN_POINT ( 'NONE',  ( 157.2533363798598600, 58.75760182111574181, -77.96873488960133614 ) ) ;
#11230=CARTESIAN_POINT ( 'NONE',  ( -23.98903001682803193, 8.486614814224621384, 63.56679523331560944 ) ) ;
#11231=CARTESIAN_POINT ( 'NONE',  ( -146.5268141329886760, 61.69196909035593990, 18.26230962334813768 ) ) ;
#11238=CARTESIAN_POINT ( 'NONE',  ( 37.70910994512001224, 9.209110272746709569, -23.58583660981673802 ) ) ;
#11239=CARTESIAN_POINT ( 'NONE',  ( -148.0058283997321666, 64.22864592525515093, 30.86948728267493181 ) ) ;
#11240=CARTESIAN_POINT ( 'NONE',  ( 58.09436971064710775, 11.58462396079456802, 69.83830878865299496 ) ) ;
#11241=CARTESIAN_POINT ( 'NONE',  ( -7.825402957745081878, 7.899365992529270741, 56.96013162991089018 ) ) ;
#11243=CARTESIAN_POINT ( 'NONE',  ( -28.53072891721389581, 10.14951062022288042, -89.57987656953713440 ) ) ;
#11251=DIRECTION ( 'NONE',  ( -0.000000000000000000, 1.000000000000000000, -0.000000000000000000 ) ) ;
#11253=CARTESIAN_POINT ( 'NONE',  ( 65.62848231372478836, 13.29388722724788074, 30.27865613481686680 ) ) ;
#11257=CARTESIAN_POINT ( 'NONE',  ( 81.57482918025355900, 17.75786713398421668, 15.91392937073483260 ) ) ;
#11261=EDGE_CURVE ( 'NONE', #3613, #52201, #17162, .T. ) ;
#11263=ORIENTED_EDGE ( 'NONE', *, *, #41915, .F. ) ;
#11266=CARTESIAN_POINT ( 'NONE',  ( 93.85846834761623825, 22.01563781856521373, 8.354306518833805484 ) ) ;
#11267=DIRECTION ( 'NONE',  ( 0.000000000000000000, 0.000000000000000000, 1.000000000000000000 ) ) ;
#11269=DIRECTION ( 'NONE',  ( 0.000000000000000000, 0.000000000000000000, 1.000000000000000000 ) ) ;
#11271=CARTESIAN_POINT ( 'NONE',  ( 150.4544126017351289, 52.39556706174410294, 34.24499968066869826 ) ) ;
#11272=CARTESIAN_POINT ( 'NONE',  ( -180.4614954900548582, 97.28277348252828460, -43.78069842929563293 ) ) ;
#11277=CARTESIAN_POINT ( 'NONE',  ( 133.8566784816069060, 42.60093787723654657, -62.86786152285933582 ) ) ;
#11280=FACE_BOUND ( 'NONE', #24325, .T. ) ;
#11281=CARTESIAN_POINT ( 'NONE',  ( -3.244108878396728901, 6.635632329121488482, -63.80409075740015368 ) ) ;
#11283=CARTESIAN_POINT ( 'NONE',  ( -122.8202784017355214, 45.69728649588466141, -35.56839789957883369 ) ) ;
#11284=CARTESIAN_POINT ( 'NONE',  ( -86.10360257264198935, 26.38663017581290759, 12.07582342592019309 ) ) ;
#11286=EDGE_CURVE ( 'NONE', #2336, #16002, #3726, .T. ) ;
#11290=CARTESIAN_POINT ( 'NONE',  ( 112.1164716692773595, 29.75790342121401366, 17.54430536651847206 ) ) ;
#11291=CARTESIAN_POINT ( 'NONE',  ( 91.50468583833760761, 22.21368636549395603, -22.19755133611119291 ) ) ;
#11293=CARTESIAN_POINT ( 'NONE',  ( -31.43908319763711390, 10.61114334766715928, 18.37190381572551701 ) ) ;
#11296=CARTESIAN_POINT ( 'NONE',  ( 84.74089592029042706, 19.84571403269345424, -77.42846521137805382 ) ) ;
#11297=CARTESIAN_POINT ( 'NONE',  ( 39.40195752203892710, 8.409560354027400209, 56.75838489642694640 ) ) ;
#11301=CARTESIAN_POINT ( 'NONE',  ( -29.50439180771546432, 10.29976981300626804, -50.07971974204068744 ) ) ;
#11309=CARTESIAN_POINT ( 'NONE',  ( 33.93974911725171495, 8.773765372885565128, 59.11309198735373371 ) ) ;
#11312=CARTESIAN_POINT ( 'NONE',  ( -168.7314919967217861, 83.83749564070829763, -9.267934599853210997 ) ) ;
#11315=CARTESIAN_POINT ( 'NONE',  ( 65.79663946071997316, 14.37086544438438196, -89.94145055465119754 ) ) ;
#11320=CARTESIAN_POINT ( 'NONE',  ( 186.5979919519637349, 85.84756789133378163, -11.79079488912463880 ) ) ;
#11321=CARTESIAN_POINT ( 'NONE',  ( 207.8398359204633721, 112.5208221429021478, 3.049908702302650099 ) ) ;
#11323=CARTESIAN_POINT ( 'NONE',  ( 40.37438610703018327, 8.537526699166107846, -23.72814077592008175 ) ) ;
#11333=CARTESIAN_POINT ( 'NONE',  ( -51.77431913897920879, 14.86466849149171132, 71.42491583832892843 ) ) ;
#11337=VERTEX_POINT ( 'NONE', #43395 ) ;
#11344=CARTESIAN_POINT ( 'NONE',  ( 102.7425154123292543, 25.56407025871218863, 36.86950736794638317 ) ) ;
#11345=ADVANCED_FACE ( 'NONE', ( #59224 ), #48305, .F. ) ;
#11347=EDGE_CURVE ( 'NONE', #50582, #10403, #7975, .T. ) ;
#11348=CARTESIAN_POINT ( 'NONE',  ( -61.75956139478098805, 16.58288496614414598, -72.92701606488500943 ) ) ;
#11350=CARTESIAN_POINT ( 'NONE',  ( 39.40195752203892710, 8.409560354027398432, -23.77526687496409608 ) ) ;
#11352=CARTESIAN_POINT ( 'NONE',  ( -157.0069571479807280, 72.18154199622283329, -69.45793912688546357 ) ) ;
#11355=VECTOR ( 'NONE', #55299, 1000.000000000000000 ) ;
#11356=AXIS2_PLACEMENT_3D ( 'NONE', #58095, #9916, #57404 ) ;
#11357=CARTESIAN_POINT ( 'NONE',  ( -48.58279704072702998, 14.07632445131079635, -38.91481426334084404 ) ) ;
#11359=CARTESIAN_POINT ( 'NONE',  ( 13.84704553156522522, 7.452804552247573433, 30.26612764413199486 ) ) ;
#11363=EDGE_LOOP ( 'NONE', ( #13795, #2521, #45036, #49200 ) ) ;
#11366=ORIENTED_EDGE ( 'NONE', *, *, #43567, .T. ) ;
#11367=CARTESIAN_POINT ( 'NONE',  ( -15.13254930056756109, 7.477527548005403979, -14.36566954603158131 ) ) ;
#11368=CARTESIAN_POINT ( 'NONE',  ( -52.66507163626135224, 14.05394608175174476, 44.94350458795448588 ) ) ;
#11371=CARTESIAN_POINT ( 'NONE',  ( -61.10880364359507411, 17.43879918625639647, -47.14754783338620570 ) ) ;
#11372=CARTESIAN_POINT ( 'NONE',  ( -15.27733754929849574, 8.502213909106947298, -15.09477148241088784 ) ) ;
#11378=ORIENTED_EDGE ( 'NONE', *, *, #58832, .T. ) ;
#11381=CARTESIAN_POINT ( 'NONE',  ( -24.85653282846401879, 9.618702155736652770, 94.99999999999866418 ) ) ;
#11382=CARTESIAN_POINT ( 'NONE',  ( 115.7731501832036116, 32.64791439093735903, -21.66803278067574468 ) ) ;
#11383=CARTESIAN_POINT ( 'NONE',  ( -102.2801239173131194, 32.78103895658057354, 18.67452391595144334 ) ) ;
#11384=CARTESIAN_POINT ( 'NONE',  ( 19.54475376904848716, 6.649964688461122542, 44.01079968644612705 ) ) ;
#11385=CARTESIAN_POINT ( 'NONE',  ( 137.4031600461560743, 44.79620770172221000, -23.29145164325822392 ) ) ;
#11386=ORIENTED_EDGE ( 'NONE', *, *, #7295, .F. ) ;
#11387=EDGE_LOOP ( 'NONE', ( #29145, #59839 ) ) ;
#11392=CARTESIAN_POINT ( 'NONE',  ( -33.13098007862451055, 9.875138601866709109, 71.87171333366060821 ) ) ;
#11393=CARTESIAN_POINT ( 'NONE',  ( -154.0718453320783112, 68.14976693162388699, -21.42403036335299049 ) ) ;
#11395=CARTESIAN_POINT ( 'NONE',  ( 188.5838389098762775, 88.03667982118678026, 63.96234997918834608 ) ) ;
#11396=CARTESIAN_POINT ( 'NONE',  ( -155.7495771807047049, 69.65980221699317099, 60.87747373296404163 ) ) ;
#11399=CARTESIAN_POINT ( 'NONE',  ( 103.4696172145934980, 25.87254488218942683, 13.49709838995913280 ) ) ;
#11404=CARTESIAN_POINT ( 'NONE',  ( 15.78827728214693060, 7.507518794609573831, 18.17015708224157322 ) ) ;
#11405=EDGE_CURVE ( 'NONE', #49946, #69216, #29774, .T. ) ;
#11410=ADVANCED_FACE ( 'NONE', ( #52154 ), #57780, .T. ) ;
#11412=CARTESIAN_POINT ( 'NONE',  ( -132.2352756077771687, 50.81350938245624604, -73.27096579721956005 ) ) ;
#11413=CARTESIAN_POINT ( 'NONE',  ( -131.2803255164625114, 50.14412978403780841, -37.18907415913850656 ) ) ;
#11415=CARTESIAN_POINT ( 'NONE',  ( 59.08202327466403858, 12.82375733818951069, -63.67486918714139676 ) ) ;
#11418=CARTESIAN_POINT ( 'NONE',  ( -128.7359537904937099, 48.39323004177004606, -89.14970310811136756 ) ) ;
#11422=CARTESIAN_POINT ( 'NONE',  ( 178.1999009735082211, 75.73911533785329198, -36.79823857645895657 ) ) ;
#11425=ORIENTED_EDGE ( 'NONE', *, *, #64872, .T. ) ;
#11427=CARTESIAN_POINT ( 'NONE',  ( 135.6647932137617829, 43.70902528961478595, 71.14781748300585207 ) ) ;
#11428=CARTESIAN_POINT ( 'NONE',  ( -71.26675986148643460, 19.63956187826083166, -41.36718459057324537 ) ) ;
#11429=CARTESIAN_POINT ( 'NONE',  ( -189.8133172329396814, 108.7279284458360564, 94.99999999999866418 ) ) ;
#11430=CARTESIAN_POINT ( 'NONE',  ( 90.91465859190773813, 20.92790537681857543, -49.48152920833616264 ) ) ;
#11431=CARTESIAN_POINT ( 'NONE',  ( -189.7987719395349302, 107.8653664616570609, 41.30349450692464330 ) ) ;
#11434=CARTESIAN_POINT ( 'NONE',  ( 112.1012908502484748, 29.75117929736500599, -50.69241971753201170 ) ) ;
#11436=CARTESIAN_POINT ( 'NONE',  ( -149.0764453401867513, 65.13297611514538232, -49.81283053149199702 ) ) ;
#11438=CARTESIAN_POINT ( 'NONE',  ( -144.3945994505580757, 59.96115386701889349, -47.80521614277407139 ) ) ;
#11440=CARTESIAN_POINT ( 'NONE',  ( 55.51528220483960041, 12.08323518953685571, 10.70683319743981343 ) ) ;
#11444=DIRECTION ( 'NONE',  ( -0.000000000000000000, 1.000000000000000000, -0.000000000000000000 ) ) ;
#11451=CARTESIAN_POINT ( 'NONE',  ( 88.52345267551655184, 20.07594890262053511, -77.42696361605551658 ) ) ;
#11452=CARTESIAN_POINT ( 'NONE',  ( 197.8436586345019919, 97.39326576892285914, 6.765139324472087878 ) ) ;
#11453=CARTESIAN_POINT ( 'NONE',  ( -98.67723517640905584, 30.98797878696539243, 17.75677604357209916 ) ) ;
#11455=ORIENTED_EDGE ( 'NONE', *, *, #3580, .F. ) ;
#11456=ORIENTED_EDGE ( 'NONE', *, *, #42622, .T. ) ;
#11458=CARTESIAN_POINT ( 'NONE',  ( 44.86216938219163097, 9.182565662897481218, 32.26643658086751998 ) ) ;
#11461=DIRECTION ( 'NONE',  ( 0.000000000000000000, 0.000000000000000000, 1.000000000000000000 ) ) ;
#11463=CARTESIAN_POINT ( 'NONE',  ( 204.6977192012829789, 108.0580384837234789, -36.32593103262158252 ) ) ;
#11465=CARTESIAN_POINT ( 'NONE',  ( -73.09214866197368110, 21.34321757515765228, -74.50211547328287054 ) ) ;
#11467=CARTESIAN_POINT ( 'NONE',  ( 45.35621884287173344, 10.27694987765648449, -47.70637205503341960 ) ) ;
#11471=ORIENTED_EDGE ( 'NONE', *, *, #10875, .T. ) ;
#11472=EDGE_CURVE ( 'NONE', #18508, #14330, #15533, .T. ) ;
#11473=CARTESIAN_POINT ( 'NONE',  ( -7.825402957745087207, 6.891034867348159842, -35.41807073194381417 ) ) ;
#11475=CARTESIAN_POINT ( 'NONE',  ( 91.12448333640236342, 22.07449368110501098, 58.03361031003960591 ) ) ;
#11476=CARTESIAN_POINT ( 'NONE',  ( 154.0293889979056985, 55.02370422818215445, -23.46008922554802467 ) ) ;
#11477=CARTESIAN_POINT ( 'NONE',  ( 36.30999198706538778, 9.040534725358941870, 17.40661586187119880 ) ) ;
#11478=CARTESIAN_POINT ( 'NONE',  ( 39.40195752203892710, -170.0000000000000000, -62.46436805589144114 ) ) ;
#11479=CARTESIAN_POINT ( 'NONE',  ( 113.9789034327318689, 31.76692991242614639, -90.59633938589010427 ) ) ;
#11480=CARTESIAN_POINT ( 'NONE',  ( 212.0873499799464525, 117.0618137521297228, 91.69696597238002767 ) ) ;
#11483=CARTESIAN_POINT ( 'NONE',  ( 59.29474530993688575, 12.86968658439548641, 70.67399659177640103 ) ) ;
#11487=CARTESIAN_POINT ( 'NONE',  ( -0.5780275525703870709, 6.527356703336897326, 35.66970812953940140 ) ) ;
#11497=CARTESIAN_POINT ( 'NONE',  ( -131.3096895243911035, 51.39228038925232056, -37.20263158582804408 ) ) ;
#11500=AXIS2_PLACEMENT_3D ( 'NONE', #61577, #28157, #60528 ) ;
#11502=CARTESIAN_POINT ( 'NONE',  ( 198.8732368717152212, 100.3103976497391017, -12.24965016599340473 ) ) ;
#11503=VECTOR ( 'NONE', #57608, 1000.000000000000000 ) ;
#11504=CARTESIAN_POINT ( 'NONE',  ( -3.253130881186334200, 7.643323950922368049, -75.72777455412368397 ) ) ;
#11506=EDGE_CURVE ( 'NONE', #62757, #49352, #7842, .T. ) ;
#11509=CARTESIAN_POINT ( 'NONE',  ( 79.52639011421921111, 18.17129627604989750, 12.82766093010378938 ) ) ;
#11510=B_SPLINE_CURVE_WITH_KNOTS ( 'NONE', 3,
 ( #6208, #64610, #21690, #22743, #28362, #16421, #22389, #49809, #42793, #38567, #60015, #32263, #17455, #53695, #64261, #5515, #11834, #33311, #26970, #44178, #38933, #60381, #48400, #43141, #7956, #2678, #55436, #45235, #61072, #29075, #12899, #28722, #34358, #66715, #35039, #13920, #24144, #35384, #50862, #45585, #44547, #51218, #40309, #56842, #23792, #56482, #2339, #67066, #18861, #29411, #50519, #66028, #13243, #61754 ),
 .UNSPECIFIED., .F., .F.,
 ( 4, 2, 2, 2, 2, 2, 2, 2, 2, 2, 2, 2, 2, 2, 2, 2, 2, 2, 2, 2, 2, 2, 2, 2, 2, 2, 4 ),
 ( 0.000000000000000000, 0.001958949513879419679, 0.002938424270819129519, 0.003917899027758839359, 0.004897373784698549198, 0.005876848541638259038, 0.006856323298577968878, 0.007835798055517678717, 0.008815272812457388557, 0.009794747569397098397, 0.01175369708327649206, 0.01273317184021620536, 0.01371264659715591867, 0.01567159611103534703, 0.01763054562491477364, 0.01958949513879420026, 0.02056896989573392398, 0.02154844465267364770, 0.02252791940961337142, 0.02350739416655309513, 0.02546634368043251828, 0.02644581843737221771, 0.02742529319431191714, 0.02840476795125161658, 0.02938424270819131601, 0.03036371746513101544, 0.03134319222207071487 ),
 .UNSPECIFIED. ) ;
#11511=CARTESIAN_POINT ( 'NONE',  ( -95.88693721180808893, 30.76307528361165922, 41.94858041200124177 ) ) ;
#11512=ADVANCED_FACE ( 'NONE', ( #65483 ), #1112, .F. ) ;
#11513=EDGE_CURVE ( 'NONE', #37653, #8034, #65133, .T. ) ;
#11514=EDGE_CURVE ( 'NONE', #19832, #29554, #53517, .T. ) ;
#11516=CARTESIAN_POINT ( 'NONE',  ( 117.3246714514015849, 33.42485879931865611, 7.745107550458741663 ) ) ;
#11519=EDGE_LOOP ( 'NONE', ( #42567, #36572 ) ) ;
#11521=CARTESIAN_POINT ( 'NONE',  ( -71.26675986148644881, 19.63956187826082456, -14.52263400010955330 ) ) ;
#11525=CARTESIAN_POINT ( 'NONE',  ( 161.7209903610254855, 61.03262545641850068, 43.10605864504380236 ) ) ;
#11528=ORIENTED_EDGE ( 'NONE', *, *, #63282, .F. ) ;
#11531=CARTESIAN_POINT ( 'NONE',  ( 157.1110115425986749, 57.37186251315585395, -89.81328548006501933 ) ) ;
#11532=CARTESIAN_POINT ( 'NONE',  ( 132.9557829392755082, 42.05591979570418459, 56.39519894757799534 ) ) ;
#11534=ORIENTED_EDGE ( 'NONE', *, *, #8440, .T. ) ;
#11535=ORIENTED_EDGE ( 'NONE', *, *, #18491, .F. ) ;
#11539=CARTESIAN_POINT ( 'NONE',  ( 63.01563776193091826, 12.67277567978500308, -23.87614024170608218 ) ) ;
#11541=CARTESIAN_POINT ( 'NONE',  ( -95.39675579260823213, 29.41944805607581159, 94.70441663738500893 ) ) ;
#11542=CARTESIAN_POINT ( 'NONE',  ( -149.5074843970971301, -170.0000000000000000, -96.00193171241933499 ) ) ;
#11544=CARTESIAN_POINT ( 'NONE',  ( -58.41593024021014458, 16.65492390105237774, 84.79537928362319121 ) ) ;
#11549=CARTESIAN_POINT ( 'NONE',  ( -100.2045077988687467, 32.86236599426410976, -88.98416475062359154 ) ) ;
#11553=CARTESIAN_POINT ( 'NONE',  ( 208.6132326550594485, 111.8685719053116969, -64.25973477317864990 ) ) ;
#11555=CARTESIAN_POINT ( 'NONE',  ( -73.81689110552359523, 20.53332132481499173, 5.347267905733100513 ) ) ;
#11556=CARTESIAN_POINT ( 'NONE',  ( 63.01563776193090405, 12.67277567978497643, 44.81296093922130552 ) ) ;
#11557=CARTESIAN_POINT ( 'NONE',  ( 22.28556289340100349, 7.803548444155007147, 33.76024460579878905 ) ) ;
#11567=ORIENTED_EDGE ( 'NONE', *, *, #12315, .T. ) ;
#11571=CARTESIAN_POINT ( 'NONE',  ( 156.3797504404255960, 58.07856685387022111, -77.89230977338574746 ) ) ;
#11573=EDGE_CURVE ( 'NONE', #27181, #780, #48230, .T. ) ;
#11575=CARTESIAN_POINT ( 'NONE',  ( 128.4224537826253822, 38.23837035195746381, -11.48689105586654335 ) ) ;
#11577=ORIENTED_EDGE ( 'NONE', *, *, #45926, .T. ) ;
#11578=VERTEX_POINT ( 'NONE', #55 ) ;
#11581=DIRECTION ( 'NONE',  ( -0.000000000000000000, 1.000000000000000000, -0.000000000000000000 ) ) ;
#11583=CARTESIAN_POINT ( 'NONE',  ( 63.01563776193090405, 12.67277567978497643, 71.65751152968501003 ) ) ;
#11584=CARTESIAN_POINT ( 'NONE',  ( -0.7076388175553633975, 7.538734751903870546, 62.04576903499332019 ) ) ;
#11593=CARTESIAN_POINT ( 'NONE',  ( -173.1211646369891071, 87.12891641440859303, -7.867406574286297527 ) ) ;
#11597=EDGE_CURVE ( 'NONE', #15908, #55797, #27880, .T. ) ;
#11602=CARTESIAN_POINT ( 'NONE',  ( 82.13067365723604496, 17.93447087949265750, 4.346969704001187651 ) ) ;
#11603=FACE_OUTER_BOUND ( 'NONE', #46869, .T. ) ;
#11605=CARTESIAN_POINT ( 'NONE',  ( -71.22878586122430988, 19.62649588091170472, 38.91628792690696059 ) ) ;
#11614=EDGE_LOOP ( 'NONE', ( #60041, #48564, #58806, #22707 ) ) ;
#11615=B_SPLINE_CURVE_WITH_KNOTS ( 'NONE', 3,
 ( #29175, #50620, #51670, #46377, #30557, #14389, #62573, #57293, #67177, #52009, #24938, #45698, #45344, #3824, #56592, #40073, #24603, #3476, #40761, #18964, #61859, #35841, #51330, #13008, #67856, #66825, #25294, #35140, #3145, #46729, #40412, #68199, #24257, #8414, #2438, #13684, #34466, #20008, #61180, #29867, #34807, #19650, #55908, #18618, #46036, #56245 ),
 .UNSPECIFIED., .F., .F.,
 ( 4, 2, 2, 2, 2, 2, 2, 2, 2, 2, 2, 2, 2, 2, 2, 2, 2, 2, 2, 2, 2, 2, 4 ),
 ( 0.02584318557310390577, 0.02743529570732764628, 0.02823135077443950786, 0.02902740584155136944, 0.03061951597577508913, 0.03221162610999880882, 0.03380373624422253198, 0.03459979131133437275, 0.03539584637844622045, 0.03619190144555806121, 0.03698795651266990892, 0.03858006664689361820, 0.03937612171400548672, 0.04017217678111735524, 0.04096823184822921682, 0.04176428691534107840, 0.04335639704956481544, 0.04494850718378853860, 0.04654061731801227564, 0.04813272745223600574, 0.04892878251934786732, 0.04972483758645972890, 0.05131694772068347288 ),
 .UNSPECIFIED. ) ;
#11620=CARTESIAN_POINT ( 'NONE',  ( -130.2196570250629293, 49.40815211106347959, -21.71403809251050632 ) ) ;
#11621=B_SPLINE_CURVE_WITH_KNOTS ( 'NONE', 3,
 ( #52545, #26163, #63802, #69415, #54249, #39489, #38446, #7496, #65535, #815, #7130, #55665, #54609, #49327, #28947, #65896, #6071, #28591, #27533, #66590, #12413, #1157, #12761, #18379, #17693, #28226, #22609, #60596, #49676, #12063, #44054, #22967, #23326, #1505, #33535, #39155, #22267, #48975, #17328, #43701, #54961, #60942, #33175, #38803 ),
 .UNSPECIFIED., .F., .F.,
 ( 4, 2, 2, 2, 2, 2, 2, 2, 2, 2, 2, 2, 2, 2, 2, 2, 2, 2, 2, 2, 2, 4 ),
 ( 0.000000000000000000, 0.003360573201437855057, 0.004200716501797282718, 0.005040859802156710812, 0.006721146402875505417, 0.007561289703234871061, 0.008401433003594235838, 0.009241576303953601482, 0.01008171960431296713, 0.01176200620503169321, 0.01260214950539103804, 0.01344229280575038113, 0.01428243610610972943, 0.01512257940646907425, 0.01680286600718778819, 0.01764300930754715210, 0.01848315260790651948, 0.02016343920862523342, 0.02184372580934394389, 0.02352401241006265437, 0.02520429901078136831, 0.02688458561150008225 ),
 .UNSPECIFIED. ) ;
#11627=CARTESIAN_POINT ( 'NONE',  ( -190.6985136298601731, 109.1272424661242582, -95.00000000000133582 ) ) ;
#11629=FACE_BOUND ( 'NONE', #32798, .T. ) ;
#11630=CARTESIAN_POINT ( 'NONE',  ( -0.3258398948454878097, 6.518608385615803691, -70.26394939446382182 ) ) ;
#11631=CARTESIAN_POINT ( 'NONE',  ( -180.0094637318086939, 96.72611451757710199, 62.18543092603484723 ) ) ;
#11632=CARTESIAN_POINT ( 'NONE',  ( 115.2709090239982714, 31.27821204311961267, -91.53183796548907480 ) ) ;
#11634=CARTESIAN_POINT ( 'NONE',  ( -84.23336401058614342, 25.60798568215574278, 16.12318571503568165 ) ) ;
#11637=CARTESIAN_POINT ( 'NONE',  ( -74.26325512636837800, 20.69286162067376367, -90.21751194609112190 ) ) ;
#11639=CARTESIAN_POINT ( 'NONE',  ( 158.3604774538084712, 58.34594647925808886, 17.52526914281743231 ) ) ;
#11640=CARTESIAN_POINT ( 'NONE',  ( 94.11733320392093560, 23.18939451097131865, -16.97069168030737174 ) ) ;
#11644=CARTESIAN_POINT ( 'NONE',  ( -31.43908319763709969, 10.61114334766715572, 3.371903815725488585 ) ) ;
#11647=CARTESIAN_POINT ( 'NONE',  ( 79.92842440418704086, 18.29578799637230802, -73.57133314052174455 ) ) ;
#11649=CARTESIAN_POINT ( 'NONE',  ( 103.5783816667154014, 27.01328802396631801, 87.34340838971257881 ) ) ;
#11650=DIRECTION ( 'NONE',  ( -0.000000000000000000, 1.000000000000000000, -0.000000000000000000 ) ) ;
#11651=CARTESIAN_POINT ( 'NONE',  ( 110.2429982417149290, 28.88204397445231209, 56.45576479620100940 ) ) ;
#11653=CARTESIAN_POINT ( 'NONE',  ( -48.23389383802714292, 13.99288361739332309, -72.69372053434236136 ) ) ;
#11655=DIRECTION ( 'NONE',  ( -0.000000000000000000, 1.000000000000000000, -0.000000000000000000 ) ) ;
#11656=DIRECTION ( 'NONE',  ( 0.000000000000000000, 0.000000000000000000, 1.000000000000000000 ) ) ;
#11657=EDGE_LOOP ( 'NONE', ( #8692, #66557, #51021, #55382 ) ) ;
#11661=VECTOR ( 'NONE', #11251, 1000.000000000000000 ) ;
#11662=CARTESIAN_POINT ( 'NONE',  ( 33.44035656425386094, 8.720466003183668491, 68.83548946330709839 ) ) ;
#11664=CARTESIAN_POINT ( 'NONE',  ( -166.5742238910466142, 81.57147158222488770, 61.49679445346814077 ) ) ;
#11668=ADVANCED_FACE ( 'NONE', ( #67240 ), #45055, .F. ) ;
#11672=CARTESIAN_POINT ( 'NONE',  ( 103.9685899589048148, 27.18106603025992740, -47.53878293330955529 ) ) ;
#11673=CARTESIAN_POINT ( 'NONE',  ( 188.5651904823862424, 88.01586411309104108, -16.26953988692886099 ) ) ;
#11674=CARTESIAN_POINT ( 'NONE',  ( -81.90266786693715062, 23.58030232261292269, -8.987966624609327937 ) ) ;
#11676=CARTESIAN_POINT ( 'NONE',  ( 43.35980717318837208, 8.957244490220903188, -9.899856988890338272 ) ) ;
#11677=CARTESIAN_POINT ( 'NONE',  ( 212.0180052085437978, 116.9552462415715297, -15.31765953654469925 ) ) ;
#11678=FACE_BOUND ( 'NONE', #45570, .T. ) ;
#11679=CARTESIAN_POINT ( 'NONE',  ( -61.51762070241281322, 16.51067482779403761, -38.90611071093341877 ) ) ;
#11682=DIRECTION ( 'NONE',  ( 0.000000000000000000, 0.000000000000000000, 1.000000000000000000 ) ) ;
#11683=CARTESIAN_POINT ( 'NONE',  ( 94.14197848494939080, 23.19876128416615657, -43.31134344884397080 ) ) ;
#11684=CARTESIAN_POINT ( 'NONE',  ( -51.77779688167512262, 14.86590802019196822, 57.91026681902796014 ) ) ;
#11686=CARTESIAN_POINT ( 'NONE',  ( 150.2794558856211040, 52.26944788078751003, 12.26467988490533578 ) ) ;
#11690=CARTESIAN_POINT ( 'NONE',  ( 55.61382797299288683, 11.07686102552914953, 9.233553562912945267 ) ) ;
#11691=LINE ( 'NONE', #44401, #11355 ) ;
#11697=CARTESIAN_POINT ( 'NONE',  ( 103.0026233023292974, 25.67408295205787994, 35.08790048083266555 ) ) ;
#11703=CARTESIAN_POINT ( 'NONE',  ( -152.5101325120252795, 68.10842280990925701, -62.27045260355250633 ) ) ;
#11704=CARTESIAN_POINT ( 'NONE',  ( 63.98689050258325750, 13.93365232918668362, 17.92090484651062354 ) ) ;
#11707=VECTOR ( 'NONE', #40828, 1000.000000000000000 ) ;
#11709=CARTESIAN_POINT ( 'NONE',  ( -52.45048892661850459, 15.03803514841137812, -35.67804398155381307 ) ) ;
#11714=CARTESIAN_POINT ( 'NONE',  ( 87.95968186927227350, 19.87904650044665900, 83.51289166538627740 ) ) ;
#11715=CARTESIAN_POINT ( 'NONE',  ( 181.0840389613909736, -170.0000000000000000, 90.49769528643878402 ) ) ;
#11719=CARTESIAN_POINT ( 'NONE',  ( -13.78293860383718972, 7.352367295275504588, -11.49084393374748281 ) ) ;
#11720=CARTESIAN_POINT ( 'NONE',  ( -47.95468448182521826, 12.89252559348045857, 40.25230722566315933 ) ) ;
#11724=CARTESIAN_POINT ( 'NONE',  ( -61.76386578474846090, 17.63453064612501819, -46.10104452603333414 ) ) ;
#11726=CARTESIAN_POINT ( 'NONE',  ( -11.13714165684778656, 8.138643170880696331, -22.80719565481673072 ) ) ;
#11729=ORIENTED_EDGE ( 'NONE', *, *, #3580, .T. ) ;
#11734=CARTESIAN_POINT ( 'NONE',  ( -142.9843132609582028, 60.12226089556227748, 15.08661930014882024 ) ) ;
#11735=CARTESIAN_POINT ( 'NONE',  ( 116.4569059613810680, 31.86445263670867334, 94.99999999999866418 ) ) ;
#11739=CARTESIAN_POINT ( 'NONE',  ( 140.8855094313933307, 47.03549517811091363, -14.04929102430893018 ) ) ;
#11743=AXIS2_PLACEMENT_3D ( 'NONE', #30170, #40369, #29126 ) ;
#11745=CARTESIAN_POINT ( 'NONE',  ( -11.57931195747592668, 7.164335452024273465, 17.28240326270761784 ) ) ;
#11746=CARTESIAN_POINT ( 'NONE',  ( 34.45817031441435319, 7.817703378455683527, -75.62602997148037787 ) ) ;
#11750=CARTESIAN_POINT ( 'NONE',  ( -37.07602570886409410, 10.58457435034603122, 59.58909574225179995 ) ) ;
#11751=CARTESIAN_POINT ( 'NONE',  ( 200.8303160266299017, 102.8412051751308809, 69.99246994815830192 ) ) ;
#11755=CARTESIAN_POINT ( 'NONE',  ( 204.6977192012829505, 108.0580384837234931, -78.17048162308530834 ) ) ;
#11762=CARTESIAN_POINT ( 'NONE',  ( 20.74852474914887424, 6.709938988646750424, 70.00598210749363659 ) ) ;
#11764=CARTESIAN_POINT ( 'NONE',  ( 13.84937401517046851, 6.446378549072247388, -62.61427068757215153 ) ) ;
#11765=VECTOR ( 'NONE', #41046, 1000.000000000000000 ) ;
#11771=DIRECTION ( 'NONE',  ( 0.000000000000000000, 0.000000000000000000, 1.000000000000000000 ) ) ;
#11772=CARTESIAN_POINT ( 'NONE',  ( 46.89006465517229572, 9.501960077668742954, -69.47552966857396939 ) ) ;
#11773=CARTESIAN_POINT ( 'NONE',  ( 56.94505604581136282, 12.37336791557970272, -74.47650229381035558 ) ) ;
#11776=DIRECTION ( 'NONE',  ( -0.000000000000000000, 1.000000000000000000, -0.000000000000000000 ) ) ;
#11780=CARTESIAN_POINT ( 'NONE',  ( 174.6176230994778109, 72.30829341023249413, -39.88575702694497238 ) ) ;
#11782=ORIENTED_EDGE ( 'NONE', *, *, #48104, .T. ) ;
#11783=CYLINDRICAL_SURFACE ( 'NONE', #44688, 7.500000000000013323 ) ;
#11784=CARTESIAN_POINT ( 'NONE',  ( 139.6326990672751549, 46.22017155708130076, 59.06439119612976896 ) ) ;
#11785=CARTESIAN_POINT ( 'NONE',  ( -75.64857587248467041, 21.19501514561450151, -35.74525540028072612 ) ) ;
#11787=DIRECTION ( 'NONE',  ( 0.000000000000000000, 0.000000000000000000, 1.000000000000000000 ) ) ;
#11788=CARTESIAN_POINT ( 'NONE',  ( -55.05276343752909440, 15.72344139423348430, -23.37177340799619785 ) ) ;
#11790=CARTESIAN_POINT ( 'NONE',  ( 113.4351684956570381, 30.38657459074488543, -50.22549693574652707 ) ) ;
#11792=CARTESIAN_POINT ( 'NONE',  ( -78.18897186942405142, 23.21604822208489338, 18.57365054920947856 ) ) ;
#11793=CARTESIAN_POINT ( 'NONE',  ( -142.0860844253783171, 59.41107357617637774, -43.43222315112575416 ) ) ;
#11797=VERTEX_POINT ( 'NONE', #28177 ) ;
#11803=CARTESIAN_POINT ( 'NONE',  ( -144.9439644317224634, 60.40328483334192811, 59.10885205279113563 ) ) ;
#11808=CARTESIAN_POINT ( 'NONE',  ( 92.21252738308862718, 22.47457138983956426, 32.18003665462427421 ) ) ;
#11810=CARTESIAN_POINT ( 'NONE',  ( -165.6754884515988522, -170.0000000000000000, -95.00000000000133582 ) ) ;
#11812=CARTESIAN_POINT ( 'NONE',  ( 94.02921784728462740, 22.08005910033070407, -68.91924186718193823 ) ) ;
#11816=CARTESIAN_POINT ( 'NONE',  ( 92.91022130985207639, 22.73448145304546131, 94.99999999999866418 ) ) ;
#11820=CARTESIAN_POINT ( 'NONE',  ( 46.76970795284346138, 9.482505412758886365, 38.87896366950010218 ) ) ;
#11824=CARTESIAN_POINT ( 'NONE',  ( 212.0075063341773216, 118.7912820769029167, -45.53480672108666027 ) ) ;
#11827=CARTESIAN_POINT ( 'NONE',  ( 42.71247067544614140, 9.879726907348455711, -49.85411309355188081 ) ) ;
#11831=CARTESIAN_POINT ( 'NONE',  ( -24.32471770265758337, 9.546495606312142002, 8.447192770170387277 ) ) ;
#11834=CARTESIAN_POINT ( 'NONE',  ( -84.60829019729341383, 24.67443150164869436, 87.01983487678488416 ) ) ;
#11837=CARTESIAN_POINT ( 'NONE',  ( 127.2107679985236217, 38.70844091144994792, 40.52525586269725721 ) ) ;
#11838=CARTESIAN_POINT ( 'NONE',  ( 35.44311777160621801, 8.940232499250164722, 16.94408402799438207 ) ) ;
#11843=DIRECTION ( 'NONE',  ( 0.000000000000000000, 0.000000000000000000, 1.000000000000000000 ) ) ;
#11845=CARTESIAN_POINT ( 'NONE',  ( 55.76255201544532270, 12.13275766515752352, 62.18578305727515243 ) ) ;
#11846=CARTESIAN_POINT ( 'NONE',  ( -26.49516976694651049, 8.831756547364873811, 16.53298603352267193 ) ) ;
#11849=CARTESIAN_POINT ( 'NONE',  ( 88.27048647651604085, 21.05338532470119262, 83.57569936033996782 ) ) ;
#11855=CARTESIAN_POINT ( 'NONE',  ( -130.5740389938243027, 49.65308610043480542, 17.15553663445870569 ) ) ;
#11858=CARTESIAN_POINT ( 'NONE',  ( -133.3923804760465543, 52.87100816290222838, -42.98098741808147594 ) ) ;
#11861=CARTESIAN_POINT ( 'NONE',  ( -120.4816138481824908, 43.03185659245511374, -47.62858304183759373 ) ) ;
#11865=LINE ( 'NONE', #49837, #50431 ) ;
#11867=CARTESIAN_POINT ( 'NONE',  ( -173.1211646369891355, -170.0000000000000000, -49.71195716475001092 ) ) ;
#11870=ORIENTED_EDGE ( 'NONE', *, *, #25827, .F. ) ;
#11871=CARTESIAN_POINT ( 'NONE',  ( -58.75378739419587504, 16.75118858561006263, 4.431123600893071668 ) ) ;
#11873=CARTESIAN_POINT ( 'NONE',  ( -152.4930836497867404, 68.09400557494207362, 31.33700391404592267 ) ) ;
#11875=CARTESIAN_POINT ( 'NONE',  ( -173.1211646369891355, 88.63826465341151106, -76.55650775521370122 ) ) ;
#11876=ORIENTED_EDGE ( 'NONE', *, *, #41160, .T. ) ;
#11880=ORIENTED_EDGE ( 'NONE', *, *, #66545, .T. ) ;
#11881=CARTESIAN_POINT ( 'NONE',  ( -120.5463017468902223, 43.07239852585537676, -90.83929640405872874 ) ) ;
#11883=CARTESIAN_POINT ( 'NONE',  ( -11.56945424397729205, 8.173256823723107800, -76.26585737041517632 ) ) ;
#11886=CARTESIAN_POINT ( 'NONE',  ( -7.825402957745085430, -170.0000000000000000, -77.26262132240753999 ) ) ;
#11889=CARTESIAN_POINT ( 'NONE',  ( -143.6098676033357435, 60.62137621171688551, -91.34574462907563941 ) ) ;
#11892=CARTESIAN_POINT ( 'NONE',  ( -36.37663950036511551, 10.45389057208229033, -10.30609290290592028 ) ) ;
#11894=CARTESIAN_POINT ( 'NONE',  ( 133.8566784816069344, 42.60093787723652525, 56.35489142945903751 ) ) ;
#11895=CARTESIAN_POINT ( 'NONE',  ( 21.44191228441539820, 7.755009954762319246, 59.40633199949923693 ) ) ;
#11899=ORIENTED_EDGE ( 'NONE', *, *, #69174, .F. ) ;
#11901=CARTESIAN_POINT ( 'NONE',  ( 207.3579397550547299, 110.0617317161169240, -90.49398837928671924 ) ) ;
#11902=CARTESIAN_POINT ( 'NONE',  ( -104.1225399044495674, 34.86084180570097857, 3.900553033110677692 ) ) ;
#11906=CARTESIAN_POINT ( 'NONE',  ( -35.99432170610151616, 10.38324794858010591, -48.79525134090449967 ) ) ;
#11907=CARTESIAN_POINT ( 'NONE',  ( -95.06174767693123329, 29.26266015133881737, 93.77071720667551347 ) ) ;
#11909=CARTESIAN_POINT ( 'NONE',  ( -130.1964689553232972, 49.39217932424203639, 71.12517339982724707 ) ) ;
#11910=CARTESIAN_POINT ( 'NONE',  ( -71.23176719684944658, 20.69188312694499032, -14.75110734384959166 ) ) ;
#11913=ORIENTED_EDGE ( 'NONE', *, *, #57575, .T. ) ;
#11914=CARTESIAN_POINT ( 'NONE',  ( -99.01653716841812525, 32.27413039285141139, -89.43734291363955435 ) ) ;
#11916=CYLINDRICAL_SURFACE ( 'NONE', #22859, 7.500000000000013323 ) ;
#11917=VERTEX_POINT ( 'NONE', #13747 ) ;
#11918=CARTESIAN_POINT ( 'NONE',  ( 182.7720841008444097, 80.32850885226588389, 29.49789156618269104 ) ) ;
#11921=CARTESIAN_POINT ( 'NONE',  ( -71.41745561414262511, 19.69148172991712187, 13.06265200711892582 ) ) ;
#11922=CARTESIAN_POINT ( 'NONE',  ( -118.7011544766493500, 43.11604763363181547, 67.10580360906620001 ) ) ;
#11923=CARTESIAN_POINT ( 'NONE',  ( -47.95468448182520405, 12.89252559348046567, 13.40775663519948679 ) ) ;
#11929=FACE_OUTER_BOUND ( 'NONE', #40187, .T. ) ;
#11930=CARTESIAN_POINT ( 'NONE',  ( -189.0973937025975999, 108.4049737838939222, 89.83184869644205151 ) ) ;
#11935=CARTESIAN_POINT ( 'NONE',  ( -83.14462298835724141, 24.07775853418030110, 31.88262967278052784 ) ) ;
#11936=CARTESIAN_POINT ( 'NONE',  ( -25.07735481787161547, 9.648965052008781740, -73.64150853364553484 ) ) ;
#11937=CARTESIAN_POINT ( 'NONE',  ( 46.65860211212412167, 10.48377752989033773, 39.37290686888943014 ) ) ;
#11938=CARTESIAN_POINT ( 'NONE',  ( -30.95355748062276291, 9.511738996772320931, 57.06100499665286918 ) ) ;
#11939=CARTESIAN_POINT ( 'NONE',  ( -145.3109762780891003, 60.69959559383372749, 17.60952691763336375 ) ) ;
#11944=CARTESIAN_POINT ( 'NONE',  ( 32.90051628396145134, 8.664124555952444240, -20.04662842472982121 ) ) ;
#11946=CARTESIAN_POINT ( 'NONE',  ( -6.843910203392213454, 7.836697961436718707, 18.22254118960022140 ) ) ;
#11947=CARTESIAN_POINT ( 'NONE',  ( 141.1579982455003233, 47.21428277316857702, 92.45156317765301424 ) ) ;
#11956=CYLINDRICAL_SURFACE ( 'NONE', #65996, 7.500000000000013323 ) ;
#11959=CARTESIAN_POINT ( 'NONE',  ( 157.4703587214989398, -170.0000000000000000, -77.96873488960135035 ) ) ;
#11960=CARTESIAN_POINT ( 'NONE',  ( -125.8938041572051105, 47.69968343338781125, -88.60280507916129977 ) ) ;
#11965=VERTEX_POINT ( 'NONE', #2688 ) ;
#11966=CARTESIAN_POINT ( 'NONE',  ( 79.38459371357855332, 17.07499996355402061, 12.37235545723701691 ) ) ;
#11968=CARTESIAN_POINT ( 'NONE',  ( -72.76696720809546548, 20.16136115364206916, 42.57569858987972822 ) ) ;
#11969=ORIENTED_EDGE ( 'NONE', *, *, #7224, .F. ) ;
#11972=CARTESIAN_POINT ( 'NONE',  ( 131.9963487224087544, 40.31229003000635913, -89.93695264016190549 ) ) ;
#11974=CARTESIAN_POINT ( 'NONE',  ( -123.6618353044034819, 46.23845779494349983, 4.100425436027088644 ) ) ;
#11975=CARTESIAN_POINT ( 'NONE',  ( 91.67571176799447130, 21.20498955963028465, 4.813890606363044000 ) ) ;
#11980=EDGE_CURVE ( 'NONE', #20401, #50694, #23794, .T. ) ;
#11982=CARTESIAN_POINT ( 'NONE',  ( 33.75794032130628608, 8.754084575552409930, 42.37720922280519886 ) ) ;
#11983=CARTESIAN_POINT ( 'NONE',  ( -180.6209674222602359, 97.47999311542514533, -42.37861601742196882 ) ) ;
#11988=ORIENTED_EDGE ( 'NONE', *, *, #55941, .F. ) ;
#11989=CARTESIAN_POINT ( 'NONE',  ( 136.7690435008551049, 44.39743995805024213, -77.28318001848430185 ) ) ;
#11990=CARTESIAN_POINT ( 'NONE',  ( -147.7925265216585444, 64.04960911618974251, -76.46199663651751166 ) ) ;
#11991=VERTEX_POINT ( 'NONE', #11556 ) ;
#11993=FACE_BOUND ( 'NONE', #51805, .T. ) ;
#11994=CARTESIAN_POINT ( 'NONE',  ( -6.840981040171505434, 6.828436339979227832, -62.31109642460706510 ) ) ;
#11995=CARTESIAN_POINT ( 'NONE',  ( -178.2448732545371115, 94.58403736950708662, 70.66284363813151970 ) ) ;
#11998=CARTESIAN_POINT ( 'NONE',  ( -6.843910203392213454, 7.836697961436722260, 45.06709178006389038 ) ) ;
#11999=CARTESIAN_POINT ( 'NONE',  ( 8.000000000000007105, 249.8719672152120381, 94.99999999999866418 ) ) ;
#12001=CARTESIAN_POINT ( 'NONE',  ( -6.125624616441583292, 7.794071945221087816, -8.764598286888389822 ) ) ;
#12002=CARTESIAN_POINT ( 'NONE',  ( -15.27733754929849930, 8.502213909106947298, 38.59432969851645367 ) ) ;
#12003=CARTESIAN_POINT ( 'NONE',  ( 116.8937673311172887, 32.08228998570057655, 6.790944445358706894 ) ) ;
#12004=CARTESIAN_POINT ( 'NONE',  ( 94.11595392909974578, 23.18887043179185525, -15.96272041242249884 ) ) ;
#12006=CARTESIAN_POINT ( 'NONE',  ( -38.16652041892307778, 11.81761816422915956, 7.520151233602119234 ) ) ;
#12009=CARTESIAN_POINT ( 'NONE',  ( 79.22872707466395070, 18.07970189365808622, -68.92354796247994386 ) ) ;
#12011=CARTESIAN_POINT ( 'NONE',  ( 106.8650810127286235, 28.45160516703612075, 84.09606632055420050 ) ) ;
#12013=CARTESIAN_POINT ( 'NONE',  ( -15.21063934378433657, 7.484993339139951019, 89.95709727327218275 ) ) ;
#12016=CARTESIAN_POINT ( 'NONE',  ( 133.8566784816069344, 42.60093787723652525, -51.02331093239568816 ) ) ;
#12018=CARTESIAN_POINT ( 'NONE',  ( -77.82491691702773551, 23.07808431488692946, -88.83991494168476777 ) ) ;
#12020=CARTESIAN_POINT ( 'NONE',  ( -188.6739852773921200, 108.2139733222100375, -67.25001060397961794 ) ) ;
#12024=CARTESIAN_POINT ( 'NONE',  ( 177.7889574972182345, 75.33777460203559428, 56.90074107153713356 ) ) ;
#12028=CARTESIAN_POINT ( 'NONE',  ( -166.7136514167008841, 81.71618216218793407, -19.27443722847174712 ) ) ;
#12029=LINE ( 'NONE', #27852, #18305 ) ;
#12031=CARTESIAN_POINT ( 'NONE',  ( 92.21252738308859875, 22.47457138983955360, 5.335486064160578579 ) ) ;
#12033=CARTESIAN_POINT ( 'NONE',  ( 10.31616749326173377, 7.393414706728906438, 59.22449557915167162 ) ) ;
#12034=B_SPLINE_CURVE_WITH_KNOTS ( 'NONE', 3,
 ( #52225, #14259, #51879, #63822, #9673, #31134, #35718, #37083, #25855, #58525, #47283, #5066, #16659, #53929, #16316, #1530, #37419, #59216, #53589, #27557, #17352, #59557, #38827, #48644, #32841, #65203, #16998, #5752, #22289, #60276, #27913, #6099, #59907, #6803, #38113, #37772, #21586, #1184, #28255, #11035, #64857, #48298, #32498, #487, #131 ),
 .UNSPECIFIED., .F., .F.,
 ( 4, 2, 2, 1, 2, 2, 2, 2, 2, 2, 2, 2, 2, 2, 2, 2, 2, 2, 2, 2, 2, 2, 4 ),
 ( 0.02345095402629350512, 0.02491692321306681820, 0.02564990780645347995, 0.02638289239984013823, 0.02711587699322679998, 0.02784886158661346173, 0.02931483077338677828, 0.03004781536677343656, 0.03078079996016009484, 0.03224676914693341834, 0.03297975374032006968, 0.03371273833370672102, 0.03517870752048002370, 0.03664467670725332638, 0.03737766130063997772, 0.03811064589402662905, 0.03957661508079992480, 0.04104258426757322747, 0.04250855345434652321, 0.04324153804773317455, 0.04397452264111982589, 0.04544049182789310082, 0.04690646101466638962 ),
 .UNSPECIFIED. ) ;
#12036=CARTESIAN_POINT ( 'NONE',  ( 46.65037935242575884, 9.463293687292223311, -14.33328965919755404 ) ) ;
#12037=CARTESIAN_POINT ( 'NONE',  ( 205.1049299651095623, 106.9023875785546096, -9.481380442157899324 ) ) ;
#12038=FACE_BOUND ( 'NONE', #3398, .T. ) ;
#12039=CARTESIAN_POINT ( 'NONE',  ( -58.76006735892197952, 15.70681061434692616, -49.24053391377918132 ) ) ;
#12041=DIRECTION ( 'NONE',  ( -0.000000000000000000, 1.000000000000000000, -0.000000000000000000 ) ) ;
#12042=FACE_OUTER_BOUND ( 'NONE', #65774, .T. ) ;
#12043=CARTESIAN_POINT ( 'NONE',  ( -52.67596829228263289, 15.09584868440940220, 57.53187801079657504 ) ) ;
#12044=CARTESIAN_POINT ( 'NONE',  ( -180.3161328724958139, 97.10341277064807741, 13.61587359508545880 ) ) ;
#12045=CARTESIAN_POINT ( 'NONE',  ( 210.9631450001601252, 117.1791136960929833, 59.39267853008134068 ) ) ;
#12049=CARTESIAN_POINT ( 'NONE',  ( 56.53635105806417016, 11.26263375223564012, 6.682842904946032725 ) ) ;
#12051=ORIENTED_EDGE ( 'NONE', *, *, #38853, .F. ) ;
#12056=CARTESIAN_POINT ( 'NONE',  ( -56.72676045871359918, 16.18052435693491375, -23.18658342442263987 ) ) ;
#12057=CARTESIAN_POINT ( 'NONE',  ( 104.7147873368644753, 26.40702926859708910, 42.20357219318257336 ) ) ;
#12062=LINE ( 'NONE', #33534, #26268 ) ;
#12063=CARTESIAN_POINT ( 'NONE',  ( 164.1352994389932292, 64.33767534192701021, 33.45996833887929967 ) ) ;
#12065=CARTESIAN_POINT ( 'NONE',  ( -151.6797345123118248, 67.37848486615943955, -61.96523196077820472 ) ) ;
#12066=CARTESIAN_POINT ( 'NONE',  ( 69.48877314113909165, 15.30784187978993138, 14.26448168032291086 ) ) ;
#12070=CARTESIAN_POINT ( 'NONE',  ( -49.12372073857199695, 14.20664392157176437, -47.33574279618618164 ) ) ;
#12071=AXIS2_PLACEMENT_3D ( 'NONE', #4718, #63816, #37077 ) ;
#12072=DIRECTION ( 'NONE',  ( -0.000000000000000000, 1.000000000000000000, -0.000000000000000000 ) ) ;
#12073=CARTESIAN_POINT ( 'NONE',  ( -133.1640943168118838, 52.70734926280010058, -13.70763724439404108 ) ) ;
#12074=EDGE_CURVE ( 'NONE', #33561, #54282, #62412, .T. ) ;
#12078=DIRECTION ( 'NONE',  ( -0.000000000000000000, 1.000000000000000000, -0.000000000000000000 ) ) ;
#12083=EDGE_LOOP ( 'NONE', ( #52099, #51515 ) ) ;
#12084=CARTESIAN_POINT ( 'NONE',  ( -14.19447842053093645, 7.389800932646227061, -12.10543927043131518 ) ) ;
#12085=CARTESIAN_POINT ( 'NONE',  ( -165.7123887345808555, 80.68215826500505727, 90.82995548501529015 ) ) ;
#12086=CARTESIAN_POINT ( 'NONE',  ( -48.57297291660696459, 13.03920345822338511, -19.68077099140970532 ) ) ;
#12087=CARTESIAN_POINT ( 'NONE',  ( 105.8203563788591026, 26.88901185006195860, -10.51577773048208364 ) ) ;
#12088=CARTESIAN_POINT ( 'NONE',  ( -31.43908319763709969, 10.61114334766715928, 72.06100499665289760 ) ) ;
#12090=CARTESIAN_POINT ( 'NONE',  ( -71.43874587651173158, 19.69883891272895227, -71.47845090063621853 ) ) ;
#12095=VERTEX_POINT ( 'NONE', #55886 ) ;
#12096=CARTESIAN_POINT ( 'NONE',  ( 65.40383840050409958, 14.27443447873231186, -23.50236838888156043 ) ) ;
#12099=CARTESIAN_POINT ( 'NONE',  ( -94.85061234775061223, 29.16417548023186157, -43.57258393726064583 ) ) ;
#12103=DIRECTION ( 'NONE',  ( 0.000000000000000000, -0.000000000000000000, -1.000000000000000000 ) ) ;
#12110=VECTOR ( 'NONE', #66719, 1000.000000000000000 ) ;
#12112=CARTESIAN_POINT ( 'NONE',  ( -15.27748264047829529, 7.491388194171917370, 11.75137412820307858 ) ) ;
#12113=CARTESIAN_POINT ( 'NONE',  ( -190.6985136298601731, 109.1272424661242582, 94.99999999999866418 ) ) ;
#12114=CARTESIAN_POINT ( 'NONE',  ( 57.39083379741710900, 11.43779987330584191, -21.36185840037164496 ) ) ;
#12121=DIRECTION ( 'NONE',  ( -0.000000000000000000, 1.000000000000000000, -0.000000000000000000 ) ) ;
#12122=CARTESIAN_POINT ( 'NONE',  ( -155.5978531700835958, 69.52241200678679434, 69.44947247927566991 ) ) ;
#12123=CARTESIAN_POINT ( 'NONE',  ( -4.506365319453816909, 7.705038994660847962, -49.64818903867375610 ) ) ;
#12125=CARTESIAN_POINT ( 'NONE',  ( -165.8758279540429896, 79.40953312850696477, -93.88874443287481597 ) ) ;
#12127=FACE_BOUND ( 'NONE', #65489, .T. ) ;
#12128=DIRECTION ( 'NONE',  ( -0.000000000000000000, 1.000000000000000000, -0.000000000000000000 ) ) ;
#12132=CARTESIAN_POINT ( 'NONE',  ( -130.1964689553233256, 49.39217932424207902, -63.09757955249121864 ) ) ;
#12133=CARTESIAN_POINT ( 'NONE',  ( -102.7447593990059005, 34.14748189312171434, -76.85912785543963821 ) ) ;
#12141=CARTESIAN_POINT ( 'NONE',  ( 186.5227155285546417, 84.28235524483832819, 85.32269636523660949 ) ) ;
#12142=ORIENTED_EDGE ( 'NONE', *, *, #7636, .F. ) ;
#12145=CARTESIAN_POINT ( 'NONE',  ( 178.4027079424739952, 75.93756746109791322, -36.71741922764324784 ) ) ;
#12146=CARTESIAN_POINT ( 'NONE',  ( 162.0862735437575282, 62.63196145447161456, 4.134242840469689817 ) ) ;
#12149=CARTESIAN_POINT ( 'NONE',  ( -78.66644367742111399, -170.0000000000000000, -15.77090004125421352 ) ) ;
#12151=CARTESIAN_POINT ( 'NONE',  ( -71.56718866013696356, 19.74312628447964357, -40.14419485704286927 ) ) ;
#12153=CARTESIAN_POINT ( 'NONE',  ( 92.21267147730743829, 21.40196534721315302, -38.29018140383976032 ) ) ;
#12154=CARTESIAN_POINT ( 'NONE',  ( -47.79955240516188297, 13.88975739862081937, -17.84404308398329064 ) ) ;
#12158=DIRECTION ( 'NONE',  ( 0.000000000000000000, 0.000000000000000000, 1.000000000000000000 ) ) ;
#12159=EDGE_CURVE ( 'NONE', #14540, #43079, #56548, .T. ) ;
#12163=CARTESIAN_POINT ( 'NONE',  ( 150.3360255159550150, -170.0000000000000000, -95.00000000000133582 ) ) ;
#12166=DIRECTION ( 'NONE',  ( -0.8160245890732938934, -0.5780171883497599028, 0.000000000000000000 ) ) ;
#12170=CYLINDRICAL_SURFACE ( 'NONE', #35634, 7.500000000000020428 ) ;
#12173=CARTESIAN_POINT ( 'NONE',  ( -119.6995109608660925, 42.54844499216733311, 60.72834450685288488 ) ) ;
#12175=CARTESIAN_POINT ( 'NONE',  ( 40.38495044702527537, 9.554194848483444247, 3.117968398919370276 ) ) ;
#12176=CARTESIAN_POINT ( 'NONE',  ( 94.06703982324145841, 22.09435144471460433, -69.16872801670120907 ) ) ;
#12180=ORIENTED_EDGE ( 'NONE', *, *, #21909, .F. ) ;
#12181=CARTESIAN_POINT ( 'NONE',  ( 43.14712943604301643, 8.926114770663669873, 43.91642105177349720 ) ) ;
#12182=CARTESIAN_POINT ( 'NONE',  ( 201.5903370237274430, 102.1785392640257726, -23.82087321366149979 ) ) ;
#12185=CARTESIAN_POINT ( 'NONE',  ( 211.8382652195006983, 118.5282575235990237, -41.50942527998029163 ) ) ;
#12187=CARTESIAN_POINT ( 'NONE',  ( -109.3553681454883844, 36.52260784104394276, 62.32349516983876470 ) ) ;
#12188=CARTESIAN_POINT ( 'NONE',  ( -25.80058235236790409, 8.733375263008339218, -37.84754545538757498 ) ) ;
#12192=CARTESIAN_POINT ( 'NONE',  ( -23.99957301099517792, 9.503061049698493079, 9.889415725718228245 ) ) ;
#12197=CARTESIAN_POINT ( 'NONE',  ( 128.3889472838589256, 39.37765603157610173, 42.16720712859076770 ) ) ;
#12202=CARTESIAN_POINT ( 'NONE',  ( 210.5879448407857808, 114.7852148663112359, 85.74156794298586703 ) ) ;
#12207=CARTESIAN_POINT ( 'NONE',  ( -15.07235766390728848, 8.482541916553470784, 8.823573041229387570 ) ) ;
#12209=CARTESIAN_POINT ( 'NONE',  ( -103.2129897037410871, 33.25684593987698889, -61.90293558496989590 ) ) ;
#12210=CARTESIAN_POINT ( 'NONE',  ( 126.4633682455861816, 38.28837286275646079, -15.39085948919035829 ) ) ;
#12216=CARTESIAN_POINT ( 'NONE',  ( -165.6397095829521788, 80.60756690931943069, -42.82113700829442138 ) ) ;
#12219=CARTESIAN_POINT ( 'NONE',  ( -165.6438506416219241, 79.17342941146682733, 91.39850628321933357 ) ) ;
#12226=CARTESIAN_POINT ( 'NONE',  ( -0.8863172752569257185, 7.545240277686259489, -66.88547064642474993 ) ) ;
#12231=CARTESIAN_POINT ( 'NONE',  ( 197.3054165770396935, 96.72615186924558373, -45.13381048724120603 ) ) ;
#12233=CARTESIAN_POINT ( 'NONE',  ( -95.05323930133205579, 30.36974142673411947, 40.08974556234316822 ) ) ;
#12234=CARTESIAN_POINT ( 'NONE',  ( 23.28785143291466042, 6.856621069835718174, -43.52013114503547087 ) ) ;
#12235=CARTESIAN_POINT ( 'NONE',  ( 116.8917656767876423, 33.20682060519247614, 13.74620126077677007 ) ) ;
#12236=ORIENTED_EDGE ( 'NONE', *, *, #32185, .F. ) ;
#12237=B_SPLINE_CURVE_WITH_KNOTS ( 'NONE', 3,
 ( #57820, #31096, #64469, #47930, #58486, #11000, #52193, #4011, #25477, #46916, #52534, #47247, #9979, #68380, #4688, #20181, #41639, #63093, #14897, #68706, #41980, #21222, #15254, #42668, #36714, #60930, #27878, #50030, #16622, #66236, #18026, #38793, #28216, #48608, #44761, #16960, #22257, #53895, #49317, #28576, #59874, #446, #38079, #32809, #49665, #5717, #17318 ),
 .UNSPECIFIED., .F., .F.,
 ( 4, 2, 2, 2, 2, 2, 2, 2, 2, 2, 2, 2, 1, 2, 2, 2, 2, 2, 2, 2, 2, 2, 2, 4 ),
 ( 0.000000000000000000, 0.001493793014771585851, 0.002240689522157379536, 0.002987586029543173004, 0.004481379044314756470, 0.005228275551700559479, 0.005975172059086361620, 0.007468965073857955494, 0.008215861581243747228, 0.008962758088629538961, 0.01045655110340111375, 0.01120344761078690202, 0.01195034411817268681, 0.01269724062555847161, 0.01344413713294425813, 0.01493793014771582772, 0.01568482665510160037, 0.01643172316248737302, 0.01792551617725893220, 0.01941930919203049138, 0.02016620569941626404, 0.02091310220680203669, 0.02240689522157357505, 0.02390068823634511341 ),
 .UNSPECIFIED. ) ;
#12238=CARTESIAN_POINT ( 'NONE',  ( 181.0840389613909736, 80.03940679743415387, 71.15314469597512925 ) ) ;
#12241=CARTESIAN_POINT ( 'NONE',  ( 180.2565361171340612, 79.19912802278402353, 29.34240539128484215 ) ) ;
#12244=CARTESIAN_POINT ( 'NONE',  ( -12.40598104375063393, 8.242193636955557068, -63.80355163731987744 ) ) ;
#12245=ORIENTED_EDGE ( 'NONE', *, *, #42965, .T. ) ;
#12246=CARTESIAN_POINT ( 'NONE',  ( 161.7048274740121201, 61.01946783654762640, 30.70182928664277355 ) ) ;
#12248=CARTESIAN_POINT ( 'NONE',  ( -78.18897186942400879, 23.21604822208488983, -35.11545063171787007 ) ) ;
#12249=ORIENTED_EDGE ( 'NONE', *, *, #63682, .T. ) ;
#12250=B_SPLINE_CURVE_WITH_KNOTS ( 'NONE', 3,
 ( #47252, #43696, #65528, #22604, #11006, #54954, #33530, #5722, #22263, #16967, #65174, #12057, #38438, #43354, #6775, #27884, #16628, #54605, #1500, #65892, #5393, #17324, #6433, #11344, #6066, #59879, #49671, #11697, #26846, #38799, #32469, #64828, #32815, #53900, #48273, #54245, #39151, #38084, #33171, #64475, #27528, #22960, #17687, #48969 ),
 .UNSPECIFIED., .F., .F.,
 ( 4, 2, 2, 2, 2, 2, 2, 2, 2, 2, 2, 2, 2, 2, 2, 2, 2, 2, 2, 2, 2, 4 ),
 ( 0.000000000000000000, 0.001533942663855609968, 0.003067885327711219936, 0.004601827991566829687, 0.005368799323494632611, 0.006135770655422436402, 0.007669713319278056995, 0.008436684651205868593, 0.009203655983133680191, 0.01073759864698928777, 0.01150456997891710111, 0.01227154131084491617, 0.01303851264277272777, 0.01380548397470054110, 0.01533942663855617124, 0.01687336930241179617, 0.01840731196626742283, 0.01994125463012304950, 0.02070822596205086283, 0.02147519729397867616, 0.02300913995783434099, 0.02454308262169000582 ),
 .UNSPECIFIED. ) ;
#12252=CARTESIAN_POINT ( 'NONE',  ( -37.07602570886410831, 10.58457435034602589, -20.94455602913923187 ) ) ;
#12253=CARTESIAN_POINT ( 'NONE',  ( 150.3360255159550150, 52.31024849487489803, -95.00000000000133582 ) ) ;
#12254=CARTESIAN_POINT ( 'NONE',  ( -126.7944042662568478, 48.29830493043728268, 3.815832165402863296 ) ) ;
#12255=CARTESIAN_POINT ( 'NONE',  ( 22.15943197741200876, 7.796127622097904109, 60.39464998070587853 ) ) ;
#12259=ORIENTED_EDGE ( 'NONE', *, *, #4218, .F. ) ;
#12262=CARTESIAN_POINT ( 'NONE',  ( -106.4728934171453716, 36.10295170132727094, 4.951394827835590817 ) ) ;
#12263=DIRECTION ( 'NONE',  ( -0.000000000000000000, 1.000000000000000000, -0.000000000000000000 ) ) ;
#12264=CARTESIAN_POINT ( 'NONE',  ( -95.10076455013715702, 29.28088892350594108, 89.51400794333316924 ) ) ;
#12266=CARTESIAN_POINT ( 'NONE',  ( -128.7810612886105446, 48.42424427998344072, 58.03872734881966977 ) ) ;
#12267=CARTESIAN_POINT ( 'NONE',  ( -73.09214866197368110, 21.34321757515764162, -20.81301429235548994 ) ) ;
#12269=CARTESIAN_POINT ( 'NONE',  ( 79.19132716134490124, 17.01584750883626995, 63.06170514846407116 ) ) ;
#12271=CARTESIAN_POINT ( 'NONE',  ( 33.76124497394584267, 7.742545529019359662, 42.38094193253945008 ) ) ;
#12278=CARTESIAN_POINT ( 'NONE',  ( 149.9872551245001375, 52.05943539582081314, -43.04961227817129554 ) ) ;
#12283=CARTESIAN_POINT ( 'NONE',  ( -189.8133172329396814, 108.7279284458360564, 94.99999999999866418 ) ) ;
#12284=ORIENTED_EDGE ( 'NONE', *, *, #8092, .F. ) ;
#12286=CARTESIAN_POINT ( 'NONE',  ( 110.2429982417149574, -170.0000000000000000, -77.76698815611739235 ) ) ;
#12288=CARTESIAN_POINT ( 'NONE',  ( -81.67992981004164221, 23.49232121719083111, 31.04606863069344769 ) ) ;
#12289=CARTESIAN_POINT ( 'NONE',  ( 150.2193536046551401, 53.46717047532149536, -72.40446139084801302 ) ) ;
#12290=CARTESIAN_POINT ( 'NONE',  ( 42.71680114082826663, 9.880016734137544887, 44.15935619967898873 ) ) ;
#12296=CARTESIAN_POINT ( 'NONE',  ( 181.0840389613909736, -170.0000000000000000, -24.38050707541595230 ) ) ;
#12297=ORIENTED_EDGE ( 'NONE', *, *, #62855, .T. ) ;
#12298=CARTESIAN_POINT ( 'NONE',  ( 32.37980458033285203, 8.611076697115699119, -13.62945249871878772 ) ) ;
#12301=CARTESIAN_POINT ( 'NONE',  ( -1.096061481932296022, 7.553048580900439291, 61.13948011263546789 ) ) ;
#12302=CARTESIAN_POINT ( 'NONE',  ( 199.3120637967379025, 100.8716943732679141, -92.27816652752858317 ) ) ;
#12305=ORIENTED_EDGE ( 'NONE', *, *, #28347, .T. ) ;
#12306=B_SPLINE_CURVE_WITH_KNOTS ( 'NONE', 3,
 ( #62129, #35405, #20595, #56868, #9362, #47324, #46645, #57212, #4093, #24855, #25558, #19926, #3397, #58235, #46992, #41028, #30473, #51923, #10052, #68454, #3735, #68781, #67771, #68120, #42058, #30827, #8687, #63179, #67422, #52943, #20261, #46293, #14976, #36442, #41381, #62838, #57895, #14639, #36103, #9715, #31180, #4430, #25894, #63517, #26915, #32538, #63866, #42406 ),
 .UNSPECIFIED., .F., .F.,
 ( 4, 2, 2, 2, 2, 2, 2, 2, 2, 2, 2, 2, 2, 2, 2, 2, 2, 2, 2, 2, 2, 2, 2, 4 ),
 ( 0.000000000000000000, 0.003619254076116482609, 0.004524067595145613886, 0.005428881114174745164, 0.007238508152232934860, 0.008143321671262049657, 0.009048135190291161853, 0.01085776222834937237, 0.01176257574737846201, 0.01266738926640754818, 0.01357220278543663783, 0.01447701630446572574, 0.01538182982349481191, 0.01628664334252390156, 0.01719145686155298947, 0.01809627038058207738, 0.01900108389961116875, 0.01990589741864025666, 0.02171552445669843595, 0.02262033797572754468, 0.02352515149475665340, 0.02533477853281487086, 0.02714440557087308831, 0.02895403260893130923 ),
 .UNSPECIFIED. ) ;
#12311=CARTESIAN_POINT ( 'NONE',  ( 160.5141379054754225, 60.05651755415397730, -9.910344286968784999 ) ) ;
#12314=CARTESIAN_POINT ( 'NONE',  ( -132.7932380098740452, 52.44226555691696490, -93.12280453660946478 ) ) ;
#12315=EDGE_CURVE ( 'NONE', #26262, #26264, #1108, .T. ) ;
#12318=EDGE_LOOP ( 'NONE', ( #38470, #65477 ) ) ;
#12319=CARTESIAN_POINT ( 'NONE',  ( 12.46277766093406569, 6.416700641561365437, 44.25508861672395966 ) ) ;
#12322=ADVANCED_FACE ( 'NONE', ( #23010 ), #44462, .T. ) ;
#12324=CARTESIAN_POINT ( 'NONE',  ( -146.1260528621668300, 61.36307454672304118, -75.86784781446887393 ) ) ;
#12326=CARTESIAN_POINT ( 'NONE',  ( 93.32502112557682494, 21.81526022999040038, 6.952080423476055593 ) ) ;
#12330=B_SPLINE_CURVE_WITH_KNOTS ( 'NONE', 3,
 ( #34453, #44639, #61843, #55530, #2425, #17909, #29495, #18252, #29157, #66462, #23882, #24589, #66122, #18951, #50959, #13333, #45684, #46022, #55180, #67489, #13668, #39024, #39363, #35123 ),
 .UNSPECIFIED., .F., .F.,
 ( 4, 2, 2, 2, 2, 2, 2, 2, 2, 2, 2, 4 ),
 ( 0.01118858214005710207, 0.01260300539470554995, 0.01401742864935399957, 0.01543185190400244745, 0.01613906353132666879, 0.01684627515865088840, 0.01826069841329931720, 0.01896791004062353680, 0.01967512166794775641, 0.02108954492259615746, 0.02179675654992035971, 0.02250396817724456891 ),
 .UNSPECIFIED. ) ;
#12332=DIRECTION ( 'NONE',  ( -0.000000000000000000, 1.000000000000000000, -0.000000000000000000 ) ) ;
#12334=DIRECTION ( 'NONE',  ( -0.000000000000000000, 1.000000000000000000, -0.000000000000000000 ) ) ;
#12336=CARTESIAN_POINT ( 'NONE',  ( -145.0695669462244553, 60.50477348111340348, -89.95188078407383614 ) ) ;
#12337=CARTESIAN_POINT ( 'NONE',  ( 126.8015497489690091, 37.32461426945040728, -72.92606890101930617 ) ) ;
#12339=CARTESIAN_POINT ( 'NONE',  ( 86.62931800182293784, -170.0000000000000000, 10.36753698201563267 ) ) ;
#12341=EDGE_LOOP ( 'NONE', ( #58911, #42681, #58237, #62569 ) ) ;
#12343=CARTESIAN_POINT ( 'NONE',  ( -151.6797345123119101, 67.37848486615946797, -35.12068137031451442 ) ) ;
#12345=CARTESIAN_POINT ( 'NONE',  ( -38.93938005333175312, 11.96888249046460828, 37.95614235521382085 ) ) ;
#12346=CARTESIAN_POINT ( 'NONE',  ( -143.2498117110515068, 60.33382252735059126, -19.61078403914306989 ) ) ;
#12351=CARTESIAN_POINT ( 'NONE',  ( -2.172839205444460742, 7.595638683704371452, -21.02768760144151727 ) ) ;
#12353=CARTESIAN_POINT ( 'NONE',  ( 117.3281529665582212, 32.29994712002883972, 12.77937192486413842 ) ) ;
#12356=CARTESIAN_POINT ( 'NONE',  ( -95.20053778133915046, 30.43887292928078026, -45.04236790332991092 ) ) ;
#12359=DIRECTION ( 'NONE',  ( 0.000000000000000000, 0.000000000000000000, 1.000000000000000000 ) ) ;
#12360=CARTESIAN_POINT ( 'NONE',  ( 114.2394011608742517, 31.89382501980991691, 84.44551190695648302 ) ) ;
#12362=DIRECTION ( 'NONE',  ( 0.000000000000000000, 0.000000000000000000, 1.000000000000000000 ) ) ;
#12364=CARTESIAN_POINT ( 'NONE',  ( 8.000000000000007105, 249.8719672152120381, 94.99999999999866418 ) ) ;
#12374=CARTESIAN_POINT ( 'NONE',  ( -166.9992034932274976, 82.01285191063135471, 69.52895971928450081 ) ) ;
#12375=CYLINDRICAL_SURFACE ( 'NONE', #57720, 7.500000000000027534 ) ;
#12376=VECTOR ( 'NONE', #36580, 1000.000000000000000 ) ;
#12379=CARTESIAN_POINT ( 'NONE',  ( 93.43270425363544973, 22.93046121381056324, 7.201044160860008425 ) ) ;
#12380=B_SPLINE_CURVE_WITH_KNOTS ( 'NONE', 3,
 ( #42387, #41363, #35742, #57539, #19907, #20239, #63850, #9696, #15658, #10366, #53267, #62816, #47992, #62466, #51905, #36082, #53617, #6491, #38859, #5778, #15993, #27236, #11395, #43756, #65228, #32520, #864, #17379, #27937, #54302, #38492, #55010, #16687, #64532, #156, #49380, #6832, #16342, #43409, #28285, #49727, #48669, #48323, #21276, #22317, #59579, #21614, #22663 ),
 .UNSPECIFIED., .F., .F.,
 ( 4, 2, 2, 2, 2, 2, 2, 2, 2, 2, 2, 2, 2, 2, 2, 2, 2, 2, 2, 2, 2, 2, 2, 4 ),
 ( 0.000000000000000000, 0.003619254076116254926, 0.004524067595145328524, 0.005428881114174403423, 0.007238508152232576640, 0.008143321671261699243, 0.009048135190290820112, 0.01085776222834899767, 0.01176257574737808557, 0.01266738926640717348, 0.01357220278543626139, 0.01447701630446534930, 0.01538182982349443895, 0.01628664334252354767, 0.01719145686155265640, 0.01809627038058176512, 0.01900108389961087385, 0.01990589741863998258, 0.02171552445669825207, 0.02262033797572739202, 0.02352515149475653197, 0.02533477853281481534, 0.02714440557087309525, 0.02895403260893137515 ),
 .UNSPECIFIED. ) ;
#12381=CARTESIAN_POINT ( 'NONE',  ( 23.28845814680232351, 7.864847136539609096, -43.50557691085024459 ) ) ;
#12384=CARTESIAN_POINT ( 'NONE',  ( 211.1200456646896555, 115.5868795682033152, -13.09781155935739960 ) ) ;
#12385=FACE_BOUND ( 'NONE', #6381, .T. ) ;
#12387=CARTESIAN_POINT ( 'NONE',  ( 160.5018603162735360, 61.33906090758085838, 56.87936049605382038 ) ) ;
#12389=EDGE_CURVE ( 'NONE', #64513, #59450, #34268, .T. ) ;
#12392=CYLINDRICAL_SURFACE ( 'NONE', #22659, 7.500000000000020428 ) ;
#12394=CARTESIAN_POINT ( 'NONE',  ( -173.5372686962700470, 89.10569330281725797, 3.977144016177344366 ) ) ;
#12396=CARTESIAN_POINT ( 'NONE',  ( 209.6698611676811481, 115.2210955123518232, 69.18533967789782935 ) ) ;
#12398=CARTESIAN_POINT ( 'NONE',  ( 84.28078136020374700, 18.63296074526051527, -63.03926293933237446 ) ) ;
#12403=DIRECTION ( 'NONE',  ( -0.000000000000000000, 1.000000000000000000, -0.000000000000000000 ) ) ;
#12405=CARTESIAN_POINT ( 'NONE',  ( -125.8938041572051105, 46.49392987655492959, -49.91370389823397602 ) ) ;
#12411=CARTESIAN_POINT ( 'NONE',  ( 39.40195752203891999, 9.424259417798145577, 71.75838489642698903 ) ) ;
#12413=CARTESIAN_POINT ( 'NONE',  ( 164.8908506817023465, 64.97619709085121542, 38.03401370118700697 ) ) ;
#12417=CARTESIAN_POINT ( 'NONE',  ( 105.2529848321548371, 27.73895015262026220, 4.662269661841498269 ) ) ;
#12421=CARTESIAN_POINT ( 'NONE',  ( -50.52615126106341137, 14.55080735582892792, 4.973081677751911123 ) ) ;
#12422=CARTESIAN_POINT ( 'NONE',  ( -132.8150886319751578, 52.45790550853839562, -18.46974180303275759 ) ) ;
#12423=CARTESIAN_POINT ( 'NONE',  ( -156.1728533452998136, 71.41054633671237184, -92.55438097918974449 ) ) ;
#12425=CARTESIAN_POINT ( 'NONE',  ( 93.98790819024357290, 22.06436042159637267, 92.50594887766449403 ) ) ;
#12427=VERTEX_POINT ( 'NONE', #51135 ) ;
#12434=CARTESIAN_POINT ( 'NONE',  ( -78.66644367742111399, 22.32174330031317311, -35.11545063171788428 ) ) ;
#12435=CARTESIAN_POINT ( 'NONE',  ( -37.39246151129639628, 11.66872370876248688, 69.14885973024283317 ) ) ;
#12437=CARTESIAN_POINT ( 'NONE',  ( -71.41745561414265353, 19.69148172991711832, -67.47099976427212198 ) ) ;
#12438=CARTESIAN_POINT ( 'NONE',  ( -14.94265033805045917, 7.459411036484911328, 35.19966624791602783 ) ) ;
#12439=ORIENTED_EDGE ( 'NONE', *, *, #1437, .T. ) ;
#12443=CARTESIAN_POINT ( 'NONE',  ( -142.0084862216822614, 59.34995487985341356, 11.95469468336700203 ) ) ;
#12444=CARTESIAN_POINT ( 'NONE',  ( 204.6977192012829789, 106.3443248447423599, -51.32593103262161094 ) ) ;
#12445=CARTESIAN_POINT ( 'NONE',  ( -33.97247179057541899, 11.04235163581741119, 84.33913446809840764 ) ) ;
#12447=CARTESIAN_POINT ( 'NONE',  ( 110.7117404013331452, 30.20916032354564607, -24.07788697519003662 ) ) ;
#12448=DIRECTION ( 'NONE',  ( -0.000000000000000000, 1.000000000000000000, -0.000000000000000000 ) ) ;
#12450=CARTESIAN_POINT ( 'NONE',  ( 138.2136629441929188, 45.30947856186674727, -22.80172309817044862 ) ) ;
#12452=EDGE_LOOP ( 'NONE', ( #45552, #44496 ) ) ;
#12457=CARTESIAN_POINT ( 'NONE',  ( 32.29989959354725926, 7.591763852038296179, -67.54129983209111288 ) ) ;
#12460=CARTESIAN_POINT ( 'NONE',  ( 197.2199569260504006, 98.22436319491369261, 64.21605170112221117 ) ) ;
#12462=CARTESIAN_POINT ( 'NONE',  ( -62.49137879463568623, 17.85440472148627933, -68.57102818547264178 ) ) ;
#12464=CARTESIAN_POINT ( 'NONE',  ( -3.255961059272216573, 7.643453059677442596, -36.95062769347506304 ) ) ;
#12466=CARTESIAN_POINT ( 'NONE',  ( -171.0814041607219451, 84.88598211196837440, 4.247423101093799502 ) ) ;
#12468=FACE_BOUND ( 'NONE', #47026, .T. ) ;
#12470=CARTESIAN_POINT ( 'NONE',  ( -189.4409533487738031, 107.3684567050774774, 90.35742019377735801 ) ) ;
#12474=EDGE_LOOP ( 'NONE', ( #65195, #66234 ) ) ;
#12477=CARTESIAN_POINT ( 'NONE',  ( -132.8123438040339863, 51.22132183644642112, -66.35088960131899682 ) ) ;
#12481=CARTESIAN_POINT ( 'NONE',  ( 62.52762183777206673, 13.59210632617624626, -62.56524142263337751 ) ) ;
#12485=CARTESIAN_POINT ( 'NONE',  ( 188.1716167230092367, 86.07821889697497397, 88.01412198095141548 ) ) ;
#12489=CARTESIAN_POINT ( 'NONE',  ( 174.9042454172880809, 72.57746269938728290, -39.44483778160518028 ) ) ;
#12490=CARTESIAN_POINT ( 'NONE',  ( -177.1539090641757923, 91.73101548694630480, -62.71746391358476558 ) ) ;
#12493=CARTESIAN_POINT ( 'NONE',  ( 117.4806398654733925, 33.50379325299403632, 61.92154777411960964 ) ) ;
#12494=CARTESIAN_POINT ( 'NONE',  ( -178.5835577246387800, 93.42126246260829703, 6.332233931154211959 ) ) ;
#12500=CARTESIAN_POINT ( 'NONE',  ( 21.11067624421128386, 6.728538062205546844, -91.35668824920195163 ) ) ;
#12501=CARTESIAN_POINT ( 'NONE',  ( -189.2739965869454863, 107.1373753350176941, 37.54313195747183585 ) ) ;
#12502=EDGE_CURVE ( 'NONE', #42723, #41204, #48536, .T. ) ;
#12504=CARTESIAN_POINT ( 'NONE',  ( -124.9927180788553898, 45.90286323198618135, -8.109744398480245309 ) ) ;
#12505=CARTESIAN_POINT ( 'NONE',  ( -74.79539698934962644, 21.95498232236882075, 4.645315566659635742 ) ) ;
#12506=CARTESIAN_POINT ( 'NONE',  ( -143.2498117110514784, 60.33382252735058415, -46.45533462960677440 ) ) ;
#12507=LINE ( 'NONE', #12163, #5037 ) ;
#12510=CARTESIAN_POINT ( 'NONE',  ( 79.52861599156693728, 17.11914630560288231, -45.78734971095504136 ) ) ;
#12512=CARTESIAN_POINT ( 'NONE',  ( -127.6992109187852265, 47.69334801994796891, 30.82611642083012882 ) ) ;
#12513=CARTESIAN_POINT ( 'NONE',  ( 84.72546926745364715, 19.84015517905188020, 44.48241298831661084 ) ) ;
#12515=CARTESIAN_POINT ( 'NONE',  ( 92.53033045403535084, 22.59263332688195192, 32.55674288556603102 ) ) ;
#12516=CARTESIAN_POINT ( 'NONE',  ( 141.2366329129481244, 46.06278879703611295, -18.04134848091257837 ) ) ;
#12518=CARTESIAN_POINT ( 'NONE',  ( 17.85632111170821190, 7.582480637908914467, -89.48644972445111989 ) ) ;
#12520=ORIENTED_EDGE ( 'NONE', *, *, #12074, .T. ) ;
#12523=CARTESIAN_POINT ( 'NONE',  ( 45.34143264614441904, 9.256465810451196319, 32.82761261990431478 ) ) ;
#12524=CARTESIAN_POINT ( 'NONE',  ( 199.3743599161302882, 99.31857334527873604, -11.67350270838394266 ) ) ;
#12527=CARTESIAN_POINT ( 'NONE',  ( 206.2957331585308793, 110.2946564621822887, -51.19906654808809066 ) ) ;
#12529=CARTESIAN_POINT ( 'NONE',  ( -73.80418150970714919, 21.59712875466424364, -75.19184975933067960 ) ) ;
#12531=CARTESIAN_POINT ( 'NONE',  ( -24.94151142167918067, 8.614613465433007988, -46.59531917729278661 ) ) ;
#12532=CARTESIAN_POINT ( 'NONE',  ( 164.3577270662354977, 63.21061577643038731, -73.44943585255833796 ) ) ;
#12535=ORIENTED_EDGE ( 'NONE', *, *, #45821, .T. ) ;
#12538=DIRECTION ( 'NONE',  ( -0.000000000000000000, 1.000000000000000000, -0.000000000000000000 ) ) ;
#12541=CARTESIAN_POINT ( 'NONE',  ( -80.54757501605355685, 23.04700348514568020, 72.02692194415921279 ) ) ;
#12542=CARTESIAN_POINT ( 'NONE',  ( 130.7260570116703775, 40.73146260246711847, 43.84148412689328467 ) ) ;
#12546=CARTESIAN_POINT ( 'NONE',  ( -99.10904156412046007, 32.31949011661293270, -8.856797566735396643 ) ) ;
#12547=CARTESIAN_POINT ( 'NONE',  ( 56.52885800925552218, 12.28784885070978561, 33.51606380828312126 ) ) ;
#12548=CARTESIAN_POINT ( 'NONE',  ( 32.21680480348707221, 7.583440910203144369, 88.92743217354535545 ) ) ;
#12550=EDGE_LOOP ( 'NONE', ( #41664, #54442 ) ) ;
#12553=CARTESIAN_POINT ( 'NONE',  ( -189.7334103489410211, 107.7745063523401114, -44.80734569376801346 ) ) ;
#12556=CARTESIAN_POINT ( 'NONE',  ( -109.7290872258106731, 36.72869630780158445, -70.37839858795491921 ) ) ;
#12557=CARTESIAN_POINT ( 'NONE',  ( 128.4157044224114657, 39.39296260757096491, -21.86358749922995059 ) ) ;
#12559=EDGE_CURVE ( 'NONE', #43039, #22496, #1991, .T. ) ;
#12564=CARTESIAN_POINT ( 'NONE',  ( -166.3231866619663890, 81.31146386205591625, -39.03154315301186017 ) ) ;
#12568=CARTESIAN_POINT ( 'NONE',  ( -118.4063383664800000, 41.75753822095644097, -41.90331656875046917 ) ) ;
#12571=CARTESIAN_POINT ( 'NONE',  ( -7.825402957745081878, 7.899365992529270741, -77.26262132240753999 ) ) ;
#12576=CARTESIAN_POINT ( 'NONE',  ( 162.8616317072115578, 63.27292930957019479, -92.08433922111466075 ) ) ;
#12577=CARTESIAN_POINT ( 'NONE',  ( 201.9777685760379313, 102.6876480786893069, -50.82744265795196981 ) ) ;
#12585=CARTESIAN_POINT ( 'NONE',  ( 60.40277045393653310, 12.08176563382369828, 44.34733751979118210 ) ) ;
#12587=AXIS2_PLACEMENT_3D ( 'NONE', #19788, #37331, #68992 ) ;
#12590=CARTESIAN_POINT ( 'NONE',  ( -74.17694007417657076, 20.66176641130876845, -9.743324496515986866 ) ) ;
#12591=CARTESIAN_POINT ( 'NONE',  ( -36.80719415492644941, 11.55793080356381175, -91.25128724788480383 ) ) ;
#12592=CARTESIAN_POINT ( 'NONE',  ( -10.23531775138760835, 8.068923942586302189, -76.86913210980220867 ) ) ;
#12594=CARTESIAN_POINT ( 'NONE',  ( -95.31607127852431915, 30.49332874523306458, 88.90476004080002781 ) ) ;
#12596=CARTESIAN_POINT ( 'NONE',  ( -28.13128612339710344, 10.08889185338653327, 44.46541057415654308 ) ) ;
#12599=CARTESIAN_POINT ( 'NONE',  ( 207.4566510040494904, 111.9649643341356438, -77.64771060859440865 ) ) ;
#12601=CARTESIAN_POINT ( 'NONE',  ( -175.1968289912784371, 90.99944698359489337, 45.54112020630180524 ) ) ;
#12602=CARTESIAN_POINT ( 'NONE',  ( -132.8257891167039020, 52.46553896898735303, 14.15040099157313236 ) ) ;
#12603=CARTESIAN_POINT ( 'NONE',  ( 16.77480716385437987, 7.540753720029939267, 56.90830145484930114 ) ) ;
#12608=CARTESIAN_POINT ( 'NONE',  ( -107.0809603157386363, 36.42942792191065138, 16.95719255189394303 ) ) ;
#12610=CARTESIAN_POINT ( 'NONE',  ( -36.37371824399145481, 10.45334302951138739, -48.48679871522361395 ) ) ;
#12611=CARTESIAN_POINT ( 'NONE',  ( -105.2142611701586503, 34.29582324647149250, 84.77962915760878104 ) ) ;
#12615=CARTESIAN_POINT ( 'NONE',  ( -75.00636493611885669, 22.03142602679956497, -9.206886202885991466 ) ) ;
#12618=CARTESIAN_POINT ( 'NONE',  ( 82.34195123877069022, 18.00239921638039320, 70.21512810070214528 ) ) ;
#12620=CARTESIAN_POINT ( 'NONE',  ( 32.15641333221390141, 7.577415570152253643, 39.36641614295111680 ) ) ;
#12623=CARTESIAN_POINT ( 'NONE',  ( 181.9406741394861342, 79.47484497224790800, 44.27164137268504618 ) ) ;
#12626=CARTESIAN_POINT ( 'NONE',  ( -120.6420427933462207, 44.31795133507805673, 59.60453931232847680 ) ) ;
#12627=EDGE_CURVE ( 'NONE', #68773, #3776, #58768, .T. ) ;
#12628=CARTESIAN_POINT ( 'NONE',  ( -51.99406906667274342, 13.88268392809765572, 17.82498527766545848 ) ) ;
#12631=CARTESIAN_POINT ( 'NONE',  ( 162.8034185388970627, 63.22443559329411755, -75.76383047087158218 ) ) ;
#12633=CARTESIAN_POINT ( 'NONE',  ( -173.1211646369891355, 88.63826465341151106, 30.82169460664101734 ) ) ;
#12634=CARTESIAN_POINT ( 'NONE',  ( -154.7934364910360330, 68.79594655117534785, -10.14203366738286860 ) ) ;
#12640=CARTESIAN_POINT ( 'NONE',  ( -84.22570405563701001, 24.51726571826274537, 42.97634706641604652 ) ) ;
#12641=CARTESIAN_POINT ( 'NONE',  ( 150.2060369882285329, 53.45752899907539302, -68.58311478360899116 ) ) ;
#12642=CARTESIAN_POINT ( 'NONE',  ( 42.48820792780864508, 9.847387255477762835, 30.57387150330147563 ) ) ;
#12644=CARTESIAN_POINT ( 'NONE',  ( 139.6203063421346826, 45.01495791936837065, -48.34818717462631099 ) ) ;
#12651=CARTESIAN_POINT ( 'NONE',  ( 133.8566784816069344, -170.0000000000000000, -16.67876034193198365 ) ) ;
#12654=CARTESIAN_POINT ( 'NONE',  ( -1.095583923122883663, 7.553030873957007785, 67.77975244133044441 ) ) ;
#12655=DIRECTION ( 'NONE',  ( 0.000000000000000000, 0.000000000000000000, 1.000000000000000000 ) ) ;
#12657=ORIENTED_EDGE ( 'NONE', *, *, #52712, .F. ) ;
#12660=CARTESIAN_POINT ( 'NONE',  ( 161.7048274740120917, 61.01946783654760509, -22.98727189428458573 ) ) ;
#12663=CARTESIAN_POINT ( 'NONE',  ( 140.2332932573541484, 45.41010019581508317, -66.38781847616553478 ) ) ;
#12665=ORIENTED_EDGE ( 'NONE', *, *, #3026, .T. ) ;
#12666=DIRECTION ( 'NONE',  ( -0.000000000000000000, 1.000000000000000000, -0.000000000000000000 ) ) ;
#12667=CARTESIAN_POINT ( 'NONE',  ( 13.37820144534468803, 6.435512790162280616, 44.62119266632897308 ) ) ;
#12668=ORIENTED_EDGE ( 'NONE', *, *, #36855, .T. ) ;
#12669=CARTESIAN_POINT ( 'NONE',  ( -62.45176220516619736, 16.79101814080731714, -68.30864959305280593 ) ) ;
#12670=CARTESIAN_POINT ( 'NONE',  ( 131.2736393829322878, 39.88634239355057076, -90.16109689038154329 ) ) ;
#12673=CARTESIAN_POINT ( 'NONE',  ( -125.8938041572051389, 47.69968343338778283, 3.775397282693376155 ) ) ;
#12680=CARTESIAN_POINT ( 'NONE',  ( 70.21232668545647471, 15.49872527826561885, 88.86438496759851091 ) ) ;
#12681=CARTESIAN_POINT ( 'NONE',  ( 37.70910994512001935, 9.209110272746713122, 30.10326457111060705 ) ) ;
#12682=CARTESIAN_POINT ( 'NONE',  ( -180.5801285865472039, 97.42945596116099694, -43.01106670952992062 ) ) ;
#12683=CARTESIAN_POINT ( 'NONE',  ( -133.3958821919892728, 51.63629593114587379, -16.08335082672273231 ) ) ;
#12685=CARTESIAN_POINT ( 'NONE',  ( 153.8366942494331226, 54.87992279068316748, 70.31910049688980280 ) ) ;
#12686=CARTESIAN_POINT ( 'NONE',  ( 128.3856248084844083, 38.21741401878864508, -75.52143459682376658 ) ) ;
#12688=ORIENTED_EDGE ( 'NONE', *, *, #16764, .F. ) ;
#12689=CARTESIAN_POINT ( 'NONE',  ( 140.5958192060901411, 46.84598876498521491, -73.66959190929182455 ) ) ;
#12690=DIRECTION ( 'NONE',  ( -0.000000000000000000, 1.000000000000000000, -0.000000000000000000 ) ) ;
#12693=CARTESIAN_POINT ( 'NONE',  ( -156.4797890011541597, 71.69341087347112307, -45.08998991706700110 ) ) ;
#12694=CARTESIAN_POINT ( 'NONE',  ( 207.4610690199662315, 111.9701171077052209, -9.997192138305063480 ) ) ;
#12695=CARTESIAN_POINT ( 'NONE',  ( -38.87871322265798568, 11.95691939779334945, 38.69778012508339060 ) ) ;
#12696=CARTESIAN_POINT ( 'NONE',  ( -169.8842709557924877, 83.59602878049474839, -48.99215875544830112 ) ) ;
#12697=DIRECTION ( 'NONE',  ( -0.000000000000000000, 1.000000000000000000, -0.000000000000000000 ) ) ;
#12699=CARTESIAN_POINT ( 'NONE',  ( -48.99162761293256096, 13.13973062091724131, -73.98514508948782975 ) ) ;
#12700=CARTESIAN_POINT ( 'NONE',  ( 204.6977192012829789, 106.3443248447423599, -51.32593103262161094 ) ) ;
#12702=CARTESIAN_POINT ( 'NONE',  ( -14.33060720034884028, 8.412649192293189415, 33.85085847379210833 ) ) ;
#12703=CARTESIAN_POINT ( 'NONE',  ( 115.0692128464502417, 31.17922615202198600, 16.02821217000574094 ) ) ;
#12710=CARTESIAN_POINT ( 'NONE',  ( 82.73618382051373032, 19.18661415186666730, -63.75104638294856585 ) ) ;
#12711=CARTESIAN_POINT ( 'NONE',  ( 44.35071890818839790, 9.104600422692275430, 69.91515779349310833 ) ) ;
#12714=CARTESIAN_POINT ( 'NONE',  ( -125.8938041572051389, -170.0000000000000000, -42.41370389823394760 ) ) ;
#12720=CARTESIAN_POINT ( 'NONE',  ( 46.68054346512387554, 9.468156054376091646, -95.00000000000133582 ) ) ;
#12721=CARTESIAN_POINT ( 'NONE',  ( 173.6710158776850506, 71.42507420636735560, 62.47632899483146218 ) ) ;
#12725=CARTESIAN_POINT ( 'NONE',  ( -173.1211646369891355, 88.63826465341151106, -22.86740657428632773 ) ) ;
#12730=CARTESIAN_POINT ( 'NONE',  ( 103.5589117581614715, 27.00490790413960340, -39.98222358844557078 ) ) ;
#12732=CARTESIAN_POINT ( 'NONE',  ( 12.47451846520756646, 7.423604437114563304, 57.62656840523505508 ) ) ;
#12733=B_SPLINE_CURVE_WITH_KNOTS ( 'NONE', 3,
 ( #61746, #46610, #19889, #51210, #41348, #14604, #36066, #45227, #3022, #39955, #24132, #61411, #18852, #57523, #45927, #34695, #9329, #56836, #56130, #7948, #45574, #67056, #40637, #62097, #15643, #59228, #57865, #69090, #37783, #26546, #64518, #11047, #142, #52237, #9682, #31819, #37430, #15302, #32171, #48309, #53250, #5080, #31147, #4060 ),
 .UNSPECIFIED., .F., .F.,
 ( 4, 2, 2, 2, 2, 2, 2, 2, 2, 2, 2, 2, 2, 2, 2, 2, 2, 2, 2, 2, 2, 4 ),
 ( 0.02814986980477068509, 0.02995274102020801035, 0.03085417662792665563, 0.03175561223564530439, 0.03355848345108267822, 0.03536135466652005899, 0.03716422588195743976, 0.03896709709739482053, 0.03986853270511350744, 0.04076996831283219436, 0.04167140392055088821, 0.04257283952826957513, 0.04347427513598826204, 0.04437571074370695590, 0.04527714635142564281, 0.04617858195914432973, 0.04798145317458171744, 0.04978432439001911902, 0.05158719560545652061, 0.05339006682089390832, 0.05519293803633130990, 0.05699580925176869761 ),
 .UNSPECIFIED. ) ;
#12735=CARTESIAN_POINT ( 'NONE',  ( -55.05276343752910151, -170.0000000000000000, 18.47277718246750311 ) ) ;
#12736=FACE_BOUND ( 'NONE', #67574, .T. ) ;
#12737=AXIS2_PLACEMENT_3D ( 'NONE', #58509, #15273, #6084 ) ;
#12740=ORIENTED_EDGE ( 'NONE', *, *, #33364, .F. ) ;
#12744=CARTESIAN_POINT ( 'NONE',  ( 31.96192885395476324, 8.569232728322415227, -68.98636584908359737 ) ) ;
#12746=CARTESIAN_POINT ( 'NONE',  ( 207.2640160519426615, 111.6867652229576464, 56.50203771818474507 ) ) ;
#12747=CARTESIAN_POINT ( 'NONE',  ( -149.5074843970971301, -170.0000000000000000, -22.96827994102829962 ) ) ;
#12749=CARTESIAN_POINT ( 'NONE',  ( 59.29615173875417611, 11.84060224810188089, 3.951100658409211430 ) ) ;
#12750=CARTESIAN_POINT ( 'NONE',  ( 201.5876148766342624, 103.8397408698165236, -36.98778679194309404 ) ) ;
#12751=ORIENTED_EDGE ( 'NONE', *, *, #54559, .F. ) ;
#12757=CARTESIAN_POINT ( 'NONE',  ( 87.59078297315399197, 20.81577753000344799, -77.61960893227724512 ) ) ;
#12760=CARTESIAN_POINT ( 'NONE',  ( 43.96062659677686213, 10.06332325923986026, 70.23394607708451076 ) ) ;
#12761=CARTESIAN_POINT ( 'NONE',  ( 164.9700808964341547, 65.04346068891115351, 37.19820718134189264 ) ) ;
#12762=CARTESIAN_POINT ( 'NONE',  ( -156.8773151811563480, 72.06122063279303802, -67.73783947574408160 ) ) ;
#12763=CARTESIAN_POINT ( 'NONE',  ( 63.99027454648603452, 13.93445177372599098, 3.016241708314831627 ) ) ;
#12764=CARTESIAN_POINT ( 'NONE',  ( 153.2523375521184050, 55.69936538551846184, 3.858872989883677107 ) ) ;
#12765=VERTEX_POINT ( 'NONE', #64057 ) ;
#12768=CARTESIAN_POINT ( 'NONE',  ( 62.04382205963242569, 13.48099884269680082, -35.76789042656609752 ) ) ;
#12770=CARTESIAN_POINT ( 'NONE',  ( -132.5976199670998597, 52.30296609017644016, -18.94205205907401179 ) ) ;
#12772=CARTESIAN_POINT ( 'NONE',  ( 117.3281529665582070, 32.29994712002883972, -14.06517866559955010 ) ) ;
#12773=CARTESIAN_POINT ( 'NONE',  ( 94.05139011108599334, 22.08843705196240137, 89.76976943065523074 ) ) ;
#12774=DIRECTION ( 'NONE',  ( -0.000000000000000000, 1.000000000000000000, -0.000000000000000000 ) ) ;
#12779=CARTESIAN_POINT ( 'NONE',  ( 43.97326221476412655, 9.047815246749991047, 16.53542767223330046 ) ) ;
#12780=CARTESIAN_POINT ( 'NONE',  ( -178.6094373798883623, 95.02303223604788229, 86.89060986716357604 ) ) ;
#12782=CARTESIAN_POINT ( 'NONE',  ( 103.5588133492864671, 25.91050225236393345, -20.01717663906335787 ) ) ;
#12783=CARTESIAN_POINT ( 'NONE',  ( 197.6145711261845292, 97.10888456119687362, 7.316670231408826552 ) ) ;
#12786=CARTESIAN_POINT ( 'NONE',  ( 211.3754067703094108, 117.8127004712419819, 93.81656004356196377 ) ) ;
#12789=DIRECTION ( 'NONE',  ( -0.000000000000000000, 1.000000000000000000, -0.000000000000000000 ) ) ;
#12790=CARTESIAN_POINT ( 'NONE',  ( -75.43953471070999228, 21.11829282998124668, -76.24709388609002758 ) ) ;
#12791=CARTESIAN_POINT ( 'NONE',  ( -12.78015296493258290, 7.264294661536300879, 43.26710858275960447 ) ) ;
#12792=ORIENTED_EDGE ( 'NONE', *, *, #35023, .F. ) ;
#12794=CARTESIAN_POINT ( 'NONE',  ( 86.62931800182293784, 20.48449268398423584, -35.82156419891171595 ) ) ;
#12795=VERTEX_POINT ( 'NONE', #43629 ) ;
#12797=CARTESIAN_POINT ( 'NONE',  ( 63.01563776193091826, 13.70579113808095073, -23.87614024170608218 ) ) ;
#12798=CARTESIAN_POINT ( 'NONE',  ( 183.9887307715837039, 83.05100282186909055, -63.65145494335473586 ) ) ;
#12800=CARTESIAN_POINT ( 'NONE',  ( -167.1619226259399227, 82.18315278115417755, 33.76076489396710656 ) ) ;
#12802=CARTESIAN_POINT ( 'NONE',  ( 117.3246714514015849, 33.42485879931864190, -19.09944304000492821 ) ) ;
#12805=CARTESIAN_POINT ( 'NONE',  ( 139.3041645503688528, 46.00819478311336042, -21.83978754804469702 ) ) ;
#12806=ORIENTED_EDGE ( 'NONE', *, *, #36825, .F. ) ;
#12812=CARTESIAN_POINT ( 'NONE',  ( 62.04326772936978784, 12.44884401098615179, -23.82859654250995973 ) ) ;
#12814=B_SPLINE_CURVE_WITH_KNOTS ( 'NONE', 3,
 ( #26343, #68883, #31281, #16469, #4199, #26001, #68558, #15778, #5561, #37577, #47778, #64661, #15445, #37224, #10492, #31964, #59024, #53390, #10840, #9475, #30935, #25663, #47096, #20361, #41828, #63284, #15096, #36552, #58004, #9823, #52707, #47428, #42168, #46716, #19286, #41449, #51994, #40744, #8402, #57281, #56231, #62902, #30543, #46024, #56938, #61517, #51657 ),
 .UNSPECIFIED., .F., .F.,
 ( 4, 2, 2, 2, 2, 2, 2, 2, 2, 2, 2, 2, 1, 2, 2, 2, 2, 2, 2, 2, 2, 2, 2, 4 ),
 ( 0.000000000000000000, 0.001493793014771570673, 0.002240689522157353081, 0.002987586029543135707, 0.004481379044314673203, 0.005228275551700448456, 0.005975172059086222842, 0.007468965073857801971, 0.008215861581243587633, 0.008962758088629372427, 0.01045655110340091946, 0.01120344761078670252, 0.01195034411817248732, 0.01269724062555827211, 0.01344413713294406211, 0.01493793014771565252, 0.01568482665510143731, 0.01643172316248721690, 0.01792551617725878302, 0.01941930919203034914, 0.02016620569941613914, 0.02091310220680193260, 0.02240689522157351954, 0.02390068823634510300 ),
 .UNSPECIFIED. ) ;
#12822=CARTESIAN_POINT ( 'NONE',  ( -62.29496909743952671, 17.79481128341706153, -67.59550361844860333 ) ) ;
#12823=CARTESIAN_POINT ( 'NONE',  ( 180.2473887773228114, 77.76029175826236894, -63.06960825634326540 ) ) ;
#12824=CARTESIAN_POINT ( 'NONE',  ( -173.1211646369891071, 87.12891641440859303, -34.71195716474998960 ) ) ;
#12826=CARTESIAN_POINT ( 'NONE',  ( -171.4867114763003997, 85.32693843184996751, 4.145646873760804318 ) ) ;
#12828=FACE_BOUND ( 'NONE', #48721, .T. ) ;
#12829=CARTESIAN_POINT ( 'NONE',  ( -189.2550107216115407, 107.1111757360096703, 92.75985481009226419 ) ) ;
#12831=CARTESIAN_POINT ( 'NONE',  ( -6.126800896373023164, 6.786243985899684361, 57.15086958430494235 ) ) ;
#12832=ORIENTED_EDGE ( 'NONE', *, *, #2302, .F. ) ;
#12833=AXIS2_PLACEMENT_3D ( 'NONE', #23455, #44893, #66375 ) ;
#12836=CARTESIAN_POINT ( 'NONE',  ( 39.40195752203892710, -170.0000000000000000, -69.96436805589145536 ) ) ;
#12844=LINE ( 'NONE', #44121, #37169 ) ;
#12849=CARTESIAN_POINT ( 'NONE',  ( -180.3153482337534967, 95.51031295027651424, -66.91522547114587383 ) ) ;
#12854=CARTESIAN_POINT ( 'NONE',  ( -1.319107422865895218, 6.554467368239826008, 7.008176618785499912 ) ) ;
#12855=CARTESIAN_POINT ( 'NONE',  ( -79.61235761536670452, 23.76245710489568452, 30.46282415610054883 ) ) ;
#12856=CARTESIAN_POINT ( 'NONE',  ( 88.99522780200241812, 20.24180937454204354, -36.20046504712779267 ) ) ;
#12857=CARTESIAN_POINT ( 'NONE',  ( -47.94536219817735656, 13.92422159065987231, -18.31751929704889292 ) ) ;
#12859=B_SPLINE_CURVE_WITH_KNOTS ( 'NONE', 3,
 ( #27715, #12248, #11188, #49157, #996, #43883, #65369, #17152, #38625, #2051, #23852, #45290, #50228, #13978, #12954, #23504, #44946, #35439, #56899, #29121, #40364, #66430, #34414, #8366, #24551, #18221, #61810, #24888, #50921, #29814, #39671, #61479, #29463, #8715, #56191, #56539, #50572, #51276, #30167, #13300, #55859, #13628, #3088, #45987, #61126 ),
 .UNSPECIFIED., .F., .F.,
 ( 4, 2, 2, 2, 2, 2, 2, 2, 2, 2, 2, 1, 2, 2, 2, 2, 2, 2, 2, 2, 2, 2, 4 ),
 ( 0.000000000000000000, 0.001512548138464682489, 0.002268822207697023842, 0.003025096276929364978, 0.004537644415394018194, 0.005293918484626360631, 0.006050192553858702200, 0.007562740692323368860, 0.009075288830788036387, 0.01058783696925270565, 0.01134411103848502814, 0.01210038510771735236, 0.01285665917694967832, 0.01361293324618200427, 0.01512548138464661976, 0.01588175545387892837, 0.01663802952311124045, 0.01815057766157585767, 0.01966312580004047836, 0.02041939986927279044, 0.02117567393850510599, 0.02268822207696976137, 0.02420077021543442022 ),
 .UNSPECIFIED. ) ;
#12860=ORIENTED_EDGE ( 'NONE', *, *, #50914, .T. ) ;
#12861=CARTESIAN_POINT ( 'NONE',  ( 116.1021807117071774, 31.68810634233423684, -38.71412669113463068 ) ) ;
#12863=CARTESIAN_POINT ( 'NONE',  ( -71.27103490383370854, 20.70545763375145398, 12.34733277340642665 ) ) ;
#12864=CARTESIAN_POINT ( 'NONE',  ( 43.97326221476411945, 9.047815246749959073, -37.15367350869404817 ) ) ;
#12866=CARTESIAN_POINT ( 'NONE',  ( -125.3944660332519447, 46.16494358222053762, 84.30437107587852097 ) ) ;
#12868=CARTESIAN_POINT ( 'NONE',  ( 85.67452303415196013, 19.09699411916382772, -35.86737280937732208 ) ) ;
#12870=CARTESIAN_POINT ( 'NONE',  ( -147.7845268487069461, 62.73119438705056439, 72.37768481507308138 ) ) ;
#12871=CARTESIAN_POINT ( 'NONE',  ( 81.04027388895738682, 18.64386073872847760, 42.23734901537720532 ) ) ;
#12873=EDGE_CURVE ( 'NONE', #67246, #34459, #3595, .T. ) ;
#12876=CARTESIAN_POINT ( 'NONE',  ( 139.1353280997809634, 44.70436000187870462, -11.34540700426408932 ) ) ;
#12878=CARTESIAN_POINT ( 'NONE',  ( -179.8989115484066872, 96.59045402602909292, -12.14446317899465733 ) ) ;
#12882=ORIENTED_EDGE ( 'NONE', *, *, #3026, .F. ) ;
#12887=CARTESIAN_POINT ( 'NONE',  ( 207.4610690199661747, 111.9701171077051924, -36.84174272876874312 ) ) ;
#12889=CARTESIAN_POINT ( 'NONE',  ( -108.0980548770427987, 35.83569586822709141, 69.62243089452121581 ) ) ;
#12891=CARTESIAN_POINT ( 'NONE',  ( -28.35330809568270638, 9.105138953156432180, -35.97708236689904027 ) ) ;
#12899=CARTESIAN_POINT ( 'NONE',  ( -75.69395121710529395, 21.21099447234451318, 84.69349098787803598 ) ) ;
#12904=CARTESIAN_POINT ( 'NONE',  ( -99.10674985723794350, 32.31836975419499680, -22.48196502616453785 ) ) ;
#12907=EDGE_CURVE ( 'NONE', #66812, #69029, #47186, .T. ) ;
#12908=CARTESIAN_POINT ( 'NONE',  ( 55.77012379229940819, 12.13428856597100669, 39.26591085917196011 ) ) ;
#12909=CARTESIAN_POINT ( 'NONE',  ( 40.06683191176360737, 8.496734820196639504, 83.62526394863175483 ) ) ;
#12913=LINE ( 'NONE', #62114, #64422 ) ;
#12914=CARTESIAN_POINT ( 'NONE',  ( -14.56151485655250255, 8.434196591921333308, 7.436944112387903871 ) ) ;
#12915=EDGE_CURVE ( 'NONE', #52201, #3613, #58891, .T. ) ;
#12917=CARTESIAN_POINT ( 'NONE',  ( -103.2169245450825343, 33.25885825286820108, -76.81501985536182531 ) ) ;
#12918=CARTESIAN_POINT ( 'NONE',  ( 132.0563630623056781, 41.51825634609595284, -23.96314219444095883 ) ) ;
#12919=EDGE_LOOP ( 'NONE', ( #14814, #33641, #50662, #31863 ) ) ;
#12925=CARTESIAN_POINT ( 'NONE',  ( -166.1340766777337024, 79.67347379767349480, 89.26157043849886463 ) ) ;
#12927=CARTESIAN_POINT ( 'NONE',  ( -120.1259246007803227, 42.81147313035988589, -37.59277727144264958 ) ) ;
#12928=CARTESIAN_POINT ( 'NONE',  ( -142.0251973982165623, 58.08401473564116202, -16.05535940763569158 ) ) ;
#12929=CARTESIAN_POINT ( 'NONE',  ( -0.7076388175553578463, 7.538734751903871434, -72.17698391732507446 ) ) ;
#12933=CARTESIAN_POINT ( 'NONE',  ( -56.72676045871359918, 16.18052435693490665, 3.657967166041028229 ) ) ;
#12937=CARTESIAN_POINT ( 'NONE',  ( 23.23895241123075905, 6.853530908437206470, -44.00714248153148134 ) ) ;
#12939=CARTESIAN_POINT ( 'NONE',  ( -56.97107423601132581, 15.20373812575555839, 3.706198643034869011 ) ) ;
#12944=VERTEX_POINT ( 'NONE', #35874 ) ;
#12949=CARTESIAN_POINT ( 'NONE',  ( -34.73299709025328497, 11.17736532835359320, -89.76496422446544443 ) ) ;
#12950=DIRECTION ( 'NONE',  ( 1.000000000000000000, 0.000000000000000000, -0.000000000000000000 ) ) ;
#12953=CARTESIAN_POINT ( 'NONE',  ( -30.94745021534355800, 10.53010394565407282, 45.21645440618919309 ) ) ;
#12954=CARTESIAN_POINT ( 'NONE',  ( -72.78270026377323632, 21.23376443558121451, -37.93819681164344360 ) ) ;
#12956=CARTESIAN_POINT ( 'NONE',  ( 211.8345664497466316, 118.5225165986914391, -72.99828217273564235 ) ) ;
#12958=FACE_OUTER_BOUND ( 'NONE', #68382, .T. ) ;
#12959=CARTESIAN_POINT ( 'NONE',  ( -173.1211646369891355, 88.63826465341152527, 45.82169460664104577 ) ) ;
#12960=DIRECTION ( 'NONE',  ( 0.000000000000000000, 0.000000000000000000, 1.000000000000000000 ) ) ;
#12962=CARTESIAN_POINT ( 'NONE',  ( 17.48988570800758424, 7.568061572928495906, 71.66776098152827501 ) ) ;
#12967=CARTESIAN_POINT ( 'NONE',  ( 210.6484376398113625, 114.8762597311295366, -92.94483523309006046 ) ) ;
#12968=CARTESIAN_POINT ( 'NONE',  ( -32.41982179707236611, 9.753975577087194537, -50.26874347964162837 ) ) ;
#12970=CARTESIAN_POINT ( 'NONE',  ( -142.6264002846223775, 58.55577336362199503, 35.22544109792448097 ) ) ;
#12974=CARTESIAN_POINT ( 'NONE',  ( 84.05098130332766004, 18.55728792516086756, 71.10367255945043041 ) ) ;
#12977=CARTESIAN_POINT ( 'NONE',  ( 32.29989959354726636, 7.591763852038292626, 39.83690252976357726 ) ) ;
#12982=CARTESIAN_POINT ( 'NONE',  ( -119.1605144823340083, 43.39823405392971267, 61.65073838172952492 ) ) ;
#12983=CARTESIAN_POINT ( 'NONE',  ( -47.55360235114365963, 12.79819361309566617, 10.46016547731527702 ) ) ;
#12985=ADVANCED_FACE ( 'NONE', ( #4548 ), #9490, .F. ) ;
#12986=VECTOR ( 'NONE', #17139, 1000.000000000000000 ) ;
#12988=AXIS2_PLACEMENT_3D ( 'NONE', #28204, #55634, #23640 ) ;
#12989=ORIENTED_EDGE ( 'NONE', *, *, #36999, .T. ) ;
#12991=CARTESIAN_POINT ( 'NONE',  ( -155.2912910578197057, 69.24479901948497229, -10.68701328854503174 ) ) ;
#12995=CARTESIAN_POINT ( 'NONE',  ( -60.98168946575805904, 17.40090852531919552, 69.28151032968872869 ) ) ;
#12997=EDGE_CURVE ( 'NONE', #10658, #4373, #11055, .T. ) ;
#12998=VERTEX_POINT ( 'NONE', #43197 ) ;
#13001=CARTESIAN_POINT ( 'NONE',  ( -12.78015296493257402, 7.264294661536300879, -64.11109377909512830 ) ) ;
#13002=CARTESIAN_POINT ( 'NONE',  ( -38.16002576456689610, 10.79155573432543491, 34.37876793671505737 ) ) ;
#13003=CARTESIAN_POINT ( 'NONE',  ( -27.70005010046228833, 9.007417901453017350, 71.06713019032800105 ) ) ;
#13007=( NAMED_UNIT ( * ) SI_UNIT ( $, .STERADIAN. ) SOLID_ANGLE_UNIT ( ) );
#13008=CARTESIAN_POINT ( 'NONE',  ( -118.3927673406137302, 41.74929850983304647, 38.35786790901878618 ) ) ;
#13010=CYLINDRICAL_SURFACE ( 'NONE', #17739, 7.500000000000013323 ) ;
#13012=CARTESIAN_POINT ( 'NONE',  ( -4.071369321747701164, 7.682719369516283869, 17.28235958677781525 ) ) ;
#13013=CARTESIAN_POINT ( 'NONE',  ( 88.52345267551653762, 20.07594890262052800, 56.79578933626290649 ) ) ;
#13018=CARTESIAN_POINT ( 'NONE',  ( 164.9534461562627143, 63.71129898458563190, -17.35706065313273783 ) ) ;
#13020=CARTESIAN_POINT ( 'NONE',  ( 65.62848231372477414, 13.29388722724787719, 57.12320672528056775 ) ) ;
#13021=CARTESIAN_POINT ( 'NONE',  ( -126.3063800003736077, 47.97292241606065488, -88.60280507916129977 ) ) ;
#13025=EDGE_CURVE ( 'NONE', #60434, #18072, #48054, .T. ) ;
#13026=CARTESIAN_POINT ( 'NONE',  ( 157.4703587214989113, 58.92748579479260229, -9.279633708673953763 ) ) ;
#13030=CARTESIAN_POINT ( 'NONE',  ( -60.65612136648954333, 16.25551606627059087, -64.55169377915926532 ) ) ;
#13031=ADVANCED_FACE ( 'NONE', ( #56198 ), #1348, .F. ) ;
#13033=CIRCLE ( 'NONE', #63580, 242.4895526022646379 ) ;
#13035=CARTESIAN_POINT ( 'NONE',  ( -142.9730935922299579, 58.82921737386681826, -65.46680488933378683 ) ) ;
#13036=CARTESIAN_POINT ( 'NONE',  ( 87.11228333101215071, 19.58587579906928866, 17.86753698201565399 ) ) ;
#13039=ORIENTED_EDGE ( 'NONE', *, *, #35506, .T. ) ;
#13041=CARTESIAN_POINT ( 'NONE',  ( -98.68609963468202295, 32.11186931716881787, 17.77450552764720371 ) ) ;
#13042=CARTESIAN_POINT ( 'NONE',  ( 69.71545454699229083, 15.36735235725339699, 87.61477549632385831 ) ) ;
#13043=CARTESIAN_POINT ( 'NONE',  ( 32.66364305947234925, 8.639871491745262588, 40.74384643876327772 ) ) ;
#13044=AXIS2_PLACEMENT_3D ( 'NONE', #38825, #34938, #28253 ) ;
#13045=CARTESIAN_POINT ( 'NONE',  ( 81.76212856587196143, 18.87332718082996408, -22.18841434000387025 ) ) ;
#13046=CARTESIAN_POINT ( 'NONE',  ( 110.2429982417149574, -170.0000000000000000, 2.766663615273646126 ) ) ;
#13047=CARTESIAN_POINT ( 'NONE',  ( 151.7956716830626362, 53.36999433148316285, 68.66416584447760840 ) ) ;
#13048=EDGE_CURVE ( 'NONE', #67011, #5837, #34760, .T. ) ;
#13052=CARTESIAN_POINT ( 'NONE',  ( -11.13714165684777768, 8.138643170880696331, 57.72645611657431886 ) ) ;
#13055=CARTESIAN_POINT ( 'NONE',  ( -149.5074843970970733, 65.50121172469319220, -34.81283053149196149 ) ) ;
#13057=CARTESIAN_POINT ( 'NONE',  ( -1.455067768715155863, 7.566780179921178906, 41.58164679007672504 ) ) ;
#13058=CARTESIAN_POINT ( 'NONE',  ( -13.97522410592632625, 7.369766281240364592, -92.29298810122654118 ) ) ;
#13059=CARTESIAN_POINT ( 'NONE',  ( -47.60396279792517760, 12.80997843568595940, -70.56710525558601432 ) ) ;
#13060=CARTESIAN_POINT ( 'NONE',  ( -7.825402957745081878, 7.899365992529268965, -23.57352014148015584 ) ) ;
#13062=CARTESIAN_POINT ( 'NONE',  ( -59.56523643198714524, 15.93788386494078502, 16.96843438806351401 ) ) ;
#13065=ORIENTED_EDGE ( 'NONE', *, *, #1437, .F. ) ;
#13066=CARTESIAN_POINT ( 'NONE',  ( 106.0171289417044136, 26.97542621030654786, -64.06623974535388300 ) ) ;
#13067=CARTESIAN_POINT ( 'NONE',  ( 44.34689728705970424, 10.12166135033765357, -10.61515644663351310 ) ) ;
#13068=CARTESIAN_POINT ( 'NONE',  ( 44.34263167748003553, 9.103379693481581825, 58.59462232353900646 ) ) ;
#13072=CARTESIAN_POINT ( 'NONE',  ( -76.78936026062119424, 21.61552955137052834, 57.49749715836401975 ) ) ;
#13073=CARTESIAN_POINT ( 'NONE',  ( -165.9122696334864884, 79.44688201528255433, 63.07591441595136672 ) ) ;
#13075=ORIENTED_EDGE ( 'NONE', *, *, #29593, .F. ) ;
#13080=CARTESIAN_POINT ( 'NONE',  ( 110.2429982417149432, 29.99119854320844070, 71.45576479620103783 ) ) ;
#13082=VECTOR ( 'NONE', #18171, 1000.000000000000000 ) ;
#13083=CARTESIAN_POINT ( 'NONE',  ( 55.99998955208977236, 12.18058389017405219, -13.71295351543068541 ) ) ;
#13084=ORIENTED_EDGE ( 'NONE', *, *, #53959, .T. ) ;
#13087=CARTESIAN_POINT ( 'NONE',  ( 22.28700331106867338, 7.803633676228379557, -39.26703075270760479 ) ) ;
#13088=CARTESIAN_POINT ( 'NONE',  ( -85.35127931077727226, 24.98147633333000073, -19.18063208637886774 ) ) ;
#13090=CARTESIAN_POINT ( 'NONE',  ( 212.1962110267000412, 117.2292732107321740, -17.35804251465089010 ) ) ;
#13091=FACE_BOUND ( 'NONE', #30499, .T. ) ;
#13096=DIRECTION ( 'NONE',  ( 0.000000000000000000, 0.000000000000000000, 1.000000000000000000 ) ) ;
#13097=CARTESIAN_POINT ( 'NONE',  ( 38.43102714813441878, 9.298961820315048143, -77.41741745035568556 ) ) ;
#13098=CARTESIAN_POINT ( 'NONE',  ( -180.0094637318086370, 96.72611451757710199, 8.496329745107461306 ) ) ;
#13099=CARTESIAN_POINT ( 'NONE',  ( 208.5936709733498162, 113.6229123546138169, 57.12947936804001614 ) ) ;
#13100=CARTESIAN_POINT ( 'NONE',  ( 15.78827728214693416, -170.0000000000000000, 91.20380885363260859 ) ) ;
#13104=CARTESIAN_POINT ( 'NONE',  ( 204.6977192012829505, 108.0580384837234931, -51.32593103262161094 ) ) ;
#13105=ADVANCED_FACE ( 'NONE', ( #39677 ), #23857, .F. ) ;
#13109=CARTESIAN_POINT ( 'NONE',  ( -82.53770812813174018, 23.83403279300014788, -75.88817085053467792 ) ) ;
#13110=CARTESIAN_POINT ( 'NONE',  ( -60.64199216239839529, 17.30050036439945416, -20.87887065183614865 ) ) ;
#13111=EDGE_CURVE ( 'NONE', #2381, #50858, #35499, .T. ) ;
#13112=CARTESIAN_POINT ( 'NONE',  ( 92.95016907945947082, 22.74936990452176033, -74.21060328399696004 ) ) ;
#13113=EDGE_LOOP ( 'NONE', ( #25821, #26800, #42905, #29775 ) ) ;
#13116=CARTESIAN_POINT ( 'NONE',  ( 45.76553115525425852, 10.34124506813255095, 60.28159494287191222 ) ) ;
#13117=CARTESIAN_POINT ( 'NONE',  ( -105.1578917446807111, 35.40396694227245433, -89.27446617212257252 ) ) ;
#13118=CARTESIAN_POINT ( 'NONE',  ( 107.9213359589209063, 28.92595015506872969, 17.41395595518270412 ) ) ;
#13119=ORIENTED_EDGE ( 'NONE', *, *, #18421, .F. ) ;
#13123=CARTESIAN_POINT ( 'NONE',  ( -49.13048465129990205, 14.20828170588045403, 15.60104833568753335 ) ) ;
#13124=CARTESIAN_POINT ( 'NONE',  ( -14.96769463968061231, 8.472501390435335011, -94.16364436271733496 ) ) ;
#13126=CARTESIAN_POINT ( 'NONE',  ( 115.0692128464502417, 31.17922615202197889, -10.81633842045794935 ) ) ;
#13127=CARTESIAN_POINT ( 'NONE',  ( 94.13651963513105159, 22.12061817498822691, 90.79928215880261178 ) ) ;
#13128=CIRCLE ( 'NONE', #49036, 242.4895526022646379 ) ;
#13130=EDGE_LOOP ( 'NONE', ( #65191, #46774, #39522, #32891 ) ) ;
#13131=ORIENTED_EDGE ( 'NONE', *, *, #47776, .F. ) ;
#13133=ORIENTED_EDGE ( 'NONE', *, *, #46371, .T. ) ;
#13134=CARTESIAN_POINT ( 'NONE',  ( 45.36109889487609337, 9.259412558041150376, 15.14959608583331807 ) ) ;
#13135=CARTESIAN_POINT ( 'NONE',  ( -180.5668250991443813, 97.41296786328892665, 91.03718869750294118 ) ) ;
#13136=CARTESIAN_POINT ( 'NONE',  ( -53.13004807512038496, 14.17398740785108657, -8.606103191301974320 ) ) ;
#13137=CARTESIAN_POINT ( 'NONE',  ( 107.2672065034543039, 27.52931006625853882, -23.46636325839187265 ) ) ;
#13139=CARTESIAN_POINT ( 'NONE',  ( 197.1974290009104891, 96.59277840252784131, 9.539146130048552052 ) ) ;
#13140=CARTESIAN_POINT ( 'NONE',  ( 197.5344360088799363, 98.61758084709093453, 88.16435646324907793 ) ) ;
#13142=DIRECTION ( 'NONE',  ( -0.000000000000000000, 1.000000000000000000, -0.000000000000000000 ) ) ;
#13143=CARTESIAN_POINT ( 'NONE',  ( -9.763294602873864747, 7.024900256480051119, 44.86506734459265999 ) ) ;
#13146=CARTESIAN_POINT ( 'NONE',  ( 9.280894575734581764, 7.385644305345137717, -19.93533336458542848 ) ) ;
#13149=CARTESIAN_POINT ( 'NONE',  ( -142.9756886485678251, 60.11539876121634052, 7.681077562724933472 ) ) ;
#13150=CARTESIAN_POINT ( 'NONE',  ( 187.2296622856351576, 86.53808614709454616, -74.87664997496398200 ) ) ;
#13151=CARTESIAN_POINT ( 'NONE',  ( -38.90277964098074648, 11.96165882689933824, 90.60046426814015774 ) ) ;
#13152=CARTESIAN_POINT ( 'NONE',  ( -96.43148989374462587, 29.90755650959364331, -37.79297082079260406 ) ) ;
#13154=CARTESIAN_POINT ( 'NONE',  ( 15.78827728214693416, 7.507518794609589818, -50.51894409868581448 ) ) ;
#13155=CARTESIAN_POINT ( 'NONE',  ( 133.6288034103010318, 41.28708886999549321, -51.02331093239571658 ) ) ;
#13158=CARTESIAN_POINT ( 'NONE',  ( 188.5556894309611948, 88.00527073660660449, 91.18024676934048500 ) ) ;
#13161=CARTESIAN_POINT ( 'NONE',  ( 58.09436971064710775, 11.58462396079456447, -10.69534298273807238 ) ) ;
#13163=CARTESIAN_POINT ( 'NONE',  ( 197.5344433744249102, 98.61756151884679866, 65.79699254537881359 ) ) ;
#13165=CARTESIAN_POINT ( 'NONE',  ( 45.89268866913129585, 10.36133864615982780, -66.19858745361412389 ) ) ;
#13166=CARTESIAN_POINT ( 'NONE',  ( -61.76386578474847511, 17.63453064612502175, -72.94559511649701733 ) ) ;
#13167=CARTESIAN_POINT ( 'NONE',  ( 201.9721407532275066, 104.3507814346148166, -63.67126515581958301 ) ) ;
#13169=VECTOR ( 'NONE', #10133, 1000.000000000000000 ) ;
#13170=CARTESIAN_POINT ( 'NONE',  ( -180.6209440844957896, 95.88392769199009535, -41.89197730208912418 ) ) ;
#13172=CARTESIAN_POINT ( 'NONE',  ( -165.6212796729685124, 79.15047440262051737, 11.17022651014945289 ) ) ;
#13173=CARTESIAN_POINT ( 'NONE',  ( -125.8938041572051389, -170.0000000000000000, -76.75825448869764500 ) ) ;
#13174=FACE_BOUND ( 'NONE', #53592, .T. ) ;
#13177=CARTESIAN_POINT ( 'NONE',  ( -5.401648928593175469, 6.744888135494087500, 71.57446707354854709 ) ) ;
#13182=DIRECTION ( 'NONE',  ( -0.000000000000000000, 1.000000000000000000, -0.000000000000000000 ) ) ;
#13185=CIRCLE ( 'NONE', #69343, 243.4957430088094839 ) ;
#13187=ORIENTED_EDGE ( 'NONE', *, *, #42078, .T. ) ;
#13192=ORIENTED_EDGE ( 'NONE', *, *, #41787, .F. ) ;
#13194=CARTESIAN_POINT ( 'NONE',  ( 154.6530827109543509, 56.75509330623211213, 43.86387257709986187 ) ) ;
#13199=CARTESIAN_POINT ( 'NONE',  ( -1.083610669212424105, 6.545642299653493978, 14.09380834579263642 ) ) ;
#13201=CARTESIAN_POINT ( 'NONE',  ( -81.23268307104839892, 24.39742801172156561, 30.86689043824910073 ) ) ;
#13202=CARTESIAN_POINT ( 'NONE',  ( 15.78827728214693416, -170.0000000000000000, 37.51470767270523510 ) ) ;
#13203=CARTESIAN_POINT ( 'NONE',  ( 136.1081004736419686, 42.80058051492063953, 3.007995494952832249 ) ) ;
#13206=CARTESIAN_POINT ( 'NONE',  ( -74.39861643904069410, 21.81123504700007487, 17.24566514567988662 ) ) ;
#13208=CARTESIAN_POINT ( 'NONE',  ( 46.65037935242577305, 9.463293687292225087, -41.17784024966125145 ) ) ;
#13210=CARTESIAN_POINT ( 'NONE',  ( -118.6806115626323930, 41.92435854543968077, 89.72766250507453378 ) ) ;
#13212=B_SPLINE_CURVE_WITH_KNOTS ( 'NONE', 3,
 ( #18200, #39654, #1670, #12933, #34736, #45271, #56173, #24179, #11871, #54775, #38967, #65702, #6601, #1320, #60413, #17494, #33694, #23133, #44582, #68132, #8347, #46654, #14312, #3070, #47004, #35068, #67782, #18894, #63188, #30836, #46302, #57221, #61791, #51933, #19937, #29792, #19579, #9727, #24866, #35416, #9036, #41037, #30151, #45629 ),
 .UNSPECIFIED., .F., .F.,
 ( 4, 2, 2, 2, 2, 2, 2, 2, 2, 2, 2, 2, 1, 2, 2, 2, 2, 2, 2, 1, 2, 2, 4 ),
 ( 0.02381751147647563627, 0.02531129726520766482, 0.02605819015957367563, 0.02680508305393968990, 0.02829886884267171498, 0.02979265463140373660, 0.03053954752576975781, 0.03128644042013577209, 0.03278022620886781452, 0.03427401199759985695, 0.03576779778633189938, 0.03651469068069792406, 0.03726158357506394181, 0.03800847646942997343, 0.03875536936379599118, 0.04024915515252804055, 0.04174294094126008992, 0.04323672672999213928, 0.04398361962435816397, 0.04473051251872418865, 0.04547740541309021334, 0.04622429830745623802, 0.04771808409618830821 ),
 .UNSPECIFIED. ) ;
#13213=CARTESIAN_POINT ( 'NONE',  ( -78.66644367742109978, 22.32174330031320508, -61.96000122218157458 ) ) ;
#13215=ORIENTED_EDGE ( 'NONE', *, *, #61006, .F. ) ;
#13216=CARTESIAN_POINT ( 'NONE',  ( -146.7345109736526467, 61.86270848728297267, 72.03746416512107942 ) ) ;
#13217=AXIS2_PLACEMENT_3D ( 'NONE', #47083, #62586, #63271 ) ;
#13221=CARTESIAN_POINT ( 'NONE',  ( 133.8566784816069628, 41.42467568809809819, -9.178760341931967659 ) ) ;
#13224=CARTESIAN_POINT ( 'NONE',  ( -173.5372686962699902, 89.10569330281722955, -22.86740657428632417 ) ) ;
#13225=CARTESIAN_POINT ( 'NONE',  ( -154.0775378574014383, 68.15437918458553668, -36.34688571082521236 ) ) ;
#13229=CARTESIAN_POINT ( 'NONE',  ( 102.8111940033034273, 25.59308899183601227, 64.99745727866086042 ) ) ;
#13235=CARTESIAN_POINT ( 'NONE',  ( -107.0751323097254186, 35.28386110859231906, 59.07576044861188791 ) ) ;
#13236=DIRECTION ( 'NONE',  ( 0.000000000000000000, 0.000000000000000000, 1.000000000000000000 ) ) ;
#13237=CARTESIAN_POINT ( 'NONE',  ( 157.4703587214989113, 57.65129005721576760, -77.96873488960135035 ) ) ;
#13241=LINE ( 'NONE', #7955, #20650 ) ;
#13243=CARTESIAN_POINT ( 'NONE',  ( -71.82968714595206450, 19.83409541362842887, 94.70823564810032735 ) ) ;
#13246=CARTESIAN_POINT ( 'NONE',  ( 63.01563776193091826, -170.0000000000000000, -77.56524142263344856 ) ) ;
#13247=CARTESIAN_POINT ( 'NONE',  ( -58.32502757340553501, 16.62877055630753631, 31.05165587581745967 ) ) ;
#13249=CARTESIAN_POINT ( 'NONE',  ( 58.09877917144281412, 12.61383386832654452, 31.62849139763403983 ) ) ;
#13250=CARTESIAN_POINT ( 'NONE',  ( 42.60443493776924839, 8.846984668533421470, 84.28900201317352980 ) ) ;
#13251=EDGE_CURVE ( 'NONE', #19626, #47003, #68157, .T. ) ;
#13255=CARTESIAN_POINT ( 'NONE',  ( -15.13464256769235838, 8.488509377255647692, 12.46951090161849862 ) ) ;
#13256=CARTESIAN_POINT ( 'NONE',  ( -142.0685766576042113, 58.11789490499572253, 12.48546705073966123 ) ) ;
#13258=CARTESIAN_POINT ( 'NONE',  ( -102.2801239173131052, 32.78103895658057354, -76.85912785543962400 ) ) ;
#13259=CARTESIAN_POINT ( 'NONE',  ( 181.0840389613909736, 80.03940679743416808, -51.22505766587963905 ) ) ;
#13261=ORIENTED_EDGE ( 'NONE', *, *, #54911, .T. ) ;
#13262=CARTESIAN_POINT ( 'NONE',  ( 132.0563630623056781, 41.51825634609595284, -50.80769278490465979 ) ) ;
#13263=CARTESIAN_POINT ( 'NONE',  ( -38.88884187334148379, 11.95889603743728280, -43.81403857136609048 ) ) ;
#13266=CARTESIAN_POINT ( 'NONE',  ( -178.0096424707516576, 92.73811996563144078, 86.29695439451984385 ) ) ;
#13272=CARTESIAN_POINT ( 'NONE',  ( 204.3129818922372749, 107.5244029525888436, 2.363170148305748341 ) ) ;
#13275=CARTESIAN_POINT ( 'NONE',  ( 162.8241818775801164, 63.24198268785130495, 85.33621435715247117 ) ) ;
#13276=EDGE_CURVE ( 'NONE', #48827, #33721, #37978, .T. ) ;
#13277=ORIENTED_EDGE ( 'NONE', *, *, #25240, .F. ) ;
#13278=CARTESIAN_POINT ( 'NONE',  ( 163.1402336665937582, 63.50458794835979148, -92.38649040534465939 ) ) ;
#13281=CARTESIAN_POINT ( 'NONE',  ( -154.8006992380338431, 70.15733562427986669, 43.55549133835197750 ) ) ;
#13283=CARTESIAN_POINT ( 'NONE',  ( 23.24028701062093916, 6.853614888934261629, -42.04100009002929994 ) ) ;
#13288=CARTESIAN_POINT ( 'NONE',  ( -1.675000714904271826, 7.575396497802214135, -92.29381673850149070 ) ) ;
#13289=ORIENTED_EDGE ( 'NONE', *, *, #52180, .F. ) ;
#13291=CARTESIAN_POINT ( 'NONE',  ( 176.6156959113759513, 75.60152827082541194, 42.85099558256738561 ) ) ;
#13293=DIRECTION ( 'NONE',  ( -0.000000000000000000, 1.000000000000000000, -0.000000000000000000 ) ) ;
#13294=CARTESIAN_POINT ( 'NONE',  ( -11.79249160485392878, 8.191429102467035150, -63.39294633506229104 ) ) ;
#13297=CARTESIAN_POINT ( 'NONE',  ( -24.32776401346968953, 9.546905915310563984, 40.14952946743263595 ) ) ;
#13300=CARTESIAN_POINT ( 'NONE',  ( -75.65611349188964141, 22.26947559308018398, -49.48898812600347696 ) ) ;
#13303=CARTESIAN_POINT ( 'NONE',  ( 211.1046732743772907, 117.3965485104337461, -66.76179994842109977 ) ) ;
#13304=CARTESIAN_POINT ( 'NONE',  ( 140.5958192060901695, 46.84598876498520781, 33.70861045256287269 ) ) ;
#13305=CARTESIAN_POINT ( 'NONE',  ( 117.3246714514015849, 33.42485879931865611, 34.58965814092242397 ) ) ;
#13306=CARTESIAN_POINT ( 'NONE',  ( -132.2161740628506266, 52.03204870034954155, 7.232691840498619129 ) ) ;
#13311=CARTESIAN_POINT ( 'NONE',  ( 211.3773738276420886, 115.9764855123643912, -94.07397666197054775 ) ) ;
#13312=CYLINDRICAL_SURFACE ( 'NONE', #57160, 7.500000000000013323 ) ;
#13316=CARTESIAN_POINT ( 'NONE',  ( -133.0808647576833437, 51.41195281028754493, 67.12459488774240413 ) ) ;
#13317=CARTESIAN_POINT ( 'NONE',  ( -73.63128929564827274, 21.53548093502884697, -10.20693752301225921 ) ) ;
#13319=CARTESIAN_POINT ( 'NONE',  ( 204.6977192012829789, -170.0000000000000000, -70.67048162308527992 ) ) ;
#13325=CARTESIAN_POINT ( 'NONE',  ( 185.5572090022886300, 83.24697331286184010, 42.84673731889779447 ) ) ;
#13328=CARTESIAN_POINT ( 'NONE',  ( -119.9771613955297340, 43.90337778233484300, 60.34853762580112146 ) ) ;
#13329=CARTESIAN_POINT ( 'NONE',  ( -47.68742944762957592, 12.82957801017946764, 12.45128233048862576 ) ) ;
#13333=CARTESIAN_POINT ( 'NONE',  ( -108.4971425592086973, 36.05284916722902722, -92.00252201140912689 ) ) ;
#13334=CARTESIAN_POINT ( 'NONE',  ( -156.9910258076866398, 70.79617246506501260, -16.04192918424444514 ) ) ;
#13337=CARTESIAN_POINT ( 'NONE',  ( -62.14837099232448026, 17.75045801599141626, 67.10412718371505036 ) ) ;
#13341=CARTESIAN_POINT ( 'NONE',  ( 157.4703587214989113, 58.92748579479259519, -62.96873488960130771 ) ) ;
#13342=CARTESIAN_POINT ( 'NONE',  ( -100.4466073551323007, 31.85873123265078988, -22.95728695924190887 ) ) ;
#13343=CARTESIAN_POINT ( 'NONE',  ( 141.2470358420065679, 46.06959063280893218, -42.21817649076449186 ) ) ;
#13350=CARTESIAN_POINT ( 'NONE',  ( 31.90170717962883273, 8.563261373066630711, -16.03511419624575751 ) ) ;
#13351=CARTESIAN_POINT ( 'NONE',  ( 183.9986899696430385, 81.60141257362811018, 3.040213554178509803 ) ) ;
#13352=CARTESIAN_POINT ( 'NONE',  ( 91.49345572560145001, 21.13836538408680710, 58.34269035543120907 ) ) ;
#13359=ORIENTED_EDGE ( 'NONE', *, *, #5924, .F. ) ;
#13362=CARTESIAN_POINT ( 'NONE',  ( 66.08620257826612487, 13.40585338179128527, 71.00441744036213265 ) ) ;
#13363=CARTESIAN_POINT ( 'NONE',  ( 135.6793972494602372, 43.71805072851428520, 2.876098451181287263 ) ) ;
#13367=CARTESIAN_POINT ( 'NONE',  ( 9.416656162223551618, 6.380306691996769253, 41.47870453118932943 ) ) ;
#13369=CARTESIAN_POINT ( 'NONE',  ( 70.11969827741708627, 15.47408882293424170, 66.61225004732548882 ) ) ;
#13373=CARTESIAN_POINT ( 'NONE',  ( 164.0073343966821824, 64.23003864582457823, -39.93842790887263305 ) ) ;
#13380=CARTESIAN_POINT ( 'NONE',  ( -101.3502439362134453, 33.43728945125134544, 3.717829675835958803 ) ) ;
#13381=CARTESIAN_POINT ( 'NONE',  ( 60.45161273195552809, 13.12223384504257062, 83.92330211886128666 ) ) ;
#13382=CARTESIAN_POINT ( 'NONE',  ( 154.6260751278567227, 56.73429849676967507, -90.36338124960292362 ) ) ;
#13383=CARTESIAN_POINT ( 'NONE',  ( 83.37782009939536465, 19.39546426214656805, -9.714140923952603757 ) ) ;
#13384=CARTESIAN_POINT ( 'NONE',  ( -165.6212796729685692, 79.15047440262054579, 38.01477710061311654 ) ) ;
#13385=CARTESIAN_POINT ( 'NONE',  ( 38.98629290190360308, 9.369974505438298351, -89.30891864635512434 ) ) ;
#13386=CARTESIAN_POINT ( 'NONE',  ( 126.4324872316702795, 37.11876756822024248, -69.27188833358552245 ) ) ;
#13388=CARTESIAN_POINT ( 'NONE',  ( -95.86163447241557378, 30.75089131639700213, 60.95167474732399882 ) ) ;
#13389=CYLINDRICAL_SURFACE ( 'NONE', #52346, 7.500000000000013323 ) ;
#13391=CARTESIAN_POINT ( 'NONE',  ( -156.3734885497381413, 71.59531449004286685, -45.34277193519254467 ) ) ;
#13392=CARTESIAN_POINT ( 'NONE',  ( 211.3757499519976761, 117.8130818709823444, -13.55636099387667315 ) ) ;
#13394=CARTESIAN_POINT ( 'NONE',  ( -196.7348448768811409, -170.0000000000000000, 38.42256797338300345 ) ) ;
#13397=CARTESIAN_POINT ( 'NONE',  ( -5.183193881612056408, 7.740932022135017299, -9.050052149217117758 ) ) ;
#13398=CARTESIAN_POINT ( 'NONE',  ( 174.9042454172879673, 72.57746269938724026, 14.24426339932219321 ) ) ;
#13399=CARTESIAN_POINT ( 'NONE',  ( -61.51762070241280611, 16.51067482779404116, 14.78299046999394228 ) ) ;
#13400=ORIENTED_EDGE ( 'NONE', *, *, #41535, .T. ) ;
#13403=CARTESIAN_POINT ( 'NONE',  ( 102.8066580714140628, 25.59117171227001108, -71.27532258126962006 ) ) ;
#13404=CARTESIAN_POINT ( 'NONE',  ( 40.38132770291768026, 9.553709436640062336, -8.823569451234918759 ) ) ;
#13405=CARTESIAN_POINT ( 'NONE',  ( 41.35041461497707616, 8.670465437677201237, 71.51759960298838337 ) ) ;
#13410=CARTESIAN_POINT ( 'NONE',  ( 55.76286625948333864, 12.13284185313540142, -95.00000000000133582 ) ) ;
#13412=VERTEX_POINT ( 'NONE', #66956 ) ;
#13418=CARTESIAN_POINT ( 'NONE',  ( -168.1811549361197251, 83.25427431521133315, 59.51798107920270553 ) ) ;
#13421=CIRCLE ( 'NONE', #2178, 242.4895526022646379 ) ;
#13422=CARTESIAN_POINT ( 'NONE',  ( 62.04382205963243280, 13.48099884269679904, -8.923339836102410771 ) ) ;
#13426=CARTESIAN_POINT ( 'NONE',  ( 18.43272992546528144, 7.606837839440253823, -35.99631868335740847 ) ) ;
#13431=EDGE_CURVE ( 'NONE', #52438, #20401, #37841, .T. ) ;
#13433=EDGE_CURVE ( 'NONE', #59702, #59334, #50442, .T. ) ;
#13438=CARTESIAN_POINT ( 'NONE',  ( -175.1895962157336726, 90.99110972060685754, 4.255677171492019184 ) ) ;
#13441=CARTESIAN_POINT ( 'NONE',  ( 188.1848725084043110, -170.0000000000000000, -95.00000000000133582 ) ) ;
#13442=EDGE_LOOP ( 'NONE', ( #2747, #2366 ) ) ;
#13444=CARTESIAN_POINT ( 'NONE',  ( 197.2199163281727579, 98.22431253015348318, -44.48933272678075213 ) ) ;
#13448=B_SPLINE_CURVE_WITH_KNOTS ( 'NONE', 3,
 ( #9084, #68510, #19630, #67831, #46705, #25617, #19987, #68182, #52666, #36851, #14695, #15048, #36158, #4154, #52330, #47051, #10110, #31567, #53698, #42797, #49105, #32266, #37883, #22394, #22045, #236, #5518, #54743, #60384, #26973, #60018, #43144, #64264, #44181, #944, #26640, #11838, #1292, #6568, #11477, #59326, #48757, #69530, #65670, #17458 ),
 .UNSPECIFIED., .F., .F.,
 ( 4, 2, 2, 2, 2, 2, 2, 2, 2, 2, 2, 2, 2, 1, 2, 2, 2, 2, 2, 2, 2, 2, 4 ),
 ( 0.02356759485890611364, 0.02503765354686411301, 0.02577268289084312311, 0.02650771223482213321, 0.02797777092278017075, 0.02944782961073821176, 0.03018285895471723573, 0.03091788829869626318, 0.03238794698665432847, 0.03312297633063336633, 0.03385800567461239724, 0.03532806436257047294, 0.03606309370654951080, 0.03679812305052855559, 0.03753315239450759344, 0.03826818173848663129, 0.03973824042644470700, 0.04120829911440278270, 0.04267835780236085841, 0.04341338714633990320, 0.04414841649031894799, 0.04561847517827702370, 0.04708853386623510634 ),
 .UNSPECIFIED. ) ;
#13449=CARTESIAN_POINT ( 'NONE',  ( -84.96580414052107244, 24.82184094495577398, -65.38213935470189142 ) ) ;
#13456=CARTESIAN_POINT ( 'NONE',  ( -104.9609170480078717, 35.30014942885841833, -89.19597386970725950 ) ) ;
#13457=CARTESIAN_POINT ( 'NONE',  ( 23.03864809957654103, 6.841061756139154681, 12.60473612569555257 ) ) ;
#13461=CARTESIAN_POINT ( 'NONE',  ( -55.05276343752909440, 15.72344139423348430, 3.472777182467473800 ) ) ;
#13462=CARTESIAN_POINT ( 'NONE',  ( -128.1282195935087316, 49.19720162550164844, -22.73222316029650614 ) ) ;
#13465=CARTESIAN_POINT ( 'NONE',  ( 79.14113188808478583, 18.05280674635440974, -42.83065476743007594 ) ) ;
#13471=CARTESIAN_POINT ( 'NONE',  ( 41.33692564073607656, 8.668977654195478166, 3.319058603837437005 ) ) ;
#13472=CARTESIAN_POINT ( 'NONE',  ( -180.6114021174235802, 97.46813718571149820, 92.54769712921735447 ) ) ;
#13474=CARTESIAN_POINT ( 'NONE',  ( 107.9362503323352627, 27.82881837607800435, -9.425457200440790828 ) ) ;
#13475=CARTESIAN_POINT ( 'NONE',  ( 203.1420903260745945, 104.2307086582027154, 17.24464569073724718 ) ) ;
#13477=CARTESIAN_POINT ( 'NONE',  ( 211.1620569867183690, 117.4844252930219142, 86.57602862735129179 ) ) ;
#13479=CARTESIAN_POINT ( 'NONE',  ( -72.76696720809545127, 20.16136115364207626, -64.80250377197498324 ) ) ;
#13481=VERTEX_POINT ( 'NONE', #67987 ) ;
#13482=CARTESIAN_POINT ( 'NONE',  ( 11.82929895397813702, 7.412564870773604930, -22.54914669578485942 ) ) ;
#13485=CARTESIAN_POINT ( 'NONE',  ( 110.2429982417149574, -170.0000000000000000, 56.45576479620100940 ) ) ;
#13486=CARTESIAN_POINT ( 'NONE',  ( 188.5653887627528036, 88.01608521313130495, -71.17894925488377567 ) ) ;
#13487=CARTESIAN_POINT ( 'NONE',  ( -36.68762645608095596, 11.53530882149086345, 86.01941686338382453 ) ) ;
#13489=CARTESIAN_POINT ( 'NONE',  ( -97.85576954355158819, 30.58918648956190367, -36.43939751378721326 ) ) ;
#13490=EDGE_CURVE ( 'NONE', #19842, #27330, #44579, .T. ) ;
#13493=FACE_OUTER_BOUND ( 'NONE', #31970, .T. ) ;
#13494=CARTESIAN_POINT ( 'NONE',  ( 126.8947007444828614, 37.37669340849691935, -46.32467590398648127 ) ) ;
#13495=ORIENTED_EDGE ( 'NONE', *, *, #58076, .T. ) ;
#13498=B_SPLINE_CURVE_WITH_KNOTS ( 'NONE', 3,
 ( #31050, #16831, #20473, #41935, #41590, #63048, #30697, #6284, #36319, #52492, #43561, #33022, #9588, #27736, #59733, #1015, #10263, #53158, #36667, #22465, #48822, #31387, #58119, #667, #20825, #20136, #9933, #52821, #4644, #65033, #63747, #14853, #46872, #38293, #11544, #47204, #52148, #65388, #26107, #69000, #25775, #49174, #15556, #68336, #57775, #43906, #57428, #37006, #9241, #3965, #25433, #4313, #18582, #2412, #22817, #54813, #34076 ),
 .UNSPECIFIED., .F., .F.,
 ( 4, 2, 2, 2, 2, 2, 2, 2, 2, 2, 2, 2, 2, 2, 2, 2, 2, 2, 2, 1, 2, 2, 2, 2, 2, 2, 2, 2, 4 ),
 ( 0.000000000000000000, 0.001945600724231584880, 0.002918401086347380356, 0.003891201448463174964, 0.004864001810578970006, 0.005836802172694765915, 0.006809602534810560090, 0.007782402896926355132, 0.009728003621157898378, 0.01070080398327367087, 0.01167360434538944162, 0.01264640470750521412, 0.01361920506962098487, 0.01459200543173675736, 0.01556480579385252812, 0.01751040651808407483, 0.01848320688019983171, 0.01945600724231559206, 0.02042880760443134547, 0.02140160796654710582, 0.02237440832866286616, 0.02334720869077861957, 0.02529280941501012639, 0.02626560977712589715, 0.02723841013924166443, 0.02821121050135743172, 0.02918401086347320247, 0.03015681122558896282, 0.03112961158770473011 ),
 .UNSPECIFIED. ) ;
#13499=CARTESIAN_POINT ( 'NONE',  ( 187.7395187440304483, 87.09941059914879702, 93.95990058528536792 ) ) ;
#13503=CARTESIAN_POINT ( 'NONE',  ( -30.47069031368414826, 9.433993659086572947, -77.11504745095709268 ) ) ;
#13507=CARTESIAN_POINT ( 'NONE',  ( 110.2429982417149432, 29.99119854320844070, 71.45576479620103783 ) ) ;
#13510=CARTESIAN_POINT ( 'NONE',  ( -62.55184817504201789, 17.87278652436698323, -70.07648453095528396 ) ) ;
#13511=CARTESIAN_POINT ( 'NONE',  ( 202.7540649946182896, 105.3989460363904698, -77.92562021146432016 ) ) ;
#13514=CARTESIAN_POINT ( 'NONE',  ( -168.2754450152258130, 81.89160173753974448, -90.15994169745837894 ) ) ;
#13516=CARTESIAN_POINT ( 'NONE',  ( -49.45858366215606594, 13.25262207532078129, 59.66029130467421027 ) ) ;
#13519=CARTESIAN_POINT ( 'NONE',  ( -99.40806599580240288, 31.34569488980110208, -89.27206661197627113 ) ) ;
#13520=ORIENTED_EDGE ( 'NONE', *, *, #54538, .F. ) ;
#13524=CARTESIAN_POINT ( 'NONE',  ( 150.2941978382489197, 53.52137138947627903, 61.55703088605018536 ) ) ;
#13525=CARTESIAN_POINT ( 'NONE',  ( 15.78827728214693416, -170.0000000000000000, 3.170157082241545687 ) ) ;
#13527=CIRCLE ( 'NONE', #52806, 242.4895526022646379 ) ;
#13535=CARTESIAN_POINT ( 'NONE',  ( 157.0316110297313514, 58.58403635656375030, 44.40946747225339664 ) ) ;
#13539=CARTESIAN_POINT ( 'NONE',  ( -179.2177980985565284, 94.18084789436635162, 7.101110558428060493 ) ) ;
#13540=CARTESIAN_POINT ( 'NONE',  ( -3.244108878396732010, 6.635632329121484041, 16.72956101399090301 ) ) ;
#13543=CARTESIAN_POINT ( 'NONE',  ( -86.15466590221103615, 26.40813842494318209, 38.41035032410803041 ) ) ;
#13544=CARTESIAN_POINT ( 'NONE',  ( 151.3976820382521851, 53.07948349322499837, 94.99999999999866418 ) ) ;
#13545=DIRECTION ( 'NONE',  ( -0.000000000000000000, 1.000000000000000000, -0.000000000000000000 ) ) ;
#13546=EDGE_LOOP ( 'NONE', ( #31855, #65207, #43147, #59425 ) ) ;
#13547=CARTESIAN_POINT ( 'NONE',  ( 117.4830770399668012, 32.37795270233550582, -41.39853099672338743 ) ) ;
#13550=B_SPLINE_CURVE_WITH_KNOTS ( 'NONE', 3,
 ( #5015, #26482, #21204, #19827, #42651, #48942, #34806, #10981, #1476, #22237, #28202, #784, #22937, #33503, #43676, #59506, #38773, #37715, #16946, #32791 ),
 .UNSPECIFIED., .F., .F.,
 ( 4, 2, 2, 2, 2, 2, 2, 2, 2, 4 ),
 ( 0.000000000000000000, 0.001358410513504409783, 0.002037615770256615000, 0.002716821027008819566, 0.004075231540513249949, 0.005433642054017679898, 0.006792052567522109847, 0.008150463081026539797, 0.009508873594530970613, 0.01086728410803540143 ),
 .UNSPECIFIED. ) ;
#13554=CARTESIAN_POINT ( 'NONE',  ( 85.67138972405899722, 19.09593469918314312, -50.77549759938765561 ) ) ;
#13557=CARTESIAN_POINT ( 'NONE',  ( -149.2910611247327779, 63.99625741915655652, 72.56537183036279259 ) ) ;
#13558=CARTESIAN_POINT ( 'NONE',  ( 86.15454111412293514, 20.32174891186169319, 29.71208757247930521 ) ) ;
#13563=CARTESIAN_POINT ( 'NONE',  ( -174.7817412490652202, 90.52199442492060655, -22.69333526547698554 ) ) ;
#13566=ORIENTED_EDGE ( 'NONE', *, *, #42878, .F. ) ;
#13567=CARTESIAN_POINT ( 'NONE',  ( 106.6228877857910646, 27.24245963308690577, 70.54164431714124817 ) ) ;
#13569=CARTESIAN_POINT ( 'NONE',  ( -189.2739965869454295, 107.1373753350176372, 64.38768254793554036 ) ) ;
#13572=CARTESIAN_POINT ( 'NONE',  ( 164.8886903222556839, 63.65672212134877839, -71.60819778663672253 ) ) ;
#13573=ORIENTED_EDGE ( 'NONE', *, *, #24510, .T. ) ;
#13576=ORIENTED_EDGE ( 'NONE', *, *, #51775, .F. ) ;
#13578=CARTESIAN_POINT ( 'NONE',  ( 39.40195752203892710, -170.0000000000000000, 10.56928371549958889 ) ) ;
#13579=CARTESIAN_POINT ( 'NONE',  ( 178.6969023688950244, 76.22585248861962270, -90.29539480279383667 ) ) ;
#13580=CARTESIAN_POINT ( 'NONE',  ( 68.95451040317566083, 14.12887482153123919, -38.61394121317524508 ) ) ;
#13582=CARTESIAN_POINT ( 'NONE',  ( -56.96436614829621448, 16.24647150911285109, 30.56099534412708252 ) ) ;
#13584=CARTESIAN_POINT ( 'NONE',  ( 133.8566784816069628, 41.42467568809809819, -9.178760341931967659 ) ) ;
#13586=CARTESIAN_POINT ( 'NONE',  ( 32.38131036485454217, 7.599882848866447382, 93.82335863281235788 ) ) ;
#13590=CARTESIAN_POINT ( 'NONE',  ( -0.7215816834507526867, 6.532459459468098473, -45.33604404609089755 ) ) ;
#13592=CARTESIAN_POINT ( 'NONE',  ( -189.2346268516247960, 107.0830361517164988, -41.89910121709165480 ) ) ;
#13593=CARTESIAN_POINT ( 'NONE',  ( -143.2464978228198333, 59.04559547356109306, 15.51374128211022985 ) ) ;
#13594=CARTESIAN_POINT ( 'NONE',  ( 16.27775141556967498, 7.523247835309955889, -23.67439350822211708 ) ) ;
#13595=CARTESIAN_POINT ( 'NONE',  ( -104.5827168854524558, 33.96561401163047833, -76.51241882879068612 ) ) ;
#13599=CARTESIAN_POINT ( 'NONE',  ( -24.85653282846401879, -170.0000000000000000, 94.99999999999866418 ) ) ;
#13600=CARTESIAN_POINT ( 'NONE',  ( -38.16652041892308489, 11.81761816422916311, -46.16894994732523827 ) ) ;
#13603=CARTESIAN_POINT ( 'NONE',  ( -165.9043865781291345, 79.43878925126232105, 89.93817603964164675 ) ) ;
#13605=CARTESIAN_POINT ( 'NONE',  ( 126.3554864210861837, 38.22801630372151749, 10.39375937215169543 ) ) ;
#13606=B_SPLINE_CURVE_WITH_KNOTS ( 'NONE', 3,
 ( #26366, #27381, #38289, #47806, #53414, #59730, #26022, #53761, #5583, #63658, #69265, #21091, #42535, #63988, #10515, #16490, #31984, #27036, #48467, #21761, #65384, #27733, #17890, #12611, #17172, #55158, #1359, #39004, #22813, #38645, #44257, #6982, #44961, #23864, #34072, #45306, #60788, #55513, #54451, #40037, #7340, #66790, #33726, #66446, #12264, #28796, #50245, #39345, #60448, #6280, #23171, #2066, #65738, #11907, #44617, #11541, #60085 ),
 .UNSPECIFIED., .F., .F.,
 ( 4, 2, 2, 2, 2, 2, 2, 2, 2, 2, 2, 2, 2, 2, 1, 2, 2, 2, 2, 2, 2, 2, 2, 2, 2, 2, 2, 2, 4 ),
 ( 0.000000000000000000, 0.001985873147602438497, 0.002978809721403657528, 0.003971746295204876993, 0.004964682869006096892, 0.005957619442807315056, 0.006950556016608534955, 0.007943492590409753987, 0.008936429164210973886, 0.009929365738012193784, 0.01092230231181341195, 0.01191523888561463011, 0.01390111203321707858, 0.01489404860701831583, 0.01588698518081955308, 0.01687992175462078859, 0.01787285832842202757, 0.01985873147602450206, 0.02085166804982573063, 0.02184460462362696268, 0.02283754119742819125, 0.02383047777122941982, 0.02581635091883191166, 0.02680928749263316452, 0.02780222406643441391, 0.02879516064023566677, 0.02978809721403691615, 0.03078103378783816901, 0.03177397036163941840 ),
 .UNSPECIFIED. ) ;
#13609=VERTEX_POINT ( 'NONE', #17981 ) ;
#13610=CARTESIAN_POINT ( 'NONE',  ( 150.7605657748150065, 53.86013773008568961, 87.22787840158356687 ) ) ;
#13614=CARTESIAN_POINT ( 'NONE',  ( -157.0079874970172682, 72.18249880494037996, 38.49446316589058625 ) ) ;
#13616=CYLINDRICAL_SURFACE ( 'NONE', #52974, 7.500000000000020428 ) ;
#13619=CARTESIAN_POINT ( 'NONE',  ( -0.6830060531215994546, 7.537854477244023244, -94.16412398650113857 ) ) ;
#13622=CARTESIAN_POINT ( 'NONE',  ( 174.4978817191264397, 73.57770570413202904, 33.21040157506908486 ) ) ;
#13623=CARTESIAN_POINT ( 'NONE',  ( 22.52576749827964520, 6.809805260274345962, -73.19476423806628418 ) ) ;
#13625=ORIENTED_EDGE ( 'NONE', *, *, #61830, .T. ) ;
#13628=CARTESIAN_POINT ( 'NONE',  ( -76.78104518372333587, 22.68568622761702613, -49.89015923587386681 ) ) ;
#13632=CARTESIAN_POINT ( 'NONE',  ( 212.0104729185451902, 118.7959000526603006, -68.97424183727284230 ) ) ;
#13636=CARTESIAN_POINT ( 'NONE',  ( 133.8566784816069060, 42.60093787723652525, 44.51034083899536142 ) ) ;
#13637=CARTESIAN_POINT ( 'NONE',  ( 117.4806398654733783, 33.50379325299404343, 35.07699718365589803 ) ) ;
#13642=CARTESIAN_POINT ( 'NONE',  ( -148.0058283997321382, 64.22864592525513672, -22.81961389825241682 ) ) ;
#13646=FACE_OUTER_BOUND ( 'NONE', #5556, .T. ) ;
#13647=CARTESIAN_POINT ( 'NONE',  ( -144.9439644317224349, 60.40328483334189258, 32.26430146232742402 ) ) ;
#13648=EDGE_CURVE ( 'NONE', #34548, #37698, #38722, .T. ) ;
#13649=CARTESIAN_POINT ( 'NONE',  ( -133.3765738414514885, 51.62252165471728915, 65.54115532702775226 ) ) ;
#13650=CARTESIAN_POINT ( 'NONE',  ( -165.7689197919844730, 79.30072199592272852, -67.54572964526467160 ) ) ;
#13655=CARTESIAN_POINT ( 'NONE',  ( 38.42020198992005220, 8.283430712587444233, 29.96235999322596300 ) ) ;
#13657=ORIENTED_EDGE ( 'NONE', *, *, #24309, .F. ) ;
#13659=B_SPLINE_CURVE_WITH_KNOTS ( 'NONE', 3,
 ( #26867, #41329, #36394, #9665, #57504, #20211, #15283, #36742, #9312, #31460, #21245, #20543, #31127, #26179, #68408, #47615, #63470, #25508, #58865, #20902, #63124, #42693, #41667, #57846, #15965, #52895, #62784, #15626, #14588, #53582, #42356, #68071, #63815, #37076, #36048, #52219 ),
 .UNSPECIFIED., .F., .F.,
 ( 4, 2, 2, 2, 2, 2, 2, 2, 2, 2, 2, 2, 2, 2, 2, 2, 2, 4 ),
 ( 0.000000000000000000, 0.001545474820159029039, 0.003090949640318058078, 0.004636424460477087985, 0.006181899280636116156, 0.007727374100795145195, 0.008500111510874661450, 0.009272848920954175969, 0.01081832374111321542, 0.01236379856127225139, 0.01390927338143128911, 0.01545474820159032682, 0.01700022302174936453, 0.01854569784190840051, 0.02009117266206743996, 0.02163664748222647594, 0.02318212230238551191, 0.02472759712254454789 ),
 .UNSPECIFIED. ) ;
#13663=CARTESIAN_POINT ( 'NONE',  ( 32.56927464314650678, 7.618924692399907883, 7.466848099861418397 ) ) ;
#13664=CARTESIAN_POINT ( 'NONE',  ( -10.24974837193994404, 8.069704751038624835, -35.80395452523003996 ) ) ;
#13668=CARTESIAN_POINT ( 'NONE',  ( -109.4756385662671221, 36.58892558929082384, -94.07530769078934441 ) ) ;
#13675=CARTESIAN_POINT ( 'NONE',  ( 153.4509883044095773, 55.84811350575044742, -76.80503978816277311 ) ) ;
#13676=CARTESIAN_POINT ( 'NONE',  ( -33.13098007862451055, 9.875138601866705557, 45.02716274319689660 ) ) ;
#13677=CARTESIAN_POINT ( 'NONE',  ( 134.3172730033263065, 41.70277427218488953, -36.02331093239567394 ) ) ;
#13681=CARTESIAN_POINT ( 'NONE',  ( -156.0204364459164594, 71.27041535366184632, 68.79358406586271713 ) ) ;
#13682=EDGE_CURVE ( 'NONE', #275, #63707, #43681, .T. ) ;
#13684=CARTESIAN_POINT ( 'NONE',  ( -121.1775535805057444, 43.46577565517550568, 43.97189950139811287 ) ) ;
#13685=CARTESIAN_POINT ( 'NONE',  ( -60.97727891098336528, 16.35024395194892577, -47.34151352721814021 ) ) ;
#13687=CARTESIAN_POINT ( 'NONE',  ( -179.8926034784145429, 96.58272071140103776, -72.29268138171191538 ) ) ;
#13691=CARTESIAN_POINT ( 'NONE',  ( 110.2429982417149290, 28.88204397445231209, 29.61121420573730489 ) ) ;
#13693=CARTESIAN_POINT ( 'NONE',  ( 92.32928948494030408, 21.44473173578322545, -92.06573559034401910 ) ) ;
#13698=CARTESIAN_POINT ( 'NONE',  ( 117.7447573007802788, 32.50990724960315958, -69.77678085006658648 ) ) ;
#13699=CARTESIAN_POINT ( 'NONE',  ( 65.40032188136231639, 13.23841673691966747, 57.04257784809311715 ) ) ;
#13700=CARTESIAN_POINT ( 'NONE',  ( 136.9822423813093337, 44.53121110416872597, 3.344055275432845420 ) ) ;
#13702=AXIS2_PLACEMENT_3D ( 'NONE', #66154, #60846, #17230 ) ;
#13703=ORIENTED_EDGE ( 'NONE', *, *, #37624, .F. ) ;
#13707=CARTESIAN_POINT ( 'NONE',  ( 137.2430147073457931, 43.50693516253637227, 83.99996777949063187 ) ) ;
#13709=CARTESIAN_POINT ( 'NONE',  ( -142.0685766576042113, 58.11789490499572963, -68.04818472065136348 ) ) ;
#13710=LINE ( 'NONE', #63886, #21239 ) ;
#13712=CARTESIAN_POINT ( 'NONE',  ( 164.8886903222557407, 63.65672212134879260, -44.76364719617309618 ) ) ;
#13715=CARTESIAN_POINT ( 'NONE',  ( -102.2801239173131052, 33.91021738430207222, 18.67452391595144334 ) ) ;
#13716=CARTESIAN_POINT ( 'NONE',  ( 204.6977192012829789, -170.0000000000000000, 44.20772073876944575 ) ) ;
#13719=DIRECTION ( 'NONE',  ( 0.000000000000000000, 0.000000000000000000, 1.000000000000000000 ) ) ;
#13720=CARTESIAN_POINT ( 'NONE',  ( -165.6393662153604964, 79.16886183052817216, 38.92739272313387033 ) ) ;
#13721=CARTESIAN_POINT ( 'NONE',  ( -142.1450925953585340, 58.17784622801090677, -94.47787185721898595 ) ) ;
#13725=CARTESIAN_POINT ( 'NONE',  ( -14.84903512415885452, 8.461292896365067762, 67.10196148585319520 ) ) ;
#13726=ORIENTED_EDGE ( 'NONE', *, *, #2103, .F. ) ;
#13728=CARTESIAN_POINT ( 'NONE',  ( -154.6085044440278864, 69.98390342970671441, -47.81608844076072273 ) ) ;
#13729=CARTESIAN_POINT ( 'NONE',  ( 211.5034924207028553, 118.0100795718635283, -13.81556118458025395 ) ) ;
#13731=CARTESIAN_POINT ( 'NONE',  ( -4.731197926646205865, 7.716745361328039898, 30.77918364689588415 ) ) ;
#13733=CARTESIAN_POINT ( 'NONE',  ( -51.77439426130688105, 13.82695438436704016, -62.81093775181126659 ) ) ;
#13734=ADVANCED_FACE ( 'NONE', ( #37247 ), #48140, .F. ) ;
#13735=CARTESIAN_POINT ( 'NONE',  ( 207.4696221732442893, 110.2206209205162111, -50.80684766909965333 ) ) ;
#13736=AXIS2_PLACEMENT_3D ( 'NONE', #48445, #36896, #20713 ) ;
#13738=CARTESIAN_POINT ( 'NONE',  ( 110.7164744784863757, 29.10110206241301611, 17.76666361527367499 ) ) ;
#13741=CARTESIAN_POINT ( 'NONE',  ( -102.2801239173131194, 33.91021738430207222, -35.01457726497591239 ) ) ;
#13745=CARTESIAN_POINT ( 'NONE',  ( 41.09759788073306908, 9.651672055033841957, -8.965407513425770247 ) ) ;
#13747=CARTESIAN_POINT ( 'NONE',  ( -173.1211646369891071, 87.12891641440859303, 18.97714401617737678 ) ) ;
#13748=CARTESIAN_POINT ( 'NONE',  ( -13.57610226747640425, 7.333588782202060230, 86.44604924231978771 ) ) ;
#13749=CARTESIAN_POINT ( 'NONE',  ( -105.4487797565983982, 35.55724615608641415, -22.48385247276568677 ) ) ;
#13750=DIRECTION ( 'NONE',  ( 0.000000000000000000, 0.000000000000000000, 1.000000000000000000 ) ) ;
#13751=CARTESIAN_POINT ( 'NONE',  ( -165.9992860119574232, 79.53569239468046703, 62.79718458295194239 ) ) ;
#13756=CARTESIAN_POINT ( 'NONE',  ( 174.9042454172879673, 72.57746269938724026, -12.60028719114147400 ) ) ;
#13757=CARTESIAN_POINT ( 'NONE',  ( 103.0004140566503281, 26.76634862952790428, 65.96999840838908824 ) ) ;
#13760=EDGE_LOOP ( 'NONE', ( #4452, #14809, #29639, #56992 ) ) ;
#13764=CARTESIAN_POINT ( 'NONE',  ( 22.90619343622340054, 7.840927939412482672, -45.43282700353950077 ) ) ;
#13765=CARTESIAN_POINT ( 'NONE',  ( 8.337549025192450003, 7.382630697225773808, 63.37153782633733812 ) ) ;
#13767=FACE_BOUND ( 'NONE', #550, .T. ) ;
#13769=EDGE_LOOP ( 'NONE', ( #14270, #12142 ) ) ;
#13775=CARTESIAN_POINT ( 'NONE',  ( -173.1211646369891355, -170.0000000000000000, 57.66624519710472185 ) ) ;
#13776=CARTESIAN_POINT ( 'NONE',  ( 13.52497250360456782, 6.438709070458922490, 84.04600024306211026 ) ) ;
#13777=CARTESIAN_POINT ( 'NONE',  ( 82.94943325692331371, 18.19803534719806137, -76.70580516979920560 ) ) ;
#13785=ORIENTED_EDGE ( 'NONE', *, *, #7224, .T. ) ;
#13786=CARTESIAN_POINT ( 'NONE',  ( -80.54757501605354264, 23.04700348514567665, -62.19583100815920318 ) ) ;
#13789=CARTESIAN_POINT ( 'NONE',  ( 94.06699947028482711, 23.17027898120150198, -71.16360367612234938 ) ) ;
#13792=CARTESIAN_POINT ( 'NONE',  ( 46.65974587859240330, 10.48396258569371398, 62.30449875318643649 ) ) ;
#13794=CARTESIAN_POINT ( 'NONE',  ( 103.0004140566503281, 26.76634862952790428, 12.28089722746173429 ) ) ;
#13795=ORIENTED_EDGE ( 'NONE', *, *, #49680, .F. ) ;
#13798=CARTESIAN_POINT ( 'NONE',  ( 177.7964363391244831, 76.75162026635257462, -77.32570004121048157 ) ) ;
#13800=CARTESIAN_POINT ( 'NONE',  ( 113.4493678088378630, 30.39339414805074213, -9.781423810587101642 ) ) ;
#13801=CARTESIAN_POINT ( 'NONE',  ( 79.22872707466396491, 18.07970189365808977, -42.07899737201626778 ) ) ;
#13805=CARTESIAN_POINT ( 'NONE',  ( 86.62931800182293784, 19.42108912189596381, -77.66611478937542756 ) ) ;
#13806=CARTESIAN_POINT ( 'NONE',  ( -78.66644367742111399, -170.0000000000000000, 57.26275173013680586 ) ) ;
#13808=CARTESIAN_POINT ( 'NONE',  ( -188.6739852773920063, 108.2139733222100375, -16.97215699203637129 ) ) ;
#13809=CARTESIAN_POINT ( 'NONE',  ( 127.6144785300460711, 37.78099129859916161, 6.000583388021733633 ) ) ;
#13812=CARTESIAN_POINT ( 'NONE',  ( 212.1393014306632381, 118.9967099399321881, 89.43627726685924983 ) ) ;
#13813=LINE ( 'NONE', #52143, #673 ) ;
#13815=CARTESIAN_POINT ( 'NONE',  ( -8.314575874103544706, 6.922894809783090686, 30.11558103944717857 ) ) ;
#13818=CARTESIAN_POINT ( 'NONE',  ( 8.683910719548897816, 7.383368463746303512, -18.59074450809671930 ) ) ;
#13819=ORIENTED_EDGE ( 'NONE', *, *, #42060, .F. ) ;
#13821=CARTESIAN_POINT ( 'NONE',  ( -102.2801239173131194, -170.0000000000000000, -42.51457726497592660 ) ) ;
#13827=CARTESIAN_POINT ( 'NONE',  ( -36.19950032668960205, 11.44450118435070429, 85.60097597857388507 ) ) ;
#13828=CARTESIAN_POINT ( 'NONE',  ( 157.4703587214989398, -170.0000000000000000, -89.81328548006499091 ) ) ;
#13829=CARTESIAN_POINT ( 'NONE',  ( 37.46254810722764717, 8.164772623042706456, -50.38115373914292405 ) ) ;
#13837=CARTESIAN_POINT ( 'NONE',  ( 185.8199718667679861, 85.00425737502088452, 84.67356966130316209 ) ) ;
#13839=CARTESIAN_POINT ( 'NONE',  ( 133.8566784816069344, -170.0000000000000000, -51.02331093239568816 ) ) ;
#13840=CARTESIAN_POINT ( 'NONE',  ( -25.35398647985413945, 8.671412257862213480, -74.05290484057726985 ) ) ;
#13845=CARTESIAN_POINT ( 'NONE',  ( -56.72676045871359207, 16.18052435693491375, -76.87568460535000270 ) ) ;
#13846=CARTESIAN_POINT ( 'NONE',  ( 178.1999009735082211, 75.73911533785327777, -63.64278916692260424 ) ) ;
#13850=CARTESIAN_POINT ( 'NONE',  ( -23.93933407965395688, 9.495050561681670942, 65.05660416612819574 ) ) ;
#13854=CARTESIAN_POINT ( 'NONE',  ( -4.513903087372272971, 6.697902023160579255, 57.72633437538576118 ) ) ;
#13857=CARTESIAN_POINT ( 'NONE',  ( 157.0357419681844533, 58.58786672900118475, 56.26341910979446936 ) ) ;
#13858=CARTESIAN_POINT ( 'NONE',  ( -108.6944271866238978, 37.30738480893075604, -65.44042506789568847 ) ) ;
#13864=ORIENTED_EDGE ( 'NONE', *, *, #18055, .F. ) ;
#13865=EDGE_LOOP ( 'NONE', ( #57816, #11038, #18027, #22306 ) ) ;
#13867=CARTESIAN_POINT ( 'NONE',  ( 180.6710448012268841, 78.18844465372403363, -51.22505766587963905 ) ) ;
#13868=CARTESIAN_POINT ( 'NONE',  ( 150.2941978382489481, 53.52137138947628614, 34.71248029558645953 ) ) ;
#13869=DIRECTION ( 'NONE',  ( -0.000000000000000000, 1.000000000000000000, -0.000000000000000000 ) ) ;
#13870=ORIENTED_EDGE ( 'NONE', *, *, #2613, .T. ) ;
#13871=CARTESIAN_POINT ( 'NONE',  ( 151.3976820382521851, 54.32583990172415156, 94.99999999999866418 ) ) ;
#13872=CARTESIAN_POINT ( 'NONE',  ( -180.6213815675304488, 95.88446356933840775, 11.16758809461633462 ) ) ;
#13875=CARTESIAN_POINT ( 'NONE',  ( -83.15209219203883606, 25.16621997697722435, 43.94856979754528226 ) ) ;
#13876=CARTESIAN_POINT ( 'NONE',  ( -24.60892750534350171, 9.584951112520229799, -19.08067319542340812 ) ) ;
#13888=LINE ( 'NONE', #8275, #7973 ) ;
#13889=DIRECTION ( 'NONE',  ( -0.000000000000000000, 0.000000000000000000, -1.000000000000000000 ) ) ;
#13892=CARTESIAN_POINT ( 'NONE',  ( 79.22946426532584496, 17.02750615740070828, -44.56886393397318358 ) ) ;
#13897=CARTESIAN_POINT ( 'NONE',  ( 79.33384730094452664, 18.11203072455028007, 35.45442786235279442 ) ) ;
#13900=CARTESIAN_POINT ( 'NONE',  ( -122.3745688183166180, 44.21964839958059912, 71.60445237168489996 ) ) ;
#13901=CARTESIAN_POINT ( 'NONE',  ( -82.32006615997345023, 24.83050031643764655, -22.33869602845198798 ) ) ;
#13902=CARTESIAN_POINT ( 'NONE',  ( -177.5288247523078837, 93.72924674643516596, -9.281560969338585210 ) ) ;
#13904=ORIENTED_EDGE ( 'NONE', *, *, #65793, .F. ) ;
#13907=ORIENTED_EDGE ( 'NONE', *, *, #50211, .T. ) ;
#13910=DIRECTION ( 'NONE',  ( -0.000000000000000000, 1.000000000000000000, -0.000000000000000000 ) ) ;
#13911=CARTESIAN_POINT ( 'NONE',  ( 160.9069879467680551, 60.37290772564307417, 57.07157262504325956 ) ) ;
#13912=CARTESIAN_POINT ( 'NONE',  ( -189.7334103489409927, 107.7745063523401399, 62.57085666808671931 ) ) ;
#13914=CARTESIAN_POINT ( 'NONE',  ( 18.66025561752211104, 6.609375019058817635, 30.57350750057610256 ) ) ;
#13915=CARTESIAN_POINT ( 'NONE',  ( 164.9697211531229755, 63.72502658717164792, -70.76554158249184923 ) ) ;
#13920=CARTESIAN_POINT ( 'NONE',  ( -73.37368996857509273, 20.37564829273156164, 86.28413825297953110 ) ) ;
#13921=CARTESIAN_POINT ( 'NONE',  ( -81.01337222286377937, 23.22902179892323460, 57.62334405355243661 ) ) ;
#13922=CARTESIAN_POINT ( 'NONE',  ( 67.93926590385567010, 13.86859831467923421, -37.54205066259513046 ) ) ;
#13924=CARTESIAN_POINT ( 'NONE',  ( -61.10880364359508832, 17.43879918625642489, 33.38610393800483678 ) ) ;
#13926=CARTESIAN_POINT ( 'NONE',  ( -32.41898580403140784, 10.77423026598438227, -62.20981738725323140 ) ) ;
#13928=CARTESIAN_POINT ( 'NONE',  ( 55.57634120535662703, 12.09544293553732608, 38.29713233239909442 ) ) ;
#13929=CARTESIAN_POINT ( 'NONE',  ( 35.91764385665408099, 7.981776510761975807, 84.45325133309545151 ) ) ;
#13932=DIRECTION ( 'NONE',  ( 0.000000000000000000, 0.000000000000000000, 1.000000000000000000 ) ) ;
#13934=CARTESIAN_POINT ( 'NONE',  ( -118.9649285217355725, 42.09781191014328527, 8.393151206171708623 ) ) ;
#13937=CARTESIAN_POINT ( 'NONE',  ( 18.20314211955701467, 7.596739727129572017, -23.29199594580876820 ) ) ;
#13942=B_SPLINE_CURVE_WITH_KNOTS ( 'NONE', 3,
 ( #55476, #22775, #44926, #50554, #28397, #66753, #39311, #44218, #55838, #50207, #60755, #12576, #13278, #2033, #33345, #34036, #65344, #2372, #55123, #23487 ),
 .UNSPECIFIED., .F., .F.,
 ( 4, 2, 2, 2, 2, 2, 2, 2, 2, 4 ),
 ( 0.01088281063028401045, 0.01226892151836797562, 0.01365503240645193905, 0.01504114329453590422, 0.01642725418261986939, 0.01781336507070383282, 0.01919947595878779972, 0.02058558684687176316, 0.02127864229091375528, 0.02197169773495574741 ),
 .UNSPECIFIED. ) ;
#13946=CARTESIAN_POINT ( 'NONE',  ( -36.37229078872274357, 11.47648211215765812, -48.48744179093426965 ) ) ;
#13952=CARTESIAN_POINT ( 'NONE',  ( -29.51060362117876323, 9.282716514427253429, -23.22459071689376486 ) ) ;
#13953=CARTESIAN_POINT ( 'NONE',  ( -125.8938041572051389, 47.69968343338780414, -61.75825448869760237 ) ) ;
#13954=ORIENTED_EDGE ( 'NONE', *, *, #49945, .T. ) ;
#13955=CARTESIAN_POINT ( 'NONE',  ( 164.7561380852247055, 64.86195321300263572, 92.41705344553244572 ) ) ;
#13957=CARTESIAN_POINT ( 'NONE',  ( 126.6464677212869248, 38.39096133771044350, -72.49914021808577047 ) ) ;
#13958=CARTESIAN_POINT ( 'NONE',  ( 132.9485794245231318, 40.87843215479636427, 44.46890670783304955 ) ) ;
#13965=CARTESIAN_POINT ( 'NONE',  ( 56.66775172211441003, 11.28938863449062779, 41.31488029608967594 ) ) ;
#13969=CARTESIAN_POINT ( 'NONE',  ( -165.6215009671261100, 80.58889799860440917, 11.79125241431325399 ) ) ;
#13972=CARTESIAN_POINT ( 'NONE',  ( -32.50312470669472731, 10.78887528550998276, -89.07914025037321437 ) ) ;
#13974=CARTESIAN_POINT ( 'NONE',  ( -132.0870433264402948, 51.94057326482882786, 69.20208566340080836 ) ) ;
#13978=CARTESIAN_POINT ( 'NONE',  ( -73.10086105983762650, 21.34631349770503306, -37.56410186751649860 ) ) ;
#13984=CARTESIAN_POINT ( 'NONE',  ( -173.1211646369891355, -170.0000000000000000, 11.47714401617735902 ) ) ;
#13988=CARTESIAN_POINT ( 'NONE',  ( 67.55199883153193241, 14.80832170058781472, -76.05753081593569220 ) ) ;
#13989=EDGE_CURVE ( 'NONE', #55679, #49789, #56284, .T. ) ;
#13992=CARTESIAN_POINT ( 'NONE',  ( -143.8634661037141029, 60.82480701605699380, -20.43370834467151198 ) ) ;
#13995=CARTESIAN_POINT ( 'NONE',  ( -54.62534944479597954, 14.56729055894799529, -88.91457369577481984 ) ) ;
#14000=CARTESIAN_POINT ( 'NONE',  ( -166.5704851812740799, 80.12110537694672985, -72.71914147894192126 ) ) ;
#14001=ORIENTED_EDGE ( 'NONE', *, *, #63614, .T. ) ;
#14005=CARTESIAN_POINT ( 'NONE',  ( 80.73462811483979351, 18.54763808182591944, 59.39265946625696557 ) ) ;
#14011=CARTESIAN_POINT ( 'NONE',  ( 31.95008798096002423, 7.556925044648910905, 11.55179525732833845 ) ) ;
#14012=DIRECTION ( 'NONE',  ( 0.000000000000000000, 0.000000000000000000, 1.000000000000000000 ) ) ;
#14015=CARTESIAN_POINT ( 'NONE',  ( -149.5074843970971017, 65.50121172469319220, 45.72082123989907387 ) ) ;
#14016=VERTEX_POINT ( 'NONE', #19976 ) ;
#14018=CARTESIAN_POINT ( 'NONE',  ( -59.57462349605614804, 16.98779896904798647, 58.65824683570725284 ) ) ;
#14019=CARTESIAN_POINT ( 'NONE',  ( -29.51060362117876679, 9.282716514427262311, 3.619959873569910336 ) ) ;
#14022=CARTESIAN_POINT ( 'NONE',  ( -13.78709718204648560, 7.352743657744184702, -74.33944143250060677 ) ) ;
#14024=CARTESIAN_POINT ( 'NONE',  ( -25.48237668717800375, 8.689083390666786144, 69.14452889623510146 ) ) ;
#14025=AXIS2_PLACEMENT_3D ( 'NONE', #14933, #69434, #47969 ) ;
#14032=CARTESIAN_POINT ( 'NONE',  ( -173.9617926765114362, 89.58633395456780590, -61.59193146985943201 ) ) ;
#14037=CARTESIAN_POINT ( 'NONE',  ( 117.6865880453675999, 32.48051379280605033, 36.05596251868298907 ) ) ;
#14039=CARTESIAN_POINT ( 'NONE',  ( 89.74347354996881165, 20.50579948213362869, -90.14040706678140680 ) ) ;
#14043=CARTESIAN_POINT ( 'NONE',  ( 201.6034029841262338, 102.1956603101140928, 43.55317564153742182 ) ) ;
#14044=CARTESIAN_POINT ( 'NONE',  ( 115.0692128464502701, 31.17922615202199310, -64.50543960138530508 ) ) ;
#14045=CARTESIAN_POINT ( 'NONE',  ( 69.08240197259640070, 14.16210831900843203, 59.74101951860149740 ) ) ;
#14046=CARTESIAN_POINT ( 'NONE',  ( 140.7888851157410102, 46.97220912571250295, 13.04025809958710624 ) ) ;
#14049=CARTESIAN_POINT ( 'NONE',  ( 164.9706294237033717, 65.04392654036658428, -17.05375542338060413 ) ) ;
#14053=CARTESIAN_POINT ( 'NONE',  ( 130.0022568700022703, 39.14528604308903681, 84.25756070950254184 ) ) ;
#14056=CARTESIAN_POINT ( 'NONE',  ( -149.0732005398558613, 63.81212100765655748, -61.66682328262454860 ) ) ;
#14057=EDGE_CURVE ( 'NONE', #40816, #25434, #41220, .T. ) ;
#14059=CARTESIAN_POINT ( 'NONE',  ( 164.7250737226289630, 63.51898362052163804, -41.70171562401918663 ) ) ;
#14062=CARTESIAN_POINT ( 'NONE',  ( 56.33018609834994095, 12.24748093153179518, 94.41788745877084921 ) ) ;
#14065=CARTESIAN_POINT ( 'NONE',  ( 86.14890207173843351, 20.31981596387580424, -8.977013608448027426 ) ) ;
#14067=DIRECTION ( 'NONE',  ( 0.000000000000000000, 0.000000000000000000, 1.000000000000000000 ) ) ;
#14068=CARTESIAN_POINT ( 'NONE',  ( 181.0840389613909736, 80.03940679743415387, 44.30859410551141764 ) ) ;
#14070=EDGE_LOOP ( 'NONE', ( #29464, #33859, #68811, #12520 ) ) ;
#14071=CARTESIAN_POINT ( 'NONE',  ( -97.86516199987804043, 31.71158167298307617, 58.78184745139680700 ) ) ;
#14072=DIRECTION ( 'NONE',  ( -0.000000000000000000, 1.000000000000000000, -0.000000000000000000 ) ) ;
#14077=CARTESIAN_POINT ( 'NONE',  ( 150.5538013146980347, 53.70974888488127164, -13.86729835050963899 ) ) ;
#14081=CARTESIAN_POINT ( 'NONE',  ( 102.7414208686707724, 26.65627265923299660, 37.60061438686749113 ) ) ;
#14082=CARTESIAN_POINT ( 'NONE',  ( -4.506365319453810692, 7.705038994660847074, 30.88546273271729348 ) ) ;
#14083=CARTESIAN_POINT ( 'NONE',  ( 55.82071269177104256, 11.11819622756448034, 88.85841515383880562 ) ) ;
#14084=CARTESIAN_POINT ( 'NONE',  ( -50.14771795543004629, 13.42081263859818385, -75.25552575325329485 ) ) ;
#14086=AXIS2_PLACEMENT_3D ( 'NONE', #58182, #48630, #21241 ) ;
#14087=FACE_OUTER_BOUND ( 'NONE', #3242, .T. ) ;
#14088=CARTESIAN_POINT ( 'NONE',  ( -62.15324028806259093, 16.70091357159900980, 13.43818584318690057 ) ) ;
#14092=CARTESIAN_POINT ( 'NONE',  ( 102.8518012651273779, 25.61025413220827929, -68.96863170923236908 ) ) ;
#14094=CARTESIAN_POINT ( 'NONE',  ( 42.49453823366106064, 8.831814337191476127, 71.09543012908832793 ) ) ;
#14096=CARTESIAN_POINT ( 'NONE',  ( -8.157890479254499283, 6.912699202480759197, 83.80498378616138666 ) ) ;
#14097=CARTESIAN_POINT ( 'NONE',  ( -107.7886332494339712, 36.81249801143974310, -10.55694427585111050 ) ) ;
#14098=VERTEX_POINT ( 'NONE', #26282 ) ;
#14101=EDGE_LOOP ( 'NONE', ( #13131, #46819 ) ) ;
#14103=CARTESIAN_POINT ( 'NONE',  ( -155.7433525314458791, 69.65452735858369238, 42.39591026950624553 ) ) ;
#14105=CARTESIAN_POINT ( 'NONE',  ( 179.0096185093688064, 76.53352131383245194, -24.10098174011748640 ) ) ;
#14106=CARTESIAN_POINT ( 'NONE',  ( 107.0555969502564153, 28.53646637607231540, 57.15036769607191758 ) ) ;
#14108=CARTESIAN_POINT ( 'NONE',  ( 55.51528220483959331, 12.08323518953685749, -16.13771739302386621 ) ) ;
#14110=CARTESIAN_POINT ( 'NONE',  ( 107.2614272668149056, 28.62909081796205513, -36.53649460854888531 ) ) ;
#14111=VERTEX_POINT ( 'NONE', #22034 ) ;
#14112=CARTESIAN_POINT ( 'NONE',  ( 210.1633650091869470, 114.1507944623966893, 4.721410748252139911 ) ) ;
#14113=CARTESIAN_POINT ( 'NONE',  ( 8.763528846667103522, 7.383598436776579454, 66.99810038742778318 ) ) ;
#14114=CARTESIAN_POINT ( 'NONE',  ( 208.9507214515059843, 112.3605999017434982, 30.51409441703008696 ) ) ;
#14116=FACE_BOUND ( 'NONE', #33499, .T. ) ;
#14122=CARTESIAN_POINT ( 'NONE',  ( -123.1629650876958948, 45.91644518770717553, 84.79916741339407338 ) ) ;
#14126=CARTESIAN_POINT ( 'NONE',  ( 8.970976835706142793, 6.378128542324178696, 88.06027136665343846 ) ) ;
#14127=CARTESIAN_POINT ( 'NONE',  ( 79.22946426532585917, 17.02750615740070828, -71.41341452443687388 ) ) ;
#14129=VECTOR ( 'NONE', #56423, 1000.000000000000000 ) ;
#14134=CARTESIAN_POINT ( 'NONE',  ( 198.8732368717152212, 100.3103976497390732, -39.09420075645709858 ) ) ;
#14139=CARTESIAN_POINT ( 'NONE',  ( -85.75947274862029701, 25.15128705015480293, -71.94837500685306964 ) ) ;
#14141=EDGE_LOOP ( 'NONE', ( #60507, #29407 ) ) ;
#14144=CARTESIAN_POINT ( 'NONE',  ( 46.89016064832839703, 10.52130577388959409, 63.77019485676617450 ) ) ;
#14147=CARTESIAN_POINT ( 'NONE',  ( 102.7938674513919040, 26.67851209377772292, 11.27790700381929945 ) ) ;
#14149=CARTESIAN_POINT ( 'NONE',  ( -28.92901790436172149, 9.192688694475796396, 84.33077190568265280 ) ) ;
#14152=CARTESIAN_POINT ( 'NONE',  ( 109.3079614081140249, 28.45126415661782460, -35.96632621749219538 ) ) ;
#14154=CARTESIAN_POINT ( 'NONE',  ( 163.5430354047457229, 62.53125887746119105, 94.99999999999866418 ) ) ;
#14157=ADVANCED_FACE ( 'NONE', ( #64603 ), #5846, .F. ) ;
#14159=EDGE_CURVE ( 'NONE', #16864, #32664, #25286, .T. ) ;
#14161=CARTESIAN_POINT ( 'NONE',  ( 43.35980717318837918, 8.957244490220908517, 16.94469360157332360 ) ) ;
#14165=CARTESIAN_POINT ( 'NONE',  ( 128.0848616812662897, 38.04676222636084049, 14.98112062868012906 ) ) ;
#14168=CARTESIAN_POINT ( 'NONE',  ( 212.1976655298228138, 119.0878071902807562, 36.52985908372631485 ) ) ;
#14169=CARTESIAN_POINT ( 'NONE',  ( -74.79002408692173276, 20.88280597089421775, -63.03483985874790108 ) ) ;
#14170=CARTESIAN_POINT ( 'NONE',  ( -108.6909373351217596, 36.15835109565443162, 34.09471970242879735 ) ) ;
#14175=CARTESIAN_POINT ( 'NONE',  ( 197.1974290009105175, 96.59277840252782710, -17.30540446041513292 ) ) ;
#14179=CARTESIAN_POINT ( 'NONE',  ( 186.2575601542430661, 85.47765906955508797, -65.13421257721934410 ) ) ;
#14180=CARTESIAN_POINT ( 'NONE',  ( -143.8756912989387047, 60.83492035645719653, 70.02464342104502748 ) ) ;
#14181=CARTESIAN_POINT ( 'NONE',  ( -96.76159256735191150, 30.06445763698411611, -37.41197554230570432 ) ) ;
#14184=CARTESIAN_POINT ( 'NONE',  ( 37.47081272996200596, 8.166145978397521432, -35.86855199365803060 ) ) ;
#14185=CARTESIAN_POINT ( 'NONE',  ( -105.8879439778144587, 34.65133284149109727, 4.582014221861286707 ) ) ;
#14186=CARTESIAN_POINT ( 'NONE',  ( 86.62931800182293784, -170.0000000000000000, 10.36753698201563267 ) ) ;
#14191=AXIS2_PLACEMENT_3D ( 'NONE', #51102, #46154, #19081 ) ;
#14193=CARTESIAN_POINT ( 'NONE',  ( 187.5460976208452735, 86.88588274757240981, 86.67476712161497687 ) ) ;
#14196=CARTESIAN_POINT ( 'NONE',  ( -30.94753041835916108, 9.510749728915508072, -62.16174795566552547 ) ) ;
#14201=CARTESIAN_POINT ( 'NONE',  ( 173.9288990958749537, 71.66475105971930759, -68.24753224134477136 ) ) ;
#14204=CARTESIAN_POINT ( 'NONE',  ( -169.8791831685529701, 83.59058982490282119, 18.25486782800532382 ) ) ;
#14206=B_SPLINE_CURVE_WITH_KNOTS ( 'NONE', 3,
 ( #5951, #18874, #37977, #43930, #694, #16858, #65411, #38315, #59761, #11575, #33050, #54486, #6311, #17202, #25883, #58226, #41370, #30814, #57884, #4082, #63170, #24512, #19204, #63507, #62117, #62823, #30129, #19915, #62474, #9703, #51580, #31498, #56857, #14290, #14964, #40664, #35397, #8675, #68441, #31169, #36430, #36090, #67413, #20247, #3387, #67760 ),
 .UNSPECIFIED., .F., .F.,
 ( 4, 2, 2, 2, 2, 2, 2, 2, 2, 2, 2, 2, 2, 2, 2, 2, 2, 2, 2, 2, 2, 2, 4 ),
 ( 3.538155541877297313E-17, 0.001572224531395696864, 0.003144449062791358600, 0.004716673594187020119, 0.006288898125582681638, 0.007861122656978343157, 0.009433347188374003808, 0.01021945945407182199, 0.01100557171976964017, 0.01179168398546745836, 0.01257779625116527654, 0.01415002078256091464, 0.01493613304825873976, 0.01572224531395656488, 0.01650835757965439174, 0.01729446984535221513, 0.01886669437674783414, 0.01965280664244563671, 0.02043891890814343928, 0.02201114343953904443, 0.02358336797093465304, 0.02436948023663245907, 0.02515559250233026858 ),
 .UNSPECIFIED. ) ;
#14207=CARTESIAN_POINT ( 'NONE',  ( -53.13004807512039207, 14.17398740785108302, 71.92754858008906638 ) ) ;
#14209=CARTESIAN_POINT ( 'NONE',  ( -100.6125620134474019, 31.94146452012412141, -88.87928813972597197 ) ) ;
#14210=VERTEX_POINT ( 'NONE', #6899 ) ;
#14213=CARTESIAN_POINT ( 'NONE',  ( -102.7494334820056565, 34.14986869751099618, -61.85912785543958137 ) ) ;
#14215=DIRECTION ( 'NONE',  ( 0.000000000000000000, 0.000000000000000000, 1.000000000000000000 ) ) ;
#14221=ORIENTED_EDGE ( 'NONE', *, *, #63975, .T. ) ;
#14223=ORIENTED_EDGE ( 'NONE', *, *, #42258, .T. ) ;
#14224=CARTESIAN_POINT ( 'NONE',  ( 8.000000000000007105, 249.8719672152120381, 94.99999999999866418 ) ) ;
#14229=DIRECTION ( 'NONE',  ( -0.000000000000000000, 1.000000000000000000, -0.000000000000000000 ) ) ;
#14231=VECTOR ( 'NONE', #40312, 1000.000000000000000 ) ;
#14232=DIRECTION ( 'NONE',  ( 0.000000000000000000, 0.000000000000000000, 1.000000000000000000 ) ) ;
#14233=CARTESIAN_POINT ( 'NONE',  ( -7.336760511143403996, 6.859209474528211281, 3.271030448983516248 ) ) ;
#14236=VECTOR ( 'NONE', #29270, 1000.000000000000000 ) ;
#14237=CARTESIAN_POINT ( 'NONE',  ( 151.9464045465396111, 53.48030587346669762, 85.51384040717854873 ) ) ;
#14238=CARTESIAN_POINT ( 'NONE',  ( 139.1353280997809065, 44.70436000187870462, 15.49914358619959209 ) ) ;
#14246=CARTESIAN_POINT ( 'NONE',  ( -118.3982140490518020, 41.75260250602053702, 91.38396685080842019 ) ) ;
#14250=EDGE_CURVE ( 'NONE', #69029, #13412, #55079, .T. ) ;
#14254=CARTESIAN_POINT ( 'NONE',  ( 199.7278513351970730, 99.76879341361772902, -65.03439541865878937 ) ) ;
#14255=EDGE_CURVE ( 'NONE', #19842, #40675, #7260, .T. ) ;
#14256=CARTESIAN_POINT ( 'NONE',  ( -31.43908319763709969, 10.61114334766716105, 45.21645440618919309 ) ) ;
#14257=CARTESIAN_POINT ( 'NONE',  ( -118.4622862908118748, 41.79153065058245886, 66.01100761066821576 ) ) ;
#14259=CARTESIAN_POINT ( 'NONE',  ( 16.27765348919937338, 6.516472002017812848, -23.67439350822213129 ) ) ;
#14263=CARTESIAN_POINT ( 'NONE',  ( -109.6752351740181695, 37.84903014964773860, 12.45126650322635165 ) ) ;
#14264=CARTESIAN_POINT ( 'NONE',  ( 107.2672065034543181, 27.52931006625851396, 57.06728851299916272 ) ) ;
#14265=CARTESIAN_POINT ( 'NONE',  ( 164.3702714028688376, 63.22112480708619131, 66.70566855636806736 ) ) ;
#14266=CARTESIAN_POINT ( 'NONE',  ( -189.2826425734428426, 107.1493800926105848, 66.14067199168205491 ) ) ;
#14268=DIRECTION ( 'NONE',  ( -1.000000000000000000, 0.000000000000000000, 0.000000000000000000 ) ) ;
#14269=CARTESIAN_POINT ( 'NONE',  ( -142.6736406357357794, 59.87555372585265445, 94.99999999999866418 ) ) ;
#14270=ORIENTED_EDGE ( 'NONE', *, *, #52494, .F. ) ;
#14272=EDGE_LOOP ( 'NONE', ( #39321, #60455 ) ) ;
#14274=AXIS2_PLACEMENT_3D ( 'NONE', #26722, #27050, #42210 ) ;
#14275=CARTESIAN_POINT ( 'NONE',  ( -152.2873556200145231, 67.91256772393731467, -22.43757778285992899 ) ) ;
#14277=CARTESIAN_POINT ( 'NONE',  ( -78.66644367742111399, -170.0000000000000000, -15.77090004125421352 ) ) ;
#14280=CARTESIAN_POINT ( 'NONE',  ( -60.95805269991217301, 17.39401718769329364, 33.18720258285724611 ) ) ;
#14281=CARTESIAN_POINT ( 'NONE',  ( -36.00304714721389132, 11.40794940913600186, -63.69002027861343862 ) ) ;
#14284=CARTESIAN_POINT ( 'NONE',  ( 9.290502160020464473, 6.379616279862541539, -19.92800821493562680 ) ) ;
#14285=VERTEX_POINT ( 'NONE', #60714 ) ;
#14286=CARTESIAN_POINT ( 'NONE',  ( -2.174378755909798233, 6.588636630831477881, -37.96269615286738031 ) ) ;
#14287=CARTESIAN_POINT ( 'NONE',  ( 188.5837490358996433, 86.53279111916958755, 63.34238295915565686 ) ) ;
#14288=CARTESIAN_POINT ( 'NONE',  ( -118.6288898061518324, 41.89286798341290563, 9.393189492624903991 ) ) ;
#14290=CARTESIAN_POINT ( 'NONE',  ( 128.9253503890652723, 38.52561778336674081, -22.33494626306552178 ) ) ;
#14291=CARTESIAN_POINT ( 'NONE',  ( 23.03546163277113124, 7.848986635155159597, -14.22797331585904779 ) ) ;
#14293=CARTESIAN_POINT ( 'NONE',  ( 9.837735240994033958, 7.389327806910500840, 6.098290571077138900 ) ) ;
#14298=CARTESIAN_POINT ( 'NONE',  ( 126.3681350380370958, 38.23508791628619008, -43.03070144732701152 ) ) ;
#14299=CARTESIAN_POINT ( 'NONE',  ( -125.8938041572051105, 46.49392987655494380, -34.91370389823391918 ) ) ;
#14300=CARTESIAN_POINT ( 'NONE',  ( -173.1211646369891355, -170.0000000000000000, -42.21195716474999671 ) ) ;
#14309=ADVANCED_FACE ( 'NONE', ( #45928 ), #8650, .F. ) ;
#14310=CARTESIAN_POINT ( 'NONE',  ( 152.9555868970377617, 55.47759417304577312, 84.60090716898641006 ) ) ;
#14312=CARTESIAN_POINT ( 'NONE',  ( -62.54086041493278714, 17.86944394914988621, 11.46389630284894245 ) ) ;
#14315=CARTESIAN_POINT ( 'NONE',  ( -155.1204242627070471, 70.44799358128194910, 33.24034032259653060 ) ) ;
#14316=CARTESIAN_POINT ( 'NONE',  ( -97.49219489034500441, 30.41416107059313134, 32.22565006754435757 ) ) ;
#14317=FACE_OUTER_BOUND ( 'NONE', #22640, .T. ) ;
#14319=ORIENTED_EDGE ( 'NONE', *, *, #19805, .T. ) ;
#14321=DIRECTION ( 'NONE',  ( 0.000000000000000000, 0.000000000000000000, 1.000000000000000000 ) ) ;
#14325=CARTESIAN_POINT ( 'NONE',  ( 174.4912080999798434, 73.57140295268871455, 40.39465835065680466 ) ) ;
#14327=CARTESIAN_POINT ( 'NONE',  ( -33.53989818724163996, 10.96657222678981647, -89.29382644890102938 ) ) ;
#14329=CARTESIAN_POINT ( 'NONE',  ( -127.6894679065405427, 48.89973668460850575, 72.26033685317716504 ) ) ;
#14330=VERTEX_POINT ( 'NONE', #68424 ) ;
#14331=CARTESIAN_POINT ( 'NONE',  ( -102.0448918136529528, 33.79000532939934942, 84.20608419455113847 ) ) ;
#14336=CARTESIAN_POINT ( 'NONE',  ( -59.57733000654211253, 15.94108165424593082, -21.87290956083888460 ) ) ;
#14339=CARTESIAN_POINT ( 'NONE',  ( 137.4031600461560458, 44.79620770172218158, 30.39764953766911404 ) ) ;
#14340=CARTESIAN_POINT ( 'NONE',  ( 117.0069443446175512, 33.26475960880694061, 40.36144550428178945 ) ) ;
#14341=CARTESIAN_POINT ( 'NONE',  ( -102.2801239173131052, 32.78103895658058065, 3.674523915951417141 ) ) ;
#14342=CARTESIAN_POINT ( 'NONE',  ( -99.98930671699734773, 31.63190627461932891, -76.51612866312223105 ) ) ;
#14343=EDGE_LOOP ( 'NONE', ( #60324, #60855 ) ) ;
#14345=CARTESIAN_POINT ( 'NONE',  ( -143.4048679855201271, 60.45763799613828837, -11.10110644613702213 ) ) ;
#14351=CARTESIAN_POINT ( 'NONE',  ( -148.4259959918497600, 63.26767374754761875, 45.64561139210511698 ) ) ;
#14353=CARTESIAN_POINT ( 'NONE',  ( 208.9507214515059843, 112.3605999017434982, 57.35864500749378436 ) ) ;
#14354=VERTEX_POINT ( 'NONE', #4061 ) ;
#14355=CARTESIAN_POINT ( 'NONE',  ( -103.2164890789475464, 34.39030697009942372, 45.47519882833343985 ) ) ;
#14357=CARTESIAN_POINT ( 'NONE',  ( -38.93922791710217979, 10.94334660650242341, 10.62999269609350073 ) ) ;
#14359=ORIENTED_EDGE ( 'NONE', *, *, #29460, .F. ) ;
#14360=CARTESIAN_POINT ( 'NONE',  ( -82.70370746070747714, 23.90061571611317959, -89.98019051878993935 ) ) ;
#14364=CARTESIAN_POINT ( 'NONE',  ( 35.44781468922823109, 7.928097401423682911, 4.191639090875672657 ) ) ;
#14365=CYLINDRICAL_SURFACE ( 'NONE', #8656, 7.500000000000013323 ) ;
#14366=CARTESIAN_POINT ( 'NONE',  ( -38.93938005333175312, 11.96888249046460473, -15.73295882571353133 ) ) ;
#14370=CARTESIAN_POINT ( 'NONE',  ( -55.05276343752910151, -170.0000000000000000, -96.40542517938723677 ) ) ;
#14374=CARTESIAN_POINT ( 'NONE',  ( -23.93965512371324422, 8.480096402797093091, 10.36685825010890660 ) ) ;
#14377=CARTESIAN_POINT ( 'NONE',  ( -59.62510596525322626, 15.95520351401966863, -90.45643964509370960 ) ) ;
#14378=ADVANCED_FACE ( 'NONE', ( #9683 ), #14947, .T. ) ;
#14379=CARTESIAN_POINT ( 'NONE',  ( -101.3602137809054398, 32.31558061113913283, -23.12788902119873313 ) ) ;
#14381=CARTESIAN_POINT ( 'NONE',  ( 155.7167524447090727, 57.56687707799952136, -36.31862843462141655 ) ) ;
#14384=ORIENTED_EDGE ( 'NONE', *, *, #14057, .T. ) ;
#14388=CARTESIAN_POINT ( 'NONE',  ( 173.8576514579035290, 72.97529922124007840, -14.85231137013811598 ) ) ;
#14389=CARTESIAN_POINT ( 'NONE',  ( -123.6699087229882252, 45.04696784753414818, 30.95361604618596019 ) ) ;
#14393=CARTESIAN_POINT ( 'NONE',  ( -173.1211646369891355, 88.63826465341151106, -76.55650775521370122 ) ) ;
#14394=CARTESIAN_POINT ( 'NONE',  ( 131.4581049088925511, 41.16307974347478904, 83.58612097971699484 ) ) ;
#14395=CARTESIAN_POINT ( 'NONE',  ( 110.7164744784864325, 29.10110206241302677, 44.61121420573734753 ) ) ;
#14400=CARTESIAN_POINT ( 'NONE',  ( 200.4600337307566349, 100.7087439352121265, 42.91312774902829830 ) ) ;
#14401=CARTESIAN_POINT ( 'NONE',  ( 110.7114632166112216, 29.09878355652111637, -77.76698815611742077 ) ) ;
#14402=CARTESIAN_POINT ( 'NONE',  ( 181.9411407973025234, 80.91291802046384873, 44.30859410551142474 ) ) ;
#14403=CARTESIAN_POINT ( 'NONE',  ( 137.4031600461560458, 44.79620770172221000, 3.553098947205445501 ) ) ;
#14406=CARTESIAN_POINT ( 'NONE',  ( 164.0073343966822392, 64.23003864582454980, -13.09387731840895164 ) ) ;
#14408=CARTESIAN_POINT ( 'NONE',  ( 70.41705859591012029, 15.55317472777717747, 62.92014748638126775 ) ) ;
#14409=CARTESIAN_POINT ( 'NONE',  ( 127.5859662773347054, 37.76488191276836659, 86.57016596594176860 ) ) ;
#14411=ORIENTED_EDGE ( 'NONE', *, *, #62422, .F. ) ;
#14412=CARTESIAN_POINT ( 'NONE',  ( 161.7031777507226593, 62.31724004902780223, -37.41578519910148515 ) ) ;
#14414=CARTESIAN_POINT ( 'NONE',  ( 160.5141379054753941, 60.05651755415394888, -36.75489487743244865 ) ) ;
#14416=CARTESIAN_POINT ( 'NONE',  ( -94.83794676023109105, 30.26879337035744655, 12.23732165643094838 ) ) ;
#14419=CARTESIAN_POINT ( 'NONE',  ( 150.4748268795259776, 53.65235499498208327, -94.57192694735240934 ) ) ;
#14420=CARTESIAN_POINT ( 'NONE',  ( 80.73462811483977930, 18.54763808182591944, -21.14099230513408401 ) ) ;
#14422=CARTESIAN_POINT ( 'NONE',  ( 152.2940756559018780, 53.73566983921582363, 58.32125015338372265 ) ) ;
#14423=CARTESIAN_POINT ( 'NONE',  ( 181.0840389613909736, -170.0000000000000000, 17.46404351504774510 ) ) ;
#14424=EDGE_LOOP ( 'NONE', ( #9158, #4578 ) ) ;
#14426=CARTESIAN_POINT ( 'NONE',  ( -11.57950265606958062, 8.174070387114795722, 70.95759044635187252 ) ) ;
#14429=CARTESIAN_POINT ( 'NONE',  ( 154.4617654203035784, 56.60942201271838314, -23.66421568052971836 ) ) ;
#14431=CARTESIAN_POINT ( 'NONE',  ( -55.38707628885372714, 14.77122047090632506, 84.00730630929061249 ) ) ;
#14432=VECTOR ( 'NONE', #65043, 1000.000000000000000 ) ;
#14433=CARTESIAN_POINT ( 'NONE',  ( 104.3759779378692514, 27.35691041569131343, 41.80980636896079972 ) ) ;
#14437=CARTESIAN_POINT ( 'NONE',  ( 188.2091813586561670, 87.61952156613880049, 12.32265291410417341 ) ) ;
#14438=CARTESIAN_POINT ( 'NONE',  ( 209.6877167158271220, 113.4449353909247549, -38.22188785752970830 ) ) ;
#14439=CARTESIAN_POINT ( 'NONE',  ( 173.6020601204681952, 71.36108012062129546, 10.56114396026872271 ) ) ;
#14441=DIRECTION ( 'NONE',  ( -0.000000000000000000, 1.000000000000000000, -0.000000000000000000 ) ) ;
#14442=EDGE_LOOP ( 'NONE', ( #46737, #17190 ) ) ;
#14443=CARTESIAN_POINT ( 'NONE',  ( 104.3805245147141534, 26.26278144139197934, -74.97124564213564213 ) ) ;
#14444=CARTESIAN_POINT ( 'NONE',  ( 43.14669449386823175, 9.942681284149132992, -9.758692608636117427 ) ) ;
#14448=CARTESIAN_POINT ( 'NONE',  ( -108.6944271866239404, 37.30738480893076314, -11.75132388696829899 ) ) ;
#14450=CARTESIAN_POINT ( 'NONE',  ( -73.79615177260654946, 20.52570924097573624, 70.48734656626530182 ) ) ;
#14451=CARTESIAN_POINT ( 'NONE',  ( -55.05276343752910151, -170.0000000000000000, 30.31732777293113301 ) ) ;
#14454=CARTESIAN_POINT ( 'NONE',  ( -153.7005182577089215, 67.81869626254723471, 44.45584362651335653 ) ) ;
#14457=CARTESIAN_POINT ( 'NONE',  ( 177.7889574972181777, 75.33777460203558007, -23.63291069985390536 ) ) ;
#14460=EDGE_CURVE ( 'NONE', #67324, #31650, #30258, .T. ) ;
#14463=ORIENTED_EDGE ( 'NONE', *, *, #21033, .F. ) ;
#14464=CARTESIAN_POINT ( 'NONE',  ( 18.88468164817598804, 7.626722602998420975, -49.85434746371562653 ) ) ;
#14465=CARTESIAN_POINT ( 'NONE',  ( 8.288696687633802185, 7.382586467017838494, 63.85837421632901822 ) ) ;
#14466=CARTESIAN_POINT ( 'NONE',  ( 211.1200456646897123, 115.5868795682033578, 40.59128962156992770 ) ) ;
#14467=FACE_BOUND ( 'NONE', #50394, .T. ) ;
#14473=CARTESIAN_POINT ( 'NONE',  ( -133.2252929082529249, 52.75117980926378891, 93.42566031637895207 ) ) ;
#14474=CARTESIAN_POINT ( 'NONE',  ( -166.9982296371934751, 80.56207291422406058, -19.70677099263670584 ) ) ;
#14476=CARTESIAN_POINT ( 'NONE',  ( 9.608296193479125336, 6.381315205148816894, 86.90354082819708026 ) ) ;
#14477=CARTESIAN_POINT ( 'NONE',  ( 79.93126905972555107, 17.24332478304276250, -73.54974159810120682 ) ) ;
#14481=CARTESIAN_POINT ( 'NONE',  ( -100.4466073551322722, 31.85873123265079698, 57.57636481214915847 ) ) ;
#14483=DIRECTION ( 'NONE',  ( -0.000000000000000000, 1.000000000000000000, -0.000000000000000000 ) ) ;
#14485=DIRECTION ( 'NONE',  ( -0.000000000000000000, 1.000000000000000000, -0.000000000000000000 ) ) ;
#14488=CARTESIAN_POINT ( 'NONE',  ( 39.40195752203892710, 9.424259417798131366, 56.75838489642694640 ) ) ;
#14489=CARTESIAN_POINT ( 'NONE',  ( -109.6829043543429236, 37.85329552808669717, -95.00000000000133582 ) ) ;
#14490=CARTESIAN_POINT ( 'NONE',  ( 104.3759779378692372, 27.35691041569131343, 14.96525577849715027 ) ) ;
#14492=CARTESIAN_POINT ( 'NONE',  ( -32.73509123563383127, 9.807531206076880892, 84.01140421885408216 ) ) ;
#14493=CARTESIAN_POINT ( 'NONE',  ( 174.4912080999798434, 73.57140295268874297, -66.98354401119793522 ) ) ;
#14495=CARTESIAN_POINT ( 'NONE',  ( 102.8066580714141054, 25.59117171226999332, -44.43077199080595108 ) ) ;
#14501=CARTESIAN_POINT ( 'NONE',  ( -78.66644367742109978, 23.39876645725288284, -76.96000122218160300 ) ) ;
#14502=CARTESIAN_POINT ( 'NONE',  ( 173.6737675136087375, 72.80308721038093722, 8.769662785337226651 ) ) ;
#14506=CARTESIAN_POINT ( 'NONE',  ( 133.8566784816069344, 41.42467568809808398, -89.71241211332301191 ) ) ;
#14507=CARTESIAN_POINT ( 'NONE',  ( 34.16438717774036604, 7.785979658506379408, -91.43666240146571056 ) ) ;
#14508=CARTESIAN_POINT ( 'NONE',  ( -85.35521056349260505, 24.98314685266450752, 94.99999999999866418 ) ) ;
#14509=CARTESIAN_POINT ( 'NONE',  ( 206.2957331585308509, 110.2946564621823029, 29.33458522330292340 ) ) ;
#14510=CARTESIAN_POINT ( 'NONE',  ( -86.16504208171677703, 26.41251233979376067, 64.23306810451259707 ) ) ;
#14511=CARTESIAN_POINT ( 'NONE',  ( -104.1244073710070239, 33.72720758483609416, 45.30355529039214701 ) ) ;
#14513=ORIENTED_EDGE ( 'NONE', *, *, #60126, .T. ) ;
#14516=CARTESIAN_POINT ( 'NONE',  ( 197.9847015768255005, 97.56951352050452897, -13.62497584703676168 ) ) ;
#14519=CYLINDRICAL_SURFACE ( 'NONE', #44443, 7.500000000000013323 ) ;
#14526=CARTESIAN_POINT ( 'NONE',  ( 199.9741262455892752, 100.0845158163269133, 84.56275067836362780 ) ) ;
#14527=CARTESIAN_POINT ( 'NONE',  ( 11.20486344102687504, 7.403248964808832433, -37.06203751448568795 ) ) ;
#14533=DIRECTION ( 'NONE',  ( 0.000000000000000000, 0.000000000000000000, 1.000000000000000000 ) ) ;
#14538=CARTESIAN_POINT ( 'NONE',  ( 14.08699529666006178, 6.452200550165255954, 17.97873554617772029 ) ) ;
#14539=CARTESIAN_POINT ( 'NONE',  ( 46.51679720856117228, 10.46086439153924630, -72.38759062435165959 ) ) ;
#14540=VERTEX_POINT ( 'NONE', #44811 ) ;
#14541=CARTESIAN_POINT ( 'NONE',  ( 186.2575601542430377, 85.47765906955505955, -11.44511139629197061 ) ) ;
#14542=CARTESIAN_POINT ( 'NONE',  ( 179.0096185093687495, 76.53352131383243773, -77.79008292104482791 ) ) ;
#14543=CARTESIAN_POINT ( 'NONE',  ( -180.0175713311536470, 95.14770835574078944, -45.17381040195942177 ) ) ;
#14544=CARTESIAN_POINT ( 'NONE',  ( 87.59061758233886508, 19.75077892934018919, -9.023281811036417466 ) ) ;
#14545=CARTESIAN_POINT ( 'NONE',  ( -25.49247221749737591, 9.706368398275744269, 69.15791252073658768 ) ) ;
#14547=CARTESIAN_POINT ( 'NONE',  ( -48.57297291660695748, 13.03920345822338156, 60.85288077998132650 ) ) ;
#14548=ADVANCED_FACE ( 'NONE', ( #50770 ), #54995, .F. ) ;
#14549=VERTEX_POINT ( 'NONE', #59920 ) ;
#14550=CARTESIAN_POINT ( 'NONE',  ( -55.05276343752909440, 14.68156374112638929, 57.16187836339483397 ) ) ;
#14552=CARTESIAN_POINT ( 'NONE',  ( -108.6622665321722963, 37.28993738537008795, -73.30661870913355926 ) ) ;
#14553=CARTESIAN_POINT ( 'NONE',  ( -48.32993240732253781, 12.98137013984324994, -39.35435737847355853 ) ) ;
#14559=VERTEX_POINT ( 'NONE', #39528 ) ;
#14566=CARTESIAN_POINT ( 'NONE',  ( 134.2360421295532831, 42.83129061307084839, -89.71241211332299770 ) ) ;
#14574=CARTESIAN_POINT ( 'NONE',  ( 150.1343759737873995, 52.16508607228156791, 88.99384000258469030 ) ) ;
#14575=DIRECTION ( 'NONE',  ( -0.000000000000000000, 1.000000000000000000, -0.000000000000000000 ) ) ;
#14577=CARTESIAN_POINT ( 'NONE',  ( 105.2529848321548513, 27.73895015262024444, -22.18228092862218048 ) ) ;
#14578=CARTESIAN_POINT ( 'NONE',  ( 10.83046137699561129, 6.392429922561258415, 70.00811123621038234 ) ) ;
#14579=CARTESIAN_POINT ( 'NONE',  ( -25.48750459758502629, 9.705678256319565378, 33.12635188977065326 ) ) ;
#14580=CARTESIAN_POINT ( 'NONE',  ( 197.3064269725219333, 98.33232022113057269, 38.02162036052619243 ) ) ;
#14581=CARTESIAN_POINT ( 'NONE',  ( -81.69214136958434835, 24.57917239217752936, 84.71714431126503086 ) ) ;
#14583=ORIENTED_EDGE ( 'NONE', *, *, #67449, .T. ) ;
#14584=CARTESIAN_POINT ( 'NONE',  ( 69.83260694998128315, 15.39825517924928810, 40.44980415152751618 ) ) ;
#14587=ORIENTED_EDGE ( 'NONE', *, *, #66674, .F. ) ;
#14588=CARTESIAN_POINT ( 'NONE',  ( 114.6797682035588934, 32.10876583290004760, -76.33282036865305997 ) ) ;
#14589=CARTESIAN_POINT ( 'NONE',  ( 110.2429982417149574, 29.99119854320845846, -89.61153874658103291 ) ) ;
#14590=CARTESIAN_POINT ( 'NONE',  ( 200.4559562755963498, 100.7034888016685414, -76.87303439381707904 ) ) ;
#14591=DIRECTION ( 'NONE',  ( 0.000000000000000000, 0.000000000000000000, 1.000000000000000000 ) ) ;
#14595=EDGE_CURVE ( 'NONE', #48145, #2888, #33908, .T. ) ;
#14596=CARTESIAN_POINT ( 'NONE',  ( -48.23389383802711450, 13.99288361739331776, 34.68448182751232167 ) ) ;
#14600=CARTESIAN_POINT ( 'NONE',  ( -81.01931326044683601, 24.31309346877659650, -35.49007369283990698 ) ) ;
#14601=CARTESIAN_POINT ( 'NONE',  ( 114.5373975997477771, 30.91911807405818635, 84.61738033458334485 ) ) ;
#14602=CARTESIAN_POINT ( 'NONE',  ( -189.5329886872043801, 107.4958891766011249, 63.13570540318301738 ) ) ;
#14603=B_SPLINE_CURVE_WITH_KNOTS ( 'NONE', 3,
 ( #46934, #3674, #68061, #30765, #42002, #52210, #19160, #9653, #3337, #30413, #14578, #4027, #36038, #4374, #25499, #51864, #47270, #20201, #25152, #41657, #63461, #67710, #63114, #31116, #14914, #46580, #19863, #36384, #15272, #57837, #40614, #25838, #24796, #41318, #62774, #19507, #67369, #68722, #52884, #20533, #36734, #58178, #8627 ),
 .UNSPECIFIED., .F., .F.,
 ( 4, 2, 2, 2, 2, 2, 2, 2, 1, 2, 2, 2, 2, 2, 2, 2, 2, 2, 2, 2, 2, 4 ),
 ( 3.469446951953614189E-18, 0.001465684626643306123, 0.002198526939964957558, 0.002931369253286608776, 0.004397053879929927259, 0.005862738506573245308, 0.007328423133216562489, 0.008061265446538238427, 0.008794107759859915233, 0.009526950073181592038, 0.01025979238650326711, 0.01172547701314661898, 0.01319116163978997260, 0.01465684626643334355, 0.01538968857975502903, 0.01612253089307671278, 0.01758821551972006986, 0.01905390014636342347, 0.01978674245968510895, 0.02051958477300678749, 0.02198526939965015498, 0.02345095402629352246 ),
 .UNSPECIFIED. ) ;
#14604=CARTESIAN_POINT ( 'NONE',  ( 183.1865184929771715, 80.75677158533829925, -50.92751890011346916 ) ) ;
#14605=CARTESIAN_POINT ( 'NONE',  ( 164.9709596662455624, 63.72607097915129515, -70.20507495433403733 ) ) ;
#14610=ORIENTED_EDGE ( 'NONE', *, *, #50038, .F. ) ;
#14611=EDGE_CURVE ( 'NONE', #27023, #51958, #18079, .T. ) ;
#14613=CARTESIAN_POINT ( 'NONE',  ( 86.62931800182293784, 19.42108912189597447, -23.97701360844805407 ) ) ;
#14617=DIRECTION ( 'NONE',  ( -0.000000000000000000, 1.000000000000000000, -0.000000000000000000 ) ) ;
#14618=CARTESIAN_POINT ( 'NONE',  ( -156.4841188516942623, 70.33041971808549420, -18.23474518811625344 ) ) ;
#14620=CARTESIAN_POINT ( 'NONE',  ( 31.90184941268614693, 7.552181687745345151, 64.01634121766176122 ) ) ;
#14621=CARTESIAN_POINT ( 'NONE',  ( 46.83265140856891406, 9.492621673067191068, 89.88835326161378703 ) ) ;
#14623=CARTESIAN_POINT ( 'NONE',  ( -4.725257700476002576, 6.708862164351561574, -36.08442693939512935 ) ) ;
#14624=CARTESIAN_POINT ( 'NONE',  ( 188.2133404574782674, 86.12414067617878288, 65.99936258389180921 ) ) ;
#14628=CARTESIAN_POINT ( 'NONE',  ( 21.75198946226450758, 7.772524967554916842, -20.74856676359930674 ) ) ;
#14629=CARTESIAN_POINT ( 'NONE',  ( 9.275903038161096958, 7.385619229189520851, 14.42232764313656901 ) ) ;
#14631=CARTESIAN_POINT ( 'NONE',  ( 188.0141161196705752, 85.90515114331881819, 12.84600617614940887 ) ) ;
#14634=CARTESIAN_POINT ( 'NONE',  ( 128.0540543950622236, 39.18660671946769725, -38.74486588045738245 ) ) ;
#14635=CARTESIAN_POINT ( 'NONE',  ( -129.3963145237381411, 48.84337839101542755, -35.77770630875843949 ) ) ;
#14637=CARTESIAN_POINT ( 'NONE',  ( -108.6622665321722963, 37.28993738537006664, -46.46206811866990449 ) ) ;
#14639=CARTESIAN_POINT ( 'NONE',  ( 185.7267155939802024, 84.90388481853123892, -49.62006233998373261 ) ) ;
#14642=EDGE_CURVE ( 'NONE', #47023, #56594, #45490, .T. ) ;
#14643=CARTESIAN_POINT ( 'NONE',  ( -26.88245755577923291, 8.887394979218511182, -21.95019337430851536 ) ) ;
#14645=ORIENTED_EDGE ( 'NONE', *, *, #59771, .F. ) ;
#14646=CARTESIAN_POINT ( 'NONE',  ( 150.9996123609081167, 54.03443948832624955, 94.40777087719918370 ) ) ;
#14648=CARTESIAN_POINT ( 'NONE',  ( 126.3681350380371242, 38.23508791628619718, -69.87525203779068761 ) ) ;
#14652=CARTESIAN_POINT ( 'NONE',  ( -95.52163045714283385, 29.47808868198299592, 34.75761988864483953 ) ) ;
#14656=B_SPLINE_CURVE_WITH_KNOTS ( 'NONE', 3,
 ( #43195, #16479, #33007, #32661, #6620, #66084, #6970, #38631, #17875, #27722, #11892, #65726, #17515, #49160, #38992, #39333, #28418, #54798, #60436, #7328, #17157, #43889, #33372, #60776, #28068, #37933, #33715, #27369, #999, #65372, #48809, #59379, #12252, #55145, #650, #23156, #54087, #49871, #5907, #28783, #1698, #65019, #16815, #44605 ),
 .UNSPECIFIED., .F., .F.,
 ( 4, 2, 2, 2, 2, 2, 2, 2, 2, 2, 2, 2, 2, 2, 2, 2, 2, 2, 2, 2, 2, 4 ),
 ( 6.938893903907228378E-18, 0.001476829494128812335, 0.002215244241193225008, 0.002953658988257637247, 0.004430488482386464762, 0.005907317976515292710, 0.007384147470644119790, 0.008122562217708531596, 0.008860976964772943401, 0.01033780645890176528, 0.01181463595303058715, 0.01255305070009499549, 0.01329146544715940383, 0.01476829494128822744, 0.01550670968835264618, 0.01624512443541706666, 0.01772195392954591109, 0.01919878342367475552, 0.01993719817073917946, 0.02067561291780359994, 0.02215244241193246172, 0.02362927190606132349 ),
 .UNSPECIFIED. ) ;
#14658=ORIENTED_EDGE ( 'NONE', *, *, #21073, .F. ) ;
#14660=CARTESIAN_POINT ( 'NONE',  ( -166.0012244511291328, 80.97916541034754800, 9.102247628649013933 ) ) ;
#14661=CARTESIAN_POINT ( 'NONE',  ( -146.5309471467636229, 62.99917515507670629, -35.42503834684312380 ) ) ;
#14662=CARTESIAN_POINT ( 'NONE',  ( -133.3944793432480651, 52.87251459353622352, 65.21942218520352696 ) ) ;
#14667=CARTESIAN_POINT ( 'NONE',  ( -60.66241560458681192, 16.25736033771446998, -20.87440278488216094 ) ) ;
#14668=CARTESIAN_POINT ( 'NONE',  ( -132.9126122820978821, 52.52752252041126724, -71.91483001303755884 ) ) ;
#14669=ADVANCED_FACE ( 'NONE', ( #50082 ), #54650, .F. ) ;
#14672=CARTESIAN_POINT ( 'NONE',  ( 69.36287815987336103, 15.27486453472190497, -74.06810378652023985 ) ) ;
#14675=CARTESIAN_POINT ( 'NONE',  ( 116.4569059613810680, 31.86445263670867334, 94.99999999999866418 ) ) ;
#14677=DIRECTION ( 'NONE',  ( -0.8118923937861950435, -0.5838071093367415143, 0.000000000000000000 ) ) ;
#14678=CARTESIAN_POINT ( 'NONE',  ( -51.75347637701212733, 13.82167660501363393, -89.66666266855726519 ) ) ;
#14679=VECTOR ( 'NONE', #66485, 1000.000000000000000 ) ;
#14680=CARTESIAN_POINT ( 'NONE',  ( -71.17846906053300415, 20.67346400882179225, 37.42370288375377640 ) ) ;
#14683=LINE ( 'NONE', #15382, #60932 ) ;
#14684=CARTESIAN_POINT ( 'NONE',  ( 210.1633650091868901, 114.1507944623966608, 58.41051192917949209 ) ) ;
#14688=CARTESIAN_POINT ( 'NONE',  ( -109.7643866341847172, 37.89854104106754562, 37.46775542559241501 ) ) ;
#14690=CARTESIAN_POINT ( 'NONE',  ( -178.3015291115128207, 93.08500010736474906, -90.45828512500401075 ) ) ;
#14694=CARTESIAN_POINT ( 'NONE',  ( -190.6985136298602015, 109.1272424661243434, -64.50448789838189612 ) ) ;
#14695=CARTESIAN_POINT ( 'NONE',  ( 34.45972925205165183, 8.830088223935245395, 4.906826754313283523 ) ) ;
#14696=EDGE_CURVE ( 'NONE', #47003, #39145, #58755, .T. ) ;
#14698=CARTESIAN_POINT ( 'NONE',  ( 31.99894129856763314, 7.561773404408294930, 9.342126976674117955 ) ) ;
#14699=CARTESIAN_POINT ( 'NONE',  ( -12.39770133248888229, 8.241491894828989473, -48.88360719805099563 ) ) ;
#14701=LINE ( 'NONE', #51989, #40508 ) ;
#14704=CARTESIAN_POINT ( 'NONE',  ( -122.6790374842361757, 45.60652803413277923, -89.31330210188735919 ) ) ;
#14705=ORIENTED_EDGE ( 'NONE', *, *, #6319, .T. ) ;
#14708=DIRECTION ( 'NONE',  ( -0.000000000000000000, 0.000000000000000000, -1.000000000000000000 ) ) ;
#14711=CARTESIAN_POINT ( 'NONE',  ( -97.85576954355160240, 30.58918648956190367, -9.594846923323533616 ) ) ;
#14712=B_SPLINE_CURVE_WITH_KNOTS ( 'NONE', 3,
 ( #67703, #14233, #18124, #39576, #35693, #35340, #8615, #56437, #2636, #61027, #50477, #56799, #45891, #24100, #29714, #51522, #12854, #18813, #23747, #34308, #55754, #45194, #66670, #3327, #18470, #7915, #39918, #61374, #51174, #45539, #13199, #34664, #29365, #50819, #61716, #13540, #34995, #2991, #24450, #68389, #20880, #25140, #63800, #41989, #26505 ),
 .UNSPECIFIED., .F., .F.,
 ( 4, 2, 2, 1, 2, 2, 2, 2, 2, 2, 2, 2, 2, 2, 2, 2, 2, 2, 2, 2, 2, 2, 4 ),
 ( 0.02348395315094740227, 0.02495010856601298163, 0.02568318627354576958, 0.02641626398107856100, 0.02714934168861135241, 0.02788241939614414036, 0.02934857481120972666, 0.03008165251874251461, 0.03081473022627530950, 0.03228088564134089233, 0.03301396334887368722, 0.03374704105640647517, 0.03521319647147206494, 0.03667935188653764778, 0.03741242959407044266, 0.03814550730160323755, 0.03961166271666881344, 0.04107781813173440322, 0.04254397354679998605, 0.04327705125433277400, 0.04401012896186556889, 0.04547628437693115172, 0.04694243979199673455 ),
 .UNSPECIFIED. ) ;
#14713=CARTESIAN_POINT ( 'NONE',  ( 150.4722669492348643, 53.65054032737663903, -46.33541081562344033 ) ) ;
#14717=CARTESIAN_POINT ( 'NONE',  ( 178.1888264190354505, 77.13727704498029425, -9.948467367157029173 ) ) ;
#14718=CARTESIAN_POINT ( 'NONE',  ( -102.2801239173131052, 33.91021738430207222, 72.36362509687883460 ) ) ;
#14721=CARTESIAN_POINT ( 'NONE',  ( -175.1895962157337010, 90.99110972060690017, -76.27797459989902507 ) ) ;
#14722=CARTESIAN_POINT ( 'NONE',  ( -0.3249717932738303561, 6.518578686837484426, -15.58535181265489022 ) ) ;
#14724=CARTESIAN_POINT ( 'NONE',  ( 112.1012908502484606, 29.75117929736499889, 29.84123205385900590 ) ) ;
#14727=CARTESIAN_POINT ( 'NONE',  ( 197.1980152960109933, 96.59350208824299955, 37.04504252498942662 ) ) ;
#14728=CARTESIAN_POINT ( 'NONE',  ( 115.0454575488273576, 31.16784721673998249, -76.03284390000987969 ) ) ;
#14729=DIRECTION ( 'NONE',  ( 0.000000000000000000, 0.000000000000000000, 1.000000000000000000 ) ) ;
#14730=CARTESIAN_POINT ( 'NONE',  ( 187.0314709137215345, 84.83273891797912825, -92.84016220200550151 ) ) ;
#14739=CARTESIAN_POINT ( 'NONE',  ( -105.8768181937898873, 34.64545164169051361, -35.91624400628371916 ) ) ;
#14740=CARTESIAN_POINT ( 'NONE',  ( 140.8375554551808477, 45.80242115643797973, 93.46421066599228311 ) ) ;
#14741=CARTESIAN_POINT ( 'NONE',  ( 151.1827182658834090, 54.16800928478853194, 5.944559561786584290 ) ) ;
#14742=ORIENTED_EDGE ( 'NONE', *, *, #65215, .T. ) ;
#14746=B_SPLINE_CURVE_WITH_KNOTS ( 'NONE', 3,
 ( #41774, #69522, #58623, #63913, #15727, #42789, #53692, #37176, #20309, #37520, #4145, #10438, #68504, #10786, #63230, #58972, #32259, #36496, #57947, #5512, #21686, #9767, #31229, #43137, #64607, #52660, #20655, #16416, #25944, #47376, #52322, #68831, #42115, #63572, #38563, #38217, #54380, #32937 ),
 .UNSPECIFIED., .F., .F.,
 ( 4, 2, 2, 2, 2, 2, 2, 2, 2, 2, 2, 2, 2, 2, 2, 2, 2, 2, 4 ),
 ( 1.561251128379126385E-17, 0.001559859933532253048, 0.003119719867064490483, 0.004679579800596727485, 0.006239439734128965354, 0.007799299667661202355, 0.008579229634427315218, 0.009359159601193428948, 0.01091901953472565120, 0.01169894950149175800, 0.01247887946825786652, 0.01403873940179008704, 0.01559859933532230583, 0.01715845926885452288, 0.01871831920238674341, 0.02027817913591895699, 0.02183803906945117751, 0.02339789900298339109, 0.02495775893651561161 ),
 .UNSPECIFIED. ) ;
#14751=ADVANCED_FACE ( 'NONE', ( #13493 ), #30018, .F. ) ;
#14755=CARTESIAN_POINT ( 'NONE',  ( 139.6203063421347395, 45.01495791936840618, 59.03001518722842889 ) ) ;
#14759=CARTESIAN_POINT ( 'NONE',  ( 88.52077179907878701, 21.14145351760140557, 44.47362131126318729 ) ) ;
#14761=CARTESIAN_POINT ( 'NONE',  ( 39.40195752203891999, 9.424259417798145577, 18.06928371549960133 ) ) ;
#14763=CARTESIAN_POINT ( 'NONE',  ( 150.2941978382489197, 53.52137138947625061, -18.97662088534088198 ) ) ;
#14765=CARTESIAN_POINT ( 'NONE',  ( 197.6319840686292082, -170.0000000000000000, -95.00000000000133582 ) ) ;
#14766=CARTESIAN_POINT ( 'NONE',  ( -152.2964402771109462, 66.58174574061955298, -62.19164853688251071 ) ) ;
#14767=CARTESIAN_POINT ( 'NONE',  ( 59.84823624668899811, 11.96014623718603964, 84.19572422589860139 ) ) ;
#14769=CARTESIAN_POINT ( 'NONE',  ( 212.0739503583954217, 117.0412199804969617, -45.22451888985740709 ) ) ;
#14770=CARTESIAN_POINT ( 'NONE',  ( 176.4367926094705581, 74.03315361639849357, 4.072456122556812552 ) ) ;
#14774=CARTESIAN_POINT ( 'NONE',  ( -76.33235143960693847, 22.51916353135074189, 71.89429839980979864 ) ) ;
#14776=CARTESIAN_POINT ( 'NONE',  ( 63.01563776193091826, 12.67277567978498709, -62.56524142263340593 ) ) ;
#14780=CARTESIAN_POINT ( 'NONE',  ( 17.72748965151693668, 7.577488030789625739, 44.76384774945338307 ) ) ;
#14781=CARTESIAN_POINT ( 'NONE',  ( -104.1225399044495816, 34.86084180570100699, -22.94399755735298996 ) ) ;
#14783=AXIS2_PLACEMENT_3D ( 'NONE', #53813, #49582, #27094 ) ;
#14785=CARTESIAN_POINT ( 'NONE',  ( 197.6319840686292082, 97.13072366387987699, -95.00000000000133582 ) ) ;
#14791=CARTESIAN_POINT ( 'NONE',  ( 177.0024338932394130, 74.57605685449964028, -10.57210100736196878 ) ) ;
#14793=CARTESIAN_POINT ( 'NONE',  ( -143.7151964745329451, 59.41799441280381444, 6.605001292783195588 ) ) ;
#14798=CARTESIAN_POINT ( 'NONE',  ( 210.9747454890631388, 115.3673079504855536, 13.97618168240338399 ) ) ;
#14799=CARTESIAN_POINT ( 'NONE',  ( 11.20486344102687504, 7.403248964808828880, 70.31616484736908035 ) ) ;
#14800=FACE_BOUND ( 'NONE', #38343, .T. ) ;
#14801=ORIENTED_EDGE ( 'NONE', *, *, #6009, .T. ) ;
#14802=ORIENTED_EDGE ( 'NONE', *, *, #60674, .F. ) ;
#14803=DIRECTION ( 'NONE',  ( -0.000000000000000000, 1.000000000000000000, -0.000000000000000000 ) ) ;
#14804=CARTESIAN_POINT ( 'NONE',  ( -118.3864719359396389, 42.92356051160688679, 91.74072687414530947 ) ) ;
#14805=CARTESIAN_POINT ( 'NONE',  ( -166.2028657618941452, 79.74389853943294781, -12.45684997849616771 ) ) ;
#14806=FACE_OUTER_BOUND ( 'NONE', #35230, .T. ) ;
#14807=CARTESIAN_POINT ( 'NONE',  ( 22.57231971038877205, 6.812631029037583552, 94.41881611565530363 ) ) ;
#14808=CARTESIAN_POINT ( 'NONE',  ( 23.28635475458051118, 7.864714260171793647, 91.57214863357140189 ) ) ;
#14809=ORIENTED_EDGE ( 'NONE', *, *, #48676, .T. ) ;
#14810=DIRECTION ( 'NONE',  ( -0.000000000000000000, 1.000000000000000000, -0.000000000000000000 ) ) ;
#14811=CARTESIAN_POINT ( 'NONE',  ( -96.43148989374459745, 29.90755650959363976, 69.58523154106214292 ) ) ;
#14813=CARTESIAN_POINT ( 'NONE',  ( -84.54326985437106146, 24.64760594531652771, 15.75942825447480189 ) ) ;
#14814=ORIENTED_EDGE ( 'NONE', *, *, #16853, .F. ) ;
#14815=CARTESIAN_POINT ( 'NONE',  ( -31.43908319763709969, 10.61114334766717171, -62.16174795566551836 ) ) ;
#14819=CARTESIAN_POINT ( 'NONE',  ( 15.78827728214693416, 6.500811158483284835, -50.51894409868581448 ) ) ;
#14821=CARTESIAN_POINT ( 'NONE',  ( 132.0582325211145474, 40.34869848118185587, 71.15012554800902933 ) ) ;
#14828=CARTESIAN_POINT ( 'NONE',  ( -28.33384212282240000, 9.102119872907532994, 84.57104976863398349 ) ) ;
#14829=CARTESIAN_POINT ( 'NONE',  ( 179.4074606910091347, 78.34362448405028090, -63.20884701633242031 ) ) ;
#14831=CARTESIAN_POINT ( 'NONE',  ( -31.43908319763710679, -170.0000000000000000, 18.37190381572551701 ) ) ;
#14832=CARTESIAN_POINT ( 'NONE',  ( 104.7034219878852213, 26.40210929103716708, -48.50262205611462463 ) ) ;
#14834=CARTESIAN_POINT ( 'NONE',  ( 80.16761386260783695, 18.37011649821943138, -47.16167432286557215 ) ) ;
#14835=CARTESIAN_POINT ( 'NONE',  ( -149.5074843970970733, 65.50121172469317798, -61.65738112195564469 ) ) ;
#14840=CARTESIAN_POINT ( 'NONE',  ( -86.11230725916328765, 26.39026888680168526, -70.49370428031920710 ) ) ;
#14841=CARTESIAN_POINT ( 'NONE',  ( -1.000266010268695327, 6.542200531770547833, -93.38246921637555431 ) ) ;
#14844=CARTESIAN_POINT ( 'NONE',  ( 126.6395826915640015, 37.23416510613628816, 8.108414546062657990 ) ) ;
#14845=CARTESIAN_POINT ( 'NONE',  ( 32.12337157895397866, 7.574134358465434147, -95.00000000000133582 ) ) ;
#14847=B_SPLINE_CURVE_WITH_KNOTS ( 'NONE', 3,
 ( #24766, #3305, #62395, #12831, #45869, #18445, #29689, #13854, #51155, #35315, #67682, #51504, #39900, #19130, #56776, #34974, #55733, #8594, #56080, #46550, #34287, #40249, #19474, #18789, #30381, #2967, #23724, #24428, #30043, #51833, #50457, #62038, #40934, #61695, #29016, #3645, #68031, #39556, #61007, #2278, #13177, #34645, #7896, #29343, #50797 ),
 .UNSPECIFIED., .F., .F.,
 ( 4, 2, 2, 1, 2, 2, 2, 2, 2, 2, 2, 2, 2, 2, 2, 2, 2, 2, 2, 2, 2, 2, 4 ),
 ( 0.02348395315094738839, 0.02495010856601294694, 0.02568318627354572795, 0.02641626398107850549, 0.02714934168861128302, 0.02788241939614406056, 0.02934857481120962258, 0.03008165251874240706, 0.03081473022627519501, 0.03228088564134074662, 0.03301396334887353456, 0.03374704105640634333, 0.03521319647147195392, 0.03667935188653756451, 0.03741242959407034552, 0.03814550730160313347, 0.03961166271666874406, 0.04107781813173435465, 0.04254397354679996524, 0.04327705125433275318, 0.04401012896186554807, 0.04547628437693113090, 0.04694243979199672068 ),
 .UNSPECIFIED. ) ;
#14848=CARTESIAN_POINT ( 'NONE',  ( 208.9585401441656245, 114.1617785893844257, 42.89634414365027482 ) ) ;
#14849=CARTESIAN_POINT ( 'NONE',  ( -74.17694007417655655, 20.66176641130876845, -63.43242567744339055 ) ) ;
#14850=CARTESIAN_POINT ( 'NONE',  ( -109.5142642360664098, 36.61018064014776741, 35.97134868343648861 ) ) ;
#14851=ORIENTED_EDGE ( 'NONE', *, *, #42638, .F. ) ;
#14853=CARTESIAN_POINT ( 'NONE',  ( -57.24869976356938395, 16.32563047877252416, 84.32812304263042336 ) ) ;
#14857=EDGE_CURVE ( 'NONE', #57612, #4893, #15216, .T. ) ;
#14862=CARTESIAN_POINT ( 'NONE',  ( 139.6326990672751265, 46.22017155708125813, -48.31381116572497803 ) ) ;
#14863=CARTESIAN_POINT ( 'NONE',  ( 206.0459564151325083, 109.9423578521132328, -90.10578531043864814 ) ) ;
#14867=ORIENTED_EDGE ( 'NONE', *, *, #43178, .T. ) ;
#14869=CARTESIAN_POINT ( 'NONE',  ( 179.2582403890615979, 78.19797385420241653, 83.21752769010527118 ) ) ;
#14871=CARTESIAN_POINT ( 'NONE',  ( -30.95355748062275936, 9.511738996772322707, -77.16174795566556099 ) ) ;
#14875=CARTESIAN_POINT ( 'NONE',  ( -7.825402957745087207, 7.899365992529248537, -62.26262132240749736 ) ) ;
#14877=CARTESIAN_POINT ( 'NONE',  ( 173.6020601204681952, 71.36108012062130967, -69.97250781112231266 ) ) ;
#14881=CARTESIAN_POINT ( 'NONE',  ( -29.03891846981456126, 10.22741474064058487, 57.43857379582767209 ) ) ;
#14883=CARTESIAN_POINT ( 'NONE',  ( -47.95468448182523247, 12.89252559348046212, 67.09685781612688515 ) ) ;
#14885=EDGE_LOOP ( 'NONE', ( #58747, #65893 ) ) ;
#14890=CARTESIAN_POINT ( 'NONE',  ( -109.4995148930278077, 37.75156937139181679, -71.45788426471575860 ) ) ;
#14892=CARTESIAN_POINT ( 'NONE',  ( 133.8566784816069060, 42.60093787723652525, 44.51034083899536142 ) ) ;
#14896=CYLINDRICAL_SURFACE ( 'NONE', #30297, 7.500000000000013323 ) ;
#14897=CARTESIAN_POINT ( 'NONE',  ( -61.86403937395562735, 16.61416349803656445, 67.81112795023058482 ) ) ;
#14900=CARTESIAN_POINT ( 'NONE',  ( 46.88995144419296679, 10.52126979626132197, 90.56259000874159426 ) ) ;
#14901=CARTESIAN_POINT ( 'NONE',  ( -175.1920326508033270, 89.46239303019292777, -76.27753814462546700 ) ) ;
#14904=DIRECTION ( 'NONE',  ( -0.000000000000000000, 1.000000000000000000, -0.000000000000000000 ) ) ;
#14906=CARTESIAN_POINT ( 'NONE',  ( 55.57634120535661992, 12.09544293553729943, -42.23651943899194805 ) ) ;
#14909=CARTESIAN_POINT ( 'NONE',  ( 93.33480479917541572, 21.81892021443993812, 40.60918334494109416 ) ) ;
#14911=ORIENTED_EDGE ( 'NONE', *, *, #48872, .T. ) ;
#14912=EDGE_CURVE ( 'NONE', #29587, #20616, #57038, .T. ) ;
#14914=CARTESIAN_POINT ( 'NONE',  ( 8.528421445032394743, 6.376778749352037146, 62.41374088788820274 ) ) ;
#14915=CARTESIAN_POINT ( 'NONE',  ( -25.07901552294942960, 9.649193085547780768, 41.69897551811279612 ) ) ;
#14916=CARTESIAN_POINT ( 'NONE',  ( 197.6329787101073805, 98.74106466892202150, 34.17182954918762050 ) ) ;
#14917=PLANE ( 'NONE',  #17390 ) ;
#14924=ORIENTED_EDGE ( 'NONE', *, *, #63378, .T. ) ;
#14928=CARTESIAN_POINT ( 'NONE',  ( 197.3707490726349363, 96.80690576410100334, -69.03806240719120524 ) ) ;
#14929=CARTESIAN_POINT ( 'NONE',  ( -38.93938005333174601, 11.96888249046459940, 64.80069294567751115 ) ) ;
#14931=CARTESIAN_POINT ( 'NONE',  ( -118.6288898061518466, 41.89286798341290563, 63.08229067355227215 ) ) ;
#14932=CARTESIAN_POINT ( 'NONE',  ( -82.93126516400697312, 25.07709093823493518, -21.94504152255926144 ) ) ;
#14933=CARTESIAN_POINT ( 'NONE',  ( -196.7348448768811409, -170.0000000000000000, -15.26653320754434162 ) ) ;
#14935=DIRECTION ( 'NONE',  ( 0.000000000000000000, -1.000000000000000000, 0.000000000000000000 ) ) ;
#14940=CARTESIAN_POINT ( 'NONE',  ( -86.16504208171676282, 26.41251233979373936, -43.14513425734210017 ) ) ;
#14942=CARTESIAN_POINT ( 'NONE',  ( 106.3034350612047518, 27.10143568295973182, 84.40989449007727785 ) ) ;
#14943=DIRECTION ( 'NONE',  ( 0.000000000000000000, 0.000000000000000000, 1.000000000000000000 ) ) ;
#14947=PLANE ( 'NONE',  #43799 ) ;
#14948=CARTESIAN_POINT ( 'NONE',  ( 164.8942204024298803, 63.66138186734712434, -69.36631708222795112 ) ) ;
#14949=ORIENTED_EDGE ( 'NONE', *, *, #16038, .T. ) ;
#14953=CARTESIAN_POINT ( 'NONE',  ( -86.10361028793438720, 25.29528064050658287, 63.76107057542620993 ) ) ;
#14954=CARTESIAN_POINT ( 'NONE',  ( 105.2224576781852363, 26.62754899994121516, -91.52473545953954215 ) ) ;
#14955=CARTESIAN_POINT ( 'NONE',  ( -35.17296606710973350, 11.25626711331310403, -76.18484644730783373 ) ) ;
#14957=CARTESIAN_POINT ( 'NONE',  ( 32.28603806442400526, 7.590310383548732887, 61.83839758995276981 ) ) ;
#14958=CARTESIAN_POINT ( 'NONE',  ( 46.40453471432315524, 9.423871119279747077, 93.80938164509879584 ) ) ;
#14960=CARTESIAN_POINT ( 'NONE',  ( 17.72748965151693668, 7.577488030789625739, 17.91929715898970699 ) ) ;
#14961=CARTESIAN_POINT ( 'NONE',  ( 185.1647878987786555, 82.82967084668430857, 57.34492923270315856 ) ) ;
#14964=CARTESIAN_POINT ( 'NONE',  ( 129.1137093889808796, 38.63348691920625555, -22.49364613101846899 ) ) ;
#14965=CARTESIAN_POINT ( 'NONE',  ( 21.43750346857337874, 7.754771113113081427, -11.21701564101427451 ) ) ;
#14966=CARTESIAN_POINT ( 'NONE',  ( 198.2545923567585078, 97.90679023593570207, 59.70290751491250347 ) ) ;
#14969=AXIS2_PLACEMENT_3D ( 'NONE', #38747, #16584, #44355 ) ;
#14970=CARTESIAN_POINT ( 'NONE',  ( 188.5645326065591405, 86.51153908883291876, 9.344684421083345072 ) ) ;
#14972=CARTESIAN_POINT ( 'NONE',  ( 173.6020601204682237, 71.36108012062136652, 37.40569455073241301 ) ) ;
#14974=CARTESIAN_POINT ( 'NONE',  ( -106.6711220790662935, 36.20923238211248929, -48.59962218315158822 ) ) ;
#14976=CARTESIAN_POINT ( 'NONE',  ( 187.5165082312810512, 86.85340440641662951, -47.59062793446263839 ) ) ;
#14984=CARTESIAN_POINT ( 'NONE',  ( 173.8971638285193819, 71.63521281801094176, 92.67731212905682980 ) ) ;
#14988=CARTESIAN_POINT ( 'NONE',  ( 116.6457744947906860, 31.95847117670279403, 60.04196747368758480 ) ) ;
#14993=AXIS2_PLACEMENT_3D ( 'NONE', #62, #15218, #42966 ) ;
#15000=ORIENTED_EDGE ( 'NONE', *, *, #33678, .T. ) ;
#15005=B_SPLINE_CURVE_WITH_KNOTS ( 'NONE', 3,
 ( #14489, #57062, #40189, #25407, #67965, #20113, #29977, #34916, #61640, #8176, #52118, #35945, #46838, #61294, #7835, #13117, #13456, #29283, #45809, #56355, #8874, #51090, #40524, #2904 ),
 .UNSPECIFIED., .F., .F.,
 ( 4, 2, 2, 2, 2, 2, 2, 2, 2, 2, 2, 4 ),
 ( 0.000000000000000000, 0.001412135740307523526, 0.002118203610461290385, 0.002824271480615057027, 0.004236407220922555616, 0.005648542961230055073, 0.007060678701537554530, 0.007766746571691303391, 0.008472814441845052252, 0.009884950182152539566, 0.01059101805230627281, 0.01129708592246000433 ),
 .UNSPECIFIED. ) ;
#15007=CARTESIAN_POINT ( 'NONE',  ( -177.5271152834791337, 92.16916858125016176, -9.280385424022256302 ) ) ;
#15010=VERTEX_POINT ( 'NONE', #49900 ) ;
#15014=CARTESIAN_POINT ( 'NONE',  ( -62.45176220516621868, 16.79101814080733490, -14.61954841212545553 ) ) ;
#15015=CARTESIAN_POINT ( 'NONE',  ( -132.0738857626834317, 51.93126104279143362, -73.51499412664540500 ) ) ;
#15019=CARTESIAN_POINT ( 'NONE',  ( 69.72789637502503979, 15.37065610545702121, -73.42043340095284520 ) ) ;
#15024=CARTESIAN_POINT ( 'NONE',  ( 183.3913492984168840, 80.96922346472079823, -77.70910907680601554 ) ) ;
#15025=DIRECTION ( 'NONE',  ( 0.000000000000000000, 0.000000000000000000, 1.000000000000000000 ) ) ;
#15027=EDGE_CURVE ( 'NONE', #37023, #19968, #14701, .T. ) ;
#15031=CARTESIAN_POINT ( 'NONE',  ( 102.7446498997619955, 26.65764321315729646, -70.80359580029494282 ) ) ;
#15032=CARTESIAN_POINT ( 'NONE',  ( -74.18622060908361959, 21.73430079572373685, 31.88400080372565171 ) ) ;
#15033=CARTESIAN_POINT ( 'NONE',  ( 79.14242532928582818, 17.00090225993928073, 37.72179837095220734 ) ) ;
#15035=CARTESIAN_POINT ( 'NONE',  ( -146.1142527948576628, 61.35394402951022386, 44.91319804243705960 ) ) ;
#15037=CARTESIAN_POINT ( 'NONE',  ( -121.2119672714299412, 44.67540322905995964, 43.99914708956819709 ) ) ;
#15038=CARTESIAN_POINT ( 'NONE',  ( -166.9982296371934751, 80.56207291422407479, -73.39587217356408644 ) ) ;
#15039=VERTEX_POINT ( 'NONE', #25274 ) ;
#15041=CYLINDRICAL_SURFACE ( 'NONE', #43389, 7.500000000000013323 ) ;
#15043=CARTESIAN_POINT ( 'NONE',  ( -176.2094613402388177, 90.62878080648660273, -89.01962546083346695 ) ) ;
#15046=DIRECTION ( 'NONE',  ( 0.000000000000000000, 0.000000000000000000, 1.000000000000000000 ) ) ;
#15047=DIRECTION ( 'NONE',  ( 0.000000000000000000, 0.000000000000000000, 1.000000000000000000 ) ) ;
#15048=CARTESIAN_POINT ( 'NONE',  ( 33.93974911725171495, 8.773765372885565128, 5.423990806426351341 ) ) ;
#15049=DIRECTION ( 'NONE',  ( 0.000000000000000000, 0.000000000000000000, 1.000000000000000000 ) ) ;
#15050=CARTESIAN_POINT ( 'NONE',  ( 33.75639351246964992, 7.742023566824295600, 5.607121423256566040 ) ) ;
#15051=CARTESIAN_POINT ( 'NONE',  ( -14.84452950307166752, 8.460866451887707029, -45.57178442109233174 ) ) ;
#15053=CARTESIAN_POINT ( 'NONE',  ( -37.05762690088740641, 11.60527003175541516, -20.94685073097974026 ) ) ;
#15054=ORIENTED_EDGE ( 'NONE', *, *, #14611, .F. ) ;
#15055=CARTESIAN_POINT ( 'NONE',  ( -118.5482723061148675, 43.02244411383185252, -94.50929498175072752 ) ) ;
#15058=CARTESIAN_POINT ( 'NONE',  ( 15.29912143387263335, 7.491799981865498559, -77.36349468914950478 ) ) ;
#15059=CARTESIAN_POINT ( 'NONE',  ( -25.35398647985413945, 8.671412257862217032, 6.480746930813777951 ) ) ;
#15061=CARTESIAN_POINT ( 'NONE',  ( -15.26524495591508490, 7.490231452641284093, -70.74238069447982014 ) ) ;
#15063=CARTESIAN_POINT ( 'NONE',  ( 157.0316110297313799, 58.58403635656377162, -36.12418429913763163 ) ) ;
#15066=CARTESIAN_POINT ( 'NONE',  ( -154.7826623253030220, 70.14150242829514070, 59.72844556814614947 ) ) ;
#15067=CARTESIAN_POINT ( 'NONE',  ( 175.8947993867357411, 74.90689716047907609, -22.31635991957287146 ) ) ;
#15069=CARTESIAN_POINT ( 'NONE',  ( -127.6881387055492354, 48.89937523111241546, -49.69948083571843256 ) ) ;
#15071=CARTESIAN_POINT ( 'NONE',  ( -180.5954680880247452, 97.44843622358467883, -69.69668263771576733 ) ) ;
#15072=CARTESIAN_POINT ( 'NONE',  ( 93.09528872995974780, 21.72934119836187961, 67.88888913272387526 ) ) ;
#15073=CARTESIAN_POINT ( 'NONE',  ( 114.6632852039171269, 30.98120524556723865, 31.04740591163416852 ) ) ;
#15077=CARTESIAN_POINT ( 'NONE',  ( 140.4897729434290738, 45.57634363643753517, 40.54951988003531937 ) ) ;
#15078=ORIENTED_EDGE ( 'NONE', *, *, #65215, .F. ) ;
#15080=CARTESIAN_POINT ( 'NONE',  ( 112.1164716692773453, 29.75790342121400656, -62.98934640487257042 ) ) ;
#15081=AXIS2_PLACEMENT_3D ( 'NONE', #32942, #5854, #1289 ) ;
#15082=CARTESIAN_POINT ( 'NONE',  ( 184.5867277229703518, 83.68414666546578928, 43.44420243020122996 ) ) ;
#15083=CARTESIAN_POINT ( 'NONE',  ( 163.5944155533006210, 63.88379440759435823, 5.727933679616943330 ) ) ;
#15088=EDGE_CURVE ( 'NONE', #40950, #48132, #25622, .T. ) ;
#15090=CIRCLE ( 'NONE', #54379, 242.4895526022646379 ) ;
#15092=CARTESIAN_POINT ( 'NONE',  ( -77.72491324796693846, 21.96482567905605876, -23.22677241843959450 ) ) ;
#15093=CARTESIAN_POINT ( 'NONE',  ( 140.9234142684720723, 45.85831937333605168, 88.16266470440997693 ) ) ;
#15095=EDGE_CURVE ( 'NONE', #29084, #48132, #51294, .T. ) ;
#15096=CARTESIAN_POINT ( 'NONE',  ( -62.49130718206701829, 16.80297926264070796, 36.82688365366426808 ) ) ;
#15098=CARTESIAN_POINT ( 'NONE',  ( 156.5993887774280608, 58.24868799840906775, 2.612442410024496731 ) ) ;
#15099=ORIENTED_EDGE ( 'NONE', *, *, #24886, .T. ) ;
#15101=CARTESIAN_POINT ( 'NONE',  ( -7.825402957745083654, 6.891034867348163395, -23.57352014148015584 ) ) ;
#15103=ORIENTED_EDGE ( 'NONE', *, *, #30928, .F. ) ;
#15107=CARTESIAN_POINT ( 'NONE',  ( 135.4423125506059193, 42.39015362494584593, 56.52087882447440137 ) ) ;
#15109=DIRECTION ( 'NONE',  ( -0.000000000000000000, 1.000000000000000000, -0.000000000000000000 ) ) ;
#15110=LINE ( 'NONE', #35875, #47314 ) ;
#15112=LINE ( 'NONE', #4216, #6175 ) ;
#15115=EDGE_CURVE ( 'NONE', #10179, #10310, #45319, .T. ) ;
#15116=CARTESIAN_POINT ( 'NONE',  ( 207.8398359204632868, 112.5208221429021336, -23.79464188816103487 ) ) ;
#15117=LINE ( 'NONE', #14765, #64990 ) ;
#15118=CARTESIAN_POINT ( 'NONE',  ( -7.336630171688589108, 7.867399454768209566, 30.11558103944719633 ) ) ;
#15119=CARTESIAN_POINT ( 'NONE',  ( 56.83144462367863525, 11.32279212915456768, 86.74568550056409322 ) ) ;
#15121=CARTESIAN_POINT ( 'NONE',  ( 182.7686108735401262, 81.77235358504610474, 2.643295075472624323 ) ) ;
#15122=CARTESIAN_POINT ( 'NONE',  ( 207.4867844023104340, 110.2451255333963900, -36.85174997040083156 ) ) ;
#15125=AXIS2_PLACEMENT_3D ( 'NONE', #13984, #34419, #61813 ) ;
#15128=CARTESIAN_POINT ( 'NONE',  ( -77.02112161466367013, 22.77583432622785153, 72.08387616735952008 ) ) ;
#15129=CARTESIAN_POINT ( 'NONE',  ( 56.66775172211443845, 11.28938863449062069, -66.06332206576500710 ) ) ;
#15132=CARTESIAN_POINT ( 'NONE',  ( -10.38456464615029518, 7.071067413477805985, 84.24719785865121935 ) ) ;
#15133=CARTESIAN_POINT ( 'NONE',  ( -104.1393288135077171, 34.86912007524087898, -8.388960353306918805 ) ) ;
#15134=VECTOR ( 'NONE', #16262, 1000.000000000000000 ) ;
#15136=CARTESIAN_POINT ( 'NONE',  ( -75.43044859198180063, 21.11535168543635876, 71.53302750611915428 ) ) ;
#15143=CARTESIAN_POINT ( 'NONE',  ( 58.48209831743722731, 11.66636741727081983, -37.22615017468061893 ) ) ;
#15144=CARTESIAN_POINT ( 'NONE',  ( 174.9053416555736646, 72.57849647436442808, -21.16220004635683694 ) ) ;
#15146=CIRCLE ( 'NONE', #60014, 243.4957430088094839 ) ;
#15147=CARTESIAN_POINT ( 'NONE',  ( -147.3641864666714696, 62.38213854487951693, 4.175494494443603877 ) ) ;
#15148=B_SPLINE_CURVE_WITH_KNOTS ( 'NONE', 3,
 ( #48691, #21983, #33601, #28305, #66659, #11418, #6510, #49403, #23042, #39566, #18109, #59957, #65610, #7207, #17766, #54325, #22338, #43776 ),
 .UNSPECIFIED., .F., .F.,
 ( 4, 2, 2, 2, 2, 2, 2, 2, 4 ),
 ( 0.01172246177653528745, 0.01320773491327431257, 0.01469300805001333941, 0.01617828118675236626, 0.01766355432349139137, 0.01914882746023041649, 0.02063410059696944160, 0.02211937373370847018, 0.02360464687044749529 ),
 .UNSPECIFIED. ) ;
#15149=ORIENTED_EDGE ( 'NONE', *, *, #45418, .T. ) ;
#15150=CARTESIAN_POINT ( 'NONE',  ( -133.3220917939969752, 52.82057604964900577, 39.18959366347132089 ) ) ;
#15152=CARTESIAN_POINT ( 'NONE',  ( 211.5175447467295839, 116.1901475271413631, 12.99830586765888185 ) ) ;
#15153=CARTESIAN_POINT ( 'NONE',  ( -142.0070007485041401, 59.34878529741516928, 37.95131792514063562 ) ) ;
#15154=CARTESIAN_POINT ( 'NONE',  ( 212.0850679406003678, 117.0583048437722198, 38.04715775346591045 ) ) ;
#15158=ORIENTED_EDGE ( 'NONE', *, *, #34494, .T. ) ;
#15161=CARTESIAN_POINT ( 'NONE',  ( -126.5321066302584825, 48.12358255329873913, 84.33085040477796213 ) ) ;
#15162=CARTESIAN_POINT ( 'NONE',  ( -165.6210506643949145, 79.15024150453838558, -15.06613721450044885 ) ) ;
#15163=DIRECTION ( 'NONE',  ( -0.000000000000000000, 1.000000000000000000, -0.000000000000000000 ) ) ;
#15164=CARTESIAN_POINT ( 'NONE',  ( 64.94794467308301478, 13.12874966082101835, 44.57620359267861687 ) ) ;
#15165=CARTESIAN_POINT ( 'NONE',  ( 14.48805533322835792, 7.468382295965534823, 83.78772674431218093 ) ) ;
#15166=ORIENTED_EDGE ( 'NONE', *, *, #7656, .T. ) ;
#15167=LINE ( 'NONE', #22085, #22444 ) ;
#15168=CARTESIAN_POINT ( 'NONE',  ( -97.88309373898363219, 30.60238467438961862, 58.76896769614690896 ) ) ;
#15170=CARTESIAN_POINT ( 'NONE',  ( -84.96580414052107244, 24.82184094495580595, 15.15151241668911730 ) ) ;
#15174=ORIENTED_EDGE ( 'NONE', *, *, #7996, .F. ) ;
#15178=CARTESIAN_POINT ( 'NONE',  ( 12.69192874957004413, 6.421326776602847453, -49.85437527733665775 ) ) ;
#15179=CARTESIAN_POINT ( 'NONE',  ( -179.2177980985565000, 94.18084789436636584, 60.79021173935545619 ) ) ;
#15181=CARTESIAN_POINT ( 'NONE',  ( 126.3541873520044021, 37.07520218256171773, 63.35537632752008363 ) ) ;
#15182=AXIS2_PLACEMENT_3D ( 'NONE', #18067, #13142, #34606 ) ;
#15185=CARTESIAN_POINT ( 'NONE',  ( -33.04857881320337754, 9.860948377235466467, 84.07333317060516720 ) ) ;
#15186=CARTESIAN_POINT ( 'NONE',  ( 154.4550750032601343, 55.34393534448155805, 43.78048194385345937 ) ) ;
#15188=DIRECTION ( 'NONE',  ( -0.000000000000000000, 1.000000000000000000, -0.000000000000000000 ) ) ;
#15189=CARTESIAN_POINT ( 'NONE',  ( 102.8518012651273494, 25.61025413220827573, -42.12408111876868588 ) ) ;
#15190=CARTESIAN_POINT ( 'NONE',  ( -28.35330809568272059, 9.105138953156457049, 44.55656940449198089 ) ) ;
#15191=CARTESIAN_POINT ( 'NONE',  ( -143.7133518487516994, 60.70463114991427034, -64.38850710249009524 ) ) ;
#15194=CARTESIAN_POINT ( 'NONE',  ( -80.54915509118112027, 24.12810583352862537, -76.72378030112859904 ) ) ;
#15195=CARTESIAN_POINT ( 'NONE',  ( 173.8623159076319666, 72.97967239795019623, 7.919453758277684940 ) ) ;
#15198=CARTESIAN_POINT ( 'NONE',  ( 132.0440382699654833, 40.34028297386453943, 2.873803673234553990 ) ) ;
#15199=CARTESIAN_POINT ( 'NONE',  ( -156.9910258076866114, 70.79617246506499839, 10.80262140621922384 ) ) ;
#15200=CARTESIAN_POINT ( 'NONE',  ( 197.2746525007791547, 98.29263840007783415, 91.49113674313775846 ) ) ;
#15201=CARTESIAN_POINT ( 'NONE',  ( 208.5936709733498446, 113.6229123546138169, 30.28492877757630453 ) ) ;
#15202=CARTESIAN_POINT ( 'NONE',  ( 163.7464701930790056, 62.69993100427431898, 5.927907296324478992 ) ) ;
#15205=DIRECTION ( 'NONE',  ( 0.000000000000000000, 0.000000000000000000, 1.000000000000000000 ) ) ;
#15211=CARTESIAN_POINT ( 'NONE',  ( -170.2856292770789537, 85.50720222068223109, 31.36520312212658723 ) ) ;
#15213=CARTESIAN_POINT ( 'NONE',  ( 134.3182571105338639, 42.88121222759019702, -36.02331093239565973 ) ) ;
#15215=B_SPLINE_CURVE_WITH_KNOTS ( 'NONE', 3,
 ( #54303, #1212, #65588, #5098, #37799, #865, #512, #48324, #53618, #33233, #38860, #157, #27237, #12122, #60301, #21963, #43410, #69457, #49381, #42726, #33585, #6492, #64181, #48670, #47993, #22664, #59936, #5779, #16688, #21277, #11396, #6125, #58898, #64887, #64533, #32521, #16343, #32187, #59246, #59580, #38493, #15994, #43061, #10713 ),
 .UNSPECIFIED., .F., .F.,
 ( 4, 2, 2, 2, 2, 2, 2, 2, 2, 2, 2, 2, 2, 2, 2, 2, 2, 2, 2, 2, 2, 4 ),
 ( 1.387778780781445676E-17, 0.003433139681083760119, 0.004291424601354644312, 0.005149709521625528072, 0.006866279362167280846, 0.007724564282438147259, 0.008582849202709011069, 0.009441134122979876614, 0.01029941904325074216, 0.01201598888379252009, 0.01373255872433429801, 0.01459084364460518611, 0.01544912856487607768, 0.01630741348514696751, 0.01716569840541785907, 0.01888226824595965608, 0.02059883808650145309, 0.02145712300677238282, 0.02231540792704331602, 0.02403197776758509915, 0.02574854760812688229, 0.02746511744866866542 ),
 .UNSPECIFIED. ) ;
#15216=LINE ( 'NONE', #47550, #1193 ) ;
#15218=DIRECTION ( 'NONE',  ( -0.000000000000000000, 1.000000000000000000, -0.000000000000000000 ) ) ;
#15222=CARTESIAN_POINT ( 'NONE',  ( 180.6785550066271924, 79.62522105737480160, 82.98728187965927816 ) ) ;
#15224=CARTESIAN_POINT ( 'NONE',  ( 126.6904219525097659, 38.41566710102375737, -95.00000000000133582 ) ) ;
#15228=CARTESIAN_POINT ( 'NONE',  ( 92.20490818459940385, 22.47175429302964034, 15.40764561472821015 ) ) ;
#15230=AXIS2_PLACEMENT_3D ( 'NONE', #40506, #46471, #68291 ) ;
#15231=DIRECTION ( 'NONE',  ( -0.000000000000000000, 1.000000000000000000, -0.000000000000000000 ) ) ;
#15234=CARTESIAN_POINT ( 'NONE',  ( 93.33480479917550099, 21.81892021443992746, -13.07991783598629532 ) ) ;
#15245=CARTESIAN_POINT ( 'NONE',  ( 126.8114659053430842, 38.48351437375814754, 7.542840871000518810 ) ) ;
#15248=CARTESIAN_POINT ( 'NONE',  ( 157.0316110297313230, 58.58403635656375741, 71.25401806271707983 ) ) ;
#15249=CARTESIAN_POINT ( 'NONE',  ( 63.01563776193091826, -170.0000000000000000, 37.31296093922129131 ) ) ;
#15250=DIRECTION ( 'NONE',  ( -0.000000000000000000, 1.000000000000000000, -0.000000000000000000 ) ) ;
#15253=CARTESIAN_POINT ( 'NONE',  ( 157.4703587214989113, 58.92748579479259519, -62.96873488960130771 ) ) ;
#15254=CARTESIAN_POINT ( 'NONE',  ( -62.48965350618344416, 16.80247907725181733, 65.66443840238910923 ) ) ;
#15257=CARTESIAN_POINT ( 'NONE',  ( 46.69842531913727157, 10.49021410897251272, 92.86971545278713336 ) ) ;
#15258=CARTESIAN_POINT ( 'NONE',  ( -180.6209440844958181, 95.88392769199010957, -68.73652789255280027 ) ) ;
#15260=EDGE_CURVE ( 'NONE', #30857, #41100, #32602, .T. ) ;
#15264=CARTESIAN_POINT ( 'NONE',  ( 32.09567473596477782, 7.571373529017940029, -14.56364366973223845 ) ) ;
#15266=CARTESIAN_POINT ( 'NONE',  ( 164.9797987607189214, 63.73352393706674235, 90.52080388245950360 ) ) ;
#15267=CARTESIAN_POINT ( 'NONE',  ( 93.61951000632932107, 21.92572933971849025, 34.48277232936159464 ) ) ;
#15271=AXIS2_PLACEMENT_3D ( 'NONE', #34163, #66874, #44706 ) ;
#15272=CARTESIAN_POINT ( 'NONE',  ( 9.290502160020466249, 6.379616279862541539, 60.60564355645543344 ) ) ;
#15273=DIRECTION ( 'NONE',  ( -0.000000000000000000, 1.000000000000000000, -0.000000000000000000 ) ) ;
#15274=CARTESIAN_POINT ( 'NONE',  ( 203.9203998321607969, 106.9845510704142413, 44.17774257179522124 ) ) ;
#15275=CARTESIAN_POINT ( 'NONE',  ( 79.26746824650808776, 17.03912548276234773, 89.42829496025042602 ) ) ;
#15277=CYLINDRICAL_SURFACE ( 'NONE', #14086, 7.500000000000020428 ) ;
#15283=CARTESIAN_POINT ( 'NONE',  ( 113.8626313173126334, 31.71036178495293711, -63.68104293568552521 ) ) ;
#15285=CARTESIAN_POINT ( 'NONE',  ( 204.6977192012829789, 106.3443248447423599, -78.17048162308530834 ) ) ;
#15288=DIRECTION ( 'NONE',  ( -0.000000000000000000, 1.000000000000000000, -0.000000000000000000 ) ) ;
#15290=CARTESIAN_POINT ( 'NONE',  ( 151.1873096904021736, 52.92629247302097184, -66.36498583336128831 ) ) ;
#15294=ORIENTED_EDGE ( 'NONE', *, *, #47825, .F. ) ;
#15298=CARTESIAN_POINT ( 'NONE',  ( -85.75002235020433261, 26.23806300442547723, -40.13818612277900399 ) ) ;
#15299=CARTESIAN_POINT ( 'NONE',  ( 160.9241720448058857, 60.38677655937334521, 70.42760667945063346 ) ) ;
#15300=CARTESIAN_POINT ( 'NONE',  ( 116.0822834687217409, 32.80169113915576418, -11.84535301537962937 ) ) ;
#15302=CARTESIAN_POINT ( 'NONE',  ( 184.3994103300443328, 82.02159554764422467, -36.98265584704628139 ) ) ;
#15304=CARTESIAN_POINT ( 'NONE',  ( -151.7334413882332456, 67.42499880430109727, 84.72756373490047110 ) ) ;
#15309=CARTESIAN_POINT ( 'NONE',  ( 90.78038362056545907, 21.94937144186732425, -90.75119527580173440 ) ) ;
#15311=CARTESIAN_POINT ( 'NONE',  ( -33.38294402636583413, 10.93918551420888363, -62.40138409474297987 ) ) ;
#15312=CARTESIAN_POINT ( 'NONE',  ( 201.9822477997853412, 104.3642793804899753, 56.54934032291012613 ) ) ;
#15313=CARTESIAN_POINT ( 'NONE',  ( 33.44527180510248598, 7.709232309484707280, 59.67497009447234291 ) ) ;
#15318=CARTESIAN_POINT ( 'NONE',  ( -120.4816138481824908, 43.03185659245511374, 6.060518139089774436 ) ) ;
#15327=CARTESIAN_POINT ( 'NONE',  ( 188.5662303205146770, 86.51341602961787203, 10.56255491576774830 ) ) ;
#15330=CARTESIAN_POINT ( 'NONE',  ( 174.9053416555736646, 72.57849647436445650, 32.52690113457052234 ) ) ;
#15339=CARTESIAN_POINT ( 'NONE',  ( 199.7291770695761102, 101.4092159658447230, 15.48654468859881561 ) ) ;
#15342=CARTESIAN_POINT ( 'NONE',  ( 117.4696399285658970, 32.37118663718648293, 61.88302862921270275 ) ) ;
#15344=ORIENTED_EDGE ( 'NONE', *, *, #50688, .F. ) ;
#15350=CARTESIAN_POINT ( 'NONE',  ( 93.70675391435746349, 21.95852801827565060, -45.81628112151712173 ) ) ;
#15352=ORIENTED_EDGE ( 'NONE', *, *, #22534, .F. ) ;
#15356=CARTESIAN_POINT ( 'NONE',  ( -118.3960663196801306, 41.75130200162922023, -16.13710083091054059 ) ) ;
#15357=CARTESIAN_POINT ( 'NONE',  ( 39.40195752203892710, 8.409560354027400209, 29.91383430596324899 ) ) ;
#15358=CARTESIAN_POINT ( 'NONE',  ( -179.2262621278718200, 94.19039042964669761, -10.98208730704558533 ) ) ;
#15359=CARTESIAN_POINT ( 'NONE',  ( -143.2464978228199470, 59.04559547356110016, -38.17535989881711345 ) ) ;
#15361=CARTESIAN_POINT ( 'NONE',  ( -108.1267491639865028, 36.99658152819874601, 86.96702877733119408 ) ) ;
#15363=ORIENTED_EDGE ( 'NONE', *, *, #61745, .F. ) ;
#15365=CARTESIAN_POINT ( 'NONE',  ( -133.3316503378478046, 52.82738260200862612, -70.36155835367432587 ) ) ;
#15366=CARTESIAN_POINT ( 'NONE',  ( 55.76286625948333864, 11.10663164471739606, -95.00000000000133582 ) ) ;
#15367=CARTESIAN_POINT ( 'NONE',  ( -95.86612279493098754, 29.64021615886203520, 15.06998184580957201 ) ) ;
#15368=CARTESIAN_POINT ( 'NONE',  ( -95.19652294162980866, 29.32558722310179888, -66.84180561699812984 ) ) ;
#15369=VERTEX_POINT ( 'NONE', #50526 ) ;
#15372=CARTESIAN_POINT ( 'NONE',  ( 181.5127080940606845, 79.03904173130082711, -63.06960825634329382 ) ) ;
#15373=CARTESIAN_POINT ( 'NONE',  ( -173.1211646369891071, 87.12891641440859303, -34.71195716474998960 ) ) ;
#15376=CARTESIAN_POINT ( 'NONE',  ( 109.3047140914111708, 29.55674059952507804, -62.81089258595097391 ) ) ;
#15377=CARTESIAN_POINT ( 'NONE',  ( -71.97658551692140350, 20.95070248419150971, 34.51833332167712598 ) ) ;
#15379=CARTESIAN_POINT ( 'NONE',  ( 79.53408731553405175, 17.12082763744058767, 39.69320813087158228 ) ) ;
#15381=CARTESIAN_POINT ( 'NONE',  ( 69.35866309798979046, 15.27376159675663203, -39.21109914877717273 ) ) ;
#15382=CARTESIAN_POINT ( 'NONE',  ( 181.0840389613909736, -170.0000000000000000, -89.91415884680696990 ) ) ;
#15385=CYLINDRICAL_SURFACE ( 'NONE', #22063, 7.500000000000013323 ) ;
#15390=CARTESIAN_POINT ( 'NONE',  ( 79.13041963748371188, 18.04952109592811738, 63.53642847383714098 ) ) ;
#15391=CARTESIAN_POINT ( 'NONE',  ( -79.51308867657013479, 22.64556585543077105, -88.84041300975997046 ) ) ;
#15393=CARTESIAN_POINT ( 'NONE',  ( -173.1211646369891071, 87.12891641440859303, 45.82169460664104577 ) ) ;
#15396=CARTESIAN_POINT ( 'NONE',  ( -95.86163447241558799, 30.75089131639700213, -73.27107820499439583 ) ) ;
#15397=CARTESIAN_POINT ( 'NONE',  ( -38.80621516088655198, 11.94263260276895267, -14.50409165160439606 ) ) ;
#15400=VERTEX_POINT ( 'NONE', #13584 ) ;
#15403=CARTESIAN_POINT ( 'NONE',  ( -30.47069031368414826, 9.433993659086572947, 3.418604320433936472 ) ) ;
#15406=CARTESIAN_POINT ( 'NONE',  ( -13.78293860383720038, 7.352367295275509029, -65.17994511467486518 ) ) ;
#15409=CARTESIAN_POINT ( 'NONE',  ( 150.9128604434957595, 53.97103482421771048, -47.30234765383832496 ) ) ;
#15411=ORIENTED_EDGE ( 'NONE', *, *, #12389, .F. ) ;
#15414=CARTESIAN_POINT ( 'NONE',  ( 141.0229350107040887, 47.12561858623062960, -95.00000000000133582 ) ) ;
#15415=CARTESIAN_POINT ( 'NONE',  ( 174.2538192999569731, 73.34752463892030505, -19.99058039971637513 ) ) ;
#15420=CARTESIAN_POINT ( 'NONE',  ( -1.728570918131775436, 6.570609986804681668, -20.44832033284899353 ) ) ;
#15423=CARTESIAN_POINT ( 'NONE',  ( -142.4971084705952649, 58.45403049551539709, 89.22328903718332072 ) ) ;
#15424=VECTOR ( 'NONE', #2083, 1000.000000000000000 ) ;
#15426=EDGE_CURVE ( 'NONE', #38200, #26520, #10792, .T. ) ;
#15429=CARTESIAN_POINT ( 'NONE',  ( 84.74089592029042706, 19.84571403269346135, 3.105186560012996200 ) ) ;
#15431=CARTESIAN_POINT ( 'NONE',  ( 63.01563776193091826, -170.0000000000000000, -16.37614024170606797 ) ) ;
#15432=CARTESIAN_POINT ( 'NONE',  ( 155.2992895652388086, 57.24699634758580657, 29.71672381646145311 ) ) ;
#15433=CARTESIAN_POINT ( 'NONE',  ( -101.3537077702550562, 33.43904726487055967, 45.47600929637822986 ) ) ;
#15434=EDGE_CURVE ( 'NONE', #3067, #41100, #68762, .T. ) ;
#15440=CARTESIAN_POINT ( 'NONE',  ( 173.6024011093110744, 72.73634049052006390, 63.05001675959219654 ) ) ;
#15443=CARTESIAN_POINT ( 'NONE',  ( -71.43874587651173158, 19.69883891272894516, -17.78934971970884149 ) ) ;
#15445=CARTESIAN_POINT ( 'NONE',  ( -60.13226458141418362, 16.10241298991027037, 43.34078196804391325 ) ) ;
#15446=DIRECTION ( 'NONE',  ( -0.000000000000000000, 1.000000000000000000, -0.000000000000000000 ) ) ;
#15448=CARTESIAN_POINT ( 'NONE',  ( -179.8996803435689174, 95.00451760716445904, 41.54311889901401145 ) ) ;
#15453=B_SPLINE_CURVE_WITH_KNOTS ( 'NONE', 3,
 ( #52127, #3260, #20121, #46153, #57405, #41572, #25065, #51786, #19422, #18739, #8540, #66946, #61647, #25415, #56365, #14834, #9224, #36302, #35263, #57756, #9572, #52473, #40199, #3597, #13465, #8187, #13801, #34923, #29632, #51101, #2910, #24373, #45817, #67296, #19080, #40532, #40881, #61984, #56721, #29987, #46495, #67628, #67978, #62343 ),
 .UNSPECIFIED., .F., .F.,
 ( 4, 2, 2, 2, 2, 2, 2, 2, 2, 2, 2, 2, 2, 2, 2, 2, 2, 2, 2, 2, 2, 4 ),
 ( 0.02416815208377489851, 0.02567033257376874489, 0.02642142281876567328, 0.02717251306376259820, 0.02867469355375640988, 0.02942578379875333480, 0.03017687404375025625, 0.03167905453374411651, 0.03318123502373797329, 0.03393232526873489474, 0.03468341551373183007, 0.03618559600372571461, 0.03693668624872264300, 0.03768777649371957139, 0.03918995698371341430, 0.04069213747370725720, 0.04219431796370110010, 0.04369649845369494301, 0.04444758869869186446, 0.04519867894368878591, 0.04670085943368267045, 0.04820303992367655499 ),
 .UNSPECIFIED. ) ;
#15455=CARTESIAN_POINT ( 'NONE',  ( 141.2470358420065679, 46.06959063280891087, 65.16002587109025512 ) ) ;
#15457=CARTESIAN_POINT ( 'NONE',  ( 155.2910738464913436, 55.97560547655807994, 56.56338629075234081 ) ) ;
#15458=CARTESIAN_POINT ( 'NONE',  ( 94.02499804464929412, 23.15433260743126453, 38.48408892620923183 ) ) ;
#15462=CARTESIAN_POINT ( 'NONE',  ( 149.9714610887121466, 53.28792066194168342, -17.08704249943660969 ) ) ;
#15463=CARTESIAN_POINT ( 'NONE',  ( 209.6642862813004911, 115.2127693334914085, -22.61907644621658164 ) ) ;
#15464=DIRECTION ( 'NONE',  ( 0.000000000000000000, 0.000000000000000000, 1.000000000000000000 ) ) ;
#15467=CARTESIAN_POINT ( 'NONE',  ( 69.85706361178125690, 14.36422398738209161, 87.91050011282558785 ) ) ;
#15470=FACE_OUTER_BOUND ( 'NONE', #32745, .T. ) ;
#15475=EDGE_LOOP ( 'NONE', ( #45403, #65208, #16648, #4174 ) ) ;
#15477=CARTESIAN_POINT ( 'NONE',  ( 206.6955592216990567, 109.1214665502617720, -77.91101188158484092 ) ) ;
#15478=CARTESIAN_POINT ( 'NONE',  ( 43.14565945994674223, 9.942782559600559011, -22.77872216780330916 ) ) ;
#15485=CARTESIAN_POINT ( 'NONE',  ( -75.43953471071002070, 21.11829282998123958, 57.97565906622840970 ) ) ;
#15491=CARTESIAN_POINT ( 'NONE',  ( -155.5978531700835674, 69.52241200678679434, 42.60492188881196540 ) ) ;
#15494=EDGE_CURVE ( 'NONE', #1914, #37583, #24276, .T. ) ;
#15495=DIRECTION ( 'NONE',  ( 0.000000000000000000, 0.000000000000000000, 1.000000000000000000 ) ) ;
#15499=ORIENTED_EDGE ( 'NONE', *, *, #30895, .F. ) ;
#15501=CARTESIAN_POINT ( 'NONE',  ( -133.3923804760466112, 52.87100816290224969, 37.55266435330955233 ) ) ;
#15502=ORIENTED_EDGE ( 'NONE', *, *, #41580, .F. ) ;
#15503=CARTESIAN_POINT ( 'NONE',  ( 33.93974911725171495, 8.773765372885575786, -21.42055978403731942 ) ) ;
#15504=CARTESIAN_POINT ( 'NONE',  ( 185.4510914867138354, 84.60702097455163084, -91.30541823130347723 ) ) ;
#15505=CARTESIAN_POINT ( 'NONE',  ( 56.19211641164837090, 11.19288081156168424, 61.03486635809458960 ) ) ;
#15506=CARTESIAN_POINT ( 'NONE',  ( -2.177337698256115672, 7.595833446947581002, 69.41885401754487361 ) ) ;
#15507=CARTESIAN_POINT ( 'NONE',  ( 15.78827728214693416, 7.507518794609588042, 3.170157082241545687 ) ) ;
#15512=DIRECTION ( 'NONE',  ( -0.000000000000000000, 1.000000000000000000, -0.000000000000000000 ) ) ;
#15514=CARTESIAN_POINT ( 'NONE',  ( 70.11438327604406595, 14.43198353181102789, 39.74598324287578066 ) ) ;
#15516=CARTESIAN_POINT ( 'NONE',  ( 8.467009815279766372, 7.382848975951745274, 92.86400164404348345 ) ) ;
#15518=EDGE_CURVE ( 'NONE', #629, #37519, #41512, .T. ) ;
#15520=CARTESIAN_POINT ( 'NONE',  ( -96.76159256735193992, 30.06445763698413032, 69.96622681954906398 ) ) ;
#15521=VERTEX_POINT ( 'NONE', #22660 ) ;
#15527=CARTESIAN_POINT ( 'NONE',  ( -118.5151419614604578, 43.00218563933589166, 12.64493271249231654 ) ) ;
#15528=CARTESIAN_POINT ( 'NONE',  ( -178.7458319892714087, 93.61502008198024782, 70.13378254355463071 ) ) ;
#15530=CARTESIAN_POINT ( 'NONE',  ( 19.75784582661441391, 6.660183274347841298, 17.03828975487343556 ) ) ;
#15531=EDGE_LOOP ( 'NONE', ( #14463, #46753, #45833, #65304 ) ) ;
#15532=CARTESIAN_POINT ( 'NONE',  ( -33.66596729176688996, 9.967356680381493916, 84.23666802118060559 ) ) ;
#15533=CIRCLE ( 'NONE', #919, 243.4957430088094839 ) ;
#15534=CARTESIAN_POINT ( 'NONE',  ( 150.0433793199863146, 52.09973307442955814, 35.82920141195970842 ) ) ;
#15536=CARTESIAN_POINT ( 'NONE',  ( 103.5588133492864955, 25.91050225236391569, -46.86172722952704817 ) ) ;
#15538=CARTESIAN_POINT ( 'NONE',  ( -29.49620345460275317, 9.280093073089041411, 44.97709496270313423 ) ) ;
#15544=CARTESIAN_POINT ( 'NONE',  ( -118.7011544766493500, 43.11604763363183679, -40.27239875278853987 ) ) ;
#15545=CARTESIAN_POINT ( 'NONE',  ( -78.66644367742111399, 23.39876645725285798, 18.57365054920947500 ) ) ;
#15547=CARTESIAN_POINT ( 'NONE',  ( -156.6819053601226415, 70.51177710383655040, 13.63498518674871107 ) ) ;
#15548=CARTESIAN_POINT ( 'NONE',  ( -122.3994536713185255, 45.42826354555017332, -62.61790137560624459 ) ) ;
#15550=FACE_OUTER_BOUND ( 'NONE', #14070, .T. ) ;
#15551=CARTESIAN_POINT ( 'NONE',  ( -86.10360257264196093, 26.38663017581290404, 65.76492460684757191 ) ) ;
#15552=CARTESIAN_POINT ( 'NONE',  ( -105.8768181937898873, 34.64545164169051361, 44.61740776510733042 ) ) ;
#15556=CARTESIAN_POINT ( 'NONE',  ( -61.76967730161514680, 17.63609381203634641, 88.10797299145480110 ) ) ;
#15559=ORIENTED_EDGE ( 'NONE', *, *, #29174, .F. ) ;
#15560=CARTESIAN_POINT ( 'NONE',  ( 15.78827728214693771, 7.507518794609575608, -62.36349468914946925 ) ) ;
#15565=CARTESIAN_POINT ( 'NONE',  ( -49.12372073857198984, 14.20664392157176081, -74.18029338664986483 ) ) ;
#15572=CARTESIAN_POINT ( 'NONE',  ( 8.000000000000007105, 249.8719672152120381, 94.99999999999866418 ) ) ;
#15580=EDGE_CURVE ( 'NONE', #66935, #45299, #49408, .T. ) ;
#15584=CARTESIAN_POINT ( 'NONE',  ( 208.0306608271318112, 112.7988899307265456, 3.141066733790039311 ) ) ;
#15586=CARTESIAN_POINT ( 'NONE',  ( 90.30166390191402570, 20.70652093100729374, -23.03453807668526565 ) ) ;
#15587=CARTESIAN_POINT ( 'NONE',  ( 204.6977192012829789, 106.3443248447423599, -24.48138044215792419 ) ) ;
#15593=CYLINDRICAL_SURFACE ( 'NONE', #28496, 7.500000000000013323 ) ;
#15594=FACE_OUTER_BOUND ( 'NONE', #29501, .T. ) ;
#15596=CARTESIAN_POINT ( 'NONE',  ( -10.07362276049133953, 8.056690395595460075, 84.14207705956837913 ) ) ;
#15598=ADVANCED_FACE ( 'NONE', ( #32492 ), #32835, .F. ) ;
#15603=CARTESIAN_POINT ( 'NONE',  ( 36.21632519057887833, 9.028958671447663065, 84.28089839341768652 ) ) ;
#15604=CARTESIAN_POINT ( 'NONE',  ( -179.5082312244189211, 94.53075638132055758, -72.99655709447104357 ) ) ;
#15605=CYLINDRICAL_SURFACE ( 'NONE', #68446, 7.500000000000020428 ) ;
#15607=CARTESIAN_POINT ( 'NONE',  ( 15.78827728214693416, -170.0000000000000000, -43.01894409868580027 ) ) ;
#15608=CARTESIAN_POINT ( 'NONE',  ( 157.4703587214989398, -170.0000000000000000, -70.46873488960132192 ) ) ;
#15609=CARTESIAN_POINT ( 'NONE',  ( -5.879983509979045841, 7.779504553499513975, 3.511211028316594707 ) ) ;
#15610=CARTESIAN_POINT ( 'NONE',  ( 178.1965488566140436, 77.14488558164484289, -50.66031209579180228 ) ) ;
#15613=ORIENTED_EDGE ( 'NONE', *, *, #45094, .T. ) ;
#15614=CARTESIAN_POINT ( 'NONE',  ( 103.0124792097646349, 26.77148435100179569, -18.63633658775954061 ) ) ;
#15615=FACE_OUTER_BOUND ( 'NONE', #35056, .T. ) ;
#15616=CARTESIAN_POINT ( 'NONE',  ( 9.837735240994037511, 7.389327806910500840, 32.94284116154079811 ) ) ;
#15617=CARTESIAN_POINT ( 'NONE',  ( 197.6341357773624452, 98.74251867088338486, 39.24647996897417102 ) ) ;
#15619=CYLINDRICAL_SURFACE ( 'NONE', #33224, 7.500000000000013323 ) ;
#15621=ORIENTED_EDGE ( 'NONE', *, *, #47260, .T. ) ;
#15624=EDGE_CURVE ( 'NONE', #47669, #47023, #17518, .T. ) ;
#15626=CARTESIAN_POINT ( 'NONE',  ( 115.0606351894211485, 32.29586232625066344, -76.03609025758434825 ) ) ;
#15630=EDGE_CURVE ( 'NONE', #39142, #42011, #24380, .T. ) ;
#15631=CARTESIAN_POINT ( 'NONE',  ( -15.32495246574475090, 8.506829480038508251, -16.57547917308654206 ) ) ;
#15633=CARTESIAN_POINT ( 'NONE',  ( 157.4703587214989113, 57.65129005721576760, -77.96873488960135035 ) ) ;
#15635=CARTESIAN_POINT ( 'NONE',  ( -156.7487895666416478, 70.57327586518564999, -44.28588653070858783 ) ) ;
#15638=CARTESIAN_POINT ( 'NONE',  ( 70.45451534980408326, 15.56315969138428379, -17.36384710539488552 ) ) ;
#15639=ADVANCED_FACE ( 'NONE', ( #45471 ), #19086, .F. ) ;
#15640=CARTESIAN_POINT ( 'NONE',  ( -62.41990535723909517, 17.83270318706536983, -95.00000000000133582 ) ) ;
#15641=CARTESIAN_POINT ( 'NONE',  ( 109.6602010289487055, 28.61221948077516686, 83.29575177580451850 ) ) ;
#15642=CARTESIAN_POINT ( 'NONE',  ( -156.4797890011541881, 71.69341087347116570, 8.599111263860363508 ) ) ;
#15643=CARTESIAN_POINT ( 'NONE',  ( 188.5662303205147055, 86.51341602961788624, -43.12654626515958967 ) ) ;
#15644=CARTESIAN_POINT ( 'NONE',  ( 21.44031696305385637, 6.747195267824410259, 42.46889706688644850 ) ) ;
#15645=CARTESIAN_POINT ( 'NONE',  ( -156.5226901298209725, 71.73305092143021966, 89.25176612992051162 ) ) ;
#15650=CARTESIAN_POINT ( 'NONE',  ( 92.56307064175635446, 22.60487289243135223, -92.40539893235690272 ) ) ;
#15658=CARTESIAN_POINT ( 'NONE',  ( 185.5457097283154440, 84.70846743303872017, 69.69978301039404300 ) ) ;
#15659=CARTESIAN_POINT ( 'NONE',  ( 12.03194517566456057, 6.409266703743584870, -9.664381073535908584 ) ) ;
#15660=B_SPLINE_CURVE_WITH_KNOTS ( 'NONE', 3,
 ( #17266, #44713, #66191, #16919, #38383, #66533, #7073, #49619, #49268, #38740, #1450, #59824, #60184, #17984, #1102, #54190, #22553, #12003, #33477, #22904, #44350, #34168, #28531, #65833, #60539, #17629, #12353, #49980, #38035, #33810, #60881, #12703, #55606, #7436, #50339, #59479, #11290, #56649, #13738, #8118 ),
 .UNSPECIFIED., .F., .F.,
 ( 4, 2, 2, 2, 2, 2, 2, 2, 2, 2, 2, 2, 2, 2, 2, 2, 2, 2, 2, 4 ),
 ( 0.02454308262169001276, 0.02608670964102879908, 0.02685852315069820612, 0.02763033666036761662, 0.02917396367970642723, 0.02994577718937583427, 0.03071759069904523784, 0.03226121771838406926, 0.03303303122805349018, 0.03380484473772291804, 0.03534847175706176681, 0.03689209877640062252, 0.03843572579573947129, 0.03997935281507832006, 0.04152297983441717577, 0.04306660685375602454, 0.04461023387309488719, 0.04615386089243374984, 0.04769748791177261249, 0.04924111493111147514 ),
 .UNSPECIFIED. ) ;
#15662=CARTESIAN_POINT ( 'NONE',  ( 182.5617509987553433, 80.11195108039726165, 56.29705353328592565 ) ) ;
#15664=CARTESIAN_POINT ( 'NONE',  ( -79.14678386417813272, 22.50468917936073154, -35.11545063171787717 ) ) ;
#15665=CARTESIAN_POINT ( 'NONE',  ( 18.21423326326596381, 6.590134686181386314, 71.47284841903351094 ) ) ;
#15667=CARTESIAN_POINT ( 'NONE',  ( 69.36122620657974380, 15.27447566922079858, 94.99999999999866418 ) ) ;
#15673=FACE_OUTER_BOUND ( 'NONE', #47950, .T. ) ;
#15674=CARTESIAN_POINT ( 'NONE',  ( -108.0902552660050731, 36.97681740369924341, -47.28325963604802951 ) ) ;
#15679=CARTESIAN_POINT ( 'NONE',  ( -30.94753041835916818, 9.510749728915508072, -8.472646774738157305 ) ) ;
#15680=CARTESIAN_POINT ( 'NONE',  ( 174.4089829827045435, 72.11302376861458185, 93.92229883193532203 ) ) ;
#15682=CARTESIAN_POINT ( 'NONE',  ( -31.43908319763710679, -170.0000000000000000, 10.87190381572550280 ) ) ;
#15683=ORIENTED_EDGE ( 'NONE', *, *, #15630, .T. ) ;
#15684=CARTESIAN_POINT ( 'NONE',  ( 130.3035708464390154, 40.48418876551454559, -63.74550792924027576 ) ) ;
#15685=DIRECTION ( 'NONE',  ( -1.000000000000000000, 0.000000000000000000, 0.000000000000000000 ) ) ;
#15686=B_SPLINE_CURVE_WITH_KNOTS ( 'NONE', 3,
 ( #19663, #29879, #67866, #62927, #14043, #51340, #14400, #19315, #4523, #3836, #9809, #24612, #30923, #25307, #68210, #20020, #41474, #52696, #14727, #56603, #68546, #36542, #68871, #57651, #67516, #20695, #46046, #42156, #40770, #9462, #20348, #56963, #52367, #4183, #25652, #30230, #3485, #41817 ),
 .UNSPECIFIED., .F., .F.,
 ( 4, 2, 2, 2, 2, 2, 2, 2, 2, 2, 2, 2, 2, 2, 2, 2, 2, 2, 4 ),
 ( 0.000000000000000000, 0.003908178031105456751, 0.005862267046658146095, 0.007816356062210835440, 0.009770445077763523917, 0.01172453409331621413, 0.01270157860109255230, 0.01367862310886889046, 0.01465566761664522863, 0.01563271212442156680, 0.01660975663219790843, 0.01758680113997424660, 0.01954089015552693681, 0.02051793466330329579, 0.02149497917107965825, 0.02344906818663237622, 0.02540315720218510112, 0.02735724621773782256, 0.03126542424884323074 ),
 .UNSPECIFIED. ) ;
#15687=CARTESIAN_POINT ( 'NONE',  ( -24.85653282846401879, 8.603185326828743484, 94.99999999999866418 ) ) ;
#15688=VECTOR ( 'NONE', #1429, 1000.000000000000000 ) ;
#15689=CARTESIAN_POINT ( 'NONE',  ( 163.6501672645067345, 62.62019911992669563, -93.05832839351816688 ) ) ;
#15690=CARTESIAN_POINT ( 'NONE',  ( 90.30166390191405412, 20.70652093100728663, -49.87908866714894884 ) ) ;
#15692=ORIENTED_EDGE ( 'NONE', *, *, #52767, .T. ) ;
#15695=CARTESIAN_POINT ( 'NONE',  ( -118.4553071845215015, 41.78724769484927037, -16.66711030142431937 ) ) ;
#15697=CARTESIAN_POINT ( 'NONE',  ( -177.5259994307673423, 92.16784265327252967, -21.45548079138242059 ) ) ;
#15698=CARTESIAN_POINT ( 'NONE',  ( -169.8972248494843029, 85.08697738648014308, -62.26996028157370944 ) ) ;
#15699=CARTESIAN_POINT ( 'NONE',  ( -145.3279998500303805, 60.71393190715793509, -48.54482469514504572 ) ) ;
#15701=CARTESIAN_POINT ( 'NONE',  ( -109.4616842129796339, 37.73062014485820015, 89.52162112396747773 ) ) ;
#15704=CARTESIAN_POINT ( 'NONE',  ( -128.9786047358386156, 48.55852351614669971, 44.96012683757445672 ) ) ;
#15705=CARTESIAN_POINT ( 'NONE',  ( -125.8938041572051389, -170.0000000000000000, -96.10280507916131398 ) ) ;
#15706=EDGE_CURVE ( 'NONE', #20401, #36151, #51107, .T. ) ;
#15707=CARTESIAN_POINT ( 'NONE',  ( 86.15410276028863734, 19.25894675708890702, -23.97701360844807184 ) ) ;
#15708=CARTESIAN_POINT ( 'NONE',  ( -130.2071229607962835, 50.62285182196875866, -63.10483451847541403 ) ) ;
#15710=EDGE_CURVE ( 'NONE', #63707, #275, #23408, .T. ) ;
#15712=CARTESIAN_POINT ( 'NONE',  ( -94.78109144324895396, 29.13179392050638228, -69.64435539242961681 ) ) ;
#15717=CARTESIAN_POINT ( 'NONE',  ( -172.7116702014380110, 86.67317892691259829, -34.71195716474999671 ) ) ;
#15721=CARTESIAN_POINT ( 'NONE',  ( -76.32456871438918711, 22.51591205926308348, 30.77704971272454770 ) ) ;
#15722=CARTESIAN_POINT ( 'NONE',  ( -71.97171223898807568, 20.94894057408426491, -66.04217098637484185 ) ) ;
#15723=CARTESIAN_POINT ( 'NONE',  ( 66.73431804020511038, 14.60294556126670784, -49.73844288260944069 ) ) ;
#15724=CARTESIAN_POINT ( 'NONE',  ( 46.89016064832838993, 10.52130577388959409, -43.60800750508858670 ) ) ;
#15726=ORIENTED_EDGE ( 'NONE', *, *, #40483, .T. ) ;
#15727=CARTESIAN_POINT ( 'NONE',  ( -104.5730787903383288, 33.96058035148152499, -8.513426699022396349 ) ) ;
#15728=EDGE_LOOP ( 'NONE', ( #11026, #2337, #6739, #25003 ) ) ;
#15729=CARTESIAN_POINT ( 'NONE',  ( -31.43908319763709969, 9.591432048623765638, 3.371903815725488585 ) ) ;
#15731=CARTESIAN_POINT ( 'NONE',  ( -85.34581468285759343, 24.97911134307621950, -92.86422577895648089 ) ) ;
#15732=EDGE_CURVE ( 'NONE', #23369, #55648, #43546, .T. ) ;
#15733=CARTESIAN_POINT ( 'NONE',  ( 151.6192474229129630, 53.24103268919208176, -21.47852014988733060 ) ) ;
#15734=CYLINDRICAL_SURFACE ( 'NONE', #55698, 7.500000000000020428 ) ;
#15735=CARTESIAN_POINT ( 'NONE',  ( 38.91493890549796220, 8.346224043800610559, -77.46436805589146957 ) ) ;
#15738=DIRECTION ( 'NONE',  ( -0.000000000000000000, 1.000000000000000000, -0.000000000000000000 ) ) ;
#15742=CARTESIAN_POINT ( 'NONE',  ( 62.05396267233467711, 13.48332220860127428, 56.70355666220334712 ) ) ;
#15743=CARTESIAN_POINT ( 'NONE',  ( 10.15118267943871722, 7.391905976536037315, -74.81668340143906448 ) ) ;
#15746=CARTESIAN_POINT ( 'NONE',  ( -1.319107422865893442, 6.554467368239795810, 33.85272720924916712 ) ) ;
#15756=CARTESIAN_POINT ( 'NONE',  ( -190.6985136298601731, 109.1272424661242582, 60.81597207375692449 ) ) ;
#15758=CARTESIAN_POINT ( 'NONE',  ( -180.2534575077006593, 95.43481063389138797, 94.35782419044186042 ) ) ;
#15759=ORIENTED_EDGE ( 'NONE', *, *, #9367, .F. ) ;
#15761=CARTESIAN_POINT ( 'NONE',  ( 93.33480479917547257, 21.81892021443992746, 67.45373393540474183 ) ) ;
#15764=CARTESIAN_POINT ( 'NONE',  ( 140.0614732283738135, 45.29930344725072899, 32.78982767501074136 ) ) ;
#15767=DIRECTION ( 'NONE',  ( -0.000000000000000000, 1.000000000000000000, -0.000000000000000000 ) ) ;
#15768=CARTESIAN_POINT ( 'NONE',  ( 160.2883311361769927, 61.16711613734478448, 17.01903432654508563 ) ) ;
#15773=CARTESIAN_POINT ( 'NONE',  ( 179.4227152810058499, 78.36166152262364903, 56.32724963102304372 ) ) ;
#15776=CARTESIAN_POINT ( 'NONE',  ( -105.4556185321791446, 34.42302275449793569, -35.70349811333863244 ) ) ;
#15777=CARTESIAN_POINT ( 'NONE',  ( 66.29961816943398389, 13.45804302849873757, -76.82535056491491332 ) ) ;
#15778=CARTESIAN_POINT ( 'NONE',  ( -58.33245019990697955, 15.58496056636070293, 44.57971224376340302 ) ) ;
#15781=CARTESIAN_POINT ( 'NONE',  ( -177.5271152834790769, 92.16916858125013334, 44.40871575690508166 ) ) ;
#15784=CARTESIAN_POINT ( 'NONE',  ( 112.1009898303695422, 30.86414810229296890, -36.14121760344119849 ) ) ;
#15789=B_SPLINE_CURVE_WITH_KNOTS ( 'NONE', 3,
 ( #54310, #64894, #43764, #873, #11764, #69465, #26905, #32878, #33241, #16694, #22673, #53626, #521, #1220, #6134, #49388, #21284, #6499, #42733, #48331, #27594, #65235, #21624, #165, #43069, #38500, #21970, #59254, #17030, #27946, #5451, #10720, #59944, #54671, #53958, #64190, #16001, #64541, #37450, #32194, #16351, #37807, #43418 ),
 .UNSPECIFIED., .F., .F.,
 ( 4, 2, 2, 2, 2, 2, 2, 2, 1, 2, 2, 2, 2, 2, 2, 2, 2, 2, 2, 2, 2, 4 ),
 ( 0.000000000000000000, 0.001465684626643354044, 0.002198526939965028681, 0.002931369253286704186, 0.004397053879930075578, 0.005862738506573445668, 0.007328423133216816626, 0.008061265446538484758, 0.008794107759860152890, 0.009526950073181819287, 0.01025979238650348742, 0.01172547701314682368, 0.01319116163979015995, 0.01465684626643349621, 0.01538968857975516261, 0.01612253089307683074, 0.01758821551972016353, 0.01905390014636349980, 0.01978674245968516446, 0.02051958477300683259, 0.02198526939965016885, 0.02345095402629350165 ),
 .UNSPECIFIED. ) ;
#15790=CARTESIAN_POINT ( 'NONE',  ( 136.9934874058118055, 43.35050367224291534, 70.68308355397081755 ) ) ;
#15791=CYLINDRICAL_SURFACE ( 'NONE', #20159, 7.500000000000027534 ) ;
#15792=CARTESIAN_POINT ( 'NONE',  ( -38.15923928782687824, 10.79140400702259228, -66.32252006240803155 ) ) ;
#15797=EDGE_CURVE ( 'NONE', #21823, #47361, #20891, .T. ) ;
#15799=CARTESIAN_POINT ( 'NONE',  ( -62.54987051470499182, 16.82069887634177974, 91.89306705351904725 ) ) ;
#15802=CARTESIAN_POINT ( 'NONE',  ( 69.71296738434152473, 14.32639855680324459, 87.60999871946472695 ) ) ;
#15810=CARTESIAN_POINT ( 'NONE',  ( 187.5272808203427530, 85.37192123373903030, 32.93173814286044632 ) ) ;
#15812=CARTESIAN_POINT ( 'NONE',  ( 61.10129719786245772, 12.23677173834305520, -62.80958882113672814 ) ) ;
#15813=CARTESIAN_POINT ( 'NONE',  ( -71.17819443284076897, 19.60909329639482834, 11.56462333534533471 ) ) ;
#15814=CARTESIAN_POINT ( 'NONE',  ( -38.29761368137835120, 10.81775503710270669, -93.35085947631458225 ) ) ;
#15815=CARTESIAN_POINT ( 'NONE',  ( 19.75315861330098244, 7.667327050329334703, 31.14372870632146828 ) ) ;
#15816=CARTESIAN_POINT ( 'NONE',  ( -149.5074843970971301, -170.0000000000000000, -49.81283053149198992 ) ) ;
#15819=CARTESIAN_POINT ( 'NONE',  ( 164.4761273435911164, 64.62485394454748189, -73.19840926013584692 ) ) ;
#15821=CARTESIAN_POINT ( 'NONE',  ( -75.01314391403413140, 20.96328762434826487, 58.19466124245714411 ) ) ;
#15824=ORIENTED_EDGE ( 'NONE', *, *, #44122, .T. ) ;
#15825=CARTESIAN_POINT ( 'NONE',  ( -27.70115495247213744, 10.02455692117576369, -63.14125139223980909 ) ) ;
#15830=EDGE_LOOP ( 'NONE', ( #44729, #21382, #46045, #41071 ) ) ;
#15833=CARTESIAN_POINT ( 'NONE',  ( -132.9227230387960503, 52.53474289881227577, 40.74974517129221852 ) ) ;
#15835=CARTESIAN_POINT ( 'NONE',  ( 206.7099580236348970, 109.1417833474364301, 17.09981171093966168 ) ) ;
#15836=CARTESIAN_POINT ( 'NONE',  ( -143.8634661037141313, 60.82480701605702222, 33.25539283625584375 ) ) ;
#15838=CARTESIAN_POINT ( 'NONE',  ( 55.51547041749725508, 11.05727559334826893, 63.91534904839117814 ) ) ;
#15846=CARTESIAN_POINT ( 'NONE',  ( -167.1540252468942356, 80.72321878831101571, -19.91812675169417801 ) ) ;
#15847=CARTESIAN_POINT ( 'NONE',  ( 139.2921620648437795, 44.80435067172499686, -75.55868156767934352 ) ) ;
#15848=CARTESIAN_POINT ( 'NONE',  ( 63.50528314073025626, 12.78634332146812724, 44.81296093922130552 ) ) ;
#15850=CARTESIAN_POINT ( 'NONE',  ( 21.57321902410670234, 7.762142431058419945, 86.38521836418507860 ) ) ;
#15853=CARTESIAN_POINT ( 'NONE',  ( -95.61819996182570947, 29.52346081122274768, 68.31800957063339297 ) ) ;
#15855=CARTESIAN_POINT ( 'NONE',  ( -76.32962633615589709, 21.44528079176260604, 30.78751738144537953 ) ) ;
#15859=CARTESIAN_POINT ( 'NONE',  ( -120.4666325602656087, 44.20829586446609483, 6.092936465464075191 ) ) ;
#15860=CARTESIAN_POINT ( 'NONE',  ( -179.5082312244188643, 94.53075638132052916, 61.22619585784733687 ) ) ;
#15861=CARTESIAN_POINT ( 'NONE',  ( 127.4953815656694758, 37.71366486045447175, 67.85928618946456936 ) ) ;
#15862=ORIENTED_EDGE ( 'NONE', *, *, #27065, .F. ) ;
#15871=CARTESIAN_POINT ( 'NONE',  ( -27.70005010046228477, 9.007417901453015574, 44.22257959986427522 ) ) ;
#15875=FACE_BOUND ( 'NONE', #43616, .T. ) ;
#15877=CARTESIAN_POINT ( 'NONE',  ( 42.49453823366108196, 8.831814337191470798, 17.40632894816096865 ) ) ;
#15879=CARTESIAN_POINT ( 'NONE',  ( -147.7895256390024485, 64.04409735547015714, -8.113308455688843068 ) ) ;
#15880=CARTESIAN_POINT ( 'NONE',  ( -119.9771613955296772, 43.90337778233485011, -47.02966473605362552 ) ) ;
#15881=CARTESIAN_POINT ( 'NONE',  ( -80.54915509118110606, 24.12810583352862892, 3.809871470262444770 ) ) ;
#15883=CARTESIAN_POINT ( 'NONE',  ( -154.7934364910360046, 68.79594655117533364, 16.70251692308080038 ) ) ;
#15884=CARTESIAN_POINT ( 'NONE',  ( 198.5545530549422608, 99.90438832179273732, 94.71449343778881769 ) ) ;
#15886=CARTESIAN_POINT ( 'NONE',  ( 69.08240197259638649, 14.16210831900842138, 6.051918337674103476 ) ) ;
#15889=CARTESIAN_POINT ( 'NONE',  ( 92.53033045403536505, 22.59263332688195902, -21.13235829536132471 ) ) ;
#15891=CARTESIAN_POINT ( 'NONE',  ( -38.80621516088655198, 11.94263260276894023, 12.34045893885926226 ) ) ;
#15895=B_SPLINE_CURVE_WITH_KNOTS ( 'NONE', 3,
 ( #37386, #5720, #63448, #15257, #47935, #20873, #41642, #32466, #14900, #10655, #4361, #26156, #63098, #9982, #53898, #41984, #69407, #27178, #42332, #58840, #36366, #52538, #68710, #21225, #26844, #4693, #43000, #63795, #20519, #32123, #26500, #37052, #15603, #59181, #42671, #9640, #58490, #57824, #5390, #31434, #64126, #53558, #10311, #52866, #47250, #47587, #48611, #31100, #25822, #36718, #48271, #11004, #69046, #58166 ),
 .UNSPECIFIED., .F., .F.,
 ( 4, 2, 2, 2, 2, 2, 2, 2, 2, 2, 2, 2, 2, 2, 2, 2, 2, 2, 2, 2, 2, 2, 2, 2, 2, 2, 4 ),
 ( 0.000000000000000000, 0.001981879248976703162, 0.002972818873465054527, 0.003963758497953406325, 0.004954698122441758557, 0.005945637746930109054, 0.006936577371418461285, 0.007927516995906812650, 0.009909396244883470276, 0.01189127549386012617, 0.01288221511834845671, 0.01387315474283678553, 0.01486409436732511434, 0.01585503399181344142, 0.01684597361630177023, 0.01783691324079009558, 0.01981879248976678443, 0.02080973211425513406, 0.02180067173874348369, 0.02279161136323183678, 0.02378255098772018641, 0.02477349061220853951, 0.02576443023669689261, 0.02774630948567364044, 0.02972818873465039174, 0.03071912835913878301, 0.03171006798362717427 ),
 .UNSPECIFIED. ) ;
#15896=CARTESIAN_POINT ( 'NONE',  ( 20.74185656603722450, 7.717159106492279541, -75.51655753953751571 ) ) ;
#15898=CARTESIAN_POINT ( 'NONE',  ( -145.5195986658808351, 62.16746116576784686, 58.70931206985594031 ) ) ;
#15899=DIRECTION ( 'NONE',  ( 0.000000000000000000, 0.000000000000000000, 1.000000000000000000 ) ) ;
#15902=EDGE_CURVE ( 'NONE', #44118, #33190, #62005, .T. ) ;
#15903=CARTESIAN_POINT ( 'NONE',  ( 133.8566784816069060, 42.60093787723652525, -36.02331093239566684 ) ) ;
#15904=CARTESIAN_POINT ( 'NONE',  ( 209.2335797101723358, 114.5704254651986957, -91.52982707713782418 ) ) ;
#15906=EDGE_CURVE ( 'NONE', #33777, #54626, #35975, .T. ) ;
#15908=VERTEX_POINT ( 'NONE', #46332 ) ;
#15909=ORIENTED_EDGE ( 'NONE', *, *, #2302, .T. ) ;
#15910=CARTESIAN_POINT ( 'NONE',  ( 69.50572373348796873, 14.27208627753790360, -39.42976292691626128 ) ) ;
#15911=CARTESIAN_POINT ( 'NONE',  ( 173.5812904811884607, 72.71661333629877788, 90.47055245242088972 ) ) ;
#15912=CARTESIAN_POINT ( 'NONE',  ( 133.8566784816069344, -170.0000000000000000, -62.86786152285933582 ) ) ;
#15913=CARTESIAN_POINT ( 'NONE',  ( 66.17193415285930769, 14.46328737281204901, -90.10321091663050197 ) ) ;
#15916=CARTESIAN_POINT ( 'NONE',  ( 184.3966782763552033, 83.48172388049826509, -23.62389823460853222 ) ) ;
#15917=CARTESIAN_POINT ( 'NONE',  ( 207.2640160519426900, 111.6867652229576322, 2.812936537257378244 ) ) ;
#15919=CARTESIAN_POINT ( 'NONE',  ( -173.9548930713591233, 88.06040582145364226, -49.67720558674120923 ) ) ;
#15921=CARTESIAN_POINT ( 'NONE',  ( 206.2980740120524672, 108.5619562183279783, -24.31977854252603422 ) ) ;
#15923=CARTESIAN_POINT ( 'NONE',  ( 164.0073343966822677, 64.23003864582459244, 67.43977445298207840 ) ) ;
#15928=CARTESIAN_POINT ( 'NONE',  ( 153.8224167330182865, 56.12711234192241250, 70.31123550504270270 ) ) ;
#15929=DIRECTION ( 'NONE',  ( 0.000000000000000000, 0.000000000000000000, 1.000000000000000000 ) ) ;
#15930=CARTESIAN_POINT ( 'NONE',  ( 151.1607415860635228, 52.90668588398087024, 5.978490512986149419 ) ) ;
#15931=CARTESIAN_POINT ( 'NONE',  ( -4.667841011628368619, 7.713338668255913966, 84.49383781058769216 ) ) ;
#15932=AXIS2_PLACEMENT_3D ( 'NONE', #16552, #54876, #1781 ) ;
#15933=ORIENTED_EDGE ( 'NONE', *, *, #55086, .F. ) ;
#15934=DIRECTION ( 'NONE',  ( -0.000000000000000000, 1.000000000000000000, -0.000000000000000000 ) ) ;
#15935=CYLINDRICAL_SURFACE ( 'NONE', #4630, 7.500000000000013323 ) ;
#15936=ORIENTED_EDGE ( 'NONE', *, *, #65270, .F. ) ;
#15937=CIRCLE ( 'NONE', #12587, 242.4895526022646379 ) ;
#15944=ORIENTED_EDGE ( 'NONE', *, *, #57210, .F. ) ;
#15946=CARTESIAN_POINT ( 'NONE',  ( -62.45356936877015386, 16.79156452995239945, -70.80215903815181377 ) ) ;
#15948=CARTESIAN_POINT ( 'NONE',  ( 34.45500533947588906, 7.817363290423887001, -10.61686954642301117 ) ) ;
#15949=CARTESIAN_POINT ( 'NONE',  ( 177.0110682437508558, 75.98481089748386808, -50.03885341334632386 ) ) ;
#15950=CARTESIAN_POINT ( 'NONE',  ( -150.3831389294225573, 66.25266777263973950, -76.60930139824938578 ) ) ;
#15955=CARTESIAN_POINT ( 'NONE',  ( -173.1211646369891355, -170.0000000000000000, -69.05650775521368701 ) ) ;
#15957=CARTESIAN_POINT ( 'NONE',  ( 9.280894575734581764, 7.385644305345140381, 33.75376781634191303 ) ) ;
#15958=CARTESIAN_POINT ( 'NONE',  ( 197.2199163281728431, 98.22431253015352581, 36.04431904461028324 ) ) ;
#15960=CARTESIAN_POINT ( 'NONE',  ( -84.60434550335787662, 25.76113146461752379, 87.01482005019980193 ) ) ;
#15962=EDGE_LOOP ( 'NONE', ( #1800, #30542 ) ) ;
#15965=CARTESIAN_POINT ( 'NONE',  ( 116.6681538161788865, 33.09439081574002017, -74.16764814704670528 ) ) ;
#15969=CARTESIAN_POINT ( 'NONE',  ( -13.45956523846225217, 8.333781915634244086, -21.03003943873567394 ) ) ;
#15970=CARTESIAN_POINT ( 'NONE',  ( 150.0433793199862862, 52.09973307442955104, -71.54900094989498882 ) ) ;
#15972=FACE_OUTER_BOUND ( 'NONE', #15531, .T. ) ;
#15973=ORIENTED_EDGE ( 'NONE', *, *, #4660, .F. ) ;
#15975=CARTESIAN_POINT ( 'NONE',  ( 65.39792658623288446, 14.27332852928128304, -9.260399453094194655 ) ) ;
#15978=CARTESIAN_POINT ( 'NONE',  ( -23.97453345597386587, 9.499725116317328855, 90.60705203038679656 ) ) ;
#15979=CARTESIAN_POINT ( 'NONE',  ( -152.9143627383494959, 68.46626892668653852, 18.07331903687195052 ) ) ;
#15981=CARTESIAN_POINT ( 'NONE',  ( 19.74724861314306423, 6.659670522263898107, 31.13995450494594763 ) ) ;
#15983=CARTESIAN_POINT ( 'NONE',  ( -156.9818039471237512, 72.15818689871304059, 91.26512449016922801 ) ) ;
#15984=ORIENTED_EDGE ( 'NONE', *, *, #38284, .T. ) ;
#15988=CARTESIAN_POINT ( 'NONE',  ( 34.83823433017389704, 8.871835168107976344, -49.09195262392610459 ) ) ;
#15989=AXIS2_PLACEMENT_3D ( 'NONE', #41048, #42076, #14321 ) ;
#15990=CARTESIAN_POINT ( 'NONE',  ( -33.84080342750783643, 9.997552308299095358, 57.43914399132651027 ) ) ;
#15991=CARTESIAN_POINT ( 'NONE',  ( -151.2410113808308836, 65.66338888995508682, -22.77829783373973527 ) ) ;
#15993=CARTESIAN_POINT ( 'NONE',  ( 188.4920037102894526, 87.93425473911921131, 64.86267653291690749 ) ) ;
#15994=CARTESIAN_POINT ( 'NONE',  ( -150.3791492925491298, 64.92185203933371440, 57.60335617069471681 ) ) ;
#15995=CARTESIAN_POINT ( 'NONE',  ( 22.90619343622340054, 7.840927939412480896, 8.256274177387846080 ) ) ;
#15996=CARTESIAN_POINT ( 'NONE',  ( 105.8203563788590884, 26.88901185006199412, 16.32877285998160133 ) ) ;
#15998=CARTESIAN_POINT ( 'NONE',  ( -7.825402957745081878, 7.899365992529270741, -50.41807073194384259 ) ) ;
#15999=CARTESIAN_POINT ( 'NONE',  ( 21.88606409348644277, 6.772455198693822176, 59.98579804294136864 ) ) ;
#16001=CARTESIAN_POINT ( 'NONE',  ( 12.46704290855392472, 6.417105965824390523, -76.59253135474965291 ) ) ;
#16002=VERTEX_POINT ( 'NONE', #14675 ) ;
#16005=CARTESIAN_POINT ( 'NONE',  ( 177.0024338932394130, 74.57605685449962607, 43.11700017356537984 ) ) ;
#16007=CARTESIAN_POINT ( 'NONE',  ( -107.0809603157386931, 36.42942792191067980, -36.73190862903344112 ) ) ;
#16008=CARTESIAN_POINT ( 'NONE',  ( 62.05396267233468421, 13.48332220860125830, -77.51919629011504753 ) ) ;
#16009=ORIENTED_EDGE ( 'NONE', *, *, #1745, .T. ) ;
#16013=CARTESIAN_POINT ( 'NONE',  ( -26.87327614295024603, 8.886070347947285342, -10.00229891119611025 ) ) ;
#16015=CARTESIAN_POINT ( 'NONE',  ( 197.1979149960397990, 98.19687999752002838, 9.527816039588145713 ) ) ;
#16019=CARTESIAN_POINT ( 'NONE',  ( 116.6734749296699221, 31.97209464358269315, 67.84770262631175797 ) ) ;
#16022=CARTESIAN_POINT ( 'NONE',  ( 128.9253503890652439, 38.52561778336671949, 31.35415491786180908 ) ) ;
#16023=CARTESIAN_POINT ( 'NONE',  ( 141.3036441389950255, 47.31002705502925920, 62.81493121066256435 ) ) ;
#16026=CARTESIAN_POINT ( 'NONE',  ( 82.47965707583895778, 18.04644375528062739, -90.75020385575585635 ) ) ;
#16030=ORIENTED_EDGE ( 'NONE', *, *, #53600, .T. ) ;
#16033=CARTESIAN_POINT ( 'NONE',  ( -118.6288898061518466, 41.89286798341289142, -17.45136109783878808 ) ) ;
#16036=ADVANCED_FACE ( 'NONE', ( #16055 ), #42779, .F. ) ;
#16038=EDGE_CURVE ( 'NONE', #65685, #27181, #66144, .T. ) ;
#16039=CARTESIAN_POINT ( 'NONE',  ( -166.2065256787326462, 81.19093426984588291, -66.13749893354456333 ) ) ;
#16040=CARTESIAN_POINT ( 'NONE',  ( -143.3925773749112693, 59.16144459815141943, -37.96278985645250259 ) ) ;
#16041=ORIENTED_EDGE ( 'NONE', *, *, #37908, .T. ) ;
#16042=CARTESIAN_POINT ( 'NONE',  ( 55.91133443650745960, 12.16263767238152660, 8.014282917357382630 ) ) ;
#16045=CARTESIAN_POINT ( 'NONE',  ( -125.8938041572051105, 46.49392987655495091, 45.61994787315711619 ) ) ;
#16047=CARTESIAN_POINT ( 'NONE',  ( 84.73231936899559003, 18.78199960571078364, -23.74888722610129577 ) ) ;
#16048=CARTESIAN_POINT ( 'NONE',  ( 133.8566784816069344, 42.60093787723652525, 29.51034083899533300 ) ) ;
#16049=B_SPLINE_CURVE_WITH_KNOTS ( 'NONE', 3,
 ( #63655, #58356, #63985, #26363, #69262, #15799, #30955, #37243, #10172, #52402, #9151, #58693, #41849, #3872, #9842, #31632, #68908, #25688, #47116, #20734, #31981, #36228, #3519, #62621, #14431, #63309, #42189, #30606, #53067, #46777, #68247, #41505, #62957, #5914, #26703, #1356, #44254, #32669, #27034, #53410, #59727, #64327, #16487, #48463, #16139, #21414, #22110, #43552, #38641, #65028, #11200 ),
 .UNSPECIFIED., .F., .F.,
 ( 4, 2, 2, 2, 2, 2, 2, 2, 2, 2, 2, 2, 2, 2, 2, 2, 1, 2, 2, 2, 2, 2, 2, 2, 2, 4 ),
 ( 0.000000000000000000, 0.001945536185327564373, 0.002918304277991350896, 0.003891072370655136985, 0.005836608555982708731, 0.006809376648646493953, 0.007782144741310279175, 0.009727680926637829670, 0.01167321711196537756, 0.01264598520462914023, 0.01361875329729290290, 0.01459152138995666557, 0.01556428948262042825, 0.01750982566794795359, 0.01945536185327547893, 0.02042812994593924333, 0.02140089803860300774, 0.02237366613126677561, 0.02334643422393054002, 0.02529197040925803067, 0.02626473850192179507, 0.02723750659458555254, 0.02821027468724931347, 0.02918304277991307441, 0.03015581087257683882, 0.03112857896524059975 ),
 .UNSPECIFIED. ) ;
#16052=CARTESIAN_POINT ( 'NONE',  ( -97.47339919287387033, 30.40512551257288010, -63.58105464508946625 ) ) ;
#16053=ORIENTED_EDGE ( 'NONE', *, *, #22290, .F. ) ;
#16055=FACE_OUTER_BOUND ( 'NONE', #43661, .T. ) ;
#16057=CARTESIAN_POINT ( 'NONE',  ( -165.7699288023689803, 79.30174988963855753, -43.72753680632582274 ) ) ;
#16059=CARTESIAN_POINT ( 'NONE',  ( 102.7414208686707582, 26.65627265923298594, -69.77758797498718479 ) ) ;
#16060=CARTESIAN_POINT ( 'NONE',  ( -73.81801970646053235, 21.60231032711190480, 43.64555415764338164 ) ) ;
#16061=CARTESIAN_POINT ( 'NONE',  ( -78.66644367742111399, 23.39876645725286153, -61.96000122218157458 ) ) ;
#16063=CARTESIAN_POINT ( 'NONE',  ( 41.33434189587760699, 9.684413566891871383, -35.86888733174379951 ) ) ;
#16068=CARTESIAN_POINT ( 'NONE',  ( -36.37371824399144060, 10.45334302951138028, 5.202302465703740886 ) ) ;
#16070=CARTESIAN_POINT ( 'NONE',  ( 94.11595392909970315, 23.18887043179184460, 64.57093135896856495 ) ) ;
#16071=CARTESIAN_POINT ( 'NONE',  ( 150.0889146124742695, 52.13243511955543141, -18.13589629245545964 ) ) ;
#16072=CARTESIAN_POINT ( 'NONE',  ( 86.62931800182293784, -170.0000000000000000, 71.55663816294304524 ) ) ;
#16073=CARTESIAN_POINT ( 'NONE',  ( 32.90953848114695290, 7.653665824624196645, -73.72727812858101970 ) ) ;
#16074=DIRECTION ( 'NONE',  ( -0.000000000000000000, 1.000000000000000000, -0.000000000000000000 ) ) ;
#16076=CARTESIAN_POINT ( 'NONE',  ( 114.3151031867488712, 31.93066835014830929, -90.80084266641746638 ) ) ;
#16077=ORIENTED_EDGE ( 'NONE', *, *, #50211, .F. ) ;
#16079=CARTESIAN_POINT ( 'NONE',  ( 39.40195752203892710, -170.0000000000000000, 18.06928371549960133 ) ) ;
#16082=CARTESIAN_POINT ( 'NONE',  ( -30.46060138092288128, 9.432375387772218289, 18.32403480767325377 ) ) ;
#16084=DIRECTION ( 'NONE',  ( -0.000000000000000000, 1.000000000000000000, -0.000000000000000000 ) ) ;
#16086=CARTESIAN_POINT ( 'NONE',  ( -99.31850058233798961, 31.30166762705809091, -8.775526202821598787 ) ) ;
#16087=CARTESIAN_POINT ( 'NONE',  ( 81.09429416756655939, 18.66109123847838447, 85.82913394444857147 ) ) ;
#16091=CIRCLE ( 'NONE', #34092, 242.4895526022646379 ) ;
#16093=CARTESIAN_POINT ( 'NONE',  ( -132.9409505933031710, 51.31241517713429801, 8.655732063095380013 ) ) ;
#16094=CARTESIAN_POINT ( 'NONE',  ( -109.5157885508427142, 37.76058765671432838, 66.90473407092159164 ) ) ;
#16097=CARTESIAN_POINT ( 'NONE',  ( -180.5185845152422814, 95.75861486247472953, 93.30168827895523975 ) ) ;
#16100=CARTESIAN_POINT ( 'NONE',  ( 88.53517449242355042, 20.08005703101044759, 71.31441284595423724 ) ) ;
#16101=CARTESIAN_POINT ( 'NONE',  ( 197.8598785550297521, 99.02620879292949496, -20.07738393529249166 ) ) ;
#16102=EDGE_CURVE ( 'NONE', #33041, #68729, #40082, .T. ) ;
#16103=CARTESIAN_POINT ( 'NONE',  ( 87.42971020158420004, 19.69418112884302374, -89.51066537983909654 ) ) ;
#16105=CARTESIAN_POINT ( 'NONE',  ( 138.1919700334460686, 44.10401742531042402, 30.87242645337029145 ) ) ;
#16108=CARTESIAN_POINT ( 'NONE',  ( 79.12879321038295188, 18.04902206524924679, 10.60344279547883062 ) ) ;
#16113=DIRECTION ( 'NONE',  ( 0.000000000000000000, 0.000000000000000000, 1.000000000000000000 ) ) ;
#16115=CARTESIAN_POINT ( 'NONE',  ( -75.01314391403414561, 20.96328762434827198, -22.33899052893390191 ) ) ;
#16123=CARTESIAN_POINT ( 'NONE',  ( -180.0179082103088035, 95.14811732286295864, 41.28284462864509408 ) ) ;
#16126=ORIENTED_EDGE ( 'NONE', *, *, #4360, .F. ) ;
#16127=B_SPLINE_CURVE_WITH_KNOTS ( 'NONE', 3,
 ( #51523, #8956, #24790, #46228, #57486, #20191, #30404, #2992, #9293, #3668, #50820, #36374, #25142, #30756, #46574, #52204, #4020, #41649, #25488, #24101, #63105, #2638, #46928, #14906, #7917, #40269, #45540, #24451, #67022, #56438, #45892, #8262, #29715, #24017, #45461, #18736, #7839, #61644, #60948, #65540, #12768, #56027, #66255 ),
 .UNSPECIFIED., .F., .F.,
 ( 4, 2, 2, 2, 2, 2, 2, 2, 2, 2, 2, 2, 1, 2, 2, 2, 2, 2, 2, 2, 2, 4 ),
 ( 0.02379577142314829794, 0.02527778373276531876, 0.02601878988757382050, 0.02675979604238232223, 0.02824180835199933612, 0.02972382066161635000, 0.03046482681642484480, 0.03120583297123334654, 0.03268784528085035002, 0.03416985759046735349, 0.03565186990008435697, 0.03639287605489284483, 0.03713388220970133963, 0.03787488836450983443, 0.03861589451931832229, 0.04009790682893532576, 0.04157991913855232230, 0.04306193144816931884, 0.04380293760297782057, 0.04454394375778632231, 0.04602595606740331191, 0.04750796837702030845 ),
 .UNSPECIFIED. ) ;
#16130=CARTESIAN_POINT ( 'NONE',  ( 138.5721691894143248, 44.34516164557649631, 58.00226450593800109 ) ) ;
#16131=CARTESIAN_POINT ( 'NONE',  ( -179.2128128997735246, 95.75254520622989673, 33.91814095447512756 ) ) ;
#16132=CARTESIAN_POINT ( 'NONE',  ( 126.4757069339777473, 38.29528077539268338, 62.49800859209678094 ) ) ;
#16137=VECTOR ( 'NONE', #23962, 1000.000000000000000 ) ;
#16139=CARTESIAN_POINT ( 'NONE',  ( -47.61659327988082424, 12.81296103674151965, 92.53618404811727771 ) ) ;
#16142=CARTESIAN_POINT ( 'NONE',  ( 70.43248927385285185, 14.51614591398291410, 89.83896190036961116 ) ) ;
#16147=CARTESIAN_POINT ( 'NONE',  ( -96.32309170788076358, 30.97039782218995541, -91.64132999366567844 ) ) ;
#16149=CARTESIAN_POINT ( 'NONE',  ( -71.23176719684946079, 20.69188312694500809, 65.78254442754143838 ) ) ;
#16151=CARTESIAN_POINT ( 'NONE',  ( 188.5645326065590837, 86.51153908883289034, 36.18923501154701938 ) ) ;
#16155=CARTESIAN_POINT ( 'NONE',  ( 21.44191228441540531, 7.755009954762291713, 32.56178140903555374 ) ) ;
#16157=CARTESIAN_POINT ( 'NONE',  ( 164.1338586910085837, 64.33646242148857652, -67.01638482620461446 ) ) ;
#16164=CARTESIAN_POINT ( 'NONE',  ( -24.18158274621863768, 9.527343002918318149, -71.61677556244950438 ) ) ;
#16165=CARTESIAN_POINT ( 'NONE',  ( 62.52742438962777527, 12.55954017561948532, -35.72069083216972984 ) ) ;
#16168=CARTESIAN_POINT ( 'NONE',  ( -143.2471548081022945, 59.04577938365767409, 7.214454213839029073 ) ) ;
#16172=CARTESIAN_POINT ( 'NONE',  ( -133.0921934900199801, 52.65587531157186874, 40.24238173231051263 ) ) ;
#16173=ORIENTED_EDGE ( 'NONE', *, *, #7557, .T. ) ;
#16175=CARTESIAN_POINT ( 'NONE',  ( -190.6985136298601731, 109.1272424661242582, 94.99999999999866418 ) ) ;
#16177=CARTESIAN_POINT ( 'NONE',  ( 56.66438910147189034, 11.28870326331392704, 60.16100584247962502 ) ) ;
#16178=CARTESIAN_POINT ( 'NONE',  ( -5.888165822225389867, 7.780336669456523246, 71.70979528173234030 ) ) ;
#16185=VERTEX_POINT ( 'NONE', #29742 ) ;
#16186=ORIENTED_EDGE ( 'NONE', *, *, #57575, .F. ) ;
#16190=CARTESIAN_POINT ( 'NONE',  ( -171.0758681675584114, 84.87997360100516175, -8.139245166615548754 ) ) ;
#16193=CARTESIAN_POINT ( 'NONE',  ( 69.49862690228272299, 14.27023134440513275, 33.50967676719564281 ) ) ;
#16194=CARTESIAN_POINT ( 'NONE',  ( 20.87644034061239751, 7.724420236077849999, 85.68391863677295817 ) ) ;
#16196=CARTESIAN_POINT ( 'NONE',  ( 86.62931800182293784, 19.42108912189598158, 2.867536982015618019 ) ) ;
#16198=LINE ( 'NONE', #59103, #26127 ) ;
#16200=EDGE_CURVE ( 'NONE', #2906, #54626, #51885, .T. ) ;
#16202=CARTESIAN_POINT ( 'NONE',  ( -119.1605144823340083, 43.39823405392969846, 7.961637200802151426 ) ) ;
#16205=EDGE_CURVE ( 'NONE', #52493, #46420, #2341, .T. ) ;
#16206=CARTESIAN_POINT ( 'NONE',  ( 17.74393407086869701, 6.570779001277777809, 17.92757028238993655 ) ) ;
#16209=CARTESIAN_POINT ( 'NONE',  ( 150.0973882686024865, 52.13852366454150911, 38.31082999385310472 ) ) ;
#16215=CARTESIAN_POINT ( 'NONE',  ( -25.48237668717799664, 8.689083390666784368, 42.29997830577138984 ) ) ;
#16216=CARTESIAN_POINT ( 'NONE',  ( -144.3939084932120807, 61.25241660819414591, -63.66557192140397348 ) ) ;
#16218=FACE_BOUND ( 'NONE', #14885, .T. ) ;
#16220=CARTESIAN_POINT ( 'NONE',  ( -177.5100621450479252, 93.70693725195827994, 59.06660155457885253 ) ) ;
#16222=CARTESIAN_POINT ( 'NONE',  ( -122.1940143064357187, 45.29738883755587153, -35.88556451797717983 ) ) ;
#16223=CARTESIAN_POINT ( 'NONE',  ( -86.06525741550315445, 26.37048289224654951, 12.32731785139721303 ) ) ;
#16226=CARTESIAN_POINT ( 'NONE',  ( -153.6931187576189473, 67.81270084382359187, 5.148524762051829740 ) ) ;
#16230=CARTESIAN_POINT ( 'NONE',  ( 164.0158927577712973, 62.92463143894072886, 6.365232034859697130 ) ) ;
#16231=CARTESIAN_POINT ( 'NONE',  ( 88.98820631332499431, 21.30618275724810218, -23.61262677780854702 ) ) ;
#16233=CARTESIAN_POINT ( 'NONE',  ( -38.45778834351241926, 11.87434869453507247, 13.52690563419841752 ) ) ;
#16235=VERTEX_POINT ( 'NONE', #37090 ) ;
#16238=CARTESIAN_POINT ( 'NONE',  ( 19.75315861330098599, 7.667327050329335592, -76.23447365553329291 ) ) ;
#16239=CARTESIAN_POINT ( 'NONE',  ( 117.7235023277067967, 33.62688311768400951, 91.44526349519324526 ) ) ;
#16242=CARTESIAN_POINT ( 'NONE',  ( -24.95029760921700301, 9.631514785009935409, -46.58639476887002928 ) ) ;
#16243=CARTESIAN_POINT ( 'NONE',  ( -48.34250119710924309, 14.01879126850790058, -72.92010011160856209 ) ) ;
#16245=CARTESIAN_POINT ( 'NONE',  ( -74.81618585058957649, 21.96255056808530881, -89.86471030265687432 ) ) ;
#16247=ORIENTED_EDGE ( 'NONE', *, *, #52014, .F. ) ;
#16248=ORIENTED_EDGE ( 'NONE', *, *, #50361, .T. ) ;
#16249=CARTESIAN_POINT ( 'NONE',  ( 32.90051628396145134, 8.664124555952430029, 60.48702334666123193 ) ) ;
#16251=CARTESIAN_POINT ( 'NONE',  ( 175.0857681883884140, 74.13486472930382831, 94.99999999999866418 ) ) ;
#16255=EDGE_LOOP ( 'NONE', ( #51130, #61123 ) ) ;
#16257=CARTESIAN_POINT ( 'NONE',  ( 187.8965227056807521, 87.27289477191496303, -13.73167551492022476 ) ) ;
#16258=CARTESIAN_POINT ( 'NONE',  ( 211.8345664497467169, 118.5225165986914817, 7.535369598655396572 ) ) ;
#16259=B_SPLINE_CURVE_WITH_KNOTS ( 'NONE', 3,
 ( #59825, #395, #59131, #4987, #64076, #21505, #58785, #10953, #33118, #10602, #6377, #27831, #26453, #21853, #22554, #32072, #53507, #26795, #48221, #60882, #28169, #49981, #24567, #55254 ),
 .UNSPECIFIED., .F., .F.,
 ( 4, 2, 2, 2, 2, 2, 2, 2, 2, 2, 2, 4 ),
 ( 0.009947828043730422634, 0.01119309618139666812, 0.01243836431906291534, 0.01306099838789603722, 0.01368363245672916083, 0.01492890059439544448, 0.01555153466322857503, 0.01617416873206170558, 0.01741943686972798055, 0.01804207093856113886, 0.01866470500739430063, 0.01990997314506061378 ),
 .UNSPECIFIED. ) ;
#16260=CARTESIAN_POINT ( 'NONE',  ( 39.40195752203892710, 9.424259417798134919, -50.61981746542779348 ) ) ;
#16261=CARTESIAN_POINT ( 'NONE',  ( 43.96465529479667111, 9.046527005589348747, -22.24810759540392269 ) ) ;
#16262=DIRECTION ( 'NONE',  ( -0.000000000000000000, 1.000000000000000000, -0.000000000000000000 ) ) ;
#16264=EDGE_CURVE ( 'NONE', #29832, #31339, #27479, .T. ) ;
#16270=CARTESIAN_POINT ( 'NONE',  ( 88.52077179907880122, 21.14145351760140912, -36.06003046012785518 ) ) ;
#16272=CARTESIAN_POINT ( 'NONE',  ( 157.4703587214989113, 58.92748579479259519, -89.81328548006499091 ) ) ;
#16274=EDGE_CURVE ( 'NONE', #11337, #41847, #60256, .T. ) ;
#16275=CARTESIAN_POINT ( 'NONE',  ( 152.3102623290679958, 53.74757787434986511, 15.51308360347570137 ) ) ;
#16276=CARTESIAN_POINT ( 'NONE',  ( -15.16750062833000001, 8.491651705883104029, 92.86961823882721490 ) ) ;
#16278=AXIS2_PLACEMENT_3D ( 'NONE', #6128, #58900, #5447 ) ;
#16279=ORIENTED_EDGE ( 'NONE', *, *, #41580, .T. ) ;
#16281=FACE_OUTER_BOUND ( 'NONE', #3468, .T. ) ;
#16288=CARTESIAN_POINT ( 'NONE',  ( 91.67776154311745529, 22.27748043241296116, -64.61425086459156830 ) ) ;
#16290=ORIENTED_EDGE ( 'NONE', *, *, #25885, .F. ) ;
#16291=B_SPLINE_CURVE_WITH_KNOTS ( 'NONE', 3,
 ( #45129, #30346, #66273, #18401, #12786, #56378, #46165, #56734, #18754, #67639, #7856, #61658, #24386, #29304, #13812, #40210, #8550, #30002, #34935, #19091, #35629, #50756, #2577, #13477, #19433, #8199, #23349, #51460, #7520, #24034, #55687, #40544, #28971, #2922, #45829, #29649, #51112, #50416, #67305, #44793, #40895, #61995, #2237, #62354, #3271, #57081, #23685, #34604, #66609, #24731, #39857, #61314, #8893, #1896, #56040, #18064, #13140, #39515, #26100, #57769, #37000, #10598, #52815, #10256, #15200, #20818, #53150, #42617, #41929, #67989, #15884, #4636 ),
 .UNSPECIFIED., .F., .F.,
 ( 4, 2, 2, 2, 2, 2, 2, 2, 2, 2, 2, 2, 2, 2, 2, 2, 2, 2, 2, 2, 2, 2, 2, 2, 2, 2, 2, 2, 2, 2, 2, 2, 2, 2, 2, 4 ),
 ( 0.000000000000000000, 0.001364161439190743471, 0.002046242158786115099, 0.002728322878381486943, 0.004092484317572176421, 0.005456645756762866332, 0.006138726476358211288, 0.006820807195953556244, 0.007502887915548901200, 0.008184968635144247023, 0.008867049354739591979, 0.009549130074334936935, 0.01091329151352568756, 0.01227745295271643992, 0.01364161439190719055, 0.01500577583109794118, 0.01636993727028869181, 0.01909826014867019306, 0.02182658302705169431, 0.02319074446624243974, 0.02455490590543318516, 0.02728322878381467601, 0.02864739022300543531, 0.03001155166219619114, 0.03137571310138694697, 0.03273987454057770974, 0.03410403597976846557, 0.03546819741895922140, 0.03615027813855459238, 0.03683235885814997029, 0.03819652029734069837, 0.03887860101693609016, 0.03956068173653147502, 0.04092484317572224473, 0.04228900461491302137, 0.04365316605410379108 ),
 .UNSPECIFIED. ) ;
#16292=CARTESIAN_POINT ( 'NONE',  ( -62.15324028806258383, 16.70091357159900980, -67.09546592820414901 ) ) ;
#16294=CARTESIAN_POINT ( 'NONE',  ( 31.90184941268615759, 7.552181687745346039, -16.51731055372926704 ) ) ;
#16301=CARTESIAN_POINT ( 'NONE',  ( -48.34250119710923599, 14.01879126850789525, -46.07554952114484337 ) ) ;
#16303=CARTESIAN_POINT ( 'NONE',  ( 9.275903038161096958, 7.385619229189526180, 41.26687823360024510 ) ) ;
#16305=CARTESIAN_POINT ( 'NONE',  ( -86.11824579438169280, 26.39279658766581349, 92.51845406669916372 ) ) ;
#16307=ORIENTED_EDGE ( 'NONE', *, *, #11472, .T. ) ;
#16309=CARTESIAN_POINT ( 'NONE',  ( -15.07200981767290671, 7.471751903425206010, -14.12493423355625310 ) ) ;
#16310=CARTESIAN_POINT ( 'NONE',  ( 204.6977192012829789, -170.0000000000000000, 9.863170148305760776 ) ) ;
#16313=CARTESIAN_POINT ( 'NONE',  ( -59.96408504033280451, 17.10126854471816316, -37.02704747533549323 ) ) ;
#16314=CARTESIAN_POINT ( 'NONE',  ( -9.524904342798459211, 8.016391612076530393, -23.38257539395581475 ) ) ;
#16315=CARTESIAN_POINT ( 'NONE',  ( 150.2076397309211870, 52.21780102759852582, -72.36031576144425514 ) ) ;
#16316=CARTESIAN_POINT ( 'NONE',  ( 21.73827885904431056, 6.764046335627708295, -20.74696102369355799 ) ) ;
#16320=VERTEX_POINT ( 'NONE', #12444 ) ;
#16322=CARTESIAN_POINT ( 'NONE',  ( 67.54641595172913071, 14.80690682047551476, -10.37962302817197013 ) ) ;
#16326=CARTESIAN_POINT ( 'NONE',  ( -153.6946616617038899, 69.16142959008688251, 5.137162390210407992 ) ) ;
#16330=CARTESIAN_POINT ( 'NONE',  ( -156.6879335332043865, 71.88581156458076293, 89.73719858978633113 ) ) ;
#16331=ORIENTED_EDGE ( 'NONE', *, *, #23228, .T. ) ;
#16336=VECTOR ( 'NONE', #30334, 1000.000000000000000 ) ;
#16337=CARTESIAN_POINT ( 'NONE',  ( -155.1204242627069902, 70.44799358128193489, -20.44876085833080381 ) ) ;
#16338=CARTESIAN_POINT ( 'NONE',  ( 36.77024545412685086, 9.095083943590518416, -50.14715022776851328 ) ) ;
#16340=FACE_OUTER_BOUND ( 'NONE', #28740, .T. ) ;
#16342=CARTESIAN_POINT ( 'NONE',  ( 185.7267155939802876, 84.90388481853130997, 57.75814002187100016 ) ) ;
#16343=CARTESIAN_POINT ( 'NONE',  ( -153.5002794404626059, 67.64160439471098130, 58.71247530986894958 ) ) ;
#16345=CARTESIAN_POINT ( 'NONE',  ( 109.7724924842966061, 28.66436020578543520, 17.76666361527367144 ) ) ;
#16347=CARTESIAN_POINT ( 'NONE',  ( -84.55373779407982227, 24.65190748253138509, -47.28824730636777218 ) ) ;
#16351=CARTESIAN_POINT ( 'NONE',  ( 14.80205238535216061, 6.470775952815777110, -77.31449080655163186 ) ) ;
#16358=CARTESIAN_POINT ( 'NONE',  ( 43.14712943604299511, 8.926114770663650333, -63.46178131008120715 ) ) ;
#16360=CARTESIAN_POINT ( 'NONE',  ( 55.64941011647476898, 12.11006142851269729, -68.59167301408281503 ) ) ;
#16363=ORIENTED_EDGE ( 'NONE', *, *, #10309, .T. ) ;
#16370=EDGE_LOOP ( 'NONE', ( #4329, #45897 ) ) ;
#16377=CARTESIAN_POINT ( 'NONE',  ( 81.83553453535668609, 17.84068330693397897, -91.23905641206360428 ) ) ;
#16380=CYLINDRICAL_SURFACE ( 'NONE', #44298, 7.500000000000013323 ) ;
#16382=EDGE_CURVE ( 'NONE', #780, #50735, #59369, .T. ) ;
#16384=VERTEX_POINT ( 'NONE', #55699 ) ;
#16387=AXIS2_PLACEMENT_3D ( 'NONE', #57693, #35890, #24999 ) ;
#16389=CARTESIAN_POINT ( 'NONE',  ( 40.37438610703016906, 8.537526699166104294, -50.57269136638377915 ) ) ;
#16390=CARTESIAN_POINT ( 'NONE',  ( -166.9992034932274976, 82.01285191063136892, -64.69379323303392937 ) ) ;
#16391=CARTESIAN_POINT ( 'NONE',  ( -146.5268141329886475, 61.69196909035589726, -35.42679155757922871 ) ) ;
#16397=CARTESIAN_POINT ( 'NONE',  ( 135.6651581599210203, 42.52720121194706593, -23.96109018709176652 ) ) ;
#16398=CARTESIAN_POINT ( 'NONE',  ( 90.31682503704260512, 20.71196693118262644, -63.61707171944141948 ) ) ;
#16399=CARTESIAN_POINT ( 'NONE',  ( 62.20100515256353901, 12.48495193239473089, -89.44322602549407009 ) ) ;
#16400=CARTESIAN_POINT ( 'NONE',  ( -98.46684543088105102, 30.88557736720389002, 17.63727003067570465 ) ) ;
#16401=CARTESIAN_POINT ( 'NONE',  ( -94.77925136849374610, 29.13093715379787341, -69.12727919511270613 ) ) ;
#16403=ORIENTED_EDGE ( 'NONE', *, *, #17879, .F. ) ;
#16404=CARTESIAN_POINT ( 'NONE',  ( 186.2651679807462415, 84.00458780104315792, -76.01284985794765703 ) ) ;
#16407=CYLINDRICAL_SURFACE ( 'NONE', #45263, 7.500000000000027534 ) ;
#16409=CARTESIAN_POINT ( 'NONE',  ( 107.2614272668149198, 28.62909081796203381, -63.38104519901254008 ) ) ;
#16410=CARTESIAN_POINT ( 'NONE',  ( -73.81801970646056077, 21.60231032711190835, -63.73264820421131560 ) ) ;
#16412=CARTESIAN_POINT ( 'NONE',  ( 46.51679720856118649, 10.46086439153924452, -45.54304003388800481 ) ) ;
#16413=CARTESIAN_POINT ( 'NONE',  ( 210.0292194063021611, 113.9511645670926612, 68.83246835844813916 ) ) ;
#16416=CARTESIAN_POINT ( 'NONE',  ( -108.1144194775597640, 35.84457139767599898, -20.40923384673128282 ) ) ;
#16419=CARTESIAN_POINT ( 'NONE',  ( -12.39413342787891281, 7.231444436041491564, -36.95011374576873209 ) ) ;
#16421=CARTESIAN_POINT ( 'NONE',  ( -86.16905982510307638, 25.32271692190228407, 91.86796594561636198 ) ) ;
#16422=CARTESIAN_POINT ( 'NONE',  ( 87.10672734544989737, 20.64813880796637235, 56.55663816294299551 ) ) ;
#16423=CARTESIAN_POINT ( 'NONE',  ( 152.2940756559018780, 53.73566983921583784, -22.21240161800733759 ) ) ;
#16425=B_SPLINE_CURVE_WITH_KNOTS ( 'NONE', 3,
 ( #43710, #33543, #48983, #10668, #38811, #37753, #38097, #48285, #6449, #11019, #33186, #27900 ),
 .UNSPECIFIED., .F., .F.,
 ( 4, 2, 2, 2, 2, 4 ),
 ( 0.000000000000000000, 0.002494459074786444484, 0.004988918149572888969, 0.007483377224359334320, 0.008730606761752562200, 0.009977836299145791815 ),
 .UNSPECIFIED. ) ;
#16426=CARTESIAN_POINT ( 'NONE',  ( -96.45303203827904781, 31.03218867996497821, -64.61131369028386473 ) ) ;
#16437=CARTESIAN_POINT ( 'NONE',  ( -10.69547592951791160, 8.103864096836385755, 3.829060544445804570 ) ) ;
#16438=CARTESIAN_POINT ( 'NONE',  ( 46.89016064832838993, 10.52130577388959409, -70.45255809555227700 ) ) ;
#16441=CARTESIAN_POINT ( 'NONE',  ( -4.081377963939786468, 6.676029627840591729, 31.11232541612353941 ) ) ;
#16443=CARTESIAN_POINT ( 'NONE',  ( 94.07925938825250967, 23.17492699065150319, 91.83144490676588134 ) ) ;
#16446=ORIENTED_EDGE ( 'NONE', *, *, #22642, .F. ) ;
#16449=CARTESIAN_POINT ( 'NONE',  ( -133.2698123908828904, 51.54642138335025692, 12.65949325828542804 ) ) ;
#16450=CARTESIAN_POINT ( 'NONE',  ( -167.1619226259399227, 82.18315278115417755, -46.77288687742393591 ) ) ;
#16451=CARTESIAN_POINT ( 'NONE',  ( -133.1566699306513613, 52.70203339370770834, -44.30393921777678656 ) ) ;
#16453=CARTESIAN_POINT ( 'NONE',  ( 157.4703587214989398, -170.0000000000000000, 71.25401806271709404 ) ) ;
#16455=CARTESIAN_POINT ( 'NONE',  ( 197.3756653044963230, 98.41886189307119537, -18.61350521218830423 ) ) ;
#16457=CARTESIAN_POINT ( 'NONE',  ( 138.6020257460769756, 44.36414356192209851, 42.83845183682598901 ) ) ;
#16458=ORIENTED_EDGE ( 'NONE', *, *, #20675, .T. ) ;
#16460=DIRECTION ( 'NONE',  ( 0.000000000000000000, 0.000000000000000000, 1.000000000000000000 ) ) ;
#16461=CARTESIAN_POINT ( 'NONE',  ( 164.8444104055694481, 64.93678790243656351, 8.668489052207666745 ) ) ;
#16464=EDGE_CURVE ( 'NONE', #30354, #34477, #34996, .T. ) ;
#16468=CARTESIAN_POINT ( 'NONE',  ( -76.31381168750407085, 21.43908608416556660, -8.633424497019335675 ) ) ;
#16469=CARTESIAN_POINT ( 'NONE',  ( -56.72814287166056602, 15.13700122306437379, 45.13175927368157403 ) ) ;
#16471=CARTESIAN_POINT ( 'NONE',  ( 151.3136733342017521, 54.26417151662143112, 14.35556273797184446 ) ) ;
#16473=CARTESIAN_POINT ( 'NONE',  ( 164.7167608259061069, 63.51199216609071385, 34.95606193614021606 ) ) ;
#16474=DIRECTION ( 'NONE',  ( 0.000000000000000000, 0.000000000000000000, 1.000000000000000000 ) ) ;
#16475=CARTESIAN_POINT ( 'NONE',  ( 157.4703587214989398, -170.0000000000000000, 63.75401806271707983 ) ) ;
#16477=CARTESIAN_POINT ( 'NONE',  ( 63.01563776193091826, 12.67277567978500130, -35.72069083216973695 ) ) ;
#16478=LINE ( 'NONE', #37931, #67089 ) ;
#16479=CARTESIAN_POINT ( 'NONE',  ( -31.93184248720560348, 9.672312402099827011, -8.472646774738155528 ) ) ;
#16480=CARTESIAN_POINT ( 'NONE',  ( -180.5801285865471471, 97.42945596116099694, 37.52258506186108633 ) ) ;
#16481=CARTESIAN_POINT ( 'NONE',  ( -37.38262509017737045, 10.64263598035110014, -65.06093979278308836 ) ) ;
#16483=ORIENTED_EDGE ( 'NONE', *, *, #62346, .T. ) ;
#16484=VERTEX_POINT ( 'NONE', #57434 ) ;
#16485=PLANE ( 'NONE',  #22767 ) ;
#16487=CARTESIAN_POINT ( 'NONE',  ( -47.54588915626003853, 12.79638599324405490, 91.55540593693795870 ) ) ;
#16490=CARTESIAN_POINT ( 'NONE',  ( -108.3113955865101161, 35.95170844434134239, 87.23892145708312285 ) ) ;
#16494=DIRECTION ( 'NONE',  ( -0.8118923937861950435, -0.5838071093367415143, 0.000000000000000000 ) ) ;
#16500=CARTESIAN_POINT ( 'NONE',  ( 181.0840389613909736, 78.60582251573003987, 29.30859410551139277 ) ) ;
#16502=CARTESIAN_POINT ( 'NONE',  ( -73.09185868250600038, 20.27574131633382137, 16.11495310017765803 ) ) ;
#16505=CARTESIAN_POINT ( 'NONE',  ( 23.04797191264876233, 7.849755664016362822, 35.56853372841017347 ) ) ;
#16508=CARTESIAN_POINT ( 'NONE',  ( 161.7031777507227162, 62.31724004902784486, -64.26033578956516124 ) ) ;
#16511=CARTESIAN_POINT ( 'NONE',  ( 110.2429982417149574, -170.0000000000000000, -43.42243756565370205 ) ) ;
#16513=ORIENTED_EDGE ( 'NONE', *, *, #8704, .F. ) ;
#16514=CARTESIAN_POINT ( 'NONE',  ( -82.93267503967652488, 23.99263498936122474, 44.09127840080141425 ) ) ;
#16515=CARTESIAN_POINT ( 'NONE',  ( 157.4703587214989113, 58.92748579479258808, -77.96873488960135035 ) ) ;
#16516=CARTESIAN_POINT ( 'NONE',  ( 46.65974587859240330, 10.48396258569371042, 35.45994816272273908 ) ) ;
#16518=CARTESIAN_POINT ( 'NONE',  ( -29.51060362117876679, 9.282716514427260535, 57.30906105449729182 ) ) ;
#16519=DIRECTION ( 'NONE',  ( 1.000000000000000000, 0.000000000000000000, -0.000000000000000000 ) ) ;
#16522=EDGE_CURVE ( 'NONE', #7422, #33643, #52826, .T. ) ;
#16526=CARTESIAN_POINT ( 'NONE',  ( -129.6079169496900931, 50.20899308323959787, 44.63993178974271814 ) ) ;
#16529=CARTESIAN_POINT ( 'NONE',  ( 182.4828945259410773, 81.47614346340601799, -90.03736357220414277 ) ) ;
#16530=CARTESIAN_POINT ( 'NONE',  ( 55.52750043885183828, 11.05966813607792787, 63.66763205657868951 ) ) ;
#16531=CARTESIAN_POINT ( 'NONE',  ( -4.071369321747696723, 7.682719369516285646, 70.97146076770519585 ) ) ;
#16534=CARTESIAN_POINT ( 'NONE',  ( 133.8566784816069060, 42.60093787723655367, 71.35489142945907304 ) ) ;
#16543=CARTESIAN_POINT ( 'NONE',  ( 63.01563776193090405, 12.67277567978497643, 44.81296093922130552 ) ) ;
#16545=CARTESIAN_POINT ( 'NONE',  ( 79.92465405224851338, 17.24122384219593940, 13.76543913484589510 ) ) ;
#16546=CYLINDRICAL_SURFACE ( 'NONE', #13702, 7.500000000000020428 ) ;
#16547=CARTESIAN_POINT ( 'NONE',  ( -75.00168449119587422, 20.95943092127970431, 44.46631830285968334 ) ) ;
#16551=CARTESIAN_POINT ( 'NONE',  ( 94.12988949694084795, 22.11811104795076588, 10.60322717497807687 ) ) ;
#16552=CARTESIAN_POINT ( 'NONE',  ( 8.000000000000007105, 249.8719672152120381, 94.99999999999866418 ) ) ;
#16558=CARTESIAN_POINT ( 'NONE',  ( 154.4429418375333114, 55.33424769452794578, 30.03275206029211830 ) ) ;
#16559=CARTESIAN_POINT ( 'NONE',  ( 63.01563776193090405, 13.70579113808097738, 44.81296093922130552 ) ) ;
#16566=FACE_BOUND ( 'NONE', #12318, .T. ) ;
#16567=DIRECTION ( 'NONE',  ( -0.000000000000000000, 1.000000000000000000, -0.000000000000000000 ) ) ;
#16575=EDGE_CURVE ( 'NONE', #26339, #21211, #29985, .T. ) ;
#16577=CARTESIAN_POINT ( 'NONE',  ( -86.15466590221103615, 26.40813842494317498, 65.25490091457173492 ) ) ;
#16578=B_SPLINE_CURVE_WITH_KNOTS ( 'NONE', 3,
 ( #14835, #10585, #68644, #32058, #31373, #20456, #59117, #53493, #63381, #16216, #5324, #10936, #15191, #36651, #21487, #58098, #26781, #48207, #47520, #9918, #32, #52802, #64404, #20808, #37670, #32408, #64758, #1436, #49962, #48900, #43633, #23254, #60170, #382, #22891, #48546, #60865, #6710, #5652, #54887, #28155, #11990, #22540, #65107, #49603, #43980 ),
 .UNSPECIFIED., .F., .F.,
 ( 4, 2, 2, 2, 2, 2, 2, 2, 2, 2, 2, 2, 2, 2, 2, 2, 2, 2, 2, 2, 2, 2, 4 ),
 ( 3.986091072867590107E-17, 0.003373244802897413987, 0.004216556003621757184, 0.005059867204346100815, 0.006746489605794788076, 0.007589800806519115227, 0.008433112007243441510, 0.009276423207967768661, 0.01011973440869209581, 0.01180635681014072062, 0.01349297921158934370, 0.01433629041231365524, 0.01517960161303797025, 0.01686622401448657424, 0.01770953521521087884, 0.01855284641593518344, 0.02023946881738376835, 0.02108278001810802785, 0.02192609121883228734, 0.02361271362028080287, 0.02445602482100502767, 0.02529933602172925594, 0.02698595842317763963 ),
 .UNSPECIFIED. ) ;
#16579=CARTESIAN_POINT ( 'NONE',  ( 91.67776154311752634, 22.27748043241297538, -10.92514968366423034 ) ) ;
#16582=CARTESIAN_POINT ( 'NONE',  ( -33.85171821065139852, 11.02091558840053764, 17.98985968378708122 ) ) ;
#16584=DIRECTION ( 'NONE',  ( -0.000000000000000000, 1.000000000000000000, -0.000000000000000000 ) ) ;
#16585=CARTESIAN_POINT ( 'NONE',  ( 82.95856197793166587, 19.25847567427441120, -76.72461906074219939 ) ) ;
#16586=CARTESIAN_POINT ( 'NONE',  ( 115.7592475865162527, 32.64122214332899574, 85.70808474779904884 ) ) ;
#16587=CARTESIAN_POINT ( 'NONE',  ( -142.1332311300253082, 59.44822332309658464, 63.66972751217561921 ) ) ;
#16588=EDGE_CURVE ( 'NONE', #805, #37653, #36720, .T. ) ;
#16590=CARTESIAN_POINT ( 'NONE',  ( -28.13527276074847805, 10.08983026464524713, -49.55478388655180311 ) ) ;
#16591=CARTESIAN_POINT ( 'NONE',  ( -54.08816720029309977, 15.46531105893042124, -62.10765360863577200 ) ) ;
#16592=CARTESIAN_POINT ( 'NONE',  ( -78.66644367742109978, 23.39876645725289706, -88.80455181264524356 ) ) ;
#16596=CARTESIAN_POINT ( 'NONE',  ( 38.91512155099544401, 9.360679678889624711, 56.75838489642694640 ) ) ;
#16597=CARTESIAN_POINT ( 'NONE',  ( 132.3682272970516465, 41.70269401232697959, -89.82203283494803259 ) ) ;
#16599=CARTESIAN_POINT ( 'NONE',  ( 69.67874066886028572, 15.35768729680762412, -93.44190485051720430 ) ) ;
#16601=CARTESIAN_POINT ( 'NONE',  ( 89.20981392318257974, 21.38519354635263525, 17.41376394564116126 ) ) ;
#16602=CARTESIAN_POINT ( 'NONE',  ( -7.825402957745087207, 6.891034867348159842, 71.96013162991091860 ) ) ;
#16603=CARTESIAN_POINT ( 'NONE',  ( 212.0779786303465357, 118.9010947973413010, 8.485549497644882422 ) ) ;
#16607=CARTESIAN_POINT ( 'NONE',  ( 210.1633650091870607, 114.1507944623967319, -22.12313984221156105 ) ) ;
#16609=CARTESIAN_POINT ( 'NONE',  ( 160.9097745014958036, 61.67033591969548922, 70.42277619118128484 ) ) ;
#16613=LINE ( 'NONE', #5377, #6582 ) ;
#16614=CARTESIAN_POINT ( 'NONE',  ( 90.91356992076215704, 21.99794663086831292, -37.16094633631047373 ) ) ;
#16615=CARTESIAN_POINT ( 'NONE',  ( -48.23389383802712871, 13.99288361739332132, 61.52903241797603329 ) ) ;
#16617=CARTESIAN_POINT ( 'NONE',  ( 157.4703587214989113, 57.65129005721576050, 17.56491688178971700 ) ) ;
#16618=CARTESIAN_POINT ( 'NONE',  ( -15.32007997986256953, 8.506358610388080166, 90.59327875642129868 ) ) ;
#16622=CARTESIAN_POINT ( 'NONE',  ( -62.30463872474476972, 16.74658165105247676, 62.68421133332508077 ) ) ;
#16623=EDGE_LOOP ( 'NONE', ( #32176, #25986, #16186, #30724, #41952 ) ) ;
#16624=AXIS2_PLACEMENT_3D ( 'NONE', #3618, #30704, #62718 ) ;
#16625=ORIENTED_EDGE ( 'NONE', *, *, #12907, .T. ) ;
#16628=CARTESIAN_POINT ( 'NONE',  ( 103.4696172145934838, 25.87254488218942328, 40.34164898042279646 ) ) ;
#16630=CARTESIAN_POINT ( 'NONE',  ( -57.43251939610647838, 15.33203492375494470, -76.68981896774998575 ) ) ;
#16631=CARTESIAN_POINT ( 'NONE',  ( 32.90953848114694580, 7.653665824624193093, -20.03817694765365331 ) ) ;
#16632=CARTESIAN_POINT ( 'NONE',  ( 173.5844030397476274, 72.71952271766127751, -44.03001291059575806 ) ) ;
#16633=CARTESIAN_POINT ( 'NONE',  ( -149.5074843970971017, 64.17983161892347255, 18.87627064943540134 ) ) ;
#16635=CARTESIAN_POINT ( 'NONE',  ( 88.99522780200238969, 20.24180937454203644, 44.33318672426325691 ) ) ;
#16638=CARTESIAN_POINT ( 'NONE',  ( 110.2429982417149574, 29.99119854320843714, -9.077886975189997543 ) ) ;
#16646=VERTEX_POINT ( 'NONE', #45763 ) ;
#16648=ORIENTED_EDGE ( 'NONE', *, *, #47937, .T. ) ;
#16649=CARTESIAN_POINT ( 'NONE',  ( -11.14880195267006435, 7.129907723790824825, -9.332131539978064438 ) ) ;
#16650=CARTESIAN_POINT ( 'NONE',  ( -169.8036256908229973, 84.98540282375472543, 85.26356001004853624 ) ) ;
#16651=CARTESIAN_POINT ( 'NONE',  ( -52.68007207639880107, 14.05813534436550150, -22.99069914386438995 ) ) ;
#16654=CARTESIAN_POINT ( 'NONE',  ( -62.55184817504200367, 17.87278652436698323, -43.23193394049161498 ) ) ;
#16656=CARTESIAN_POINT ( 'NONE',  ( -12.40598104375062860, 8.242193636955580160, -10.11445045639250040 ) ) ;
#16658=CARTESIAN_POINT ( 'NONE',  ( 152.1327777395850660, 53.61712543276776444, -65.19409239134269285 ) ) ;
#16659=CARTESIAN_POINT ( 'NONE',  ( 21.25987915030396280, 6.737472588634915382, -21.30969410552895127 ) ) ;
#16666=CARTESIAN_POINT ( 'NONE',  ( -142.5087559769084748, 59.74468185400777998, 14.12501252483976977 ) ) ;
#16667=CARTESIAN_POINT ( 'NONE',  ( -55.90809155135389830, 15.95534155093521633, -88.95128615556963325 ) ) ;
#16668=CARTESIAN_POINT ( 'NONE',  ( -24.43167697712097208, 9.560946958255405193, 88.71272639884266198 ) ) ;
#16670=CARTESIAN_POINT ( 'NONE',  ( -152.4930836497867404, 68.09400557494205941, 4.492453323582243918 ) ) ;
#16671=CARTESIAN_POINT ( 'NONE',  ( -108.5289085648060450, 36.07014995015116199, 15.32950029942471737 ) ) ;
#16673=CARTESIAN_POINT ( 'NONE',  ( -154.6185427734352515, 69.99209860720225151, 86.39051265489474929 ) ) ;
#16676=ORIENTED_EDGE ( 'NONE', *, *, #65529, .T. ) ;
#16678=CARTESIAN_POINT ( 'NONE',  ( -149.9475539515598541, 65.87716206616011050, -7.968279941028271196 ) ) ;
#16679=CARTESIAN_POINT ( 'NONE',  ( 90.44107021831128179, 21.82636779519387105, -90.53914462835739130 ) ) ;
#16681=CARTESIAN_POINT ( 'NONE',  ( -31.43908319763710679, 9.591432048623762086, 72.06100499665289760 ) ) ;
#16683=CARTESIAN_POINT ( 'NONE',  ( -154.7998111145352027, 68.80117179139328698, -20.80406720516667463 ) ) ;
#16687=CARTESIAN_POINT ( 'NONE',  ( 187.5165082312809659, 86.85340440641661530, 59.78757442739207306 ) ) ;
#16688=CARTESIAN_POINT ( 'NONE',  ( -156.3790798118593841, 70.23422112803316963, 62.04827372833165100 ) ) ;
#16694=CARTESIAN_POINT ( 'NONE',  ( 11.21653854975268949, 6.397128675385706842, -63.89780128798599890 ) ) ;
#16697=CARTESIAN_POINT ( 'NONE',  ( -131.2803255164624829, 50.14412978403780130, -64.03362474960219686 ) ) ;
#16698=CARTESIAN_POINT ( 'NONE',  ( -133.3765738414514885, 51.62252165471728915, -41.83704703482699472 ) ) ;
#16699=CARTESIAN_POINT ( 'NONE',  ( 43.35980717318837208, 8.957244490220915623, -63.58895816981770110 ) ) ;
#16702=EDGE_LOOP ( 'NONE', ( #56253, #49401, #28186, #20785 ) ) ;
#16703=CARTESIAN_POINT ( 'NONE',  ( -30.46060138092287772, 9.432375387772211184, -8.520515782790420545 ) ) ;
#16704=CARTESIAN_POINT ( 'NONE',  ( 185.5791793180738694, 83.26975658156528937, 84.46066206085653505 ) ) ;
#16707=CARTESIAN_POINT ( 'NONE',  ( 188.5653887627528036, 88.01608521313127653, 36.19925310697095711 ) ) ;
#16710=CARTESIAN_POINT ( 'NONE',  ( 112.5537757279407032, 31.07998172410697180, 71.10680706731751854 ) ) ;
#16712=CARTESIAN_POINT ( 'NONE',  ( 137.6104751318276840, 44.92718313329107360, 57.35758373017568346 ) ) ;
#16713=CYLINDRICAL_SURFACE ( 'NONE', #26342, 7.500000000000013323 ) ;
#16714=CARTESIAN_POINT ( 'NONE',  ( 162.2907419228889410, 61.49817556009425346, -91.55379821537337648 ) ) ;
#16717=CARTESIAN_POINT ( 'NONE',  ( -189.4223925288096382, 107.3427006758676470, 40.14341618987140947 ) ) ;
#16719=VERTEX_POINT ( 'NONE', #58370 ) ;
#16723=CARTESIAN_POINT ( 'NONE',  ( 43.14356474118745410, 8.925336319666900664, -49.63851462474485743 ) ) ;
#16727=CARTESIAN_POINT ( 'NONE',  ( 63.01563776193091826, 13.70579113808096849, 17.96841034875761878 ) ) ;
#16729=CARTESIAN_POINT ( 'NONE',  ( -149.5074843970971301, -170.0000000000000000, 65.06537183036276417 ) ) ;
#16730=CARTESIAN_POINT ( 'NONE',  ( -55.05276343752910151, 14.68156374112636264, -50.21632399845989170 ) ) ;
#16736=CARTESIAN_POINT ( 'NONE',  ( 79.92465405224847075, 17.24122384219593584, -13.07911145561778099 ) ) ;
#16737=CARTESIAN_POINT ( 'NONE',  ( 93.09528872995971938, 21.72934119836187250, -66.33386381959452649 ) ) ;
#16738=CARTESIAN_POINT ( 'NONE',  ( 197.6316695787931224, 97.13022718399025734, 12.39526483620049291 ) ) ;
#16739=CARTESIAN_POINT ( 'NONE',  ( -101.3492134984965105, 32.31003911421604613, 18.63133054193531635 ) ) ;
#16745=CARTESIAN_POINT ( 'NONE',  ( 46.89006465517228861, 9.501960077668739402, 37.90267269328078470 ) ) ;
#16746=CARTESIAN_POINT ( 'NONE',  ( 15.29899606819416924, 6.485153354884285903, 30.01470767270521733 ) ) ;
#16753=CARTESIAN_POINT ( 'NONE',  ( -121.1841775822198457, 44.65790002524552449, 32.26246926628499523 ) ) ;
#16754=CARTESIAN_POINT ( 'NONE',  ( 207.8675797643809631, 110.7908513421271692, 70.36262409475189372 ) ) ;
#16758=CARTESIAN_POINT ( 'NONE',  ( -35.17600017528510392, 10.23461991275926586, 4.364559136216419333 ) ) ;
#16759=CARTESIAN_POINT ( 'NONE',  ( 93.87111289824404992, 23.09598275302505854, 66.07224964266130485 ) ) ;
#16760=CARTESIAN_POINT ( 'NONE',  ( 150.0501577908836452, 52.10460126680130344, -15.65376044760501806 ) ) ;
#16761=DIRECTION ( 'NONE',  ( -0.000000000000000000, 1.000000000000000000, -0.000000000000000000 ) ) ;
#16762=CARTESIAN_POINT ( 'NONE',  ( -101.3502439362134737, 33.43728945125135965, -76.81582209555509166 ) ) ;
#16763=CARTESIAN_POINT ( 'NONE',  ( 117.1629420986868695, 33.34326655207112822, -94.18893269630353871 ) ) ;
#16764=EDGE_CURVE ( 'NONE', #58835, #56347, #61866, .T. ) ;
#16767=CARTESIAN_POINT ( 'NONE',  ( 207.0580434617101560, 109.6333291630981250, 83.25781485285460803 ) ) ;
#16772=CARTESIAN_POINT ( 'NONE',  ( -25.80058235236790765, 8.733375263008339218, 15.84155572553979141 ) ) ;
#16774=CARTESIAN_POINT ( 'NONE',  ( 43.14669449386823885, 9.942681284149134768, -63.44779378956349802 ) ) ;
#16776=CARTESIAN_POINT ( 'NONE',  ( -107.0584934212648278, 35.27493744466469394, -63.55753797633620650 ) ) ;
#16777=CARTESIAN_POINT ( 'NONE',  ( 79.37286005156086333, 18.12402286788021044, 92.82794357717375533 ) ) ;
#16780=AXIS2_PLACEMENT_3D ( 'NONE', #63648, #31294, #58017 ) ;
#16782=CARTESIAN_POINT ( 'NONE',  ( -131.2803255164625114, 50.14412978403783683, 16.50002702178883851 ) ) ;
#16783=CARTESIAN_POINT ( 'NONE',  ( -168.0052514572427071, 83.06849406765624622, -36.72215715079727261 ) ) ;
#16789=CARTESIAN_POINT ( 'NONE',  ( 200.4574930424075490, 102.3536505870638393, -10.77782775283908379 ) ) ;
#16790=CARTESIAN_POINT ( 'NONE',  ( -143.4430361498845343, 59.20144672606826219, 87.48578625622529614 ) ) ;
#16791=CARTESIAN_POINT ( 'NONE',  ( 8.000000000000007105, 249.8719672152120381, -95.00000000000133582 ) ) ;
#16792=ORIENTED_EDGE ( 'NONE', *, *, #28778, .F. ) ;
#16794=CARTESIAN_POINT ( 'NONE',  ( 79.92842440418705507, 18.29578799637232578, 6.962318630869309466 ) ) ;
#16799=CARTESIAN_POINT ( 'NONE',  ( 180.2494929075577943, 79.18888319146950039, 71.15314469597512925 ) ) ;
#16801=ORIENTED_EDGE ( 'NONE', *, *, #25667, .F. ) ;
#16802=CARTESIAN_POINT ( 'NONE',  ( -78.18913509716431065, 22.13995206110505265, -8.270900041254195756 ) ) ;
#16806=CARTESIAN_POINT ( 'NONE',  ( 154.4435090467314637, 56.59612921827834953, 16.93085897233502379 ) ) ;
#16808=CARTESIAN_POINT ( 'NONE',  ( 159.6725804802005655, 59.38339663535511903, 44.09291707571413355 ) ) ;
#16811=DIRECTION ( 'NONE',  ( -0.000000000000000000, 1.000000000000000000, -0.000000000000000000 ) ) ;
#16813=CARTESIAN_POINT ( 'NONE',  ( -146.7478996615323013, 63.17828545741220836, -89.01584858309800552 ) ) ;
#16814=EDGE_CURVE ( 'NONE', #30284, #59217, #60099, .T. ) ;
#16815=CARTESIAN_POINT ( 'NONE',  ( -31.92580063159128301, 9.671320706097189301, -23.47264677473817684 ) ) ;
#16816=CARTESIAN_POINT ( 'NONE',  ( -179.8989115484066303, 96.59045402602910713, 41.54463800193268241 ) ) ;
#16817=CARTESIAN_POINT ( 'NONE',  ( 126.6464677212869532, 38.39096133771044350, 61.72361273423263839 ) ) ;
#16818=EDGE_CURVE ( 'NONE', #54444, #27441, #48481, .T. ) ;
#16827=CARTESIAN_POINT ( 'NONE',  ( -38.15923928782687824, 10.79140400702259406, -39.47796947194431993 ) ) ;
#16830=CARTESIAN_POINT ( 'NONE',  ( -128.1219934350341418, 47.97781708504714970, 72.14052271541459049 ) ) ;
#16831=CARTESIAN_POINT ( 'NONE',  ( -48.11161266749828513, 13.96357804763626120, 94.42152535799866087 ) ) ;
#16834=B_SPLINE_CURVE_WITH_KNOTS ( 'NONE', 3,
 ( #67805, #19608, #41068, #62527, #14342, #27292, #10087, #47360, #26613, #5835, #48052, #68817, #52982, #213, #69507, #21327, #5498, #42442, #42775, #43121, #15712, #16401, #53676, #63559, #4470, #57933, #15368, #48730, #64241, #64947, #32582, #37503, #20636, #16052, #47707, #20993, #26951, #10423, #36831, #64594, #63900, #54006, #58269, #42099 ),
 .UNSPECIFIED., .F., .F.,
 ( 4, 2, 2, 2, 2, 2, 2, 2, 2, 2, 2, 2, 2, 2, 2, 2, 2, 2, 2, 2, 2, 4 ),
 ( 0.02495775893651560814, 0.02650251144344294152, 0.02804726395037027489, 0.02959201645729760827, 0.03113676896422493817, 0.03268152147115227502, 0.03345389772461594691, 0.03422627397807962574, 0.03577102648500703197, 0.03654340273847073856, 0.03731577899193443820, 0.03808815524539813785, 0.03886053149886183750, 0.04040528400578929230, 0.04117766025925302664, 0.04195003651271676792, 0.04349478901964425048, 0.04503954152657171917, 0.04581191778003547432, 0.04658429403349922254, 0.04812904654042673980, 0.04967379904735427093 ),
 .UNSPECIFIED. ) ;
#16836=CARTESIAN_POINT ( 'NONE',  ( -98.26894608163135558, 31.90835830144592222, -89.86268561939382948 ) ) ;
#16839=CARTESIAN_POINT ( 'NONE',  ( 210.4897348480408255, 114.6382060222044430, -75.44159559921389757 ) ) ;
#16843=CARTESIAN_POINT ( 'NONE',  ( 19.10949903373832015, 7.636938177523840743, 30.78566702077129591 ) ) ;
#16844=CARTESIAN_POINT ( 'NONE',  ( 197.2820712633967730, 96.69730079225780628, 89.25354394473986019 ) ) ;
#16846=CARTESIAN_POINT ( 'NONE',  ( 164.6561571795775194, 64.77723933022093661, -68.24917283303342685 ) ) ;
#16849=CYLINDRICAL_SURFACE ( 'NONE', #18414, 7.500000000000013323 ) ;
#16853=EDGE_CURVE ( 'NONE', #46836, #60768, #1369, .T. ) ;
#16855=CARTESIAN_POINT ( 'NONE',  ( -84.55373779407982227, 24.65190748253136732, 33.24540446502325608 ) ) ;
#16856=CARTESIAN_POINT ( 'NONE',  ( -28.35957743809534648, 10.12373109553625206, -76.50474426647431869 ) ) ;
#16857=CARTESIAN_POINT ( 'NONE',  ( 43.14565945994675644, 9.942782559600567893, 30.91037901312404657 ) ) ;
#16858=CARTESIAN_POINT ( 'NONE',  ( 130.7531879853686121, 39.58149302537889724, -9.835301198007991630 ) ) ;
#16864=VERTEX_POINT ( 'NONE', #7704 ) ;
#16867=CARTESIAN_POINT ( 'NONE',  ( 59.95259601283825646, 11.98300577492411456, 57.30717056780049745 ) ) ;
#16868=CARTESIAN_POINT ( 'NONE',  ( -0.5658006089934847216, 7.533733779014707643, 62.51359026650904127 ) ) ;
#16869=CARTESIAN_POINT ( 'NONE',  ( -26.87787777325848992, 9.903749977739218835, -90.54880160837116421 ) ) ;
#16872=CARTESIAN_POINT ( 'NONE',  ( -119.5576859660651508, 42.46117483543970650, -73.27934440310555431 ) ) ;
#16876=DIRECTION ( 'NONE',  ( 0.000000000000000000, 0.000000000000000000, 1.000000000000000000 ) ) ;
#16883=CARTESIAN_POINT ( 'NONE',  ( 79.22946426532584496, 17.02750615740071183, 9.120237246954173926 ) ) ;
#16885=LINE ( 'NONE', #65798, #219 ) ;
#16886=CARTESIAN_POINT ( 'NONE',  ( -78.19460645047367109, 22.14203592077027949, 30.41820113967310490 ) ) ;
#16887=ORIENTED_EDGE ( 'NONE', *, *, #4436, .T. ) ;
#16889=CARTESIAN_POINT ( 'NONE',  ( 63.01563776193091826, -170.0000000000000000, 17.96841034875761878 ) ) ;
#16898=CARTESIAN_POINT ( 'NONE',  ( 32.09610685027467980, 8.582590950734841684, 35.70073703131771481 ) ) ;
#16899=CARTESIAN_POINT ( 'NONE',  ( -173.5372686962700755, 89.10569330281724376, -49.71195716475001802 ) ) ;
#16905=CARTESIAN_POINT ( 'NONE',  ( 141.2361973397653401, 47.26569015399787332, -69.00318946062078851 ) ) ;
#16909=FACE_BOUND ( 'NONE', #34496, .T. ) ;
#16910=CARTESIAN_POINT ( 'NONE',  ( -1.728570918131772993, 6.570609986804656799, -74.13742151377635992 ) ) ;
#16912=CARTESIAN_POINT ( 'NONE',  ( 111.7879975195216815, 29.60186808535944891, -89.73033128225488042 ) ) ;
#16916=CARTESIAN_POINT ( 'NONE',  ( -151.2410113808308552, 65.66338888995507261, 4.066252756723934603 ) ) ;
#16917=CARTESIAN_POINT ( 'NONE',  ( -73.26882986836166367, 20.33842609887990704, -91.07877570767612951 ) ) ;
#16918=CARTESIAN_POINT ( 'NONE',  ( -10.24974837193994404, 8.069704751038626611, 44.72969724616100251 ) ) ;
#16919=CARTESIAN_POINT ( 'NONE',  ( 111.8699272271189216, 29.64190505307780654, 2.941473855310829943 ) ) ;
#16920=CARTESIAN_POINT ( 'NONE',  ( 93.08174259058942823, 22.79847752828720786, -12.62219101434053847 ) ) ;
#16921=EDGE_LOOP ( 'NONE', ( #7121, #28218 ) ) ;
#16923=ORIENTED_EDGE ( 'NONE', *, *, #29596, .T. ) ;
#16925=CARTESIAN_POINT ( 'NONE',  ( 81.05403189674299824, 18.64820877954959499, -75.20638625924833320 ) ) ;
#16926=CARTESIAN_POINT ( 'NONE',  ( 102.7974068605285396, 26.68003355195580539, 91.76817536871718062 ) ) ;
#16927=CARTESIAN_POINT ( 'NONE',  ( 39.40195752203892710, -170.0000000000000000, 71.75838489642698903 ) ) ;
#16930=CARTESIAN_POINT ( 'NONE',  ( -27.70185240367226598, 10.02491413133430953, -49.32437352143211484 ) ) ;
#16931=CARTESIAN_POINT ( 'NONE',  ( -47.80251179448169552, 13.89045662648309687, -67.57686690419204467 ) ) ;
#16932=CARTESIAN_POINT ( 'NONE',  ( -76.99081612991844281, 22.76418914851637254, -88.98189906751177602 ) ) ;
#16935=ORIENTED_EDGE ( 'NONE', *, *, #48989, .F. ) ;
#16936=CARTESIAN_POINT ( 'NONE',  ( 31.90170717962883273, 8.563261373066632487, 64.49853757514532049 ) ) ;
#16937=CARTESIAN_POINT ( 'NONE',  ( 175.8855729601531550, 73.50624012737691260, 58.22573703953762703 ) ) ;
#16939=CARTESIAN_POINT ( 'NONE',  ( -165.7140086129056442, 80.68381997492571145, -16.58285276488415150 ) ) ;
#16941=CYLINDRICAL_SURFACE ( 'NONE', #311, 7.500000000000027534 ) ;
#16943=CARTESIAN_POINT ( 'NONE',  ( 87.10672734544989737, 20.64813880796635104, 2.867536982015616687 ) ) ;
#16944=CARTESIAN_POINT ( 'NONE',  ( 188.0103583326377361, 87.39896620268120842, -13.98969534752448496 ) ) ;
#16945=CARTESIAN_POINT ( 'NONE',  ( -80.54757501605355685, 23.04700348514568020, -8.506729827231833241 ) ) ;
#16946=CARTESIAN_POINT ( 'NONE',  ( -79.09055197094342304, 23.56106361828856777, -88.80455181264522935 ) ) ;
#16947=CARTESIAN_POINT ( 'NONE',  ( 45.90693067088658808, 9.344800815249305614, -12.51017037632520790 ) ) ;
#16948=CARTESIAN_POINT ( 'NONE',  ( 211.3917124729449881, 115.9987099435923028, -13.58743899467040528 ) ) ;
#16949=FACE_BOUND ( 'NONE', #37163, .T. ) ;
#16950=CARTESIAN_POINT ( 'NONE',  ( -59.94781924509481286, 16.04872117907065743, -37.02872815368100845 ) ) ;
#16953=CARTESIAN_POINT ( 'NONE',  ( 94.06699947028484132, 23.17027898120150198, -44.31905308565868040 ) ) ;
#16956=CARTESIAN_POINT ( 'NONE',  ( 151.7956716830626647, 53.36999433148312733, 14.97506466355020471 ) ) ;
#16959=CARTESIAN_POINT ( 'NONE',  ( 56.53776994993147298, 11.26292242501185115, 14.25638008219111619 ) ) ;
#16960=CARTESIAN_POINT ( 'NONE',  ( -60.66241560458681903, 16.25736033771447708, 59.65924898650886377 ) ) ;
#16963=ORIENTED_EDGE ( 'NONE', *, *, #40963, .T. ) ;
#16964=CARTESIAN_POINT ( 'NONE',  ( -79.61931371420119774, 22.68640080971621487, -62.00571751209825777 ) ) ;
#16967=CARTESIAN_POINT ( 'NONE',  ( 105.4375968828853161, 26.72149058755205431, 42.87463743524401139 ) ) ;
#16968=ORIENTED_EDGE ( 'NONE', *, *, #24320, .T. ) ;
#16970=AXIS2_PLACEMENT_3D ( 'NONE', #49920, #65779, #33763 ) ;
#16972=CARTESIAN_POINT ( 'NONE',  ( 86.62931800182293784, -170.0000000000000000, 2.867536982015617575 ) ) ;
#16974=CARTESIAN_POINT ( 'NONE',  ( 106.0228389049370321, 28.07756796303169722, 4.061978269566077770 ) ) ;
#16975=CARTESIAN_POINT ( 'NONE',  ( 63.49941241090384381, 13.81848793187418600, 2.968410348757589912 ) ) ;
#16979=AXIS2_PLACEMENT_3D ( 'NONE', #15572, #54572, #420 ) ;
#16980=CARTESIAN_POINT ( 'NONE',  ( -55.05276343752909440, 15.72344139423349141, -35.21632399845986328 ) ) ;
#16982=CARTESIAN_POINT ( 'NONE',  ( 15.29305096970403710, 7.491604910111013815, 45.01470767270526352 ) ) ;
#16991=CARTESIAN_POINT ( 'NONE',  ( -12.39413342787891104, 7.231444436041488011, -10.10556315530504889 ) ) ;
#16992=CARTESIAN_POINT ( 'NONE',  ( -165.6292614779507346, 80.59684587977122305, 92.52285916119727460 ) ) ;
#16995=CARTESIAN_POINT ( 'NONE',  ( -62.41727061481083183, 17.83188723492277461, -41.23329363980502649 ) ) ;
#16996=CARTESIAN_POINT ( 'NONE',  ( -7.825402957745081878, 7.899365992529268965, -23.57352014148015584 ) ) ;
#16997=CARTESIAN_POINT ( 'NONE',  ( -74.40004226286976063, 20.74218500375955898, -75.63308164639384756 ) ) ;
#16998=CARTESIAN_POINT ( 'NONE',  ( 23.09784929786602703, 6.844738137842332648, -14.47737765197590853 ) ) ;
#17003=CARTESIAN_POINT ( 'NONE',  ( -144.9412191745148846, 61.69548892475975066, 17.34567004948121749 ) ) ;
#17005=CARTESIAN_POINT ( 'NONE',  ( 63.01563776193091826, -170.0000000000000000, 91.00206212014866480 ) ) ;
#17007=CARTESIAN_POINT ( 'NONE',  ( -104.1244073710070097, 33.72720758483609416, 18.45900469992847093 ) ) ;
#17009=CARTESIAN_POINT ( 'NONE',  ( 134.7708899521911121, 43.15864772107689618, -24.12637467660490387 ) ) ;
#17014=CARTESIAN_POINT ( 'NONE',  ( -149.5074843970971017, 65.50121172469319220, -7.968279941028269420 ) ) ;
#17015=CARTESIAN_POINT ( 'NONE',  ( 55.51597771111714508, 11.05737652677078664, -15.87642975587560912 ) ) ;
#17017=CARTESIAN_POINT ( 'NONE',  ( -38.16002576456689610, 10.79155573432543491, 61.22331852717874767 ) ) ;
#17024=CARTESIAN_POINT ( 'NONE',  ( -0.3252226420479328861, 7.525368746738510417, -43.40480950733539345 ) ) ;
#17025=CARTESIAN_POINT ( 'NONE',  ( -14.35185884954381308, 8.414771159230838293, 94.99999999999866418 ) ) ;
#17026=CARTESIAN_POINT ( 'NONE',  ( -125.8938041572051389, 46.49392987655491538, 18.77539728269342945 ) ) ;
#17028=CARTESIAN_POINT ( 'NONE',  ( 23.28869764673362042, 6.856674305776600420, 64.84761802070974568 ) ) ;
#17030=CARTESIAN_POINT ( 'NONE',  ( 9.290502160020464473, 6.379616279862540651, -73.61710939586298252 ) ) ;
#17035=CIRCLE ( 'NONE', #56369, 243.4957430088094839 ) ;
#17038=CARTESIAN_POINT ( 'NONE',  ( 46.50207827473963107, 9.439498081273468344, -72.39330090572757115 ) ) ;
#17039=CARTESIAN_POINT ( 'NONE',  ( 60.40531521312254171, 13.11276739283243309, -77.10049446495987979 ) ) ;
#17040=VERTEX_POINT ( 'NONE', #28449 ) ;
#17051=CARTESIAN_POINT ( 'NONE',  ( 140.4769819293526893, 46.76840769395179365, 60.32113923860118376 ) ) ;
#17052=CARTESIAN_POINT ( 'NONE',  ( -78.66644367742111399, 22.32174330031317311, -35.11545063171788428 ) ) ;
#17055=CARTESIAN_POINT ( 'NONE',  ( 16.63342912721455491, 6.527857407601582729, -89.20804527961315955 ) ) ;
#17056=CARTESIAN_POINT ( 'NONE',  ( -189.4248691432192686, 107.3461292335514798, 36.68996308917169813 ) ) ;
#17058=CARTESIAN_POINT ( 'NONE',  ( 112.7784411285249035, 30.07270878825232430, -50.48479703671700491 ) ) ;
#17061=CARTESIAN_POINT ( 'NONE',  ( 39.40195752203892710, 8.409560354027394879, -50.61981746542779348 ) ) ;
#17063=CARTESIAN_POINT ( 'NONE',  ( -129.7656201304987746, 49.09621953108914028, 85.37891732438063741 ) ) ;
#17068=EDGE_CURVE ( 'NONE', #12427, #10027, #41783, .T. ) ;
#17070=CIRCLE ( 'NONE', #24942, 242.4895526022646379 ) ;
#17076=CARTESIAN_POINT ( 'NONE',  ( 79.14242532928582818, 17.00090225993928428, -15.96730280997515194 ) ) ;
#17078=CARTESIAN_POINT ( 'NONE',  ( 93.08533330311585985, 21.72562315962721868, -74.01562841799706405 ) ) ;
#17085=CYLINDRICAL_SURFACE ( 'NONE', #54215, 7.500000000000020428 ) ;
#17089=CARTESIAN_POINT ( 'NONE',  ( -71.22896441287285541, 20.69091426169410397, -70.45909810321082034 ) ) ;
#17091=CARTESIAN_POINT ( 'NONE',  ( 45.76553115525425852, 10.34124506813254918, -47.09660741898280634 ) ) ;
#17092=CARTESIAN_POINT ( 'NONE',  ( 160.4963793545268800, 60.04225845346907420, -77.34568484721802406 ) ) ;
#17093=EDGE_LOOP ( 'NONE', ( #27174, #12989, #52996, #35907 ) ) ;
#17098=CARTESIAN_POINT ( 'NONE',  ( 93.32756701508621688, 22.89083686918420213, 67.46732691414862870 ) ) ;
#17104=CARTESIAN_POINT ( 'NONE',  ( -7.825402957745085430, 7.899365992529246761, 18.27103044898354511 ) ) ;
#17108=CARTESIAN_POINT ( 'NONE',  ( 59.08202327466402437, 12.82375733818954089, 70.54788376517701920 ) ) ;
#17109=CARTESIAN_POINT ( 'NONE',  ( 10.82760985890678640, 7.398654328676807168, -64.21712473681512279 ) ) ;
#17112=CARTESIAN_POINT ( 'NONE',  ( -0.7215816834507543520, 6.532459459468098473, 35.19760772530012360 ) ) ;
#17113=CARTESIAN_POINT ( 'NONE',  ( 83.19706090114061681, 19.33633638213343531, 84.22436956647520390 ) ) ;
#17119=CARTESIAN_POINT ( 'NONE',  ( -129.3963145237381127, 48.84337839101545597, 17.91139487216891624 ) ) ;
#17120=CARTESIAN_POINT ( 'NONE',  ( -167.4860113959265391, 82.52233889531184730, -37.25610511775715850 ) ) ;
#17122=CARTESIAN_POINT ( 'NONE',  ( -133.0835080491125098, 52.64966140620843049, -44.56526587904586734 ) ) ;
#17128=CARTESIAN_POINT ( 'NONE',  ( -147.7860806339125475, 62.73248524776227697, -22.78099747642112760 ) ) ;
#17136=CARTESIAN_POINT ( 'NONE',  ( -99.98584758882479662, 32.75338129098886242, 30.86302090401612119 ) ) ;
#17137=EDGE_CURVE ( 'NONE', #14098, #12427, #41711, .T. ) ;
#17139=DIRECTION ( 'NONE',  ( -0.000000000000000000, 1.000000000000000000, -0.000000000000000000 ) ) ;
#17140=ORIENTED_EDGE ( 'NONE', *, *, #46793, .T. ) ;
#17144=CARTESIAN_POINT ( 'NONE',  ( -118.4753258120605324, 41.79945864152914936, -95.00000000000133582 ) ) ;
#17145=CARTESIAN_POINT ( 'NONE',  ( 8.000000000000007105, 249.8719672152120381, -95.00000000000133582 ) ) ;
#17146=CARTESIAN_POINT ( 'NONE',  ( -14.84903512415885629, 8.461292896365065985, -67.12079146646519234 ) ) ;
#17148=CARTESIAN_POINT ( 'NONE',  ( 164.8471526211110927, 63.62172173173269130, 38.29138183902061598 ) ) ;
#17152=CARTESIAN_POINT ( 'NONE',  ( -75.43271753227892873, 22.18711452892410918, -35.83126050068450041 ) ) ;
#17156=CARTESIAN_POINT ( 'NONE',  ( 174.3243312526346642, 73.41378903026858893, -94.13505484421320091 ) ) ;
#17157=CARTESIAN_POINT ( 'NONE',  ( -38.93878980550033475, 10.94326053663841769, -15.47548683381646129 ) ) ;
#17160=CARTESIAN_POINT ( 'NONE',  ( -34.74312654625182972, 10.15703162223799971, -76.39920896306614395 ) ) ;
#17161=CARTESIAN_POINT ( 'NONE',  ( 19.54452863209719382, 7.657034792877148277, 70.86930329570787990 ) ) ;
#17162=B_SPLINE_CURVE_WITH_KNOTS ( 'NONE', 3,
 ( #8296, #55426, #23777, #7252, #29063, #18153, #13911, #51208, #39952, #56834, #34344, #24819, #29743, #3020, #45923, #67391, #2328, #35026, #61405, #46256, #55787, #45224, #34691, #67735, #19534, #40993, #67053, #56473, #63140, #62451, #14265, #31473, #9680, #10022, #25861, #47289, #31816, #15299, #36754, #10350, #52908, #53248, #4058, #26542 ),
 .UNSPECIFIED., .F., .F.,
 ( 4, 2, 2, 2, 2, 2, 2, 2, 2, 2, 2, 2, 2, 2, 2, 2, 2, 2, 2, 2, 2, 4 ),
 ( 0.02638217555535139758, 0.02805347641364859188, 0.02972477727194578964, 0.03139607813024298394, 0.03306737898854018171, 0.03390302941768880141, 0.03473867984683742804, 0.03640998070513465357, 0.03724563113428327327, 0.03808128156343189297, 0.03891693199258051267, 0.03975258242172913237, 0.04058823285087774513, 0.04142388328002636483, 0.04225953370917498453, 0.04309518413832360423, 0.04476648499662086444, 0.04643778585491813160, 0.04810908671321538488, 0.04978038757151265203, 0.05145168842980990531, 0.05312298928810717247 ),
 .UNSPECIFIED. ) ;
#17163=ORIENTED_EDGE ( 'NONE', *, *, #43245, .F. ) ;
#17168=CARTESIAN_POINT ( 'NONE',  ( -102.2801239173131052, 33.91021738430207222, 3.674523915951417585 ) ) ;
#17171=CARTESIAN_POINT ( 'NONE',  ( -38.55214349681827457, 10.86754840574842262, -45.24580720952189239 ) ) ;
#17172=CARTESIAN_POINT ( 'NONE',  ( -104.6581597602948221, 34.00455924016704046, 84.57040083051070667 ) ) ;
#17174=CARTESIAN_POINT ( 'NONE',  ( -129.6001310305488516, 48.98284622040321068, 71.48886441875946218 ) ) ;
#17177=CARTESIAN_POINT ( 'NONE',  ( 79.52861599156695149, 17.11914630560287875, 61.59085265089968431 ) ) ;
#17180=AXIS2_PLACEMENT_3D ( 'NONE', #57037, #56332, #46463 ) ;
#17182=CARTESIAN_POINT ( 'NONE',  ( 209.6877167158270368, 113.4449353909247407, -65.06643844799334886 ) ) ;
#17184=CARTESIAN_POINT ( 'NONE',  ( -72.21652659655762818, 19.96855882996548459, 7.213640616729523281 ) ) ;
#17186=CARTESIAN_POINT ( 'NONE',  ( -51.34325167237331300, 13.71819364263221708, 17.49572699254425245 ) ) ;
#17188=CARTESIAN_POINT ( 'NONE',  ( 153.8366942494330374, 54.87992279068316037, -37.05910186496495129 ) ) ;
#17190=ORIENTED_EDGE ( 'NONE', *, *, #13648, .F. ) ;
#17194=CARTESIAN_POINT ( 'NONE',  ( 164.6046919270428930, 63.41782451559755174, -95.00000000000133582 ) ) ;
#17196=B_SPLINE_CURVE_WITH_KNOTS ( 'NONE', 3,
 ( #5301, #47167, #52455, #14481, #31352, #58749, #41899, #15168, #36634, #52109, #48188, #31014, #58081, #30659, #21144, #57737, #3926, #31688, #52780, #4607, #20783, #41556, #32037, #42251, #63709, #15, #64043, #53471, #15853, #37297, #20103, #14811, #15520, #25398, #36974, #21470, #26759, #47857, #69320, #35936, #46829, #25737, #68298, #63010 ),
 .UNSPECIFIED., .F., .F.,
 ( 4, 2, 2, 2, 2, 2, 2, 2, 2, 2, 2, 2, 2, 2, 2, 2, 2, 2, 2, 2, 2, 4 ),
 ( 0.02495775893651562202, 0.02650251144344300744, 0.02804726395037039632, 0.02959201645729778174, 0.03113676896422517063, 0.03268152147115255951, 0.03345389772461624528, 0.03422627397807993799, 0.03577102648500731646, 0.03654340273847100223, 0.03731577899193469494, 0.03808815524539838071, 0.03886053149886206648, 0.04040528400578949353, 0.04117766025925322093, 0.04195003651271693446, 0.04349478901964438926, 0.04503954152657183019, 0.04581191778003557147, 0.04658429403349930581, 0.04812904654042679531, 0.04967379904735429175 ),
 .UNSPECIFIED. ) ;
#17197=CARTESIAN_POINT ( 'NONE',  ( -85.91089317961402116, 25.21459833389209493, 35.91092548939403883 ) ) ;
#17198=CARTESIAN_POINT ( 'NONE',  ( -25.48750459758503339, 9.705678256319570707, -74.25185047208405820 ) ) ;
#17199=CARTESIAN_POINT ( 'NONE',  ( 46.90208227351339332, 10.52324439420451618, 37.17192485722242168 ) ) ;
#17202=CARTESIAN_POINT ( 'NONE',  ( 126.9201538765324386, 37.39093565120715112, -13.81500352634632378 ) ) ;
#17208=DIRECTION ( 'NONE',  ( -0.000000000000000000, 1.000000000000000000, -0.000000000000000000 ) ) ;
#17210=CARTESIAN_POINT ( 'NONE',  ( -3.253130881186333756, 7.643323950922366272, 58.49497839819474621 ) ) ;
#17212=CARTESIAN_POINT ( 'NONE',  ( 198.0161777302107851, 99.22276840862558345, -94.07682923140444586 ) ) ;
#17214=ORIENTED_EDGE ( 'NONE', *, *, #12997, .F. ) ;
#17217=CARTESIAN_POINT ( 'NONE',  ( -122.3963566076408114, 44.23346594671846788, -75.90953027873555925 ) ) ;
#17218=EDGE_LOOP ( 'NONE', ( #5968, #40866, #12860, #11528 ) ) ;
#17222=FACE_OUTER_BOUND ( 'NONE', #46725, .T. ) ;
#17224=CARTESIAN_POINT ( 'NONE',  ( 136.1037846510192821, 43.98155406734452555, 17.33612899941342178 ) ) ;
#17228=AXIS2_PLACEMENT_3D ( 'NONE', #4230, #14441, #63318 ) ;
#17230=DIRECTION ( 'NONE',  ( 0.000000000000000000, 0.000000000000000000, 1.000000000000000000 ) ) ;
#17232=CARTESIAN_POINT ( 'NONE',  ( -77.71448999903257970, 21.96089801565738853, 45.37296549835471637 ) ) ;
#17238=FACE_OUTER_BOUND ( 'NONE', #51093, .T. ) ;
#17239=CARTESIAN_POINT ( 'NONE',  ( 93.86680996363769225, 22.01878169039503419, 12.35045139323386643 ) ) ;
#17241=FACE_OUTER_BOUND ( 'NONE', #46103, .T. ) ;
#17246=( BOUNDED_CURVE ( )  B_SPLINE_CURVE ( 3, ( #8772, #30218, #41464, #15756 ),
 .UNSPECIFIED., .F., .F. ) 
 B_SPLINE_CURVE_WITH_KNOTS ( ( 4, 4 ),
 ( 2.506209174768083692, 3.776976132411494103 ),
 .UNSPECIFIED. ) 
 CURVE ( )  GEOMETRIC_REPRESENTATION_ITEM ( )  RATIONAL_B_SPLINE_CURVE ( ( 1.000000000000000000, 0.8698961108463045822, 0.8698961108463045822, 1.000000000000000000 ) ) 
 REPRESENTATION_ITEM ( '' )  );
#17247=CARTESIAN_POINT ( 'NONE',  ( 31.96192885395476679, 8.569232728322429438, 38.39183651277110698 ) ) ;
#17248=CARTESIAN_POINT ( 'NONE',  ( -179.2210908201800521, 95.76260491022613053, -37.81988327838237751 ) ) ;
#17249=CARTESIAN_POINT ( 'NONE',  ( -133.1527834403230770, 51.46311219732125153, -13.66430714595139051 ) ) ;
#17256=FACE_BOUND ( 'NONE', #28707, .T. ) ;
#17257=CARTESIAN_POINT ( 'NONE',  ( -1.319107422865891888, 6.554467368239800251, -73.52547515260555144 ) ) ;
#17258=CARTESIAN_POINT ( 'NONE',  ( -175.9944734395085675, 91.92390745845760591, 72.10689250308911369 ) ) ;
#17259=CARTESIAN_POINT ( 'NONE',  ( -143.8756912989387047, 60.83492035645719653, -10.50900835034600433 ) ) ;
#17262=CARTESIAN_POINT ( 'NONE',  ( 15.78827728214693416, 6.500811158483329244, -62.36349468914946925 ) ) ;
#17265=CARTESIAN_POINT ( 'NONE',  ( 55.76286625948333864, 11.10663164471739606, -95.00000000000133582 ) ) ;
#17266=CARTESIAN_POINT ( 'NONE',  ( 110.2429982417149290, 28.88204397445231209, 2.766663615273646570 ) ) ;
#17267=CARTESIAN_POINT ( 'NONE',  ( 90.91356992076214283, 21.99794663086828450, -10.31639574584678343 ) ) ;
#17268=VERTEX_POINT ( 'NONE', #65222 ) ;
#17269=VECTOR ( 'NONE', #27888, 1000.000000000000000 ) ;
#17270=CARTESIAN_POINT ( 'NONE',  ( -38.54237244144231056, 11.89088379031761811, 13.29149674035523176 ) ) ;
#17271=ORIENTED_EDGE ( 'NONE', *, *, #58265, .F. ) ;
#17273=CARTESIAN_POINT ( 'NONE',  ( 81.57915404881514121, 18.81499384983930057, -75.71637441921426159 ) ) ;
#17274=AXIS2_PLACEMENT_3D ( 'NONE', #13578, #7269, #39963 ) ;
#17275=CARTESIAN_POINT ( 'NONE',  ( 109.0088647218444464, 29.42125915259915203, 83.39562742996727707 ) ) ;
#17277=CARTESIAN_POINT ( 'NONE',  ( 70.11766033381769603, 14.43277633974326335, -18.83692018523840517 ) ) ;
#17278=CARTESIAN_POINT ( 'NONE',  ( -27.49195330402088544, 9.993776132065304907, -49.19917853453215173 ) ) ;
#17280=DIRECTION ( 'NONE',  ( -1.000000000000000000, 0.000000000000000000, 0.000000000000000000 ) ) ;
#17282=CARTESIAN_POINT ( 'NONE',  ( -71.98415129531598211, 20.95325475002097804, -92.86987620278186739 ) ) ;
#17284=AXIS2_PLACEMENT_3D ( 'NONE', #26807, #25448, #47216 ) ;
#17291=CARTESIAN_POINT ( 'NONE',  ( -165.7713056973201731, 80.74264649718247711, 66.68892821721664177 ) ) ;
#17295=VECTOR ( 'NONE', #48936, 1000.000000000000000 ) ;
#17298=CARTESIAN_POINT ( 'NONE',  ( 105.4134760436918441, 27.80903124201756427, -37.66340175651738775 ) ) ;
#17299=CARTESIAN_POINT ( 'NONE',  ( 182.7686108735401547, 81.77235358504611895, -24.20125551499105754 ) ) ;
#17300=CARTESIAN_POINT ( 'NONE',  ( -85.75947274862031122, 25.15128705015481358, -18.25927382592571036 ) ) ;
#17304=FACE_BOUND ( 'NONE', #35211, .T. ) ;
#17305=CARTESIAN_POINT ( 'NONE',  ( -62.15799747763097827, 16.70234469631019536, -45.16847623433110925 ) ) ;
#17306=EDGE_CURVE ( 'NONE', #50199, #34598, #1917, .T. ) ;
#17311=CARTESIAN_POINT ( 'NONE',  ( 92.21252738308864139, 22.47457138983956781, -48.35361511676679669 ) ) ;
#17312=CARTESIAN_POINT ( 'NONE',  ( -47.61402178322637013, 13.84598486314981969, 63.67307924642992845 ) ) ;
#17313=CARTESIAN_POINT ( 'NONE',  ( -180.6021503146988607, 97.45669259943416307, 12.09742955499907247 ) ) ;
#17314=CARTESIAN_POINT ( 'NONE',  ( 211.8345664497466032, 118.5225165986914533, 61.22447077958275941 ) ) ;
#17317=CARTESIAN_POINT ( 'NONE',  ( 56.19513604272052021, 11.19349063094195174, 13.59754376101736817 ) ) ;
#17318=CARTESIAN_POINT ( 'NONE',  ( -55.05276343752909440, 14.68156374112638929, 57.16187836339483397 ) ) ;
#17321=VECTOR ( 'NONE', #42765, 1000.000000000000000 ) ;
#17324=CARTESIAN_POINT ( 'NONE',  ( 102.7571040248401033, 25.57023079238897267, 37.63868481140666944 ) ) ;
#17328=CARTESIAN_POINT ( 'NONE',  ( 160.5018603162735360, 61.33906090758085838, 30.03480990559012298 ) ) ;
#17329=CARTESIAN_POINT ( 'NONE',  ( 103.8325688302027316, 27.12251147381400784, 6.365378839190652727 ) ) ;
#17330=CARTESIAN_POINT ( 'NONE',  ( 67.54641595172915913, 14.80690682047551299, 16.46492756229169530 ) ) ;
#17332=CARTESIAN_POINT ( 'NONE',  ( 88.53517449242353621, 20.08005703101045114, 44.46986225549056115 ) ) ;
#17337=CARTESIAN_POINT ( 'NONE',  ( 181.0840389613909736, 80.03940679743416808, 56.15314469597509373 ) ) ;
#17338=CARTESIAN_POINT ( 'NONE',  ( -149.9125899128210051, 65.84729237358621390, -88.50193171241929235 ) ) ;
#17340=CARTESIAN_POINT ( 'NONE',  ( 89.81152435583800298, 20.53127581368840282, 84.10198394837142644 ) ) ;
#17342=ORIENTED_EDGE ( 'NONE', *, *, #34077, .T. ) ;
#17343=EDGE_LOOP ( 'NONE', ( #3238, #66763, #25825, #6216 ) ) ;
#17344=ORIENTED_EDGE ( 'NONE', *, *, #66988, .T. ) ;
#17345=CARTESIAN_POINT ( 'NONE',  ( -15.22871623201694646, 7.486724405784664249, -17.29878459576774574 ) ) ;
#17346=CARTESIAN_POINT ( 'NONE',  ( -50.13771638889891591, 13.41835215703893347, 43.50352009537876086 ) ) ;
#17349=CARTESIAN_POINT ( 'NONE',  ( -62.29496909743951960, 17.79481128341706153, -40.75095302798493435 ) ) ;
#17352=CARTESIAN_POINT ( 'NONE',  ( 23.03578842369135415, 6.840884649289440844, -18.11974505773217103 ) ) ;
#17355=ORIENTED_EDGE ( 'NONE', *, *, #55101, .T. ) ;
#17357=CARTESIAN_POINT ( 'NONE',  ( -142.0860844253782886, 59.41107357617635643, 10.25687802980160690 ) ) ;
#17358=CARTESIAN_POINT ( 'NONE',  ( -28.93113808661575703, 10.21102608966478265, 84.32986548825184059 ) ) ;
#17359=CARTESIAN_POINT ( 'NONE',  ( -95.21430597939259144, 29.33390900154321912, -45.08002014446414307 ) ) ;
#17364=CARTESIAN_POINT ( 'NONE',  ( 139.2794027252093940, 45.99190465195507471, -11.47524523421667553 ) ) ;
#17371=CARTESIAN_POINT ( 'NONE',  ( -154.8006992380339000, 70.15733562427992354, -10.13360984257536579 ) ) ;
#17374=CARTESIAN_POINT ( 'NONE',  ( 55.76066037845579615, 11.10616952318092387, -18.34132239558550737 ) ) ;
#17379=CARTESIAN_POINT ( 'NONE',  ( 188.2962140587030149, 87.71627202537838741, 61.57422339708019621 ) ) ;
#17380=CARTESIAN_POINT ( 'NONE',  ( 203.9228889538744909, 106.9879579748728275, -78.14080293397877597 ) ) ;
#17383=CARTESIAN_POINT ( 'NONE',  ( 103.0103829243729194, 25.67737053862328622, 12.31638664800049909 ) ) ;
#17384=CARTESIAN_POINT ( 'NONE',  ( -166.2546536130332981, 79.79692681634925577, -92.87286366454794972 ) ) ;
#17386=AXIS2_PLACEMENT_3D ( 'NONE', #32273, #11843, #37189 ) ;
#17390=AXIS2_PLACEMENT_3D ( 'NONE', #45904, #13889, #35352 ) ;
#17394=CARTESIAN_POINT ( 'NONE',  ( 180.2572128312847894, 77.77323980479704346, 29.34246328274604210 ) ) ;
#17395=CARTESIAN_POINT ( 'NONE',  ( -102.2801239173131052, 33.91021738430207932, -76.85912785543962400 ) ) ;
#17396=CARTESIAN_POINT ( 'NONE',  ( 46.50704915687942531, 9.440294391580046351, -67.55012544208800307 ) ) ;
#17400=DIRECTION ( 'NONE',  ( -0.000000000000000000, 1.000000000000000000, -0.000000000000000000 ) ) ;
#17401=CARTESIAN_POINT ( 'NONE',  ( 176.0086785549255239, 73.62390276844820391, 84.96622182719073635 ) ) ;
#17403=EDGE_LOOP ( 'NONE', ( #32111, #34903 ) ) ;
#17404=CARTESIAN_POINT ( 'NONE',  ( -190.6985136298601731, 109.1272424661242582, -95.00000000000133582 ) ) ;
#17408=CARTESIAN_POINT ( 'NONE',  ( 133.8566784816069344, 42.60093787723652525, 56.35489142945903751 ) ) ;
#17409=CARTESIAN_POINT ( 'NONE',  ( -75.00168449119584579, 20.95943092127969365, -36.06733346853133071 ) ) ;
#17412=CARTESIAN_POINT ( 'NONE',  ( -52.68206656346369243, 15.09776187114412593, -8.752186859763938287 ) ) ;
#17413=ORIENTED_EDGE ( 'NONE', *, *, #68150, .T. ) ;
#17414=CARTESIAN_POINT ( 'NONE',  ( 115.0454575488273576, 31.16784721673995406, -49.18829330954620360 ) ) ;
#17416=CARTESIAN_POINT ( 'NONE',  ( -71.86568654225716557, 20.91200104397923809, 7.901464635737869280 ) ) ;
#17417=CARTESIAN_POINT ( 'NONE',  ( -142.1332311300252798, 59.44822332309656332, -43.70847484967913488 ) ) ;
#17418=CARTESIAN_POINT ( 'NONE',  ( -171.0950923142953570, 86.38958441093222973, -76.29032179032941485 ) ) ;
#17420=CARTESIAN_POINT ( 'NONE',  ( -120.6555520024721488, 43.14028137839566313, 86.43234750685729750 ) ) ;
#17422=CARTESIAN_POINT ( 'NONE',  ( 56.52205390515079131, 12.28646189164057390, 14.25333810830040804 ) ) ;
#17423=AXIS2_PLACEMENT_3D ( 'NONE', #49104, #6567, #33660 ) ;
#17424=VECTOR ( 'NONE', #21291, 1000.000000000000000 ) ;
#17426=CARTESIAN_POINT ( 'NONE',  ( -131.3154845336012500, 50.16828105866952825, 32.91510348359927463 ) ) ;
#17432=CARTESIAN_POINT ( 'NONE',  ( 88.98820631332496589, 21.30618275724810573, 30.07647440311880871 ) ) ;
#17433=CARTESIAN_POINT ( 'NONE',  ( 134.3172730033262496, 41.70277427218488953, -9.178760341931965883 ) ) ;
#17434=CARTESIAN_POINT ( 'NONE',  ( -79.14094329813315198, 23.58034730000056811, -23.27090004125423661 ) ) ;
#17435=CARTESIAN_POINT ( 'NONE',  ( 90.30166390191405412, 20.70652093100730440, -76.72363925761264625 ) ) ;
#17436=VECTOR ( 'NONE', #30089, 1000.000000000000000 ) ;
#17437=CARTESIAN_POINT ( 'NONE',  ( -24.80529805274337463, 8.596106904667630388, -92.98064582061705607 ) ) ;
#17438=CARTESIAN_POINT ( 'NONE',  ( -156.9402586331177361, 70.74941713998435944, -95.00000000000133582 ) ) ;
#17441=CARTESIAN_POINT ( 'NONE',  ( 46.85206196242845067, 9.495795933269473466, 36.42025845728678490 ) ) ;
#17442=FACE_OUTER_BOUND ( 'NONE', #36251, .T. ) ;
#17445=CARTESIAN_POINT ( 'NONE',  ( 212.1978255065450583, 119.0880569674902603, -43.47704106856255635 ) ) ;
#17448=CARTESIAN_POINT ( 'NONE',  ( -23.93880457192868860, 8.479983864459176957, -42.57752331243816002 ) ) ;
#17449=DIRECTION ( 'NONE',  ( -0.000000000000000000, 1.000000000000000000, -0.000000000000000000 ) ) ;
#17451=CARTESIAN_POINT ( 'NONE',  ( -24.18158274621863413, 9.527343002918312820, 8.916876208941543425 ) ) ;
#17453=EDGE_LOOP ( 'NONE', ( #28439, #67569, #39886, #58487 ) ) ;
#17455=CARTESIAN_POINT ( 'NONE',  ( -85.57988666922054222, 25.07649479135944048, 88.68161927237834163 ) ) ;
#17457=CARTESIAN_POINT ( 'NONE',  ( 130.3035708464390154, 40.48418876551452428, 43.63269443261444991 ) ) ;
#17458=CARTESIAN_POINT ( 'NONE',  ( 39.40195752203891999, 9.424259417798145577, 18.06928371549960133 ) ) ;
#17467=CARTESIAN_POINT ( 'NONE',  ( 15.29305096970403355, 7.491604910111013815, -62.36349468914947636 ) ) ;
#17468=CARTESIAN_POINT ( 'NONE',  ( -14.56631729561072675, 8.434645566888201884, 14.09560095912131139 ) ) ;
#17471=CARTESIAN_POINT ( 'NONE',  ( 85.36151321841643380, 20.05356632597361255, 83.50184739982738336 ) ) ;
#17473=VERTEX_POINT ( 'NONE', #62729 ) ;
#17476=CARTESIAN_POINT ( 'NONE',  ( -190.6985136298602015, 109.1272424661243434, -10.81538671745452795 ) ) ;
#17477=CARTESIAN_POINT ( 'NONE',  ( -131.6508182719823878, 50.40277850441008667, 6.442247626404384420 ) ) ;
#17479=CARTESIAN_POINT ( 'NONE',  ( -165.7713056973202015, 80.74264649718247711, -40.68927414463811232 ) ) ;
#17481=CARTESIAN_POINT ( 'NONE',  ( -169.0769811399541709, 82.73718697014336954, 85.68819937027275557 ) ) ;
#17488=CARTESIAN_POINT ( 'NONE',  ( -1.096061481932293358, 7.553048580900442843, -73.08327283968297650 ) ) ;
#17489=AXIS2_PLACEMENT_3D ( 'NONE', #9157, #66880, #18676 ) ;
#17490=B_SPLINE_CURVE_WITH_KNOTS ( 'NONE', 3,
 ( #32138, #31792, #52885, #53226, #11359, #32827, #10667, #53575, #58179, #21918, #20892, #54256, #42684, #64143, #15616, #48284, #15957, #37401, #48982, #115, #9998, #64842, #4711, #36735, #69060, #21571, #825, #22273, #43015, #64492, #31451, #16303, #37752, #59200, #11018, #32480, #53913, #5736, #26170, #48626, #42349, #470, #44421, #16982, #39503 ),
 .UNSPECIFIED., .F., .F.,
 ( 4, 2, 2, 1, 2, 2, 2, 2, 2, 2, 2, 2, 2, 2, 2, 2, 2, 2, 2, 2, 2, 2, 4 ),
 ( 0.02346057189573570387, 0.02492590417315497867, 0.02565857031186461606, 0.02639123645057425346, 0.02712390258928389086, 0.02785656872799353173, 0.02932190100541279265, 0.03005456714412241964, 0.03078723328283204316, 0.03225256556025128674, 0.03298523169896092067, 0.03371789783767055459, 0.03518323011508982245, 0.03664856239250909031, 0.03738122853121871036, 0.03811389466992833736, 0.03957922694734757746, 0.04104455922476682450, 0.04250989150218606460, 0.04324255764089569160, 0.04397522377960531165, 0.04544055605702455869, 0.04690588833444379879 ),
 .UNSPECIFIED. ) ;
#17494=CARTESIAN_POINT ( 'NONE',  ( -61.52761555060400411, 17.56359742150278791, 7.155479614208617001 ) ) ;
#17495=CARTESIAN_POINT ( 'NONE',  ( 201.9869293910475392, 102.6997661182766990, -36.82124265982815814 ) ) ;
#17496=CARTESIAN_POINT ( 'NONE',  ( -95.04371414958066566, 30.36527049547257917, 35.98012675971163787 ) ) ;
#17497=CARTESIAN_POINT ( 'NONE',  ( 20.37135563017389828, 6.690359945346088466, -37.06178491685137288 ) ) ;
#17505=CARTESIAN_POINT ( 'NONE',  ( -14.84452950307166752, 8.460866451887705253, -72.41633501155601493 ) ) ;
#17507=CARTESIAN_POINT ( 'NONE',  ( 164.7250737226289914, 63.51898362052163804, 38.83193614737182742 ) ) ;
#17509=FACE_OUTER_BOUND ( 'NONE', #44683, .T. ) ;
#17511=ADVANCED_FACE ( 'NONE', ( #56755 ), #45147, .F. ) ;
#17513=EDGE_CURVE ( 'NONE', #29791, #6856, #34187, .T. ) ;
#17515=CARTESIAN_POINT ( 'NONE',  ( -37.38262509017738466, 10.64263598035110192, -11.37183861185575751 ) ) ;
#17517=CARTESIAN_POINT ( 'NONE',  ( -133.3220917939969468, 52.82057604964899866, 12.34504307300762882 ) ) ;
#17518=B_SPLINE_CURVE_WITH_KNOTS ( 'NONE', 3,
 ( #833, #32149, #53583, #22631, #22281, #49343, #65197, #16992, #1523, #6458, #44070, #22986, #12085, #43719, #5413, #38461, #43027, #28247, #48292, #60615, #37763, #33552, #54979, #6092, #59208, #64850, #16650, #6796, #11028, #44430, #59898, #53923, #5746, #27551, #38107, #65916, #27201, #17713, #24726, #29642, #66952, #7515, #50061, #39852, #12780, #46160, #3266, #39511, #28967, #2572, #67634, #61310, #19428, #13135, #40888, #34242, #13472, #60958, #56036, #29299 ),
 .UNSPECIFIED., .F., .F.,
 ( 4, 2, 2, 2, 2, 2, 2, 2, 2, 2, 2, 2, 2, 2, 2, 2, 2, 2, 2, 2, 2, 2, 2, 2, 2, 2, 2, 2, 2, 4 ),
 ( 0.000000000000000000, 0.001130461533176197342, 0.001695692299764287123, 0.002260923066352376904, 0.003391384599528505725, 0.003956615366116568618, 0.004521846132704631510, 0.005652307665880724336, 0.006782769199056818028, 0.007913230732232909986, 0.009043692265409002812, 0.01017415379858509737, 0.01130461533176118846, 0.01356553839811334809, 0.01469599993128941490, 0.01582646146446547650, 0.01808738453081752684, 0.01921784606399359191, 0.02034830759716966392, 0.02260923066352179406, 0.02487015372987392767, 0.02600061526304999968, 0.02713107679622606822, 0.02826153832940213328, 0.02939199986257820529, 0.03052246139575427383, 0.03165292292893034237, 0.03278338446210641438, 0.03391384599528247945, 0.03617476906163466510 ),
 .UNSPECIFIED. ) ;
#17521=ORIENTED_EDGE ( 'NONE', *, *, #50890, .T. ) ;
#17530=CARTESIAN_POINT ( 'NONE',  ( 8.000000000000007105, 249.8719672152120381, -95.00000000000133582 ) ) ;
#17534=CARTESIAN_POINT ( 'NONE',  ( -133.3926783185151521, 51.63401075114365568, 65.26579531883123764 ) ) ;
#17539=ADVANCED_FACE ( 'NONE', ( #58810 ), #57445, .T. ) ;
#17541=CARTESIAN_POINT ( 'NONE',  ( -95.38834349408374180, 30.52734377185649350, -93.20934587920034176 ) ) ;
#17542=AXIS2_PLACEMENT_3D ( 'NONE', #22566, #65486, #17280 ) ;
#17545=CARTESIAN_POINT ( 'NONE',  ( 187.9007786055418308, 85.78077355327279463, 39.94804133362764276 ) ) ;
#17552=CARTESIAN_POINT ( 'NONE',  ( 151.7956716830626362, 53.36999433148314154, -38.71403651737715279 ) ) ;
#17554=VERTEX_POINT ( 'NONE', #64097 ) ;
#17556=FACE_OUTER_BOUND ( 'NONE', #58132, .T. ) ;
#17557=EDGE_LOOP ( 'NONE', ( #65306, #34157 ) ) ;
#17559=LINE ( 'NONE', #12286, #52032 ) ;
#17562=CARTESIAN_POINT ( 'NONE',  ( -7.825402957745087207, 6.891034867348160731, -62.26262132240749736 ) ) ;
#17569=EDGE_CURVE ( 'NONE', #47669, #25095, #68658, .T. ) ;
#17574=CYLINDRICAL_SURFACE ( 'NONE', #21146, 7.500000000000013323 ) ;
#17576=DIRECTION ( 'NONE',  ( -0.000000000000000000, 1.000000000000000000, -0.000000000000000000 ) ) ;
#17577=CARTESIAN_POINT ( 'NONE',  ( 141.2164820244224188, 47.25271033009985189, 89.21155399097146699 ) ) ;
#17579=FACE_OUTER_BOUND ( 'NONE', #59747, .T. ) ;
#17582=CARTESIAN_POINT ( 'NONE',  ( -118.4553071845215015, 41.78724769484929169, -70.35621148235168221 ) ) ;
#17585=CARTESIAN_POINT ( 'NONE',  ( 164.7250737226290482, 63.51898362052163804, -14.85716503355553186 ) ) ;
#17589=CARTESIAN_POINT ( 'NONE',  ( 137.5911612413395630, 44.91497189902067078, 16.67414218509417267 ) ) ;
#17591=VECTOR ( 'NONE', #45793, 1000.000000000000000 ) ;
#17594=CARTESIAN_POINT ( 'NONE',  ( 79.93126905972556528, 17.24332478304278027, 6.983910173289804568 ) ) ;
#17596=DIRECTION ( 'NONE',  ( -0.000000000000000000, 1.000000000000000000, -0.000000000000000000 ) ) ;
#17600=ORIENTED_EDGE ( 'NONE', *, *, #17782, .F. ) ;
#17602=CARTESIAN_POINT ( 'NONE',  ( 87.10668362745096260, 19.58396519288861981, 2.867536982015615799 ) ) ;
#17606=CARTESIAN_POINT ( 'NONE',  ( 15.78827728214693416, 7.507518794609589818, 30.01470767270522089 ) ) ;
#17608=CARTESIAN_POINT ( 'NONE',  ( 34.82939798935584719, 8.870855050008911391, 43.37903875302355061 ) ) ;
#17609=CARTESIAN_POINT ( 'NONE',  ( -180.5234362879040191, 97.35934147644944403, -40.96444954319694887 ) ) ;
#17610=CARTESIAN_POINT ( 'NONE',  ( -129.4098618459772183, 48.85263848239744533, -22.19798343946113306 ) ) ;
#17613=ORIENTED_EDGE ( 'NONE', *, *, #66169, .F. ) ;
#17617=CARTESIAN_POINT ( 'NONE',  ( -155.7455325080990747, 71.01834415181984639, -38.14091650697321967 ) ) ;
#17619=CARTESIAN_POINT ( 'NONE',  ( -173.9617926765113509, 89.58633395456782011, 72.63082148245895553 ) ) ;
#17620=CARTESIAN_POINT ( 'NONE',  ( -142.0729208125266609, 59.40063722436772053, -14.33066429808441455 ) ) ;
#17623=DIRECTION ( 'NONE',  ( 0.000000000000000000, 0.000000000000000000, 1.000000000000000000 ) ) ;
#17625=EDGE_CURVE ( 'NONE', #39196, #66387, #66888, .T. ) ;
#17628=CARTESIAN_POINT ( 'NONE',  ( -12.77550690612892481, 8.273784096785062658, 31.96002631522175363 ) ) ;
#17629=CARTESIAN_POINT ( 'NONE',  ( 117.4830770399667728, 32.37795270233550582, 12.29057018420397540 ) ) ;
#17631=CARTESIAN_POINT ( 'NONE',  ( -51.01327085356715685, 14.67279453898819774, -90.08252356086848067 ) ) ;
#17634=CARTESIAN_POINT ( 'NONE',  ( -98.68609963468200874, 32.11186931716878945, -35.91459565328016623 ) ) ;
#17636=CYLINDRICAL_SURFACE ( 'NONE', #14969, 7.500000000000020428 ) ;
#17637=EDGE_CURVE ( 'NONE', #68404, #3111, #47517, .T. ) ;
#17638=CARTESIAN_POINT ( 'NONE',  ( 81.74250361646205931, 18.86685472882136949, -64.45562340701054893 ) ) ;
#17640=CARTESIAN_POINT ( 'NONE',  ( 117.6852192568308197, 33.60745169181582526, 91.79304235087180075 ) ) ;
#17643=CARTESIAN_POINT ( 'NONE',  ( -25.49247221749738301, 9.706368398275721177, -38.22028984111819483 ) ) ;
#17646=VECTOR ( 'NONE', #67327, 1000.000000000000000 ) ;
#17647=CARTESIAN_POINT ( 'NONE',  ( -121.5680658099883829, 44.89994870382101055, -21.71427755356253897 ) ) ;
#17648=ORIENTED_EDGE ( 'NONE', *, *, #58052, .T. ) ;
#17651=CARTESIAN_POINT ( 'NONE',  ( 177.0075766083212443, 74.58167636505953624, 57.35343608575345797 ) ) ;
#17653=CARTESIAN_POINT ( 'NONE',  ( -169.8972248494843313, 85.08697738648015729, 71.95279267074467100 ) ) ;
#17654=AXIS2_PLACEMENT_3D ( 'NONE', #20544, #52896, #63471 ) ;
#17655=CARTESIAN_POINT ( 'NONE',  ( -165.6404838346739155, 80.60836113891888033, -14.74958753143211077 ) ) ;
#17656=DIRECTION ( 'NONE',  ( -0.8160245890732938934, -0.5780171883497599028, 0.000000000000000000 ) ) ;
#17660=CARTESIAN_POINT ( 'NONE',  ( 104.7042813665017746, 27.49927371769996753, -38.34174927681518597 ) ) ;
#17661=CARTESIAN_POINT ( 'NONE',  ( -13.78709718204647139, 7.352743657744180261, 59.88331151981780209 ) ) ;
#17665=CARTESIAN_POINT ( 'NONE',  ( 206.7099580236349254, 109.1417833474364301, -9.744738879524000197 ) ) ;
#17666=FACE_BOUND ( 'NONE', #30682, .T. ) ;
#17673=CARTESIAN_POINT ( 'NONE',  ( -173.1211646369891355, 88.63826465341151106, 3.977144016177345254 ) ) ;
#17674=CARTESIAN_POINT ( 'NONE',  ( 212.0779786303465926, 118.9010947973413579, 62.17465067857224881 ) ) ;
#17678=CARTESIAN_POINT ( 'NONE',  ( 57.07734607129818016, 11.37318329671160377, 5.860985816944734417 ) ) ;
#17681=( BOUNDED_CURVE ( )  B_SPLINE_CURVE ( 3, ( #21262, #42030, #47636, #27223 ),
 .UNSPECIFIED., .F., .F. ) 
 B_SPLINE_CURVE_WITH_KNOTS ( ( 4, 4 ),
 ( 2.506209174768083692, 3.034697867209401601 ),
 .UNSPECIFIED. ) 
 CURVE ( )  GEOMETRIC_REPRESENTATION_ITEM ( )  RATIONAL_B_SPLINE_CURVE ( ( 1.000000000000000000, 0.9768600920338827986, 0.9768600920338827986, 1.000000000000000000 ) ) 
 REPRESENTATION_ITEM ( '' )  );
#17686=CARTESIAN_POINT ( 'NONE',  ( -55.05276343752910151, -170.0000000000000000, -69.56087458892355357 ) ) ;
#17687=CARTESIAN_POINT ( 'NONE',  ( 109.7774723066848424, 28.66666416591278832, 29.61121420573730489 ) ) ;
#17692=CARTESIAN_POINT ( 'NONE',  ( 36.99625334683020128, 8.108440754877195289, -23.39589001747485497 ) ) ;
#17693=CARTESIAN_POINT ( 'NONE',  ( 164.9547823171479877, 65.03046442419433504, 36.34978599136820776 ) ) ;
#17695=CARTESIAN_POINT ( 'NONE',  ( -156.4797890011541597, 71.69341087347113728, -71.93454050753067008 ) ) ;
#17697=CARTESIAN_POINT ( 'NONE',  ( 87.59061758233885087, 19.75077892934018919, 44.66581936989094004 ) ) ;
#17699=CARTESIAN_POINT ( 'NONE',  ( -54.57263979903870421, 15.59415114099632049, -50.21632399845990591 ) ) ;
#17702=CARTESIAN_POINT ( 'NONE',  ( -49.43836229152577744, 14.28302414152159905, 5.975335436052684912 ) ) ;
#17703=CARTESIAN_POINT ( 'NONE',  ( -132.9227230387960788, 52.53474289881226156, -12.93935600963513721 ) ) ;
#17706=DIRECTION ( 'NONE',  ( 0.000000000000000000, 0.000000000000000000, 1.000000000000000000 ) ) ;
#17707=LINE ( 'NONE', #2226, #45621 ) ;
#17711=B_SPLINE_CURVE_WITH_KNOTS ( 'NONE', 3,
 ( #19043, #35922, #62992, #30642, #19387, #46117, #4259, #9883, #40845, #36262, #52763, #4589, #47150, #68613, #56679, #20420, #67588, #62302, #35576, #41884, #63341, #15153, #36611, #58064, #26741, #37631, #42227, #32369, #27072, #10202, #5232, #15836, #53451, #37280, #53106, #58730, #21454, #59427, #38323, #48510, #59768, #10549, #11239, #31671, #5960, #64718 ),
 .UNSPECIFIED., .F., .F.,
 ( 4, 2, 2, 2, 2, 2, 2, 2, 2, 2, 2, 2, 2, 2, 2, 2, 2, 2, 2, 2, 2, 2, 4 ),
 ( 0.000000000000000000, 0.003373244802897285618, 0.004216556003621607131, 0.005059867204345928210, 0.006746489605794571236, 0.007589800806518892315, 0.008433112007243214261, 0.009276423207967534473, 0.01011973440869185642, 0.01180635681014048990, 0.01349297921158912339, 0.01433629041231343146, 0.01517960161303773606, 0.01686622401448635220, 0.01770953521521063945, 0.01855284641593493364, 0.02023946881738356018, 0.02108278001810784397, 0.02192609121883212428, 0.02361271362028066756, 0.02445602482100491318, 0.02529933602172915880, 0.02698595842317764310 ),
 .UNSPECIFIED. ) ;
#17713=CARTESIAN_POINT ( 'NONE',  ( -175.2570726302115247, 91.06836304649893066, 84.80383358225134316 ) ) ;
#17717=CARTESIAN_POINT ( 'NONE',  ( -32.41898580403142205, 10.77423026598439648, 72.01293556506519167 ) ) ;
#17719=CARTESIAN_POINT ( 'NONE',  ( -71.26675986148646302, 19.63956187826083166, -68.21173518103694278 ) ) ;
#17724=ADVANCED_FACE ( 'NONE', ( #46806 ), #4252, .F. ) ;
#17727=CARTESIAN_POINT ( 'NONE',  ( -146.1201263095600780, 62.66021356509621398, 18.07158695027811035 ) ) ;
#17729=CARTESIAN_POINT ( 'NONE',  ( -166.0012244511291328, 80.97916541034756222, 35.94679821911269357 ) ) ;
#17732=CIRCLE ( 'NONE', #3739, 243.4957430088094839 ) ;
#17735=CARTESIAN_POINT ( 'NONE',  ( 140.7888851157409817, 46.97220912571249585, -13.80429249087656451 ) ) ;
#17739=AXIS2_PLACEMENT_3D ( 'NONE', #33762, #17208, #49919 ) ;
#17741=CARTESIAN_POINT ( 'NONE',  ( -14.76369756425704161, 7.442560416198674034, 13.65010214637367447 ) ) ;
#17743=CARTESIAN_POINT ( 'NONE',  ( 55.57657751403271362, 11.06944050856662187, -17.36232739209965459 ) ) ;
#17745=CARTESIAN_POINT ( 'NONE',  ( -47.61380558691495679, 12.81230778489787703, 38.80435849991815189 ) ) ;
#17746=CARTESIAN_POINT ( 'NONE',  ( 198.7129816317746247, 100.1061386900356069, 68.08044006511057944 ) ) ;
#17749=CARTESIAN_POINT ( 'NONE',  ( -62.15063206372443005, 17.75106610013996189, -72.03382600977727179 ) ) ;
#17750=CARTESIAN_POINT ( 'NONE',  ( 198.4045886930829568, 99.71425793793704884, -74.75928238610738674 ) ) ;
#17752=CARTESIAN_POINT ( 'NONE',  ( -168.7150276173047700, 82.35404041280325771, 17.56479690237895142 ) ) ;
#17753=LINE ( 'NONE', #13173, #364 ) ;
#17754=FACE_BOUND ( 'NONE', #57706, .T. ) ;
#17756=CARTESIAN_POINT ( 'NONE',  ( -189.6160969562817229, 107.6113660112011843, 89.72857030643531573 ) ) ;
#17760=CARTESIAN_POINT ( 'NONE',  ( 179.4279766878530609, 76.94722012158234747, 29.48164326234083887 ) ) ;
#17761=CARTESIAN_POINT ( 'NONE',  ( -104.7956873821849086, 35.21322275870667795, -76.42854020113006186 ) ) ;
#17762=CARTESIAN_POINT ( 'NONE',  ( 44.35071890818839790, 9.104600422692254114, -64.30759515882533606 ) ) ;
#17765=EDGE_LOOP ( 'NONE', ( #2901, #50975 ) ) ;
#17766=CARTESIAN_POINT ( 'NONE',  ( -132.7866146733880726, 51.20302913291856584, -93.10660668597851952 ) ) ;
#17767=CARTESIAN_POINT ( 'NONE',  ( 188.0368405038881860, 85.93000590718348519, 87.66130298660245046 ) ) ;
#17769=ORIENTED_EDGE ( 'NONE', *, *, #41809, .F. ) ;
#17771=CARTESIAN_POINT ( 'NONE',  ( 150.7770046255793090, 53.87214803240242844, 40.30350261447307503 ) ) ;
#17775=CARTESIAN_POINT ( 'NONE',  ( -173.1211646369891071, 87.12891641440859303, 3.977144016177345254 ) ) ;
#17778=CARTESIAN_POINT ( 'NONE',  ( 21.66908387089111443, 6.759772951853439515, -91.97708651838377136 ) ) ;
#17780=CARTESIAN_POINT ( 'NONE',  ( -189.5329886872043232, 107.4958891766010964, 36.29115481271927734 ) ) ;
#17782=EDGE_CURVE ( 'NONE', #20616, #25774, #21118, .T. ) ;
#17786=EDGE_CURVE ( 'NONE', #41171, #24590, #53784, .T. ) ;
#17787=CARTESIAN_POINT ( 'NONE',  ( -78.19438069111008360, 23.21811806230640229, 3.573650549209444804 ) ) ;
#17788=CARTESIAN_POINT ( 'NONE',  ( -148.0058283997320814, 64.22864592525513672, -49.66416448871609646 ) ) ;
#17790=CARTESIAN_POINT ( 'NONE',  ( -167.1619226259399227, 82.18315278115416334, -73.61743746788761200 ) ) ;
#17791=CARTESIAN_POINT ( 'NONE',  ( 126.6904219525097659, -170.0000000000000000, -95.00000000000133582 ) ) ;
#17793=CARTESIAN_POINT ( 'NONE',  ( 79.19132716134487282, 17.01584750883626995, -44.31649721339067582 ) ) ;
#17797=DIRECTION ( 'NONE',  ( -0.000000000000000000, 1.000000000000000000, -0.000000000000000000 ) ) ;
#17799=CARTESIAN_POINT ( 'NONE',  ( 187.2354698746857196, 85.05376776489252677, -21.20039874324467988 ) ) ;
#17802=CARTESIAN_POINT ( 'NONE',  ( 94.07616572255072640, 22.09777530676766943, -71.19049505762396279 ) ) ;
#17803=CARTESIAN_POINT ( 'NONE',  ( -31.43908319763710679, 10.61114334766715928, -35.31719736520183517 ) ) ;
#17809=CARTESIAN_POINT ( 'NONE',  ( 42.71504753277077526, 8.863481902720392824, 44.14684118498996668 ) ) ;
#17810=CARTESIAN_POINT ( 'NONE',  ( 197.8436586345019919, 97.39326576892290177, -20.07941126599159887 ) ) ;
#17813=CARTESIAN_POINT ( 'NONE',  ( 212.0104729185452186, 118.7959000526603148, -42.12969124680917332 ) ) ;
#17814=CARTESIAN_POINT ( 'NONE',  ( -71.97658551692138929, 20.95070248419150261, -72.85986904017757126 ) ) ;
#17816=CARTESIAN_POINT ( 'NONE',  ( -29.75049355503753645, 9.320234381800286627, -50.12873137353120256 ) ) ;
#17821=DIRECTION ( 'NONE',  ( 0.000000000000000000, 0.000000000000000000, 1.000000000000000000 ) ) ;
#17822=CARTESIAN_POINT ( 'NONE',  ( -86.09999398724994535, 25.29376521564880065, 65.79117337328426629 ) ) ;
#17828=CARTESIAN_POINT ( 'NONE',  ( 45.18191557310396433, 9.231730719146584718, 86.31199235815032011 ) ) ;
#17833=CARTESIAN_POINT ( 'NONE',  ( -11.14668121284976010, 8.139398342256731311, 17.50002341736112399 ) ) ;
#17836=CARTESIAN_POINT ( 'NONE',  ( 126.7877523219523255, 38.47018873135925077, -14.11887035946164204 ) ) ;
#17841=CARTESIAN_POINT ( 'NONE',  ( -35.17718245314462422, 11.25729435722175786, -36.31055870647146833 ) ) ;
#17842=CARTESIAN_POINT ( 'NONE',  ( -169.1122507277982834, 84.24359299875008844, -48.56609460568329695 ) ) ;
#17846=ORIENTED_EDGE ( 'NONE', *, *, #13433, .F. ) ;
#17847=CARTESIAN_POINT ( 'NONE',  ( -118.3960663196801306, 41.75130200162921312, -42.98165142137420958 ) ) ;
#17849=CARTESIAN_POINT ( 'NONE',  ( -146.5341851369305743, 61.69744206542952014, -22.36787375243187981 ) ) ;
#17850=CARTESIAN_POINT ( 'NONE',  ( -3.862560291631544018, 7.672660553664876204, -76.13487047467812374 ) ) ;
#17851=DIRECTION ( 'NONE',  ( -0.000000000000000000, 1.000000000000000000, -0.000000000000000000 ) ) ;
#17853=CARTESIAN_POINT ( 'NONE',  ( -102.2801239173131194, -170.0000000000000000, -69.35912785543959558 ) ) ;
#17854=CARTESIAN_POINT ( 'NONE',  ( 199.3743599161302882, 99.31857334527873604, -38.51805329884761164 ) ) ;
#17856=CARTESIAN_POINT ( 'NONE',  ( 21.42484406671928809, 6.746536496442158359, -47.97273126929388809 ) ) ;
#17857=CARTESIAN_POINT ( 'NONE',  ( 117.6924004117966689, 33.61107268965020722, 9.252808361665987746 ) ) ;
#17860=EDGE_CURVE ( 'NONE', #37583, #1914, #57591, .T. ) ;
#17863=CARTESIAN_POINT ( 'NONE',  ( -125.8938041572051105, 46.49392987655493670, -88.60280507916129977 ) ) ;
#17864=EDGE_CURVE ( 'NONE', #64513, #69562, #9747, .T. ) ;
#17866=FACE_OUTER_BOUND ( 'NONE', #67352, .T. ) ;
#17868=CARTESIAN_POINT ( 'NONE',  ( 163.2886151008987667, 62.32020850087170061, 32.17011112544247453 ) ) ;
#17874=CARTESIAN_POINT ( 'NONE',  ( 173.9832054143776077, 73.09312616907610050, -95.00000000000133582 ) ) ;
#17875=CARTESIAN_POINT ( 'NONE',  ( -35.17686701826945495, 10.23452050416467962, -9.452137265833972180 ) ) ;
#17876=CARTESIAN_POINT ( 'NONE',  ( 112.5537757279407316, 31.07998172410697180, 44.26225647685382114 ) ) ;
#17877=DIRECTION ( 'NONE',  ( -0.000000000000000000, 1.000000000000000000, -0.000000000000000000 ) ) ;
#17878=CARTESIAN_POINT ( 'NONE',  ( 19.10949903373830594, 7.636938177523838078, 57.63021761123498266 ) ) ;
#17879=EDGE_CURVE ( 'NONE', #25774, #37010, #1396, .T. ) ;
#17882=ORIENTED_EDGE ( 'NONE', *, *, #60011, .F. ) ;
#17884=CARTESIAN_POINT ( 'NONE',  ( 210.5151926960689366, 114.6764308336227600, -92.77687245054279686 ) ) ;
#17886=CARTESIAN_POINT ( 'NONE',  ( -109.3386876948163859, 37.66246927061209249, 8.589132535061098750 ) ) ;
#17888=B_SPLINE_CURVE_WITH_KNOTS ( 'NONE', 3,
 ( #52897, #20545, #41669, #52563, #69070, #52221, #8976, #14254, #63472, #42358, #30426, #46948, #63817, #35361, #63126, #14928, #3349, #4719, #24809, #56821, #46244, #47279, #35713, #36396, #41332, #62786, #68073, #26182, #68732, #47617, #19876, #14590, #57848, #9667, #4387, #25850, #42013, #15285 ),
 .UNSPECIFIED., .F., .F.,
 ( 4, 2, 2, 2, 2, 2, 2, 2, 2, 2, 2, 2, 2, 2, 2, 2, 2, 2, 4 ),
 ( 0.000000000000000000, 0.003908178031105422924, 0.005862267046658093186, 0.007816356062210764316, 0.009770445077763435446, 0.01172453409331610484, 0.01270157860109243607, 0.01367862310886876556, 0.01465566761664509506, 0.01563271212442142455, 0.01660975663219775231, 0.01758680113997408007, 0.01954089015552678762, 0.02051793466330317436, 0.02149497917107956110, 0.02344906818663230683, 0.02540315720218505602, 0.02735724621773780174, 0.03126542424884326543 ),
 .UNSPECIFIED. ) ;
#17889=CARTESIAN_POINT ( 'NONE',  ( -31.93184248720559637, 9.672312402099827011, -35.31719736520184227 ) ) ;
#17890=CARTESIAN_POINT ( 'NONE',  ( -106.0165346013910721, 34.71969978529867262, 85.19816686951331519 ) ) ;
#17891=CARTESIAN_POINT ( 'NONE',  ( -144.7571537022063808, 60.25265659240450589, 32.41201323233473630 ) ) ;
#17893=CARTESIAN_POINT ( 'NONE',  ( -71.26746920569854638, 20.70422440535244135, -17.02378192568739479 ) ) ;
#17895=CARTESIAN_POINT ( 'NONE',  ( 79.92465405224845654, 17.24122384219593229, 67.45454031577327214 ) ) ;
#17897=CARTESIAN_POINT ( 'NONE',  ( 38.90894112122320081, 8.345444037631239098, 44.91383430596326320 ) ) ;
#17899=ORIENTED_EDGE ( 'NONE', *, *, #24220, .F. ) ;
#17903=CARTESIAN_POINT ( 'NONE',  ( 37.70762885381311236, 8.195134395012281914, 17.87944627234856299 ) ) ;
#17909=CARTESIAN_POINT ( 'NONE',  ( -105.1656308559908410, 34.27066904145148385, -89.26805114713427258 ) ) ;
#17910=LINE ( 'NONE', #65403, #4895 ) ;
#17915=ORIENTED_EDGE ( 'NONE', *, *, #42965, .F. ) ;
#17916=CARTESIAN_POINT ( 'NONE',  ( -84.97622048504842951, 24.82614411847758262, 33.85642420924052232 ) ) ;
#17918=CARTESIAN_POINT ( 'NONE',  ( 46.23113030541875190, 10.41513832761375902, 40.52388841428868460 ) ) ;
#17919=CARTESIAN_POINT ( 'NONE',  ( -30.94753041835915042, 9.510749728915506296, 72.06100499665289760 ) ) ;
#17925=CARTESIAN_POINT ( 'NONE',  ( 32.15284246740099405, 8.588257691344876932, -14.33592182630315293 ) ) ;
#17927=CARTESIAN_POINT ( 'NONE',  ( -2.177337698256113452, 7.595833446947584555, 15.72975283661752499 ) ) ;
#17928=EDGE_CURVE ( 'NONE', #964, #347, #59319, .T. ) ;
#17929=CARTESIAN_POINT ( 'NONE',  ( 139.9539301108215739, 46.42810403146213361, 86.31909232689017131 ) ) ;
#17930=CARTESIAN_POINT ( 'NONE',  ( -26.06926405629031862, 9.787505506543544342, -91.25298045410747250 ) ) ;
#17936=CARTESIAN_POINT ( 'NONE',  ( 157.9160637431159842, 57.99786926216935257, -9.279633708673957315 ) ) ;
#17939=CARTESIAN_POINT ( 'NONE',  ( -132.1086844338047968, 51.95575954690575315, -91.87852830952506622 ) ) ;
#17942=VERTEX_POINT ( 'NONE', #21709 ) ;
#17944=VERTEX_POINT ( 'NONE', #13259 ) ;
#17945=B_SPLINE_CURVE_WITH_KNOTS ( 'NONE', 3,
 ( #11277, #43282, #64757, #68979, #32746, #38021, #32407, #59466, #10584, #31707, #20807, #42267, #36989, #58428, #4970, #53492, #39416, #50325, #6709, #16905, #34155, #60864, #38365, #7423, #1798, #17968, #65460, #12689, #2143, #60523, #33460, #55590, #22192, #43632, #45034, #28517, #27815, #54535, #66517, #7059, #11989, #54176, #5998, #23253, #1435, #28875, #59810, #6361 ),
 .UNSPECIFIED., .F., .F.,
 ( 4, 2, 2, 2, 2, 2, 2, 2, 2, 2, 2, 2, 2, 2, 2, 2, 2, 2, 2, 2, 2, 2, 2, 4 ),
 ( 0.000000000000000000, 0.001591515129442145314, 0.003183030258884290628, 0.003978787823605363719, 0.004774545388326435942, 0.006366060517768672329, 0.007957575647210907849, 0.009549090776653144236, 0.01034484834137428325, 0.01114060590609542052, 0.01193636347081656127, 0.01273212103553770028, 0.01432363616497998003, 0.01591515129442225632, 0.01671090885914341614, 0.01750666642386457250, 0.01830242398858572886, 0.01909818155330688522, 0.02068969668274922222, 0.02148545424747039245, 0.02228121181219156269, 0.02387272694163382683, 0.02466848450635492421, 0.02546424207107601118 ),
 .UNSPECIFIED. ) ;
#17946=EDGE_CURVE ( 'NONE', #32357, #23050, #35792, .T. ) ;
#17947=CARTESIAN_POINT ( 'NONE',  ( 8.288104306525688969, 6.376394648992966374, 37.02812928323293562 ) ) ;
#17949=CARTESIAN_POINT ( 'NONE',  ( -62.15799747763099248, 16.70234469631019891, -72.01302682479479245 ) ) ;
#17952=CARTESIAN_POINT ( 'NONE',  ( -142.6264002846223491, 58.55577336362196661, -72.15276126393024470 ) ) ;
#17953=EDGE_CURVE ( 'NONE', #40777, #45231, #65183, .T. ) ;
#17955=CARTESIAN_POINT ( 'NONE',  ( 93.08533330311588827, 21.72562315962718316, 6.518023353393929575 ) ) ;
#17960=CARTESIAN_POINT ( 'NONE',  ( 68.58775259640211175, 15.07340320468039430, 85.97092029086265086 ) ) ;
#17962=CARTESIAN_POINT ( 'NONE',  ( -180.2188652555597059, 96.98354576637424884, -44.65256448004029721 ) ) ;
#17963=CARTESIAN_POINT ( 'NONE',  ( -127.6861178856153174, 47.68458428355324941, -8.272562232425640261 ) ) ;
#17966=EDGE_CURVE ( 'NONE', #38367, #62594, #14847, .T. ) ;
#17968=CARTESIAN_POINT ( 'NONE',  ( 141.0792860804899362, 47.16255757051794006, -72.45897467894479860 ) ) ;
#17969=LINE ( 'NONE', #39417, #19754 ) ;
#17974=CARTESIAN_POINT ( 'NONE',  ( -156.9919426121902575, 72.16759471857101005, -41.74996328242564658 ) ) ;
#17976=CARTESIAN_POINT ( 'NONE',  ( -34.52542994698665524, 11.14027065218092538, 44.55630013575089521 ) ) ;
#17977=B_SPLINE_CURVE_WITH_KNOTS ( 'NONE', 3,
 ( #7505, #13124, #60602, #7840, #24019, #28958, #39502, #45463, #27898, #65541 ),
 .UNSPECIFIED., .F., .F.,
 ( 4, 2, 2, 2, 4 ),
 ( 0.000000000000000000, 0.002532684671119367868, 0.005065369342238735736, 0.007598054013358103605, 0.01013073868447747147 ),
 .UNSPECIFIED. ) ;
#17978=CARTESIAN_POINT ( 'NONE',  ( -125.4463376280758666, 47.40387005565908396, -49.90373998702522584 ) ) ;
#17981=CARTESIAN_POINT ( 'NONE',  ( 204.6977192012829789, 106.3443248447423315, -90.01503221354893469 ) ) ;
#17983=CARTESIAN_POINT ( 'NONE',  ( -8.800520192024523070, 7.964629484975260354, 30.16296264417345796 ) ) ;
#17984=CARTESIAN_POINT ( 'NONE',  ( 115.7561705820728832, 31.51689401996054940, 5.158855458972969821 ) ) ;
#17985=CARTESIAN_POINT ( 'NONE',  ( -49.24265782934394764, 14.23563200896309944, -91.65785725018901076 ) ) ;
#17986=VERTEX_POINT ( 'NONE', #15507 ) ;
#17987=CARTESIAN_POINT ( 'NONE',  ( -95.88693721180811735, 30.76307528361166632, -38.58507135938980781 ) ) ;
#17991=CARTESIAN_POINT ( 'NONE',  ( 46.50207827473964528, 9.439498081273466568, 61.82945204659085903 ) ) ;
#17995=DIRECTION ( 'NONE',  ( 0.000000000000000000, 0.000000000000000000, 1.000000000000000000 ) ) ;
#18000=CARTESIAN_POINT ( 'NONE',  ( 173.6718135456487175, 71.42581476597409562, 64.83443665985362259 ) ) ;
#18003=FACE_OUTER_BOUND ( 'NONE', #25734, .T. ) ;
#18007=CARTESIAN_POINT ( 'NONE',  ( 103.1695711638930675, 26.83837309506523994, -45.96618726772155128 ) ) ;
#18008=CARTESIAN_POINT ( 'NONE',  ( -13.47680110791658414, 7.324966777230640602, 59.50465629245588417 ) ) ;
#18010=FACE_OUTER_BOUND ( 'NONE', #6956, .T. ) ;
#18013=FACE_BOUND ( 'NONE', #12083, .T. ) ;
#18018=CARTESIAN_POINT ( 'NONE',  ( -47.55256438668344998, 13.83151366677316751, 64.41967513731664496 ) ) ;
#18020=CARTESIAN_POINT ( 'NONE',  ( 212.0104729185451617, 118.7959000526603148, 65.24851111504561629 ) ) ;
#18026=CARTESIAN_POINT ( 'NONE',  ( -61.86845765289631771, 16.61548683002701310, 61.52210724104570261 ) ) ;
#18027=ORIENTED_EDGE ( 'NONE', *, *, #34391, .F. ) ;
#18033=CARTESIAN_POINT ( 'NONE',  ( 93.87650740736114585, 23.09802612281732337, -72.16249582444707755 ) ) ;
#18038=CARTESIAN_POINT ( 'NONE',  ( 45.35146934743632841, 10.27620685439441672, 68.85146973395555392 ) ) ;
#18040=CARTESIAN_POINT ( 'NONE',  ( -153.6994314938755508, 69.16570456337667849, -62.92160878217510600 ) ) ;
#18041=CARTESIAN_POINT ( 'NONE',  ( 65.39792658623288446, 14.27332852928128304, 17.58415113736946722 ) ) ;
#18042=DIRECTION ( 'NONE',  ( 0.000000000000000000, 0.000000000000000000, 1.000000000000000000 ) ) ;
#18045=CARTESIAN_POINT ( 'NONE',  ( -52.45048892661851170, 15.03803514841137989, 18.01105719937357108 ) ) ;
#18046=CARTESIAN_POINT ( 'NONE',  ( -133.1566699306513613, 52.70203339370773676, -17.45938862731309982 ) ) ;
#18048=CARTESIAN_POINT ( 'NONE',  ( 116.6457744947906576, 31.95847117670277271, -20.49168429770345057 ) ) ;
#18049=CARTESIAN_POINT ( 'NONE',  ( 89.21144084104753347, 20.31809526687001011, 83.85219840701643079 ) ) ;
#18055=EDGE_CURVE ( 'NONE', #5211, #62965, #53110, .T. ) ;
#18057=CARTESIAN_POINT ( 'NONE',  ( 39.40195752203892710, 8.409560354027373563, 3.069283715499574683 ) ) ;
#18060=CARTESIAN_POINT ( 'NONE',  ( -47.55235941796723154, 12.79790236059689690, -15.63410455582077496 ) ) ;
#18061=CARTESIAN_POINT ( 'NONE',  ( 109.3079614081140249, 28.45126415661782104, -9.121775627028522848 ) ) ;
#18063=DIRECTION ( 'NONE',  ( 0.000000000000000000, 0.000000000000000000, 1.000000000000000000 ) ) ;
#18064=CARTESIAN_POINT ( 'NONE',  ( 197.6004232003112691, 98.70028881297372436, 87.96336489920018664 ) ) ;
#18066=DIRECTION ( 'NONE',  ( 0.000000000000000000, 0.000000000000000000, 1.000000000000000000 ) ) ;
#18067=CARTESIAN_POINT ( 'NONE',  ( -31.43908319763710679, -170.0000000000000000, -69.66174795566553257 ) ) ;
#18068=CARTESIAN_POINT ( 'NONE',  ( -14.66033866466834290, 7.432913330382390882, 34.51814378902125213 ) ) ;
#18071=VERTEX_POINT ( 'NONE', #343 ) ;
#18072=VERTEX_POINT ( 'NONE', #16534 ) ;
#18073=CARTESIAN_POINT ( 'NONE',  ( 66.94365390260637128, 14.65531706601760220, -22.76986491362554332 ) ) ;
#18074=CARTESIAN_POINT ( 'NONE',  ( 185.1660960081723601, 84.30194217633005849, -76.86554811553853028 ) ) ;
#18075=CARTESIAN_POINT ( 'NONE',  ( -165.7713056973201731, 80.74264649718247711, 39.84437762675292305 ) ) ;
#18077=LINE ( 'NONE', #65214, #41948 ) ;
#18079=LINE ( 'NONE', #60633, #65164 ) ;
#18085=CARTESIAN_POINT ( 'NONE',  ( -14.66033866466835178, 7.432913330382392658, 7.673593198557576045 ) ) ;
#18088=CARTESIAN_POINT ( 'NONE',  ( -50.52927270563907314, 13.51486287463704450, 31.81483795138946036 ) ) ;
#18089=CARTESIAN_POINT ( 'NONE',  ( 200.4574930424075774, 102.3536505870638393, 69.75582401855196224 ) ) ;
#18091=DIRECTION ( 'NONE',  ( -0.000000000000000000, 1.000000000000000000, -0.000000000000000000 ) ) ;
#18092=CARTESIAN_POINT ( 'NONE',  ( 203.9203998321608537, 106.9845510704142697, -63.20045979005953285 ) ) ;
#18094=CARTESIAN_POINT ( 'NONE',  ( -176.3791001330698975, 90.82833141237287577, -35.44199699171532103 ) ) ;
#18095=CARTESIAN_POINT ( 'NONE',  ( 104.3805245147141392, 26.26278144139197579, 5.562406129255382581 ) ) ;
#18096=CARTESIAN_POINT ( 'NONE',  ( -166.6071433144410037, 80.15880179908651826, -92.17533033734891035 ) ) ;
#18099=CARTESIAN_POINT ( 'NONE',  ( -189.2325002986007689, 107.0800987204799526, 92.40455112761441114 ) ) ;
#18103=CARTESIAN_POINT ( 'NONE',  ( -132.9409505933031710, 51.31241517713429090, -71.87791970829563581 ) ) ;
#18106=LINE ( 'NONE', #61015, #42342 ) ;
#18109=CARTESIAN_POINT ( 'NONE',  ( -131.2343730941296371, 50.11186611108016820, -90.81774647483901219 ) ) ;
#18110=EDGE_CURVE ( 'NONE', #59334, #67246, #54851, .T. ) ;
#18111=CARTESIAN_POINT ( 'NONE',  ( 188.5644522364758870, 86.51145810658317714, 91.17804384666513329 ) ) ;
#18116=CARTESIAN_POINT ( 'NONE',  ( 176.6258282025055166, 74.21441092921637050, -49.76063806208458118 ) ) ;
#18117=CARTESIAN_POINT ( 'NONE',  ( -179.5178913137216341, 94.54206947403386607, -65.10235975007549314 ) ) ;
#18124=CARTESIAN_POINT ( 'NONE',  ( -6.851003965218992242, 6.829052369041588300, 3.318326975726704209 ) ) ;
#18127=CARTESIAN_POINT ( 'NONE',  ( 187.0823097343935331, -170.0000000000000000, 94.99999999999866418 ) ) ;
#18128=CARTESIAN_POINT ( 'NONE',  ( -28.81071653159242629, 10.19258396314335080, -8.944014519512462513 ) ) ;
#18129=CARTESIAN_POINT ( 'NONE',  ( -51.34562532494748410, 14.75613283840036694, -9.333915665647241511 ) ) ;
#18132=CARTESIAN_POINT ( 'NONE',  ( -73.80418150970712077, 21.59712875466423654, 5.341802012060386851 ) ) ;
#18133=CARTESIAN_POINT ( 'NONE',  ( 39.40195752203891999, 8.409560354027407314, -35.61981746542776506 ) ) ;
#18134=CARTESIAN_POINT ( 'NONE',  ( 93.85477471612979627, -170.0000000000000000, -95.00000000000133582 ) ) ;
#18135=CARTESIAN_POINT ( 'NONE',  ( -127.0849870577083749, 47.28206282326217291, 84.38230841396455162 ) ) ;
#18137=CARTESIAN_POINT ( 'NONE',  ( 81.57482918025354479, 17.75786713398421313, -37.77517181019251780 ) ) ;
#18139=DIRECTION ( 'NONE',  ( -0.000000000000000000, 1.000000000000000000, -0.000000000000000000 ) ) ;
#18140=CARTESIAN_POINT ( 'NONE',  ( 86.62931800182293784, 20.48449268398422518, 29.71208757247930521 ) ) ;
#18146=CARTESIAN_POINT ( 'NONE',  ( -178.2448732545370547, 94.58403736950705820, -9.870808133259494355 ) ) ;
#18150=MANIFOLD_SOLID_BREP ( 'Cut-Extrude1', #60892 ) ;
#18152=CARTESIAN_POINT ( 'NONE',  ( 45.04360969585144403, 9.210232288266709588, 42.37982661523464856 ) ) ;
#18153=CARTESIAN_POINT ( 'NONE',  ( 160.4963793545269084, 60.04225845346905999, 56.87706810510036348 ) ) ;
#18155=CARTESIAN_POINT ( 'NONE',  ( 212.1734186221015932, 119.0499290057855291, -43.13375900917836248 ) ) ;
#18156=B_SPLINE_CURVE_WITH_KNOTS ( 'NONE', 3,
 ( #44586, #34399, #33700, #44223, #7306, #33350, #50215, #28402, #60054, #2376, #23491, #6606, #65709, #12235, #66067, #50559, #65350, #23836, #54782, #55843, #17857, #44931, #11516, #66416, #18206, #39659, #45278, #18551, #32986, #54420, #6248, #27702, #10793, #11138, #37526, #21348 ),
 .UNSPECIFIED., .F., .F.,
 ( 4, 2, 2, 2, 2, 2, 2, 2, 2, 2, 2, 2, 2, 2, 2, 2, 2, 4 ),
 ( 3.469446951953614189E-18, 0.001545474820159047037, 0.003090949640318090604, 0.004636424460477133955, 0.006181899280636177739, 0.007727374100795224125, 0.008500111510874739512, 0.009272848920954255766, 0.01081832374111328654, 0.01236379856127231558, 0.01390927338143134462, 0.01545474820159037539, 0.01700022302174940617, 0.01854569784190843520, 0.02009117266206746424, 0.02163664748222649328, 0.02318212230238552579, 0.02472759712254455136 ),
 .UNSPECIFIED. ) ;
#18157=CARTESIAN_POINT ( 'NONE',  ( -75.65611349188964141, 22.26947559308019819, -76.33353871646717437 ) ) ;
#18158=CARTESIAN_POINT ( 'NONE',  ( -109.7078892845591582, 36.71702188566217728, 65.93493008401821953 ) ) ;
#18159=CARTESIAN_POINT ( 'NONE',  ( -31.43908319763710679, -170.0000000000000000, -96.50629854612921577 ) ) ;
#18170=CARTESIAN_POINT ( 'NONE',  ( 132.9453095272139649, 42.04754713161463542, 44.51034083899536853 ) ) ;
#18171=DIRECTION ( 'NONE',  ( -0.000000000000000000, 1.000000000000000000, -0.000000000000000000 ) ) ;
#18175=CARTESIAN_POINT ( 'NONE',  ( 61.33840119549017800, 13.32121602003046590, 29.99886885364463041 ) ) ;
#18176=CARTESIAN_POINT ( 'NONE',  ( 33.20336330085616083, 7.683867620844146984, 86.82877894857017509 ) ) ;
#18179=CARTESIAN_POINT ( 'NONE',  ( 55.64941011647476898, 12.11006142851271505, 65.63107993823560093 ) ) ;
#18181=CARTESIAN_POINT ( 'NONE',  ( 80.34841469379381351, 17.37275484083203381, 94.99999999999866418 ) ) ;
#18183=CARTESIAN_POINT ( 'NONE',  ( 203.9181091394787302, 105.2759068139671399, 71.05227132923315025 ) ) ;
#18184=CARTESIAN_POINT ( 'NONE',  ( -95.30586079737264527, 29.37688003290242733, -93.43552264237898441 ) ) ;
#18186=ORIENTED_EDGE ( 'NONE', *, *, #1415, .T. ) ;
#18192=CARTESIAN_POINT ( 'NONE',  ( -173.0336157925723910, 87.03110432393005169, 84.50715133059941309 ) ) ;
#18195=CARTESIAN_POINT ( 'NONE',  ( -142.1381007084227406, 58.17237452544243581, -16.88903420692564339 ) ) ;
#18196=CARTESIAN_POINT ( 'NONE',  ( -4.502148936856957384, 7.704491846230415497, -63.02114756112786864 ) ) ;
#18199=EDGE_LOOP ( 'NONE', ( #1495, #55031, #69116, #52228 ) ) ;
#18200=CARTESIAN_POINT ( 'NONE',  ( -55.05276343752909440, 15.72344139423348430, 3.472777182467473800 ) ) ;
#18203=CARTESIAN_POINT ( 'NONE',  ( -98.67557579989345129, 32.10670856967971076, 31.42459644286125453 ) ) ;
#18204=CARTESIAN_POINT ( 'NONE',  ( 18.19980344696536534, 6.589834367837007711, -50.12491448036190889 ) ) ;
#18206=CARTESIAN_POINT ( 'NONE',  ( 116.6681538161788865, 33.09439081574000596, 6.366003624344346967 ) ) ;
#18214=CARTESIAN_POINT ( 'NONE',  ( 173.9405361758639117, 73.05302209498820787, 39.11095342079327963 ) ) ;
#18216=CARTESIAN_POINT ( 'NONE',  ( 22.29513692215318343, 6.796052026456516515, -73.62533078381031260 ) ) ;
#18217=CARTESIAN_POINT ( 'NONE',  ( -15.07533778868020136, 8.482826962130836534, -67.82638443619325130 ) ) ;
#18220=CARTESIAN_POINT ( 'NONE',  ( -30.46358361599563480, 10.45190018822943578, 45.16857927621155966 ) ) ;
#18221=CARTESIAN_POINT ( 'NONE',  ( -71.26746920569853216, 20.70422440535242359, -43.86833251615107088 ) ) ;
#18223=CARTESIAN_POINT ( 'NONE',  ( 210.0122310839192039, 115.7355030290287488, -65.35538431068530940 ) ) ;
#18225=CARTESIAN_POINT ( 'NONE',  ( -180.5234362879040191, 97.35934147644942982, 39.56920222819405808 ) ) ;
#18227=CARTESIAN_POINT ( 'NONE',  ( 23.04797191264876233, 7.849755664016357493, 62.41308431887384955 ) ) ;
#18231=CARTESIAN_POINT ( 'NONE',  ( 207.0339556760109474, 109.6008634273003111, -90.38007673268727160 ) ) ;
#18232=CARTESIAN_POINT ( 'NONE',  ( -33.36721086971962080, 9.915747831546610769, -35.56515356514455561 ) ) ;
#18234=CARTESIAN_POINT ( 'NONE',  ( -142.0062637385109952, 58.06920992247431457, 38.77129379673751686 ) ) ;
#18235=CARTESIAN_POINT ( 'NONE',  ( -127.6992109187851980, 47.69334801994794049, 57.67066701129382267 ) ) ;
#18237=ORIENTED_EDGE ( 'NONE', *, *, #8738, .F. ) ;
#18240=CARTESIAN_POINT ( 'NONE',  ( -94.87734348028330089, 30.28727895192195874, -95.00000000000133582 ) ) ;
#18245=CARTESIAN_POINT ( 'NONE',  ( -47.95193882091086834, 12.89180642785319897, 8.508404476638974145 ) ) ;
#18247=CARTESIAN_POINT ( 'NONE',  ( 156.5977259323288138, 56.97512126940429766, -51.08633290075279376 ) ) ;
#18249=CARTESIAN_POINT ( 'NONE',  ( 159.2258951716709419, 60.31399909112328572, -77.77388725095455868 ) ) ;
#18250=ORIENTED_EDGE ( 'NONE', *, *, #42370, .T. ) ;
#18252=CARTESIAN_POINT ( 'NONE',  ( -106.1135431881943134, 34.77124450854139326, -89.75381755830838415 ) ) ;
#18256=CARTESIAN_POINT ( 'NONE',  ( -56.01329802674225533, 15.98369420723827083, 57.20787140630700662 ) ) ;
#18257=CARTESIAN_POINT ( 'NONE',  ( 126.6904219525097659, 37.26255867422720058, -95.00000000000133582 ) ) ;
#18260=CARTESIAN_POINT ( 'NONE',  ( -12.39413342787891459, 7.231444436041488899, -63.79466433623242949 ) ) ;
#18262=CARTESIAN_POINT ( 'NONE',  ( -34.06864996337442619, 10.03773626259441976, 44.74462983094167612 ) ) ;
#18264=CARTESIAN_POINT ( 'NONE',  ( -28.13266652174641180, 9.071935854491416151, 71.29729791657065618 ) ) ;
#18275=CARTESIAN_POINT ( 'NONE',  ( -2.869721780807581002, 7.625909776230889392, 16.42176429208887711 ) ) ;
#18276=CARTESIAN_POINT ( 'NONE',  ( -0.5178428571329636299, 7.532057582089301206, 66.16617111386234740 ) ) ;
#18278=EDGE_CURVE ( 'NONE', #63051, #18617, #41470, .T. ) ;
#18279=CARTESIAN_POINT ( 'NONE',  ( -123.4531143159639157, 44.90777521523904880, -76.35369456291449808 ) ) ;
#18280=ORIENTED_EDGE ( 'NONE', *, *, #28584, .F. ) ;
#18283=CARTESIAN_POINT ( 'NONE',  ( 70.11766033381769603, 14.43277633974325980, 61.69673158615264441 ) ) ;
#18284=CARTESIAN_POINT ( 'NONE',  ( -131.2399641789143061, 51.34350731997123063, -90.82310783052086833 ) ) ;
#18286=EDGE_LOOP ( 'NONE', ( #10547, #44440 ) ) ;
#18287=CARTESIAN_POINT ( 'NONE',  ( 164.8914542114683286, 64.97670918603530765, -17.90087482810826813 ) ) ;
#18288=CARTESIAN_POINT ( 'NONE',  ( 9.058156535714477542, 6.378495712187263855, 34.19564460572066622 ) ) ;
#18290=CARTESIAN_POINT ( 'NONE',  ( -58.33245019990697244, 15.58496056636070470, -62.79849011809130133 ) ) ;
#18291=DIRECTION ( 'NONE',  ( -0.000000000000000000, 1.000000000000000000, -0.000000000000000000 ) ) ;
#18293=ORIENTED_EDGE ( 'NONE', *, *, #49593, .T. ) ;
#18294=CARTESIAN_POINT ( 'NONE',  ( 164.9700808964341832, 65.04346068891118193, -43.33544459004915694 ) ) ;
#18299=CARTESIAN_POINT ( 'NONE',  ( -96.43817545481741149, 31.02509717589734706, 6.444619006422381169 ) ) ;
#18301=CARTESIAN_POINT ( 'NONE',  ( 69.86170716612186027, 15.40591680861103363, 87.92076547287929600 ) ) ;
#18303=CARTESIAN_POINT ( 'NONE',  ( -179.2128128997734962, 95.75254520622993937, -46.61551081691593623 ) ) ;
#18304=CARTESIAN_POINT ( 'NONE',  ( -128.9786047358386156, 48.55852351614670681, -8.728974343352884802 ) ) ;
#18305=VECTOR ( 'NONE', #66556, 1000.000000000000000 ) ;
#18306=CARTESIAN_POINT ( 'NONE',  ( -145.7962722587128894, 61.09447270426119303, -89.48102063609030665 ) ) ;
#18307=CARTESIAN_POINT ( 'NONE',  ( 130.3019683985926349, 39.31883119822048656, -76.98905284259865311 ) ) ;
#18313=CARTESIAN_POINT ( 'NONE',  ( -154.0716379918897303, 69.49957566103796580, -48.28304949762831910 ) ) ;
#18315=CARTESIAN_POINT ( 'NONE',  ( -31.93169728792083362, 10.69234447276977029, 45.21645440618919309 ) ) ;
#18316=EDGE_CURVE ( 'NONE', #11917, #51047, #36189, .T. ) ;
#18317=FACE_OUTER_BOUND ( 'NONE', #22447, .T. ) ;
#18318=LINE ( 'NONE', #39773, #64040 ) ;
#18320=CARTESIAN_POINT ( 'NONE',  ( -1.454841858088666839, 7.566772088227303961, -20.03908844737443218 ) ) ;
#18321=CARTESIAN_POINT ( 'NONE',  ( -13.92109095214680003, 8.375243258322932149, 33.23919069653987179 ) ) ;
#18322=CARTESIAN_POINT ( 'NONE',  ( -31.43908319763709258, 9.591432048623767415, -35.31719736520183517 ) ) ;
#18323=VERTEX_POINT ( 'NONE', #52364 ) ;
#18326=CARTESIAN_POINT ( 'NONE',  ( 105.2506154496929867, 26.63995206619730638, -64.66458505761366382 ) ) ;
#18327=CARTESIAN_POINT ( 'NONE',  ( 45.04020069093780876, 10.22779424730543063, -11.30540839519373719 ) ) ;
#18333=CARTESIAN_POINT ( 'NONE',  ( 204.6977192012829789, 106.3443248447423315, 71.05227132923315025 ) ) ;
#18334=VERTEX_POINT ( 'NONE', #35497 ) ;
#18339=CARTESIAN_POINT ( 'NONE',  ( 46.68054346512387554, 9.468156054376091646, -95.00000000000133582 ) ) ;
#18340=CARTESIAN_POINT ( 'NONE',  ( 109.3047140914111708, 29.55674059952506738, 71.41186036636744916 ) ) ;
#18342=CARTESIAN_POINT ( 'NONE',  ( -170.2856292770788684, 85.50720222068218845, -22.32389805880076850 ) ) ;
#18346=VERTEX_POINT ( 'NONE', #63268 ) ;
#18347=CARTESIAN_POINT ( 'NONE',  ( 106.4072861358878441, 28.24787347451998443, -36.97294736244227664 ) ) ;
#18348=CARTESIAN_POINT ( 'NONE',  ( 20.35964562795319921, 7.697260051881318788, -37.05298214970821391 ) ) ;
#18352=FACE_BOUND ( 'NONE', #59547, .T. ) ;
#18357=ORIENTED_EDGE ( 'NONE', *, *, #13431, .F. ) ;
#18359=CARTESIAN_POINT ( 'NONE',  ( 90.51709546286271291, 21.85407654229979713, -49.73978282941543938 ) ) ;
#18361=CARTESIAN_POINT ( 'NONE',  ( 36.09469435220862721, 9.015003538710471886, -76.71338776024327899 ) ) ;
#18362=CARTESIAN_POINT ( 'NONE',  ( 181.0840389613909736, -170.0000000000000000, -70.56960825634330092 ) ) ;
#18363=CARTESIAN_POINT ( 'NONE',  ( 152.1190604254709626, 53.60705199010332933, 4.804158789010992692 ) ) ;
#18369=CARTESIAN_POINT ( 'NONE',  ( 200.8303160266299301, 102.8412051751308809, -37.38573241369641664 ) ) ;
#18373=CARTESIAN_POINT ( 'NONE',  ( -85.10774223992955001, 24.88053943842881566, -73.31006263638853682 ) ) ;
#18374=CARTESIAN_POINT ( 'NONE',  ( -60.95805269991217301, 17.39401718769327232, -20.50189859807008830 ) ) ;
#18375=CARTESIAN_POINT ( 'NONE',  ( -189.2776534485022069, 108.4862893474047638, -95.00000000000133582 ) ) ;
#18378=CARTESIAN_POINT ( 'NONE',  ( 46.90170507415071910, 10.52318308703818417, 64.75371562520641078 ) ) ;
#18379=CARTESIAN_POINT ( 'NONE',  ( 164.9706294237034570, 65.04392654036658428, 36.63534575754673028 ) ) ;
#18385=CARTESIAN_POINT ( 'NONE',  ( -128.1267916618074594, 49.19573276651588856, -8.394488801384238030 ) ) ;
#18387=CYLINDRICAL_SURFACE ( 'NONE', #2897, 7.500000000000013323 ) ;
#18388=DIRECTION ( 'NONE',  ( -0.000000000000000000, 1.000000000000000000, -0.000000000000000000 ) ) ;
#18392=ORIENTED_EDGE ( 'NONE', *, *, #7295, .T. ) ;
#18394=CARTESIAN_POINT ( 'NONE',  ( 42.03492317486906416, 8.766487167902388578, 3.542427428059454986 ) ) ;
#18395=CARTESIAN_POINT ( 'NONE',  ( 174.6307688320643479, 73.70327352127003451, 6.133243260141832742 ) ) ;
#18398=CARTESIAN_POINT ( 'NONE',  ( 105.2506154496929014, 26.63995206619730638, -10.97548387668630809 ) ) ;
#18399=CARTESIAN_POINT ( 'NONE',  ( 140.7314320101251610, 45.73329916786966720, -94.18496931662966176 ) ) ;
#18401=CARTESIAN_POINT ( 'NONE',  ( 211.2889559786411269, 117.6796425177967507, 93.97986437182990471 ) ) ;
#18404=CARTESIAN_POINT ( 'NONE',  ( -73.10694748374055507, 20.28107308417883914, -74.51766719739275402 ) ) ;
#18406=EDGE_CURVE ( 'NONE', #18346, #31575, #57987, .T. ) ;
#18407=EDGE_LOOP ( 'NONE', ( #28057, #60553 ) ) ;
#18412=DIRECTION ( 'NONE',  ( -0.000000000000000000, 1.000000000000000000, -0.000000000000000000 ) ) ;
#18413=CARTESIAN_POINT ( 'NONE',  ( 183.7875981612219789, 82.83906702837187197, -63.57054041331110028 ) ) ;
#18414=AXIS2_PLACEMENT_3D ( 'NONE', #43582, #28458, #44640 ) ;
#18415=CARTESIAN_POINT ( 'NONE',  ( -167.4860113959265675, 82.52233889531186151, 43.27754665363389108 ) ) ;
#18416=CARTESIAN_POINT ( 'NONE',  ( -98.69283175933884422, 30.99524616306738523, -49.11836846358093567 ) ) ;
#18419=CARTESIAN_POINT ( 'NONE',  ( 139.6150621148398159, 46.20856238844172026, -11.84746746713147481 ) ) ;
#18421=EDGE_CURVE ( 'NONE', #18508, #49272, #25709, .T. ) ;
#18424=CARTESIAN_POINT ( 'NONE',  ( 187.9768140620194856, 87.36183560332112563, 93.45980768820729168 ) ) ;
#18425=CARTESIAN_POINT ( 'NONE',  ( -10.23867141318105922, 7.059827648235819098, 3.652912843573254076 ) ) ;
#18427=CARTESIAN_POINT ( 'NONE',  ( 56.53776994993148008, 11.26292242501184937, -12.58817050827255990 ) ) ;
#18430=EDGE_CURVE ( 'NONE', #22557, #47203, #66833, .T. ) ;
#18431=CARTESIAN_POINT ( 'NONE',  ( -190.6985136298601731, 109.1272424661242582, 33.97142148329322708 ) ) ;
#18434=CARTESIAN_POINT ( 'NONE',  ( 43.96062659677685502, 10.06332325923985849, -63.98880687523393362 ) ) ;
#18435=CARTESIAN_POINT ( 'NONE',  ( -55.53456145826333312, 15.85318253404851419, -77.06087458892361042 ) ) ;
#18436=CARTESIAN_POINT ( 'NONE',  ( 201.9822477997852843, 104.3642793804899469, -77.67341262940828983 ) ) ;
#18437=CARTESIAN_POINT ( 'NONE',  ( -178.0633751203918393, 92.80295726428047942, -36.56588663441552711 ) ) ;
#18438=CARTESIAN_POINT ( 'NONE',  ( 103.5588133492865239, 25.91050225236394056, 6.827373951400315555 ) ) ;
#18439=CARTESIAN_POINT ( 'NONE',  ( -166.7068579965636559, 80.26142964949319492, 7.581365930921141860 ) ) ;
#18440=DIRECTION ( 'NONE',  ( -0.000000000000000000, 1.000000000000000000, -0.000000000000000000 ) ) ;
#18441=FACE_BOUND ( 'NONE', #40769, .T. ) ;
#18442=B_SPLINE_CURVE_WITH_KNOTS ( 'NONE', 3,
 ( #9347, #31167, #25545, #51912, #36427, #57882, #42045, #68439, #63168, #45944, #41368, #15318, #8673, #58224, #67411, #30811, #9701, #13934, #36781, #9017, #14288, #52596, #3719, #19557, #57544, #4417, #25881, #68768, #30127, #52258, #20583, #4080, #56855, #19202, #41017, #51578, #24842, #46281, #46980, #35748, #57199, #25198, #46633, #161, #516, #17026 ),
 .UNSPECIFIED., .F., .F.,
 ( 4, 2, 2, 2, 2, 2, 2, 2, 2, 2, 2, 2, 2, 2, 2, 2, 2, 2, 2, 2, 2, 2, 4 ),
 ( 0.02584318557310394740, 0.02743529570732768444, 0.02823135077443953908, 0.02902740584155139719, 0.03061951597577510994, 0.03221162610999882270, 0.03380373624422253892, 0.03459979131133440050, 0.03539584637844626902, 0.03619190144555813060, 0.03698795651266999218, 0.03858006664689372228, 0.03937612171400558386, 0.04017217678111744544, 0.04096823184822930702, 0.04176428691534117554, 0.04335639704956488483, 0.04494850718378860799, 0.04654061731801232421, 0.04813272745223604043, 0.04892878251934790201, 0.04972483758645974972, 0.05131694772068350757 ),
 .UNSPECIFIED. ) ;
#18445=CARTESIAN_POINT ( 'NONE',  ( -5.416136198635856935, 6.745992685878681172, 57.35339821038935781 ) ) ;
#18449=CARTESIAN_POINT ( 'NONE',  ( 150.7770046255792522, 53.87214803240241423, 67.14805320493677243 ) ) ;
#18453=EDGE_CURVE ( 'NONE', #68783, #42507, #60045, .T. ) ;
#18454=CARTESIAN_POINT ( 'NONE',  ( 63.01563776193090405, 13.70579113808097382, -62.56524142263340593 ) ) ;
#18459=CARTESIAN_POINT ( 'NONE',  ( -190.6985136298602015, 109.1272424661243434, -91.34903848884556510 ) ) ;
#18465=CARTESIAN_POINT ( 'NONE',  ( 157.4703587214989113, 58.92748579479260229, 44.40946747225338953 ) ) ;
#18468=CARTESIAN_POINT ( 'NONE',  ( 112.5612011511789916, 31.08353758940340583, 56.80732943995488426 ) ) ;
#18469=CARTESIAN_POINT ( 'NONE',  ( -173.9548930713590948, 88.06040582145364226, 4.011895594186154490 ) ) ;
#18470=CARTESIAN_POINT ( 'NONE',  ( -0.3249717932738292459, 6.518578686837482650, 11.25919877780879119 ) ) ;
#18471=CARTESIAN_POINT ( 'NONE',  ( -80.54915509118116290, 24.12810583352861826, 30.65442206072611597 ) ) ;
#18472=CARTESIAN_POINT ( 'NONE',  ( -24.95010104166213694, 9.631487977190600347, -12.20383126445008948 ) ) ;
#18477=CARTESIAN_POINT ( 'NONE',  ( -75.00636493611888511, 22.03142602679957207, 17.63766438757768995 ) ) ;
#18478=CARTESIAN_POINT ( 'NONE',  ( 46.76970795284346138, 9.482505412758889918, -41.65468810189092608 ) ) ;
#18479=CARTESIAN_POINT ( 'NONE',  ( 175.0857681883884140, 74.13486472930382831, 94.99999999999866418 ) ) ;
#18484=CARTESIAN_POINT ( 'NONE',  ( -149.0732005398558329, 63.81212100765652906, 72.55592966969389579 ) ) ;
#18485=CARTESIAN_POINT ( 'NONE',  ( 79.13041963748371188, 18.04952109592811738, 36.69187788337345069 ) ) ;
#18487=CARTESIAN_POINT ( 'NONE',  ( 187.5325688887158435, 85.37769363979909087, -13.01233762806074168 ) ) ;
#18488=CARTESIAN_POINT ( 'NONE',  ( 136.1310312718402713, 42.81430973242787985, -9.516980025434266466 ) ) ;
#18490=CARTESIAN_POINT ( 'NONE',  ( -179.2128128997735246, 95.75254520622988252, -19.77096022645222106 ) ) ;
#18491=EDGE_CURVE ( 'NONE', #30189, #12795, #18969, .T. ) ;
#18493=CARTESIAN_POINT ( 'NONE',  ( -152.9121563765243934, 67.12206067149027433, -35.62635434278646329 ) ) ;
#18496=CARTESIAN_POINT ( 'NONE',  ( 104.3805245147141818, 26.26278144139195447, 59.25150731018273831 ) ) ;
#18502=CARTESIAN_POINT ( 'NONE',  ( -107.7893514267588273, 35.66840175773126731, 59.75090616082049166 ) ) ;
#18504=CARTESIAN_POINT ( 'NONE',  ( -29.51060362117876323, 9.282716514427262311, -50.06914130735744095 ) ) ;
#18508=VERTEX_POINT ( 'NONE', #67099 ) ;
#18510=ORIENTED_EDGE ( 'NONE', *, *, #52020, .F. ) ;
#18511=DIRECTION ( 'NONE',  ( -0.000000000000000000, 1.000000000000000000, -0.000000000000000000 ) ) ;
#18513=CYLINDRICAL_SURFACE ( 'NONE', #17274, 7.500000000000013323 ) ;
#18521=CARTESIAN_POINT ( 'NONE',  ( 62.05396267233468421, 13.48332220860126185, 29.85900607173965682 ) ) ;
#18526=CARTESIAN_POINT ( 'NONE',  ( -190.6985136298601731, 109.1272424661242582, -46.56223028809779407 ) ) ;
#18527=CARTESIAN_POINT ( 'NONE',  ( -143.8566410313463280, 59.53044870492033880, 16.33386445224493144 ) ) ;
#18529=DIRECTION ( 'NONE',  ( 0.000000000000000000, 0.000000000000000000, 1.000000000000000000 ) ) ;
#18530=CARTESIAN_POINT ( 'NONE',  ( 129.5225439633634892, 40.02995148249141266, -22.81789598513682549 ) ) ;
#18533=CARTESIAN_POINT ( 'NONE',  ( 128.3889472838589256, 39.37765603157611594, -38.36644464280026057 ) ) ;
#18534=CARTESIAN_POINT ( 'NONE',  ( -38.54237244144231056, 11.89088379031760034, -40.39760444057212396 ) ) ;
#18537=CARTESIAN_POINT ( 'NONE',  ( -190.6985136298602015, 109.1272424661243434, -37.65993730791821292 ) ) ;
#18538=VERTEX_POINT ( 'NONE', #35765 ) ;
#18539=CARTESIAN_POINT ( 'NONE',  ( -121.5677746760273834, 43.71038933438992302, -36.26883008344502457 ) ) ;
#18542=CARTESIAN_POINT ( 'NONE',  ( -142.2166122762983491, 58.23386571792348576, 93.70268379333128905 ) ) ;
#18547=CARTESIAN_POINT ( 'NONE',  ( 197.5334904971816741, 97.00846725096931777, -41.58470127245635695 ) ) ;
#18548=CARTESIAN_POINT ( 'NONE',  ( -156.9232798886536955, 72.10386843399173529, 37.06393818096253767 ) ) ;
#18549=CARTESIAN_POINT ( 'NONE',  ( 22.52576749827964164, 6.809805260274350402, -46.35021364760256546 ) ) ;
#18551=CARTESIAN_POINT ( 'NONE',  ( 115.0606351894211201, 32.29586232625067055, 4.497561513806664024 ) ) ;
#18557=CARTESIAN_POINT ( 'NONE',  ( 173.6024011093111028, 72.73634049052010653, 36.20546616912848492 ) ) ;
#18558=VECTOR ( 'NONE', #44861, 1000.000000000000000 ) ;
#18559=CARTESIAN_POINT ( 'NONE',  ( -38.78626392836186909, 10.91334659013840103, -95.00000000000133582 ) ) ;
#18560=CARTESIAN_POINT ( 'NONE',  ( -8.810383862755527318, 7.965311326754785703, -62.31117607751706089 ) ) ;
#18561=ORIENTED_EDGE ( 'NONE', *, *, #38763, .T. ) ;
#18563=CARTESIAN_POINT ( 'NONE',  ( -24.18158274621863768, 9.527343002918312820, 35.76142679940522129 ) ) ;
#18566=CARTESIAN_POINT ( 'NONE',  ( 207.8407634284391463, 112.5209879629464069, -63.84769439563109472 ) ) ;
#18568=CARTESIAN_POINT ( 'NONE',  ( 141.3586046882815310, 47.34625111366352002, 36.50144467960451777 ) ) ;
#18571=CARTESIAN_POINT ( 'NONE',  ( 133.8566784816069060, 42.60093787723655367, 71.35489142945907304 ) ) ;
#18578=CARTESIAN_POINT ( 'NONE',  ( -53.36220652957118915, 14.23444203126018337, -89.08613737882753014 ) ) ;
#18582=CARTESIAN_POINT ( 'NONE',  ( -62.29227808534486144, 17.79399661465416926, 93.49242969035836381 ) ) ;
#18585=CARTESIAN_POINT ( 'NONE',  ( -107.0544991134679691, 36.41543129049375693, 32.22994866574824613 ) ) ;
#18588=CARTESIAN_POINT ( 'NONE',  ( 32.67604581760325289, 7.629767527669977234, 40.74140668430740675 ) ) ;
#18592=CARTESIAN_POINT ( 'NONE',  ( -7.825402957745085430, 7.899365992529246761, 45.11558103944722120 ) ) ;
#18598=CARTESIAN_POINT ( 'NONE',  ( -11.78188048797445653, 8.190559674012728664, -49.29436824631886083 ) ) ;
#18601=CIRCLE ( 'NONE', #47803, 243.4957430088094839 ) ;
#18608=CARTESIAN_POINT ( 'NONE',  ( -55.05276343752909440, 15.72344139423348430, 57.16187836339483397 ) ) ;
#18613=CARTESIAN_POINT ( 'NONE',  ( 150.0516754638056511, 53.34587188591232376, -71.60412932141241527 ) ) ;
#18614=CARTESIAN_POINT ( 'NONE',  ( -97.88309373898358956, 30.60238467438961862, -21.76468407524414417 ) ) ;
#18615=CARTESIAN_POINT ( 'NONE',  ( 136.1081004736419402, 42.80058051492065374, -50.68110568597454346 ) ) ;
#18617=VERTEX_POINT ( 'NONE', #13953 ) ;
#18618=CARTESIAN_POINT ( 'NONE',  ( -124.9927180788553898, 45.90286323198616714, 45.57935678244711397 ) ) ;
#18620=DIRECTION ( 'NONE',  ( 0.000000000000000000, 0.000000000000000000, 1.000000000000000000 ) ) ;
#18621=CARTESIAN_POINT ( 'NONE',  ( 182.7720841008444097, 80.32850885226589810, 2.653340975719014949 ) ) ;
#18630=CARTESIAN_POINT ( 'NONE',  ( 66.94779593213117153, 13.61918177102166361, 70.54877072614397093 ) ) ;
#18631=CARTESIAN_POINT ( 'NONE',  ( 159.2325040199867203, 60.31699144791975442, 17.41041423679662259 ) ) ;
#18633=B_SPLINE_CURVE_WITH_KNOTS ( 'NONE', 3,
 ( #62878, #19973, #30180, #45662, #67812, #3782, #51292, #68166, #67468, #67141, #57255, #51634, #62175, #19262, #14678, #19615, #34769, #40716, #18578, #30520, #56555, #13995, #9068, #35451 ),
 .UNSPECIFIED., .F., .F.,
 ( 4, 2, 2, 2, 2, 2, 2, 2, 2, 2, 2, 4 ),
 ( 0.000000000000000000, 0.001312585275339593583, 0.002625170550679187167, 0.003937755826018780533, 0.004594048463688570928, 0.005250341101358362191, 0.006562926376697901347, 0.007219219014367670925, 0.007875511652037439636, 0.009188096927376999609, 0.009844389565046790871, 0.01050068220271658387 ),
 .UNSPECIFIED. ) ;
#18635=CARTESIAN_POINT ( 'NONE',  ( 162.8034185388970059, 63.22443559329413176, -22.07472928994418737 ) ) ;
#18637=VERTEX_POINT ( 'NONE', #56512 ) ;
#18639=CARTESIAN_POINT ( 'NONE',  ( 70.45451534980408326, 15.56315969138428557, 63.16980466599618182 ) ) ;
#18640=CARTESIAN_POINT ( 'NONE',  ( 132.3624812100102304, 40.52933787053994052, -89.85320261638416639 ) ) ;
#18643=CARTESIAN_POINT ( 'NONE',  ( 164.1352994389932007, 64.33767534192698179, -47.07368343251171439 ) ) ;
#18646=EDGE_CURVE ( 'NONE', #62158, #1104, #3898, .T. ) ;
#18647=CARTESIAN_POINT ( 'NONE',  ( 159.2319614735956179, 59.03334608081210177, -50.92782365232224606 ) ) ;
#18649=AXIS2_PLACEMENT_3D ( 'NONE', #18714, #60576, #2195 ) ;
#18652=CARTESIAN_POINT ( 'NONE',  ( -99.10674985723787245, 32.31836975419498970, 4.362585564299135577 ) ) ;
#18653=EDGE_CURVE ( 'NONE', #47821, #15908, #27285, .T. ) ;
#18655=EDGE_CURVE ( 'NONE', #52004, #35148, #12844, .T. ) ;
#18656=CARTESIAN_POINT ( 'NONE',  ( 65.29852862277677161, 14.24903302186932841, 83.85046607615447556 ) ) ;
#18658=AXIS2_PLACEMENT_3D ( 'NONE', #26451, #26793, #48219 ) ;
#18659=CARTESIAN_POINT ( 'NONE',  ( 79.12879321038293767, 18.04902206524927166, -16.24110779498484547 ) ) ;
#18661=CARTESIAN_POINT ( 'NONE',  ( -165.6398193834832853, 79.16932278174807891, 37.71096669259078737 ) ) ;
#18662=CARTESIAN_POINT ( 'NONE',  ( 37.76393697770887314, 9.215659441295981580, -89.47842326396359169 ) ) ;
#18663=CARTESIAN_POINT ( 'NONE',  ( 129.5193594945039308, 38.86618897895344560, -64.23098118280410063 ) ) ;
#18664=VERTEX_POINT ( 'NONE', #50467 ) ;
#18666=CARTESIAN_POINT ( 'NONE',  ( -14.93280618462406650, 8.469244267267916015, 66.86749277915568257 ) ) ;
#18667=EDGE_LOOP ( 'NONE', ( #61356, #55529 ) ) ;
#18669=CARTESIAN_POINT ( 'NONE',  ( -156.9232798886536671, 72.10386843399172108, -43.46971359042848349 ) ) ;
#18670=CARTESIAN_POINT ( 'NONE',  ( 208.9585401441656245, 114.1617785893844399, -10.79275703727707203 ) ) ;
#18672=CARTESIAN_POINT ( 'NONE',  ( -0.5178428571329642960, 7.532057582089303871, 39.32162052339865710 ) ) ;
#18673=FACE_OUTER_BOUND ( 'NONE', #2666, .T. ) ;
#18674=CARTESIAN_POINT ( 'NONE',  ( -52.66507163626135224, 14.05394608175174476, -62.43469777390021136 ) ) ;
#18675=CARTESIAN_POINT ( 'NONE',  ( -0.3732240621745012144, 7.527003275829102336, -15.09420860379144891 ) ) ;
#18676=DIRECTION ( 'NONE',  ( 0.000000000000000000, 0.000000000000000000, 1.000000000000000000 ) ) ;
#18677=CARTESIAN_POINT ( 'NONE',  ( -59.57733000654213384, 15.94108165424592016, 4.971641029624789709 ) ) ;
#18680=EDGE_LOOP ( 'NONE', ( #44285, #28630, #15149, #64999 ) ) ;
#18681=CARTESIAN_POINT ( 'NONE',  ( 109.7774723066848850, 28.66666416591279187, -77.76698815611739235 ) ) ;
#18685=CARTESIAN_POINT ( 'NONE',  ( 42.03492317486906416, 8.766487167902386801, 57.23152860898684224 ) ) ;
#18688=CARTESIAN_POINT ( 'NONE',  ( 15.78827728214693416, -170.0000000000000000, 10.67015708224156079 ) ) ;
#18690=CARTESIAN_POINT ( 'NONE',  ( -171.4867114763003713, 85.32693843184999594, 57.83474805468819113 ) ) ;
#18697=CARTESIAN_POINT ( 'NONE',  ( 103.5849290181279230, 27.01613348792539071, 60.49401056488979833 ) ) ;
#18700=CARTESIAN_POINT ( 'NONE',  ( 55.64941011647476898, 12.11006142851270617, -14.90257183315545397 ) ) ;
#18704=CARTESIAN_POINT ( 'NONE',  ( -82.32931163805226049, 23.75065981441937879, -22.32008095138030157 ) ) ;
#18707=CARTESIAN_POINT ( 'NONE',  ( 8.581702583691640740, 6.376899981419158259, -94.58808349776735724 ) ) ;
#18708=CARTESIAN_POINT ( 'NONE',  ( -23.95089599695169014, 9.496585844566151735, -70.15026316693982267 ) ) ;
#18713=CARTESIAN_POINT ( 'NONE',  ( 37.46876540261053634, 9.179568636624027889, -77.21507226135139490 ) ) ;
#18714=CARTESIAN_POINT ( 'NONE',  ( 204.6977192012829789, -170.0000000000000000, 90.39682191969680503 ) ) ;
#18715=CARTESIAN_POINT ( 'NONE',  ( 210.5008983495071675, 116.4753531594350591, 68.30981121570347625 ) ) ;
#18716=CARTESIAN_POINT ( 'NONE',  ( 79.14242532928582818, 17.00090225993928783, -69.65640399090251833 ) ) ;
#18721=CARTESIAN_POINT ( 'NONE',  ( -78.66644367742111399, -170.0000000000000000, 45.41820113967312977 ) ) ;
#18723=CARTESIAN_POINT ( 'NONE',  ( -80.55742067659895156, 23.05042616197515315, -76.73329829129131952 ) ) ;
#18724=CYLINDRICAL_SURFACE ( 'NONE', #42245, 7.500000000000013323 ) ;
#18725=CARTESIAN_POINT ( 'NONE',  ( 94.02861641584115659, 23.15570573563315548, -71.41699682199956101 ) ) ;
#18730=CARTESIAN_POINT ( 'NONE',  ( 23.28785143291466397, 6.856621069835718174, 10.16897003589188841 ) ) ;
#18735=AXIS2_PLACEMENT_3D ( 'NONE', #8908, #2330, #30705 ) ;
#18736=CARTESIAN_POINT ( 'NONE',  ( 59.29474530993687154, 12.86968658439546509, -36.70420577007838858 ) ) ;
#18737=CARTESIAN_POINT ( 'NONE',  ( -132.0870433264402948, 51.94057326482882075, -11.33156610799026609 ) ) ;
#18738=CARTESIAN_POINT ( 'NONE',  ( 117.3110050642448101, 32.29133253383018598, -19.13666864001427470 ) ) ;
#18739=CARTESIAN_POINT ( 'NONE',  ( 82.34401416830215226, 19.05992892018825557, -49.48157865267160105 ) ) ;
#18740=FACE_OUTER_BOUND ( 'NONE', #25014, .T. ) ;
#18741=ORIENTED_EDGE ( 'NONE', *, *, #63302, .T. ) ;
#18747=CARTESIAN_POINT ( 'NONE',  ( -55.05276343752910151, -170.0000000000000000, 64.66187836339484818 ) ) ;
#18753=CARTESIAN_POINT ( 'NONE',  ( -24.09190246691234805, 8.500289797445409690, -95.00000000000133582 ) ) ;
#18754=CARTESIAN_POINT ( 'NONE',  ( 211.9552723536948520, 118.7100180530116518, 92.33883945253931813 ) ) ;
#18756=CARTESIAN_POINT ( 'NONE',  ( -80.54915509118114869, 24.12810583352862182, 57.49897265118980982 ) ) ;
#18760=CARTESIAN_POINT ( 'NONE',  ( 8.679939806240508204, 7.383357464882122301, -13.76982068021760064 ) ) ;
#18765=CARTESIAN_POINT ( 'NONE',  ( 186.7642514597453101, 86.02880938169739977, -65.66567118133815484 ) ) ;
#18766=CARTESIAN_POINT ( 'NONE',  ( -168.1839487819770511, 83.25723186408070831, 43.97232250669951981 ) ) ;
#18767=LINE ( 'NONE', #10182, #25145 ) ;
#18769=CARTESIAN_POINT ( 'NONE',  ( -104.5827168854524558, 33.96561401163044991, 4.021232942600325266 ) ) ;
#18771=CARTESIAN_POINT ( 'NONE',  ( 128.0848616812662897, 38.04676222636084049, -38.70798055224722134 ) ) ;
#18772=ORIENTED_EDGE ( 'NONE', *, *, #66585, .T. ) ;
#18773=ORIENTED_EDGE ( 'NONE', *, *, #19891, .F. ) ;
#18775=CARTESIAN_POINT ( 'NONE',  ( -8.811275908848671179, 6.956777180392053950, 3.320008556540252620 ) ) ;
#18777=CARTESIAN_POINT ( 'NONE',  ( -24.07146903340143140, 8.497560047608729406, -68.19585695038200868 ) ) ;
#18778=CARTESIAN_POINT ( 'NONE',  ( 8.288104306525687193, 6.376394648992964598, 10.18357869276926309 ) ) ;
#18780=CARTESIAN_POINT ( 'NONE',  ( 46.23113030541875190, 10.41513832761375902, -66.85431394756601264 ) ) ;
#18781=CARTESIAN_POINT ( 'NONE',  ( -58.33157376762797242, 16.63098604184965978, -62.81118730508888603 ) ) ;
#18782=CARTESIAN_POINT ( 'NONE',  ( 181.0840389613909736, 78.60582251573005408, -63.06960825634327961 ) ) ;
#18786=CARTESIAN_POINT ( 'NONE',  ( -165.9122696334864600, 79.44688201528255433, 9.386813235023986124 ) ) ;
#18789=CARTESIAN_POINT ( 'NONE',  ( -0.3258398948454879207, 6.518608385615799250, 63.95880355785457994 ) ) ;
#18791=B_SPLINE_CURVE_WITH_KNOTS ( 'NONE', 3,
 ( #37080, #63818, #10340, #4720, #26183, #53238, #26531, #26871, #46949, #69431, #9669, #21248, #42696, #41670, #64154, #48295, #127, #62787, #36052, #57507, #63128, #14929, #60273, #53926, #6096, #43031, #59554, #33894, #21932, #27910, #12435, #836, #32495, #49347, #48641, #55331, #1180, #32838, #59212, #54271, #17717, #484, #12088 ),
 .UNSPECIFIED., .F., .F.,
 ( 4, 2, 2, 2, 2, 2, 2, 2, 2, 2, 2, 2, 1, 2, 2, 2, 2, 2, 2, 2, 2, 4 ),
 ( 0.02358007599568759036, 0.02505677178601666347, 0.02579511968118119308, 0.02653346757634571923, 0.02801016336667479581, 0.02948685915700387239, 0.03022520705216840894, 0.03096355494733294550, 0.03244025073766201861, 0.03391694652799109866, 0.03539364231832017177, 0.03613199021348469098, 0.03687033810864921018, 0.03760868600381372939, 0.03834703389897824860, 0.03982372968930728008, 0.04130042547963631155, 0.04277712126996534303, 0.04351546916512986918, 0.04425381706029438145, 0.04573051285062339905, 0.04720720864095240971 ),
 .UNSPECIFIED. ) ;
#18800=VERTEX_POINT ( 'NONE', #67010 ) ;
#18808=CARTESIAN_POINT ( 'NONE',  ( 151.3136733342017237, 54.26417151662144533, 41.20011332843551344 ) ) ;
#18809=CARTESIAN_POINT ( 'NONE',  ( 8.485361335568063268, -170.0000000000000000, -95.00000000000133582 ) ) ;
#18810=ORIENTED_EDGE ( 'NONE', *, *, #56622, .F. ) ;
#18813=CARTESIAN_POINT ( 'NONE',  ( -1.088326810997879424, 6.545818265928947888, 7.438908920697859806 ) ) ;
#18815=DIRECTION ( 'NONE',  ( -0.000000000000000000, 1.000000000000000000, -0.000000000000000000 ) ) ;
#18816=CARTESIAN_POINT ( 'NONE',  ( 155.1792092232399227, 55.88996826282357233, 83.43110084902221502 ) ) ;
#18817=CARTESIAN_POINT ( 'NONE',  ( 136.9798231265810671, 43.34196232604180210, 3.331182321761577469 ) ) ;
#18819=VERTEX_POINT ( 'NONE', #62049 ) ;
#18821=CARTESIAN_POINT ( 'NONE',  ( 117.6865880453676283, 32.48051379280607165, -44.47768925270803209 ) ) ;
#18822=CARTESIAN_POINT ( 'NONE',  ( -71.97171223898807568, 20.94894057408424359, 14.49148078501619707 ) ) ;
#18823=CARTESIAN_POINT ( 'NONE',  ( 46.64694836521739774, 9.462741877720617367, -45.07469269781585552 ) ) ;
#18825=CYLINDRICAL_SURFACE ( 'NONE', #9623, 7.500000000000020428 ) ;
#18828=EDGE_CURVE ( 'NONE', #47781, #3682, #35328, .T. ) ;
#18830=CARTESIAN_POINT ( 'NONE',  ( -145.9095871962850879, 61.18682730038539574, 71.65010240623834648 ) ) ;
#18834=B_SPLINE_CURVE_WITH_KNOTS ( 'NONE', 3,
 ( #39237, #61030, #54697, #17778, #12500, #54339, #55393, #27621, #17055, #23415 ),
 .UNSPECIFIED., .F., .F.,
 ( 4, 2, 2, 2, 4 ),
 ( 0.000000000000000000, 0.002504193092414286771, 0.005008386184828573541, 0.007512579277242860745, 0.01001677236965714708 ),
 .UNSPECIFIED. ) ;
#18835=CARTESIAN_POINT ( 'NONE',  ( 188.5645326065591689, 86.51153908883284771, -17.49986616938031503 ) ) ;
#18836=CARTESIAN_POINT ( 'NONE',  ( 140.9169160367233360, 45.85398962664667977, -14.09481450478372544 ) ) ;
#18838=CARTESIAN_POINT ( 'NONE',  ( -80.56139928459660382, 24.13290941644248022, -8.510312252193591220 ) ) ;
#18839=CARTESIAN_POINT ( 'NONE',  ( -175.1895962157336726, 90.99110972060685754, -22.58887341897165513 ) ) ;
#18840=CARTESIAN_POINT ( 'NONE',  ( -48.23766733091051861, 13.99378332280059034, 40.95827912834796081 ) ) ;
#18848=CARTESIAN_POINT ( 'NONE',  ( -189.3111515777349894, 107.1887855376296983, 66.35551062646212017 ) ) ;
#18852=CARTESIAN_POINT ( 'NONE',  ( 186.6054783416232397, 84.37128553200975034, -48.82557464685664428 ) ) ;
#18854=CARTESIAN_POINT ( 'NONE',  ( -24.19091603582230832, 8.513464105188679909, -40.87426144925215965 ) ) ;
#18861=CARTESIAN_POINT ( 'NONE',  ( -71.26082837647275880, 19.63751494688351684, 92.83733660865655679 ) ) ;
#18862=CARTESIAN_POINT ( 'NONE',  ( -81.23297981660238065, 23.31577157498399089, 71.81404419543271445 ) ) ;
#18863=CARTESIAN_POINT ( 'NONE',  ( 68.61679388097590504, 14.04192738700837140, -48.21445178305530987 ) ) ;
#18865=CARTESIAN_POINT ( 'NONE',  ( -60.47589866267035319, 17.25153113855766307, 32.63091271826195339 ) ) ;
#18867=CARTESIAN_POINT ( 'NONE',  ( 59.94652978725886783, 13.01168383647461901, 44.16053422060780065 ) ) ;
#18868=CARTESIAN_POINT ( 'NONE',  ( 32.56653645198905878, 7.618633747641397669, 87.99861145309087362 ) ) ;
#18871=CARTESIAN_POINT ( 'NONE',  ( -1.319107422865894774, 6.554467368239797587, -46.68092456214186114 ) ) ;
#18873=CARTESIAN_POINT ( 'NONE',  ( -190.4968431727838833, 108.8425311198514862, -46.28873902368739124 ) ) ;
#18874=CARTESIAN_POINT ( 'NONE',  ( 133.3996297101684547, 41.14871796345730104, -9.178760341931967659 ) ) ;
#18876=DIRECTION ( 'NONE',  ( -0.000000000000000000, 1.000000000000000000, -0.000000000000000000 ) ) ;
#18877=CARTESIAN_POINT ( 'NONE',  ( 129.4887940973039804, 40.01039828304092794, -10.56306520635085988 ) ) ;
#18881=CARTESIAN_POINT ( 'NONE',  ( -33.83721310978700814, 11.01869210665941878, -49.92765374023623082 ) ) ;
#18882=FACE_OUTER_BOUND ( 'NONE', #42007, .T. ) ;
#18883=CARTESIAN_POINT ( 'NONE',  ( -176.6810441562621747, 91.17854316950446503, 85.38946104415586547 ) ) ;
#18887=CARTESIAN_POINT ( 'NONE',  ( -149.0732005398557760, 63.81212100765654327, -7.977722101697186652 ) ) ;
#18892=CARTESIAN_POINT ( 'NONE',  ( 164.0474223553472370, 64.26366484389406253, 86.97719845451288734 ) ) ;
#18894=CARTESIAN_POINT ( 'NONE',  ( -62.06231780744543869, 17.72446026058426227, 13.65205514321663394 ) ) ;
#18898=CARTESIAN_POINT ( 'NONE',  ( -190.6985136298601731, 109.1272424661242582, 94.99999999999866418 ) ) ;
#18904=CARTESIAN_POINT ( 'NONE',  ( 62.04326772936978784, 12.44884401098615534, 29.86050463841740665 ) ) ;
#18906=EDGE_LOOP ( 'NONE', ( #10211, #32487, #59363, #57100 ) ) ;
#18907=ADVANCED_FACE ( 'NONE', ( #25818 ), #15935, .F. ) ;
#18909=CARTESIAN_POINT ( 'NONE',  ( -167.4860113959264822, 82.52233889531183308, 16.43299606317020078 ) ) ;
#18910=CARTESIAN_POINT ( 'NONE',  ( 19.11168290073779730, 6.629794975642855803, -63.13554536250090621 ) ) ;
#18912=CARTESIAN_POINT ( 'NONE',  ( -128.1282195935087884, 49.19720162550163423, 57.80142861109457186 ) ) ;
#18914=DIRECTION ( 'NONE',  ( -0.000000000000000000, 1.000000000000000000, -0.000000000000000000 ) ) ;
#18915=CARTESIAN_POINT ( 'NONE',  ( -25.80443741485380471, 9.749985135376009637, 42.69045884007576319 ) ) ;
#18918=CARTESIAN_POINT ( 'NONE',  ( 207.8398359204632868, 112.5208221429021336, -77.48374306908839060 ) ) ;
#18921=CARTESIAN_POINT ( 'NONE',  ( -133.3923804760465543, 52.87100816290226390, 10.70811376284584426 ) ) ;
#18923=ORIENTED_EDGE ( 'NONE', *, *, #48178, .T. ) ;
#18925=CARTESIAN_POINT ( 'NONE',  ( -146.5230751932348880, 62.99205605665031271, -22.36346160708336228 ) ) ;
#18932=CARTESIAN_POINT ( 'NONE',  ( -142.9728934044261734, 58.82891228489260982, 34.50119712044075015 ) ) ;
#18934=CARTESIAN_POINT ( 'NONE',  ( -171.0758681675583830, 84.87997360100516175, -61.82834634754290448 ) ) ;
#18936=CARTESIAN_POINT ( 'NONE',  ( -103.2061297292849531, 34.38496953192503014, 30.56187840025431512 ) ) ;
#18938=CARTESIAN_POINT ( 'NONE',  ( 35.65775178405257151, 7.951994368745591402, 30.91065945747581267 ) ) ;
#18939=CARTESIAN_POINT ( 'NONE',  ( 85.68197636629479064, 20.16141071296262766, 56.60131216792452591 ) ) ;
#18940=VERTEX_POINT ( 'NONE', #5034 ) ;
#18941=CARTESIAN_POINT ( 'NONE',  ( 186.2722199822850655, 84.01218714714249813, 42.24469577624778083 ) ) ;
#18942=CARTESIAN_POINT ( 'NONE',  ( -189.4223925288096098, 107.3427006758676185, -67.23478617198331619 ) ) ;
#18947=CARTESIAN_POINT ( 'NONE',  ( -14.56631729561072142, 8.434645566888205437, -39.59350022180603901 ) ) ;
#18951=CARTESIAN_POINT ( 'NONE',  ( -108.0942684325822825, 35.83382830275052555, -91.46080949164959861 ) ) ;
#18952=ORIENTED_EDGE ( 'NONE', *, *, #20397, .F. ) ;
#18954=CARTESIAN_POINT ( 'NONE',  ( -59.96408504033279740, 17.10126854471815605, 70.35115488651923954 ) ) ;
#18958=CARTESIAN_POINT ( 'NONE',  ( 150.2805372522807090, 53.51147386362153213, -68.31707538700877080 ) ) ;
#18959=CARTESIAN_POINT ( 'NONE',  ( -95.88718821240200896, 29.65015105908826243, -19.60004368519706475 ) ) ;
#18960=CARTESIAN_POINT ( 'NONE',  ( 134.3159642998340075, 41.70198410084975649, -51.02331093239570947 ) ) ;
#18963=DIRECTION ( 'NONE',  ( -0.000000000000000000, 1.000000000000000000, -0.000000000000000000 ) ) ;
#18964=CARTESIAN_POINT ( 'NONE',  ( -118.7011677090247588, 41.93687969120207981, 35.97862495719843423 ) ) ;
#18965=CARTESIAN_POINT ( 'NONE',  ( -56.02027488966931656, 14.94257193099085512, -35.26346284988749602 ) ) ;
#18966=ORIENTED_EDGE ( 'NONE', *, *, #45649, .T. ) ;
#18967=CARTESIAN_POINT ( 'NONE',  ( -173.5372686962700755, 89.10569330281728639, -76.55650775521371543 ) ) ;
#18968=CARTESIAN_POINT ( 'NONE',  ( 131.7631832018459761, 41.34383094671487413, 83.49070356861206221 ) ) ;
#18969=B_SPLINE_CURVE_WITH_KNOTS ( 'NONE', 3,
 ( #39307, #55833, #33342, #50550, #55472, #60408, #65697, #18196, #49133, #38603, #54769, #50203, #32978, #66056, #22424, #6597, #12226, #33690, #22770, #2369, #44213, #44578, #23825, #39650, #66750, #12929, #2029, #17488, #55120, #23484, #61107, #6942, #34390, #11504, #17850, #6240, #28393, #49838, #60751, #27693, #1665, #43863, #12571 ),
 .UNSPECIFIED., .F., .F.,
 ( 4, 2, 2, 2, 2, 2, 2, 2, 1, 2, 2, 2, 2, 2, 2, 2, 2, 2, 2, 2, 2, 4 ),
 ( 1.734723475976807094E-18, 0.001466540241398116458, 0.002199810362097173819, 0.002933080482796231181, 0.004399620724194333761, 0.005866160965592434606, 0.007332701206990535452, 0.008065971327689585441, 0.008799241448388634562, 0.009532511569087683684, 0.01026578168978673281, 0.01173232193118487442, 0.01319886217258301256, 0.01466540241398115590, 0.01539867253468024319, 0.01613194265537933048, 0.01759848289677747729, 0.01906502313817561717, 0.01979829325887470098, 0.02053156337957378480, 0.02199810362097197325, 0.02346464386237015476 ),
 .UNSPECIFIED. ) ;
#18970=CARTESIAN_POINT ( 'NONE',  ( 200.4590013143046576, 102.3556155835302945, -23.18599784113892781 ) ) ;
#18975=CARTESIAN_POINT ( 'NONE',  ( 164.0298848570286339, 62.93631132702878972, -13.10447936278614023 ) ) ;
#18976=CARTESIAN_POINT ( 'NONE',  ( 114.4640969196986191, 30.88424258798503530, -76.47100256968519716 ) ) ;
#18978=CARTESIAN_POINT ( 'NONE',  ( 187.1594815608683859, 84.97172738281348359, -93.01128905854854168 ) ) ;
#18982=CARTESIAN_POINT ( 'NONE',  ( 162.6205203824432317, 63.07332653227190633, -11.32221202892962708 ) ) ;
#18985=CARTESIAN_POINT ( 'NONE',  ( 126.3481178384318611, 37.07182590705851055, 90.63207038995997777 ) ) ;
#18986=EDGE_CURVE ( 'NONE', #38218, #55323, #36361, .T. ) ;
#18989=EDGE_CURVE ( 'NONE', #34631, #37469, #12237, .T. ) ;
#18991=CARTESIAN_POINT ( 'NONE',  ( -142.0062637385109952, 58.06920992247430746, -68.60690856511718039 ) ) ;
#18994=CARTESIAN_POINT ( 'NONE',  ( 163.1265310614427051, 62.18610413911356005, -48.55550286496519163 ) ) ;
#18995=ORIENTED_EDGE ( 'NONE', *, *, #66585, .F. ) ;
#18996=CARTESIAN_POINT ( 'NONE',  ( -94.78138776532236420, 30.24234841992712930, 11.71057004227387210 ) ) ;
#18997=CARTESIAN_POINT ( 'NONE',  ( 56.83393674870969647, 12.35044717442195150, 86.74189108956782945 ) ) ;
#18999=CARTESIAN_POINT ( 'NONE',  ( 85.67165909753197184, 20.15791549876372812, -9.022809353226582729 ) ) ;
#19002=CARTESIAN_POINT ( 'NONE',  ( 133.3990214534116205, 41.14886683286416513, -77.85737058891160700 ) ) ;
#19003=VERTEX_POINT ( 'NONE', #27173 ) ;
#19005=CARTESIAN_POINT ( 'NONE',  ( 204.6977192012829789, -170.0000000000000000, 36.70772073876943153 ) ) ;
#19008=CARTESIAN_POINT ( 'NONE',  ( -151.2511071212631464, 67.00426547928867649, -35.00508260455636389 ) ) ;
#19010=CARTESIAN_POINT ( 'NONE',  ( -35.17296606710973350, 11.25626711331309693, 31.19335591454689194 ) ) ;
#19011=CARTESIAN_POINT ( 'NONE',  ( -154.7934364910360330, 68.79594655117531943, -63.83113484831022788 ) ) ;
#19015=CARTESIAN_POINT ( 'NONE',  ( 206.2980740120524388, 108.5619562183280067, -51.16432913298972807 ) ) ;
#19016=CARTESIAN_POINT ( 'NONE',  ( 177.0075766083211590, 74.58167636505949361, 3.664334904826073824 ) ) ;
#19017=CARTESIAN_POINT ( 'NONE',  ( -61.75629144857965258, 16.58190704077738076, 14.34543443704044741 ) ) ;
#19018=EDGE_LOOP ( 'NONE', ( #60676, #40985, #10437, #34355 ) ) ;
#19019=CARTESIAN_POINT ( 'NONE',  ( -96.77705718164445159, 31.18700926299573695, -37.39494439648063917 ) ) ;
#19021=CARTESIAN_POINT ( 'NONE',  ( 107.0477776024378613, 27.43148174916616000, -77.05657040992022644 ) ) ;
#19023=CARTESIAN_POINT ( 'NONE',  ( 42.70988075781783522, 8.862408058333489436, 57.50971735983328870 ) ) ;
#19025=CARTESIAN_POINT ( 'NONE',  ( -5.586713254917526683, 6.755371726299415513, 84.13907536519101882 ) ) ;
#19026=CARTESIAN_POINT ( 'NONE',  ( -102.2801239173131194, 33.91021738430207222, -23.17002667451225406 ) ) ;
#19027=CARTESIAN_POINT ( 'NONE',  ( 59.84413847313641810, 12.98802251483526149, -90.06398035839559668 ) ) ;
#19028=CARTESIAN_POINT ( 'NONE',  ( -166.5704851812740230, 80.12110537694668722, 61.50361147337653023 ) ) ;
#19033=CARTESIAN_POINT ( 'NONE',  ( 178.4027079424739100, 75.93756746109791322, -9.872868637179553986 ) ) ;
#19034=CARTESIAN_POINT ( 'NONE',  ( 109.3154830994003390, 29.56170298203815960, 56.49859460758455754 ) ) ;
#19037=CARTESIAN_POINT ( 'NONE',  ( 60.63380853769236722, 13.16344960520421559, -23.49203963615685353 ) ) ;
#19038=ORIENTED_EDGE ( 'NONE', *, *, #21832, .T. ) ;
#19042=CARTESIAN_POINT ( 'NONE',  ( 23.03546163277112413, 7.848986635155161373, -41.07252390632271499 ) ) ;
#19043=CARTESIAN_POINT ( 'NONE',  ( -149.5074843970971017, 65.50121172469319220, 45.72082123989907387 ) ) ;
#19045=CARTESIAN_POINT ( 'NONE',  ( -125.8938041572051389, 47.69968343338778283, 30.61994787315706290 ) ) ;
#19048=EDGE_CURVE ( 'NONE', #41326, #44052, #11691, .T. ) ;
#19052=CARTESIAN_POINT ( 'NONE',  ( 91.12448333640237763, 22.07449368110503229, -49.34459205181515529 ) ) ;
#19054=CARTESIAN_POINT ( 'NONE',  ( -173.5422248620772905, 89.11126078969415687, 18.97714401617738034 ) ) ;
#19055=CARTESIAN_POINT ( 'NONE',  ( 10.00452960006446723, 6.384031490329864056, 86.38374501823878404 ) ) ;
#19057=CARTESIAN_POINT ( 'NONE',  ( 79.19132716134490124, 17.01584750883626995, -71.16104780385437323 ) ) ;
#19060=CARTESIAN_POINT ( 'NONE',  ( 197.5344433744249102, 98.61756151884684130, -41.58120981647593339 ) ) ;
#19063=EDGE_LOOP ( 'NONE', ( #29850, #41287, #48970, #1716 ) ) ;
#19064=CARTESIAN_POINT ( 'NONE',  ( -82.32750425780474757, 23.74963782027935721, -62.89668749667942649 ) ) ;
#19065=DIRECTION ( 'NONE',  ( 0.000000000000000000, 0.000000000000000000, 1.000000000000000000 ) ) ;
#19068=ORIENTED_EDGE ( 'NONE', *, *, #8491, .F. ) ;
#19071=CARTESIAN_POINT ( 'NONE',  ( 12.46277766093406214, 6.416700641561361884, -36.27856315466706860 ) ) ;
#19074=CARTESIAN_POINT ( 'NONE',  ( 22.29513692215317988, 6.796052026456516515, 6.908320987580739647 ) ) ;
#19075=ORIENTED_EDGE ( 'NONE', *, *, #33754, .T. ) ;
#19076=CARTESIAN_POINT ( 'NONE',  ( -78.66644367742111399, 23.39876645725285798, -8.270900041254197532 ) ) ;
#19077=CARTESIAN_POINT ( 'NONE',  ( 175.8947993867356843, 74.90689716047906188, -76.00546110050024140 ) ) ;
#19079=CARTESIAN_POINT ( 'NONE',  ( 110.2429982417149432, 28.88204397445231564, -9.077886975189997543 ) ) ;
#19080=CARTESIAN_POINT ( 'NONE',  ( 82.12277968641507186, 18.98848723477813039, -37.30662462622972697 ) ) ;
#19081=DIRECTION ( 'NONE',  ( 0.000000000000000000, 0.000000000000000000, 1.000000000000000000 ) ) ;
#19082=EDGE_LOOP ( 'NONE', ( #22472, #14411 ) ) ;
#19083=VECTOR ( 'NONE', #68960, 1000.000000000000000 ) ;
#19086=CYLINDRICAL_SURFACE ( 'NONE', #61889, 7.500000000000020428 ) ;
#19089=CARTESIAN_POINT ( 'NONE',  ( 198.3926538463958593, 98.07933330386025261, 13.96394819647072794 ) ) ;
#19091=CARTESIAN_POINT ( 'NONE',  ( 211.7299983131283057, 118.3604252729061130, 87.78175077331377452 ) ) ;
#19092=CARTESIAN_POINT ( 'NONE',  ( 209.6698611676812050, 115.2210955123518659, 42.34078908743409642 ) ) ;
#19094=CARTESIAN_POINT ( 'NONE',  ( -12.39413342787891104, 7.231444436041488899, 43.58353802562231039 ) ) ;
#19096=CARTESIAN_POINT ( 'NONE',  ( 10.15118267943872077, 7.391905976536036427, -21.12758222051168033 ) ) ;
#19098=CARTESIAN_POINT ( 'NONE',  ( 198.2545923567585646, 97.90679023593575891, -20.83074425647854611 ) ) ;
#19100=CARTESIAN_POINT ( 'NONE',  ( -147.1538409485623333, 63.51600817366542628, 4.251635946998408855 ) ) ;
#19101=CARTESIAN_POINT ( 'NONE',  ( 185.5412249395996014, 84.70425786166002524, -76.60579427066070934 ) ) ;
#19102=CARTESIAN_POINT ( 'NONE',  ( -166.9992034932274976, 82.01285191063134050, 42.68440912882079630 ) ) ;
#19104=CARTESIAN_POINT ( 'NONE',  ( -100.4262673593280368, 31.84860241619273680, -35.23214805985528386 ) ) ;
#19105=CARTESIAN_POINT ( 'NONE',  ( 31.91375106836930087, 7.553354707452893280, -43.60781062558567811 ) ) ;
#19107=CARTESIAN_POINT ( 'NONE',  ( 12.46490660984524723, 7.423426948220649635, -36.29097311990165053 ) ) ;
#19108=CARTESIAN_POINT ( 'NONE',  ( 131.6005058089755551, 40.07838125795768036, -50.69123583781497189 ) ) ;
#19111=CARTESIAN_POINT ( 'NONE',  ( 186.9531721782180966, 86.23502673300468757, 85.81665300944044361 ) ) ;
#19112=CARTESIAN_POINT ( 'NONE',  ( -15.32550079334879278, 7.496023944924839810, 10.52911393437325849 ) ) ;
#19116=CARTESIAN_POINT ( 'NONE',  ( 9.416656162223555171, 6.380306691996769253, 14.63415394072566400 ) ) ;
#19119=CARTESIAN_POINT ( 'NONE',  ( 39.88975917505626967, 9.487965272711658571, -77.46436805589148378 ) ) ;
#19121=CARTESIAN_POINT ( 'NONE',  ( 198.8752826725510658, 100.3130050945023157, -75.40481520914208602 ) ) ;
#19123=CARTESIAN_POINT ( 'NONE',  ( -180.2252811616041583, 95.40045830523430936, -39.79017893922387117 ) ) ;
#19124=CARTESIAN_POINT ( 'NONE',  ( 107.0477776024379040, 27.43148174916616355, 3.477081361470783616 ) ) ;
#19125=CARTESIAN_POINT ( 'NONE',  ( -170.2747214445850261, 84.01465441107043830, 18.42892912042381326 ) ) ;
#19127=CARTESIAN_POINT ( 'NONE',  ( -51.34325167237332721, 13.71819364263220997, 71.18482817347160108 ) ) ;
#19130=CARTESIAN_POINT ( 'NONE',  ( -2.190131154568196514, 6.589492063460817839, 59.50486936982123609 ) ) ;
#19134=CARTESIAN_POINT ( 'NONE',  ( -129.4098618459771899, 48.85263848239745954, -75.88708462038850655 ) ) ;
#19135=CARTESIAN_POINT ( 'NONE',  ( -109.7079446832839267, 37.86719386855317282, -70.42946416363754736 ) ) ;
#19136=CARTESIAN_POINT ( 'NONE',  ( -49.43915770973590895, 13.24768844696976089, -37.71853435192636539 ) ) ;
#19146=CARTESIAN_POINT ( 'NONE',  ( 150.5744176759382924, 53.72473166688034496, 33.94873877333132839 ) ) ;
#19151=CARTESIAN_POINT ( 'NONE',  ( -179.5082312244189495, 94.53075638132055758, 7.537094676919972258 ) ) ;
#19152=DIRECTION ( 'NONE',  ( 0.000000000000000000, -1.000000000000000000, 0.000000000000000000 ) ) ;
#19155=CARTESIAN_POINT ( 'NONE',  ( -85.89078989036970313, 26.29712602777647845, 35.88770218881549567 ) ) ;
#19156=CARTESIAN_POINT ( 'NONE',  ( 150.0625426684546255, 52.11349418987130377, 89.36692820587143160 ) ) ;
#19157=CARTESIAN_POINT ( 'NONE',  ( 140.1999945597798671, 45.38880890490929687, 6.156068824733499589 ) ) ;
#19160=CARTESIAN_POINT ( 'NONE',  ( 13.14401442664831166, 6.430459733718342008, 71.38195679730273469 ) ) ;
#19161=CARTESIAN_POINT ( 'NONE',  ( 45.90693067088656676, 9.344800815249319825, -39.35472096678888931 ) ) ;
#19162=CARTESIAN_POINT ( 'NONE',  ( -72.73902111355396016, 21.21842696158244479, 87.00106551046614811 ) ) ;
#19164=VERTEX_POINT ( 'NONE', #24354 ) ;
#19165=CARTESIAN_POINT ( 'NONE',  ( 86.15410276028860892, 19.25894675708890702, -50.82156419891174437 ) ) ;
#19167=ORIENTED_EDGE ( 'NONE', *, *, #38766, .F. ) ;
#19171=CARTESIAN_POINT ( 'NONE',  ( 181.0840389613909736, 78.60582251573003987, -9.380507075415925655 ) ) ;
#19173=CARTESIAN_POINT ( 'NONE',  ( -85.75002235020438945, 26.23806300442548434, -13.29363553231531903 ) ) ;
#19174=CARTESIAN_POINT ( 'NONE',  ( -180.3161328724957855, 97.10341277064810583, -13.22867699537820663 ) ) ;
#19179=CARTESIAN_POINT ( 'NONE',  ( 103.4696172145934554, 25.87254488218942328, 67.18619957088650096 ) ) ;
#19184=CARTESIAN_POINT ( 'NONE',  ( 17.48889770758266948, 6.561062909825354339, 30.20590664838920603 ) ) ;
#19185=CARTESIAN_POINT ( 'NONE',  ( -142.0103255789723846, 59.35140309638574507, 92.31801490858313741 ) ) ;
#19189=DIRECTION ( 'NONE',  ( -0.000000000000000000, 1.000000000000000000, -0.000000000000000000 ) ) ;
#19190=CARTESIAN_POINT ( 'NONE',  ( -82.53770812813169755, 23.83403279300014788, 58.33458210178376646 ) ) ;
#19191=CARTESIAN_POINT ( 'NONE',  ( 70.45466089417030275, 14.52203022703029944, -42.23427169726421937 ) ) ;
#19193=CARTESIAN_POINT ( 'NONE',  ( -58.97243502469717669, 16.81420332340174895, 44.21623767979525610 ) ) ;
#19195=CARTESIAN_POINT ( 'NONE',  ( -37.05762690088739930, 11.60527003175538852, -74.63595191190708533 ) ) ;
#19196=CARTESIAN_POINT ( 'NONE',  ( 33.76124497394584267, 7.742545529019362327, 69.22549252300315459 ) ) ;
#19197=CARTESIAN_POINT ( 'NONE',  ( 42.00028371212653866, 8.760846226116838054, 84.03640436414383430 ) ) ;
#19200=CARTESIAN_POINT ( 'NONE',  ( -0.3747453031323924044, 6.520267647591905025, -43.90647717188161181 ) ) ;
#19202=CARTESIAN_POINT ( 'NONE',  ( -120.1259246007803370, 42.81147313035990010, 16.09632390948472391 ) ) ;
#19204=CARTESIAN_POINT ( 'NONE',  ( 126.4083787442699958, 37.10531539900949838, -17.70407539275910480 ) ) ;
#19205=CARTESIAN_POINT ( 'NONE',  ( 18.88468164817598449, 7.626722602998417422, -23.00979687325194334 ) ) ;
#19208=EDGE_CURVE ( 'NONE', #53253, #9716, #30674, .T. ) ;
#19214=CARTESIAN_POINT ( 'NONE',  ( 127.2358066117906787, 38.72257733469225371, -47.08406076428676812 ) ) ;
#19219=ORIENTED_EDGE ( 'NONE', *, *, #65, .T. ) ;
#19223=CARTESIAN_POINT ( 'NONE',  ( 152.6935468464033079, 55.28251231414122913, 84.80687879366244886 ) ) ;
#19226=CARTESIAN_POINT ( 'NONE',  ( 132.0563630623057065, 41.51825634609597415, -77.65224337536834298 ) ) ;
#19229=EDGE_CURVE ( 'NONE', #32664, #16864, #17196, .T. ) ;
#19235=B_SPLINE_CURVE_WITH_KNOTS ( 'NONE', 3,
 ( #68111, #36432, #5105, #36785, #19917, #26565, #47660, #41373, #9021, #58228, #41021, #10043, #31500, #62476, #14293, #52933, #69114, #4421, #20940, #42396, #10374, #63858, #25886, #46984, #30464, #31172, #58557, #4084, #62826, #51916, #3723, #14629, #57548, #9352, #68444, #20250, #63172, #57886, #9705, #22324, #49033, #38148, #58906, #59588, #11404 ),
 .UNSPECIFIED., .F., .F.,
 ( 4, 2, 2, 1, 2, 2, 2, 2, 2, 2, 2, 2, 2, 2, 2, 2, 2, 2, 2, 2, 2, 2, 4 ),
 ( 0.02346057189573570387, 0.02492590417315496132, 0.02565857031186458831, 0.02639123645057421877, 0.02712390258928384923, 0.02785656872799347622, 0.02932190100541273367, 0.03005456714412236413, 0.03078723328283199112, 0.03225256556025124510, 0.03298523169896087903, 0.03371789783767050602, 0.03518323011508976000, 0.03664856239250902092, 0.03738122853121864098, 0.03811389466992827491, 0.03957922694734752889, 0.04104455922476678287, 0.04250989150218603685, 0.04324255764089565690, 0.04397522377960528389, 0.04544055605702453093, 0.04690588833444377798 ),
 .UNSPECIFIED. ) ;
#19236=CARTESIAN_POINT ( 'NONE',  ( -2.487553394779416394, 7.609150130527738476, -91.32180055539627972 ) ) ;
#19237=EDGE_LOOP ( 'NONE', ( #16625, #3551, #33054, #29358 ) ) ;
#19238=ORIENTED_EDGE ( 'NONE', *, *, #19682, .T. ) ;
#19239=CARTESIAN_POINT ( 'NONE',  ( -165.6404838346739155, 80.60836113891892296, 12.09496305903157243 ) ) ;
#19241=CARTESIAN_POINT ( 'NONE',  ( 22.81270948571149049, 6.827178363529885274, -67.22380911626287059 ) ) ;
#19242=CARTESIAN_POINT ( 'NONE',  ( -133.0921934900200085, 52.65587531157186163, 67.08693232277423135 ) ) ;
#19244=CARTESIAN_POINT ( 'NONE',  ( -98.60532234565044973, 32.07256199879358149, 85.16297041932693901 ) ) ;
#19249=CARTESIAN_POINT ( 'NONE',  ( 175.8200436508851965, 74.83544132389157255, -92.05719928250275075 ) ) ;
#19250=AXIS2_PLACEMENT_3D ( 'NONE', #10583, #59808, #64756 ) ;
#19252=CARTESIAN_POINT ( 'NONE',  ( 138.5943620234099569, 45.55242290395138127, 31.17580979822920639 ) ) ;
#19253=CARTESIAN_POINT ( 'NONE',  ( 111.1865443042262029, 30.43181341527239070, 29.65596660664464679 ) ) ;
#19257=VERTEX_POINT ( 'NONE', #65797 ) ;
#19262=CARTESIAN_POINT ( 'NONE',  ( -51.56239267699974960, 13.77339621164778727, -89.76365528998427123 ) ) ;
#19263=CARTESIAN_POINT ( 'NONE',  ( -47.89046518825391985, 13.91124031206838296, -94.13781639831633186 ) ) ;
#19264=EDGE_CURVE ( 'NONE', #59320, #68287, #8878, .T. ) ;
#19266=CARTESIAN_POINT ( 'NONE',  ( 70.51522979775972999, 15.57935281015687146, -42.71848339722297538 ) ) ;
#19267=CARTESIAN_POINT ( 'NONE',  ( -118.3918229753714968, 42.92682904595255877, 37.61031292237963441 ) ) ;
#19268=CARTESIAN_POINT ( 'NONE',  ( 207.4696221732442325, 110.2206209205162111, 56.57135469275507234 ) ) ;
#19269=ORIENTED_EDGE ( 'NONE', *, *, #56681, .T. ) ;
#19272=ADVANCED_FACE ( 'NONE', ( #42914 ), #59444, .F. ) ;
#19273=CARTESIAN_POINT ( 'NONE',  ( 79.62991792432430316, 18.20325130265939251, -94.18765078435455962 ) ) ;
#19274=DIRECTION ( 'NONE',  ( 0.000000000000000000, 0.000000000000000000, 1.000000000000000000 ) ) ;
#19276=DIRECTION ( 'NONE',  ( -0.8160245890732938934, -0.5780171883497599028, 0.000000000000000000 ) ) ;
#19280=CARTESIAN_POINT ( 'NONE',  ( 36.09137906183515554, 8.001963043161770983, 3.835010927944524362 ) ) ;
#19281=CARTESIAN_POINT ( 'NONE',  ( -7.825402957745085430, 7.899365992529248537, -35.41807073194381417 ) ) ;
#19286=CARTESIAN_POINT ( 'NONE',  ( -60.97727891098336528, 16.35024395194893287, 33.19213824417288095 ) ) ;
#19292=CARTESIAN_POINT ( 'NONE',  ( -14.55425570676089286, 7.423011834016143951, -66.44103785447590838 ) ) ;
#19293=CARTESIAN_POINT ( 'NONE',  ( -35.99432170610150195, 10.38324794858010414, 31.73840043048652149 ) ) ;
#19295=CARTESIAN_POINT ( 'NONE',  ( 138.2204650371259333, 44.12203217345472694, -37.40497479428969285 ) ) ;
#19298=ADVANCED_FACE ( 'NONE', ( #9731 ), #57912, .F. ) ;
#19299=CARTESIAN_POINT ( 'NONE',  ( -155.5977325361978387, 70.88311713755702215, 69.44969795258840861 ) ) ;
#19301=CARTESIAN_POINT ( 'NONE',  ( 162.0862735437575566, 62.63196145447164298, 57.82334402139706953 ) ) ;
#19303=CARTESIAN_POINT ( 'NONE',  ( -180.3114074031036580, 97.09758726817788954, -71.21099496842563781 ) ) ;
#19305=CARTESIAN_POINT ( 'NONE',  ( 126.3749122082473377, 38.23888021981338170, 91.33587154719414514 ) ) ;
#19307=CARTESIAN_POINT ( 'NONE',  ( 204.0485454264722023, 107.1608795776555922, -90.03598187893172167 ) ) ;
#19315=CARTESIAN_POINT ( 'NONE',  ( 199.7278513351970162, 99.76879341361765796, 42.34380694319595761 ) ) ;
#19316=CARTESIAN_POINT ( 'NONE',  ( 116.9200705848630264, 32.09536795999727588, -66.81303021653259577 ) ) ;
#19318=CARTESIAN_POINT ( 'NONE',  ( 138.2136629441928903, 45.30947856186672595, 4.042827492293223024 ) ) ;
#19325=CARTESIAN_POINT ( 'NONE',  ( 161.1112535418156426, 61.83422628788724751, -10.21864072077471874 ) ) ;
#19328=CARTESIAN_POINT ( 'NONE',  ( 140.1990463068371469, 45.38811834026235204, 94.71732886340767266 ) ) ;
#19330=EDGE_LOOP ( 'NONE', ( #31956, #65786 ) ) ;
#19331=CARTESIAN_POINT ( 'NONE',  ( 164.9547823171480161, 65.03046442419432083, -44.18386578002282761 ) ) ;
#19333=CARTESIAN_POINT ( 'NONE',  ( 159.6593397521790507, 59.37286298965128140, -50.81150672396304913 ) ) ;
#19336=CARTESIAN_POINT ( 'NONE',  ( -126.8005235842505840, 47.09307471149450919, 45.57853283965476265 ) ) ;
#19337=B_SPLINE_CURVE_WITH_KNOTS ( 'NONE', 3,
 ( #22723, #1615, #55069, #7246, #28706, #40628, #67048, #3693, #51202, #51880, #29390, #52227, #68080, #56829, #62791, #2664, #18840, #56465, #67729, #19881, #3015, #25169, #29738, #24478, #50846, #24125, #39947, #14596, #45568, #61738, #30431, #41338, #40295, #36057, #57511, #9321, #19528, #40984, #45917, #30782, #35719, #62088, #67386, #62446 ),
 .UNSPECIFIED., .F., .F.,
 ( 4, 2, 2, 2, 2, 2, 2, 2, 2, 2, 2, 2, 2, 2, 2, 2, 2, 2, 2, 2, 2, 4 ),
 ( 0.000000000000000000, 0.001488594467279753288, 0.002232891700919617355, 0.002977188934559481422, 0.004465783401839182667, 0.005954377869118883913, 0.007442972336398583424, 0.008187269570038440553, 0.008931566803678297681, 0.01042016127095802928, 0.01190875573823776089, 0.01265305297187762842, 0.01339735020551749423, 0.01488594467279723971, 0.01563024190643711592, 0.01637453914007698866, 0.01786313360735673761, 0.01935172807463648656, 0.02009602530827635236, 0.02084032254191621816, 0.02232891700919592895, 0.02381751147647563974 ),
 .UNSPECIFIED. ) ;
#19338=CARTESIAN_POINT ( 'NONE',  ( 150.3360255159550150, 53.55172128635252449, -95.00000000000133582 ) ) ;
#19339=CARTESIAN_POINT ( 'NONE',  ( 79.19119222799091062, 18.06817527909836230, -15.48292693387985608 ) ) ;
#19341=CARTESIAN_POINT ( 'NONE',  ( -34.06864996337441909, 10.03773626259441798, -62.63357253091302113 ) ) ;
#19345=CARTESIAN_POINT ( 'NONE',  ( -94.78138776532239262, 30.24234841992714351, 65.39967122320125270 ) ) ;
#19346=CARTESIAN_POINT ( 'NONE',  ( -10.23531775138760835, 8.068923942586303966, 57.35362084251622150 ) ) ;
#19349=CARTESIAN_POINT ( 'NONE',  ( 155.7167524447090727, 57.56687707799950715, -9.474077844157728023 ) ) ;
#19351=CARTESIAN_POINT ( 'NONE',  ( 109.7782172510783596, 29.77507867835875288, 29.61121420573730845 ) ) ;
#19353=CARTESIAN_POINT ( 'NONE',  ( -7.825402957745081878, 7.899365992529270741, 30.11558103944718923 ) ) ;
#19356=CARTESIAN_POINT ( 'NONE',  ( 157.4703587214989113, 57.65129005721576050, 71.25401806271709404 ) ) ;
#19357=CARTESIAN_POINT ( 'NONE',  ( 175.8963338753313792, 73.51705463274393537, 15.38615084967059410 ) ) ;
#19358=CARTESIAN_POINT ( 'NONE',  ( -58.76005811686688673, 15.70653557534867595, 17.51043486912802649 ) ) ;
#19364=CARTESIAN_POINT ( 'NONE',  ( 46.90208227351340753, 10.52324439420451085, -16.51717632370492339 ) ) ;
#19365=CARTESIAN_POINT ( 'NONE',  ( 40.37438610703017616, 8.537526699166106070, 56.80551099547096072 ) ) ;
#19367=CARTESIAN_POINT ( 'NONE',  ( -1.700272545523339840, 6.569435498413836783, 86.96418197045451848 ) ) ;
#19368=CARTESIAN_POINT ( 'NONE',  ( -109.6752351740181979, 37.84903014964774570, -14.39328408723732800 ) ) ;
#19370=CARTESIAN_POINT ( 'NONE',  ( 23.09119322872580682, -170.0000000000000000, -95.00000000000133582 ) ) ;
#19371=CARTESIAN_POINT ( 'NONE',  ( -165.7143741370937278, 79.24519349471961505, 63.94847269051136607 ) ) ;
#19377=CARTESIAN_POINT ( 'NONE',  ( 173.7246046907419554, 71.47482343504563573, -15.40631472208198005 ) ) ;
#19378=CARTESIAN_POINT ( 'NONE',  ( 106.4072861358878157, 28.24787347451998087, 70.40525499941243481 ) ) ;
#19379=DIRECTION ( 'NONE',  ( -0.000000000000000000, 1.000000000000000000, -0.000000000000000000 ) ) ;
#19382=CARTESIAN_POINT ( 'NONE',  ( 58.47885130911549822, 12.69429933094348684, -22.36869975670756361 ) ) ;
#19384=DIRECTION ( 'NONE',  ( -0.000000000000000000, 1.000000000000000000, -0.000000000000000000 ) ) ;
#19386=CARTESIAN_POINT ( 'NONE',  ( 21.75198946226450403, 7.772524967554915953, -47.59311735406298993 ) ) ;
#19387=CARTESIAN_POINT ( 'NONE',  ( -146.5309471467636513, 62.99917515507676313, 45.10861342454792577 ) ) ;
#19388=CARTESIAN_POINT ( 'NONE',  ( 212.1983751099433277, 117.2326047784726910, 36.84905167329434050 ) ) ;
#19389=FACE_BOUND ( 'NONE', #26201, .T. ) ;
#19390=ORIENTED_EDGE ( 'NONE', *, *, #18430, .T. ) ;
#19394=CARTESIAN_POINT ( 'NONE',  ( 32.09610685027467269, 8.582590950734788393, -71.67746533053700375 ) ) ;
#19396=CARTESIAN_POINT ( 'NONE',  ( 8.730760620888057488, 6.377258547620704654, 93.82534041452976226 ) ) ;
#19398=CARTESIAN_POINT ( 'NONE',  ( 22.85407693638847348, 7.837765153256906814, 88.66769795570787949 ) ) ;
#19399=AXIS2_PLACEMENT_3D ( 'NONE', #4120, #25588, #62520 ) ;
#19400=ORIENTED_EDGE ( 'NONE', *, *, #32858, .F. ) ;
#19403=CARTESIAN_POINT ( 'NONE',  ( 199.7291770695759965, 101.4092159658446946, -38.20255649232857564 ) ) ;
#19406=CARTESIAN_POINT ( 'NONE',  ( 107.2081108419789359, 28.60378084105236240, -90.20802963420143783 ) ) ;
#19408=CARTESIAN_POINT ( 'NONE',  ( -78.66644367742111399, 22.32174330031318377, -76.96000122218160300 ) ) ;
#19409=CARTESIAN_POINT ( 'NONE',  ( -56.97556689808916985, 16.24958672959847661, -8.618408225133944001 ) ) ;
#19416=CARTESIAN_POINT ( 'NONE',  ( 105.4134760436918299, 27.80903124201758558, 16.02569942440996087 ) ) ;
#19417=ORIENTED_EDGE ( 'NONE', *, *, #37908, .F. ) ;
#19418=CARTESIAN_POINT ( 'NONE',  ( -24.67506180694751450, 8.578306485686441718, 88.10122643889526728 ) ) ;
#19419=CARTESIAN_POINT ( 'NONE',  ( 175.5498284945444709, 74.57669191966280664, -75.65732398570116857 ) ) ;
#19422=CARTESIAN_POINT ( 'NONE',  ( 82.95856197793166587, 19.25847567427440765, -49.88006847027852331 ) ) ;
#19423=CARTESIAN_POINT ( 'NONE',  ( -169.3509183217342127, 84.49925590041679868, -89.40419402843292573 ) ) ;
#19428=CARTESIAN_POINT ( 'NONE',  ( -180.4355333984925096, 97.25072438123878271, 90.31203738677328374 ) ) ;
#19430=CYLINDRICAL_SURFACE ( 'NONE', #20889, 7.500000000000027534 ) ;
#19432=CARTESIAN_POINT ( 'NONE',  ( -27.40035611173194852, 8.962996713195352072, -90.17232150666276880 ) ) ;
#19433=CARTESIAN_POINT ( 'NONE',  ( 210.9748732031754628, 117.1974929539830441, 86.27819310157629218 ) ) ;
#19434=ADVANCED_FACE ( 'NONE', ( #14317 ), #13616, .F. ) ;
#19435=CARTESIAN_POINT ( 'NONE',  ( 207.2640160519426047, 111.6867652229576322, 29.65748712772104767 ) ) ;
#19437=CARTESIAN_POINT ( 'NONE',  ( -109.7793173546316723, 36.75648380851384900, 38.30271184306513277 ) ) ;
#19439=EDGE_CURVE ( 'NONE', #26339, #41403, #66479, .T. ) ;
#19440=CARTESIAN_POINT ( 'NONE',  ( 13.36262230781615301, 7.441298897118794997, -9.060692098087766766 ) ) ;
#19442=CARTESIAN_POINT ( 'NONE',  ( 197.5334904971816741, 97.00846725096933199, -14.74015068199268441 ) ) ;
#19444=CARTESIAN_POINT ( 'NONE',  ( -147.3669217311067428, 63.69361261596462498, 4.184853556603538749 ) ) ;
#19446=CARTESIAN_POINT ( 'NONE',  ( 188.2091813586561386, 87.61952156613882892, -68.21099885728685308 ) ) ;
#19447=CARTESIAN_POINT ( 'NONE',  ( -144.9412191745148277, 61.69548892475974355, 71.03477123040856611 ) ) ;
#19449=CARTESIAN_POINT ( 'NONE',  ( 39.40195752203891999, 8.409560354027407314, -35.61981746542776506 ) ) ;
#19452=CARTESIAN_POINT ( 'NONE',  ( 14.80291736570133843, 7.477373894757625372, -35.56751837549798978 ) ) ;
#19453=CARTESIAN_POINT ( 'NONE',  ( 128.0568017572569204, 38.03085713813910473, -48.30530462611437770 ) ) ;
#19461=CARTESIAN_POINT ( 'NONE',  ( -28.13852122803041667, 9.072484007196644384, -76.41398812605804380 ) ) ;
#19465=CARTESIAN_POINT ( 'NONE',  ( 12.03194517566455701, 6.409266703743583093, 17.18016951692776217 ) ) ;
#19468=CARTESIAN_POINT ( 'NONE',  ( 174.9042454172880241, 72.57746269938726869, -66.28938837206885637 ) ) ;
#19470=CARTESIAN_POINT ( 'NONE',  ( 93.85846834761628088, 22.01563781856518887, -18.49024407162987416 ) ) ;
#19471=CARTESIAN_POINT ( 'NONE',  ( -24.71645982722741408, 9.599558729461495687, 67.89525075705670076 ) ) ;
#19473=CARTESIAN_POINT ( 'NONE',  ( -54.57280099357648595, 14.55288945003961665, 57.16187836339484107 ) ) ;
#19474=CARTESIAN_POINT ( 'NONE',  ( -0.3747453031323929595, 6.520267647591904137, 63.47172518997308543 ) ) ;
#19475=ORIENTED_EDGE ( 'NONE', *, *, #15710, .T. ) ;
#19476=CARTESIAN_POINT ( 'NONE',  ( 63.01563776193091826, 13.70579113808095073, -23.87614024170608218 ) ) ;
#19477=CARTESIAN_POINT ( 'NONE',  ( 150.0980941434704903, 53.37942190380066876, 62.34908842616228242 ) ) ;
#19478=CARTESIAN_POINT ( 'NONE',  ( -109.7156874346698316, 37.87149323084331343, -68.34337640632028865 ) ) ;
#19479=CARTESIAN_POINT ( 'NONE',  ( -47.55360235114365963, 12.79819361309568215, -43.22893570361206628 ) ) ;
#19495=CARTESIAN_POINT ( 'NONE',  ( 104.0290905220488469, -170.0000000000000000, 94.99999999999866418 ) ) ;
#19496=AXIS2_PLACEMENT_3D ( 'NONE', #5929, #50254, #19274 ) ;
#19498=CARTESIAN_POINT ( 'NONE',  ( -84.23336401058611500, 25.60798568215573923, 42.96773630549936485 ) ) ;
#19499=CARTESIAN_POINT ( 'NONE',  ( 8.000000000000007105, 249.8719672152120381, 94.99999999999866418 ) ) ;
#19501=CARTESIAN_POINT ( 'NONE',  ( 141.0645618855930650, 45.95036951196543384, 8.026184627116476733 ) ) ;
#19502=VECTOR ( 'NONE', #34413, 1000.000000000000000 ) ;
#19507=CARTESIAN_POINT ( 'NONE',  ( 12.03317402819681803, 6.409531826169462931, 57.86235655824060586 ) ) ;
#19508=B_SPLINE_CURVE_WITH_KNOTS ( 'NONE', 3,
 ( #55061, #28333, #27637, #914, #1606, #22363, #22714, #50146, #1970, #11803, #43801, #38540, #44153, #23068, #37848, #11110, #44520, #65995, #23429, #44868, #59294, #32575, #46242, #30084, #3007, #56819, #40288, #29052, #50493, #45557, #51540, #3684, #24466, #67720, #25161, #3347, #46589, #18830, #24807, #2315, #13216, #30424, #12870, #7595, #61731, #18484, #13557, #45910 ),
 .UNSPECIFIED., .F., .F.,
 ( 4, 2, 2, 2, 2, 2, 2, 2, 2, 2, 2, 2, 2, 2, 2, 2, 2, 2, 2, 2, 2, 2, 2, 4 ),
 ( 0.02746511744866866542, 0.02914922134997094058, 0.03083332525127321228, 0.03251742915257548744, 0.03335948110322665278, 0.03420153305387781811, 0.03504358500452898345, 0.03588563695518015573, 0.03756974085648243783, 0.03841179280713359623, 0.03925384475778478238, 0.04009589670843596160, 0.04093794865908714081, 0.04262205256038945761, 0.04430615646169178135, 0.04514820841234293974, 0.04599026036299409814, 0.04767436426429639412, 0.04935846816559869010, 0.05020052011624982768, 0.05104257206690095833, 0.05272667596820322655, 0.05356872791885436413, 0.05441077986950550865 ),
 .UNSPECIFIED. ) ;
#19509=CARTESIAN_POINT ( 'NONE',  ( -125.8938041572051389, 47.69968343338780414, 18.77539728269342945 ) ) ;
#19510=CARTESIAN_POINT ( 'NONE',  ( -78.40344607829260326, 23.29806210341294914, 84.10570090962099243 ) ) ;
#19515=AXIS2_PLACEMENT_3D ( 'NONE', #37439, #58546, #6121 ) ;
#19516=EDGE_CURVE ( 'NONE', #43039, #58488, #10750, .T. ) ;
#19518=CARTESIAN_POINT ( 'NONE',  ( 15.78827728214693416, -170.0000000000000000, -16.17439350822211352 ) ) ;
#19526=CARTESIAN_POINT ( 'NONE',  ( 17.45129144173298386, 7.566322476434613975, -89.38286583354187087 ) ) ;
#19528=CARTESIAN_POINT ( 'NONE',  ( -51.34542473642581939, 14.75635007918829089, 31.29311869111193900 ) ) ;
#19530=EDGE_LOOP ( 'NONE', ( #68339, #9043 ) ) ;
#19531=CARTESIAN_POINT ( 'NONE',  ( -103.2164890789475464, 34.39030697009940951, 18.63064823786974245 ) ) ;
#19534=CARTESIAN_POINT ( 'NONE',  ( 164.9559213734325169, 63.71338633026441300, 64.29752433092906472 ) ) ;
#19543=CARTESIAN_POINT ( 'NONE',  ( -153.6946616617039467, 69.16142959008689672, -21.70738820025326632 ) ) ;
#19544=CARTESIAN_POINT ( 'NONE',  ( -79.14127775978546708, 22.50259208414362178, 57.26275173013681297 ) ) ;
#19548=DIRECTION ( 'NONE',  ( 0.000000000000000000, 0.000000000000000000, 1.000000000000000000 ) ) ;
#19552=CARTESIAN_POINT ( 'NONE',  ( 32.90878072717890035, 7.653588083204840409, 68.01993794000820515 ) ) ;
#19553=CARTESIAN_POINT ( 'NONE',  ( 10.83418588031599228, 6.392467435475929882, -21.82701683438974882 ) ) ;
#19555=CARTESIAN_POINT ( 'NONE',  ( -31.43908319763710679, -170.0000000000000000, 64.56100499665288339 ) ) ;
#19557=CARTESIAN_POINT ( 'NONE',  ( -118.3927673406137586, 41.74929850983304647, 11.51331731855512075 ) ) ;
#19573=ORIENTED_EDGE ( 'NONE', *, *, #1780, .F. ) ;
#19575=CARTESIAN_POINT ( 'NONE',  ( 201.9822477997853127, 104.3642793804899895, 2.860239141982756195 ) ) ;
#19577=CARTESIAN_POINT ( 'NONE',  ( 164.9669969155543185, 65.04083371431683247, 90.15876886485268926 ) ) ;
#19579=CARTESIAN_POINT ( 'NONE',  ( -58.33157376762795820, 16.63098604184964557, 17.72246446630213512 ) ) ;
#19581=CARTESIAN_POINT ( 'NONE',  ( -156.9262190792699414, 72.10659547035872663, 39.35937735580755970 ) ) ;
#19582=CARTESIAN_POINT ( 'NONE',  ( -101.3602137809054540, 32.31558061113913993, 30.56121215972862615 ) ) ;
#19585=ORIENTED_EDGE ( 'NONE', *, *, #28499, .T. ) ;
#19588=EDGE_LOOP ( 'NONE', ( #43297, #40481, #48192, #23884 ) ) ;
#19590=CARTESIAN_POINT ( 'NONE',  ( 174.2538192999570299, 73.34752463892031926, 33.69852078121099481 ) ) ;
#19591=VECTOR ( 'NONE', #59712, 1000.000000000000000 ) ;
#19592=CARTESIAN_POINT ( 'NONE',  ( 21.75684465274325063, 6.764994602232766496, -65.29556045911284912 ) ) ;
#19594=CARTESIAN_POINT ( 'NONE',  ( -130.1938957973835613, 50.61368074696269304, 58.80196259642822554 ) ) ;
#19596=CARTESIAN_POINT ( 'NONE',  ( -101.7497140795961883, 33.63993131142439807, 84.22103294299186871 ) ) ;
#19597=CYLINDRICAL_SURFACE ( 'NONE', #19399, 7.500000000000020428 ) ;
#19600=CARTESIAN_POINT ( 'NONE',  ( -59.95707852844800101, 16.05120821151901822, -21.56757814541855112 ) ) ;
#19603=EDGE_CURVE ( 'NONE', #22089, #47148, #32292, .T. ) ;
#19605=CARTESIAN_POINT ( 'NONE',  ( 116.8917656767876565, 33.20682060519247614, 40.59075185124044793 ) ) ;
#19606=VECTOR ( 'NONE', #49236, 1000.000000000000000 ) ;
#19608=CARTESIAN_POINT ( 'NONE',  ( -101.8191498210054959, 32.54686850610961812, -76.85912785543960979 ) ) ;
#19612=CARTESIAN_POINT ( 'NONE',  ( -143.3980294393559234, 60.45217072626395094, -19.82599328075919232 ) ) ;
#19615=CARTESIAN_POINT ( 'NONE',  ( -52.14489132612000333, 13.92110435672092450, -89.48874280495719802 ) ) ;
#19616=CARTESIAN_POINT ( 'NONE',  ( -50.48111445489777793, 14.53992017381783697, -90.45588132977169948 ) ) ;
#19618=CARTESIAN_POINT ( 'NONE',  ( 70.45451534980409747, 15.56315969138428557, -44.20839769585855805 ) ) ;
#19620=CARTESIAN_POINT ( 'NONE',  ( -170.2747214445849977, 84.01465441107040988, -62.10472265096723987 ) ) ;
#19622=CARTESIAN_POINT ( 'NONE',  ( -109.3386876948163575, 37.66246927061209959, 35.43368312552478017 ) ) ;
#19623=ORIENTED_EDGE ( 'NONE', *, *, #9005, .F. ) ;
#19624=CARTESIAN_POINT ( 'NONE',  ( -38.54881010929333485, 10.86689971295296786, 13.30968753690000383 ) ) ;
#19626=VERTEX_POINT ( 'NONE', #898 ) ;
#19630=CARTESIAN_POINT ( 'NONE',  ( 38.43102714813441878, 9.298961820315049920, 3.116234321035345811 ) ) ;
#19632=CARTESIAN_POINT ( 'NONE',  ( 36.08729376665094435, 8.001156100723203934, 17.31492220065397447 ) ) ;
#19634=CARTESIAN_POINT ( 'NONE',  ( -33.38294402636582703, 10.93918551420889962, -8.712282913815599272 ) ) ;
#19636=CARTESIAN_POINT ( 'NONE',  ( -123.0640300519512635, 45.85328288118120810, -89.14461900415201967 ) ) ;
#19640=CARTESIAN_POINT ( 'NONE',  ( -26.88245755577922580, 8.887394979218512958, 4.894357216155159840 ) ) ;
#19643=CARTESIAN_POINT ( 'NONE',  ( -15.27748264047829352, 7.491388194171920034, -68.78227764318798165 ) ) ;
#19644=CARTESIAN_POINT ( 'NONE',  ( -35.17600017528511103, 10.23461991275926941, 31.20910972668009009 ) ) ;
#19650=CARTESIAN_POINT ( 'NONE',  ( -124.1033713525885673, 45.32626312604506325, 45.40670476773291142 ) ) ;
#19654=CARTESIAN_POINT ( 'NONE',  ( -180.3161328724958423, 97.10341277064809162, -66.91777817630556058 ) ) ;
#19656=CARTESIAN_POINT ( 'NONE',  ( 126.3615183855829116, 38.23138460739041022, 90.24396629769827882 ) ) ;
#19657=CARTESIAN_POINT ( 'NONE',  ( 111.1868021579657153, 29.32055685204860396, 44.56662876905394199 ) ) ;
#19663=CARTESIAN_POINT ( 'NONE',  ( 204.6977192012829789, 106.3443248447423457, 44.20772073876944575 ) ) ;
#19664=CARTESIAN_POINT ( 'NONE',  ( 56.67004931728209982, -170.0000000000000000, 94.99999999999866418 ) ) ;
#19665=CARTESIAN_POINT ( 'NONE',  ( 187.6511924654682275, 87.00187850361886888, 33.17587653223696265 ) ) ;
#19666=CARTESIAN_POINT ( 'NONE',  ( 181.4360341826970853, 78.96155396928541848, -89.91415884680696990 ) ) ;
#19670=CARTESIAN_POINT ( 'NONE',  ( 163.2911130186310515, 63.63047778106599139, -12.04342320290372470 ) ) ;
#19672=ADVANCED_FACE ( 'NONE', ( #33959 ), #65625, .F. ) ;
#19673=DIRECTION ( 'NONE',  ( 0.000000000000000000, 0.000000000000000000, 1.000000000000000000 ) ) ;
#19674=CARTESIAN_POINT ( 'NONE',  ( 138.5902997793499196, 44.35633795166239679, 84.84391433248465830 ) ) ;
#19675=CARTESIAN_POINT ( 'NONE',  ( 155.7265855639938650, 57.57443315515123317, 2.757056929193004713 ) ) ;
#19677=CARTESIAN_POINT ( 'NONE',  ( -146.1142527948576912, 61.35394402951023096, -62.46500431941766607 ) ) ;
#19679=CARTESIAN_POINT ( 'NONE',  ( 161.7209903610255139, 61.03262545641850068, -37.42759312634723301 ) ) ;
#19680=EDGE_LOOP ( 'NONE', ( #24228, #66088, #67002, #49137 ) ) ;
#19681=CARTESIAN_POINT ( 'NONE',  ( -95.63694837622352907, 30.64472169584718841, 14.66480637497265604 ) ) ;
#19682=EDGE_CURVE ( 'NONE', #5387, #2906, #18834, .T. ) ;
#19684=CARTESIAN_POINT ( 'NONE',  ( -131.1078488676298832, 50.02394948559179255, 43.51637233646730607 ) ) ;
#19687=CARTESIAN_POINT ( 'NONE',  ( 82.12277968641507186, 18.98848723477811262, -10.46207403576605621 ) ) ;
#19688=CARTESIAN_POINT ( 'NONE',  ( -7.825402957745085430, 7.899365992529248537, -35.41807073194381417 ) ) ;
#19689=CARTESIAN_POINT ( 'NONE',  ( 155.7277429502854034, 56.30804678861343859, 56.44591023570471577 ) ) ;
#19690=CARTESIAN_POINT ( 'NONE',  ( 89.88147981065577596, 21.62466191578946351, 43.98752394672685284 ) ) ;
#19693=CARTESIAN_POINT ( 'NONE',  ( -13.79190010541702982, 8.363435739308561878, 69.03078841869681526 ) ) ;
#19695=EDGE_CURVE ( 'NONE', #48132, #29084, #45619, .T. ) ;
#19697=CARTESIAN_POINT ( 'NONE',  ( 212.0779786303466210, 118.9010947973413437, -18.35900109281879367 ) ) ;
#19700=CARTESIAN_POINT ( 'NONE',  ( 103.8055367708241334, 27.11070767929348690, 40.99165044060047336 ) ) ;
#19702=CARTESIAN_POINT ( 'NONE',  ( 62.38297021405776377, 12.52668572540603975, 83.52147531495063504 ) ) ;
#19704=CARTESIAN_POINT ( 'NONE',  ( 185.7267155939802024, 84.90388481853132419, 4.069038840943626667 ) ) ;
#19705=CARTESIAN_POINT ( 'NONE',  ( 212.0180052085437694, 116.9552462415714871, -42.16221012700841442 ) ) ;
#19706=AXIS2_PLACEMENT_3D ( 'NONE', #9658, #52889, #26173 ) ;
#19707=CARTESIAN_POINT ( 'NONE',  ( 180.2572128312846758, 77.77323980479702925, 2.497912692282359792 ) ) ;
#19708=CARTESIAN_POINT ( 'NONE',  ( -57.65733424639442717, 15.39521790791522982, 18.01019561178333817 ) ) ;
#19710=CARTESIAN_POINT ( 'NONE',  ( 181.0840389613909736, -170.0000000000000000, -51.22505766587963905 ) ) ;
#19713=CARTESIAN_POINT ( 'NONE',  ( 103.0103829243728768, 25.67737053862327556, -68.21726512339051851 ) ) ;
#19714=EDGE_CURVE ( 'NONE', #9829, #9227, #6950, .T. ) ;
#19718=CARTESIAN_POINT ( 'NONE',  ( -0.4222246928121727860, 6.521921806359222806, 92.54939115416705420 ) ) ;
#19720=EDGE_CURVE ( 'NONE', #10221, #7307, #21308, .T. ) ;
#19723=CARTESIAN_POINT ( 'NONE',  ( -71.96390573417176029, 19.88067451234326910, 68.16606071164316916 ) ) ;
#19727=CARTESIAN_POINT ( 'NONE',  ( -151.2497169612549328, 65.66843968092749151, 45.56996481252021880 ) ) ;
#19729=CARTESIAN_POINT ( 'NONE',  ( 176.4367926094704728, 74.03315361639846515, -22.77209446790686442 ) ) ;
#19732=LINE ( 'NONE', #9182, #57010 ) ;
#19734=CARTESIAN_POINT ( 'NONE',  ( 22.15943197741200521, 7.796127622097904997, -46.98355238114885424 ) ) ;
#19735=CARTESIAN_POINT ( 'NONE',  ( 8.540564391411908929, 7.383006541823029956, 62.41466723577283204 ) ) ;
#19736=CARTESIAN_POINT ( 'NONE',  ( 212.1931396682532807, 117.2245435827729239, 37.02143851943622366 ) ) ;
#19737=FACE_BOUND ( 'NONE', #19082, .T. ) ;
#19741=EDGE_LOOP ( 'NONE', ( #48806, #52788, #63849, #39047 ) ) ;
#19743=CARTESIAN_POINT ( 'NONE',  ( -119.0183326251804345, 43.31072671377873462, 88.79436413878467249 ) ) ;
#19745=CARTESIAN_POINT ( 'NONE',  ( 34.82939798935585429, 8.870855050008909615, -63.99916360883118926 ) ) ;
#19747=CARTESIAN_POINT ( 'NONE',  ( 21.33146652848267522, 6.741339414847635325, 86.14122630416260051 ) ) ;
#19748=CARTESIAN_POINT ( 'NONE',  ( 23.18757945110744600, 7.858491809880083778, 89.93510652474785161 ) ) ;
#19750=AXIS2_PLACEMENT_3D ( 'NONE', #52855, #51508, #3309 ) ;
#19754=VECTOR ( 'NONE', #12690, 1000.000000000000000 ) ;
#19755=CARTESIAN_POINT ( 'NONE',  ( 197.9843579228224542, 99.18296459057403069, -40.47005908839251731 ) ) ;
#19757=CARTESIAN_POINT ( 'NONE',  ( -86.15441609607630369, 25.31657638323078530, 10.57859359723828518 ) ) ;
#19761=CARTESIAN_POINT ( 'NONE',  ( -57.89360549284268842, 16.50663738101751221, -8.918089600607720158 ) ) ;
#19765=CARTESIAN_POINT ( 'NONE',  ( 8.540853903193186270, 6.376814430361480213, -41.07341765948896750 ) ) ;
#19767=CARTESIAN_POINT ( 'NONE',  ( 17.48889770758266593, 6.561062909825351674, 3.361356057925529939 ) ) ;
#19772=CARTESIAN_POINT ( 'NONE',  ( -23.94826066252556274, 8.481232536276079870, 91.89930965450892586 ) ) ;
#19773=CARTESIAN_POINT ( 'NONE',  ( 173.8576514579035290, 72.97529922124006418, -68.54141255106546282 ) ) ;
#19775=CARTESIAN_POINT ( 'NONE',  ( 104.3805245147141818, 26.26278144139195447, -48.12669505167198736 ) ) ;
#19776=B_SPLINE_CURVE_WITH_KNOTS ( 'NONE', 3,
 ( #3922, #29965, #51425, #20099, #3569, #3236, #14808, #57734, #8861, #19748, #41210, #9545, #19398, #40860, #53119, #58405, #15850, #16194, #48523, #36970, #42911, #5633, #27090, #25732, #64376, #37294, #20780, #53466, #26069, #20430, #15165, #47497, #68958, #42243, #5298, #26756, #47163, #68625, #41895, #10911, #32035, #53808, #63355, #36627, #32382, #31347, #63705, #10567, #9894, #58077, #15516, #31685, #10219, #58745, #52776, #59095 ),
 .UNSPECIFIED., .F., .F.,
 ( 4, 2, 2, 2, 2, 2, 2, 2, 2, 2, 2, 2, 2, 2, 2, 2, 2, 2, 2, 2, 2, 2, 2, 2, 2, 2, 2, 4 ),
 ( 0.000000000000000000, 0.001960836769587751254, 0.002941255154381627098, 0.003921673539175502508, 0.004902091923969378352, 0.005882510308763254196, 0.006862928693557130040, 0.007843347078351005017, 0.009804183847938715071, 0.01078460223273256663, 0.01176502061752641645, 0.01274543900232026801, 0.01372585738711412130, 0.01470627577190797113, 0.01568669415670182268, 0.01764753092628952580, 0.01960836769587722545, 0.02058878608067108915, 0.02156920446546494591, 0.02254962285025880267, 0.02353004123505265943, 0.02451045961984651966, 0.02549087800464037643, 0.02745171477422813505, 0.02843213315902201610, 0.02941255154381589368, 0.03039296992860977473, 0.03137338831340365231 ),
 .UNSPECIFIED. ) ;
#19782=CARTESIAN_POINT ( 'NONE',  ( 41.35041461497708326, 8.670465437677201237, 17.82849842206101343 ) ) ;
#19783=CARTESIAN_POINT ( 'NONE',  ( 174.1348882614952629, 73.23561817543360064, 12.79949674401064996 ) ) ;
#19786=CARTESIAN_POINT ( 'NONE',  ( 126.5710838895481913, 37.19597237024180458, 8.365867632742146398 ) ) ;
#19787=CARTESIAN_POINT ( 'NONE',  ( -155.7495771807047333, 69.65980221699318520, 7.188372552036696561 ) ) ;
#19788=CARTESIAN_POINT ( 'NONE',  ( 8.000000000000007105, 249.8719672152120381, 94.99999999999866418 ) ) ;
#19789=CARTESIAN_POINT ( 'NONE',  ( 211.8345664497467169, 118.5225165986914106, 34.37992018911904779 ) ) ;
#19790=CARTESIAN_POINT ( 'NONE',  ( -85.95621526752231034, 26.32462117888286457, 62.98115503426731010 ) ) ;
#19791=CARTESIAN_POINT ( 'NONE',  ( -107.7893514267588273, 35.66840175773127442, 32.90635557035678715 ) ) ;
#19801=B_SPLINE_CURVE_WITH_KNOTS ( 'NONE', 3,
 ( #58591, #42083, #9739, #41743, #68146, #62860, #15007, #9392, #26259, #42761, #5140, #15358, #64224, #47347, #58258, #20977, #68805, #10409, #36817, #26598, #48035, #57583, #63887, #10076, #20621, #31535, #47690, #37488, #69154, #19952, #31879, #4116, #42428, #30851, #52634, #58939, #41406, #15697, #32226, #20284, #63204, #31201, #10759, #52296, #37147, #69495 ),
 .UNSPECIFIED., .F., .F.,
 ( 4, 2, 2, 2, 2, 2, 2, 2, 2, 2, 2, 2, 2, 2, 2, 2, 2, 2, 2, 2, 2, 2, 4 ),
 ( 0.000000000000000000, 0.003736383952885354628, 0.005604575929328017847, 0.007472767905770679765, 0.008406863893992011158, 0.009340959882213341683, 0.01120915185865600794, 0.01214324784687734714, 0.01307734383509868981, 0.01401143982332003247, 0.01494553581154137514, 0.01587963179976271955, 0.01681372778798406048, 0.01774782377620540141, 0.01868191976442674582, 0.01961601575264808675, 0.02055011174086943115, 0.02148420772909077209, 0.02241830371731211302, 0.02428649569375482264, 0.02615468767019753227, 0.02802287964664024536, 0.02989107162308295151 ),
 .UNSPECIFIED. ) ;
#19805=EDGE_CURVE ( 'NONE', #39302, #145, #2027, .T. ) ;
#19807=VECTOR ( 'NONE', #55029, 1000.000000000000000 ) ;
#19809=CARTESIAN_POINT ( 'NONE',  ( 34.45500533947588195, 7.817363290423887001, -37.46142013688670858 ) ) ;
#19814=CARTESIAN_POINT ( 'NONE',  ( 130.7531879853686121, 39.58149302537893277, -36.67985178847166594 ) ) ;
#19820=CARTESIAN_POINT ( 'NONE',  ( -31.43908319763709969, 9.591432048623765638, -77.16174795566554678 ) ) ;
#19822=CARTESIAN_POINT ( 'NONE',  ( 15.78827728214693416, 6.500811158483328356, 18.17015708224157322 ) ) ;
#19823=CARTESIAN_POINT ( 'NONE',  ( 45.04506994399699948, 10.22854084020124077, -74.92927396681155017 ) ) ;
#19825=CARTESIAN_POINT ( 'NONE',  ( 175.3815143714021758, 73.02838262207001208, -65.69146865943324087 ) ) ;
#19827=CARTESIAN_POINT ( 'NONE',  ( -85.61911145880966956, 26.18322756479841473, -93.48309464426087345 ) ) ;
#19829=CARTESIAN_POINT ( 'NONE',  ( -26.88234027341226096, 9.904106450608205492, 58.58403535530551665 ) ) ;
#19832=VERTEX_POINT ( 'NONE', #1506 ) ;
#19834=CARTESIAN_POINT ( 'NONE',  ( -129.6165111262478717, 48.99406349865700605, -75.77339883365759476 ) ) ;
#19836=CARTESIAN_POINT ( 'NONE',  ( -51.13073217147959326, 13.66490163179657458, -36.31884843616727210 ) ) ;
#19842=VERTEX_POINT ( 'NONE', #16633 ) ;
#19853=CYLINDRICAL_SURFACE ( 'NONE', #47661, 7.500000000000020428 ) ;
#19857=CARTESIAN_POINT ( 'NONE',  ( -25.48750459758502984, 9.705678256319565378, -20.56274929115669181 ) ) ;
#19860=EDGE_CURVE ( 'NONE', #5706, #29569, #46478, .T. ) ;
#19862=CARTESIAN_POINT ( 'NONE',  ( 107.9342863085848450, 28.93180871323605530, -23.72930682673416314 ) ) ;
#19863=CARTESIAN_POINT ( 'NONE',  ( 8.951900209438536038, 6.378066731449595572, 61.26501831331611214 ) ) ;
#19865=CARTESIAN_POINT ( 'NONE',  ( 198.4059165548112276, 99.71594270191988585, 40.79851715686629632 ) ) ;
#19867=CARTESIAN_POINT ( 'NONE',  ( -74.08105192128697070, 21.69630190401540304, 85.63813808529961591 ) ) ;
#19870=CARTESIAN_POINT ( 'NONE',  ( 69.48877314113907744, 15.30784187978995092, 41.10903227078659938 ) ) ;
#19876=CARTESIAN_POINT ( 'NONE',  ( 199.7255144154429161, 99.76581417577203581, -76.30443167248331804 ) ) ;
#19877=DIRECTION ( 'NONE',  ( -0.000000000000000000, 1.000000000000000000, -0.000000000000000000 ) ) ;
#19878=CARTESIAN_POINT ( 'NONE',  ( -119.5267374018686297, 42.44190186039714519, 68.96077536236255412 ) ) ;
#19879=CARTESIAN_POINT ( 'NONE',  ( -84.23336401058614342, 25.60798568215575344, -10.72136487542798555 ) ) ;
#19881=CARTESIAN_POINT ( 'NONE',  ( -47.60266343315662141, 13.84328785304053078, 38.81655012327907173 ) ) ;
#19885=B_SPLINE_CURVE_WITH_KNOTS ( 'NONE', 3,
 ( #50596, #24227, #18939, #29486, #2417, #50949, #45674, #56568, #8390, #29835, #51306, #3115, #67478, #62187, #14005, #8744, #30191, #3452, #62548, #41434, #42118, #36848, #15390, #3797, #62890, #47380, #31916, #20314, #51980, #68834, #68178, #53343, #20659, #52327, #9080, #4150, #63576, #57614, #5175, #58286, #46700, #30531, #10107, #69187 ),
 .UNSPECIFIED., .F., .F.,
 ( 4, 2, 2, 2, 2, 2, 2, 2, 2, 2, 2, 2, 2, 2, 2, 2, 2, 2, 2, 2, 2, 4 ),
 ( 0.02416815208377490198, 0.02567033257376879693, 0.02642142281876574961, 0.02717251306376269882, 0.02867469355375655907, 0.02942578379875347705, 0.03017687404375039156, 0.03167905453374424141, 0.03318123502373808431, 0.03393232526873501270, 0.03468341551373193415, 0.03618559600372577012, 0.03693668624872267076, 0.03768777649371957139, 0.03918995698371340736, 0.04069213747370724332, 0.04219431796370107929, 0.04369649845369491525, 0.04444758869869185058, 0.04519867894368877204, 0.04670085943368265657, 0.04820303992367653417 ),
 .UNSPECIFIED. ) ;
#19886=CARTESIAN_POINT ( 'NONE',  ( 103.9652201950894721, 26.08439499369982073, 68.06684849509201740 ) ) ;
#19887=CARTESIAN_POINT ( 'NONE',  ( 112.8036877771481699, 30.08463150275148124, 83.74363904605614550 ) ) ;
#19889=CARTESIAN_POINT ( 'NONE',  ( 181.9295719569814480, 79.46350097013164770, -51.18950099341775228 ) ) ;
#19890=DIRECTION ( 'NONE',  ( -0.000000000000000000, 1.000000000000000000, -0.000000000000000000 ) ) ;
#19891=EDGE_CURVE ( 'NONE', #18664, #61225, #61564, .T. ) ;
#19892=CARTESIAN_POINT ( 'NONE',  ( -145.9251124924754208, 62.49975471021623008, 85.31446015602850252 ) ) ;
#19900=CARTESIAN_POINT ( 'NONE',  ( 133.8566784816069344, 42.60093787723652525, -51.02331093239568816 ) ) ;
#19903=CARTESIAN_POINT ( 'NONE',  ( -55.53456145826332602, 15.85318253404850353, 30.31732777293112946 ) ) ;
#19904=CARTESIAN_POINT ( 'NONE',  ( -36.38071096718372388, 11.47804921491336216, -63.99874941106702408 ) ) ;
#19907=CARTESIAN_POINT ( 'NONE',  ( 183.9887307715836471, 83.05100282186907634, 70.57129800896366589 ) ) ;
#19908=CARTESIAN_POINT ( 'NONE',  ( 9.416656162223555171, 6.380306691996769253, -12.21039664973801209 ) ) ;
#19911=CARTESIAN_POINT ( 'NONE',  ( -5.885876544836656343, 6.772369038004115716, -50.16710263326163499 ) ) ;
#19912=CARTESIAN_POINT ( 'NONE',  ( 188.5843222076478867, 86.53342480589837749, 63.94975097486255322 ) ) ;
#19915=CARTESIAN_POINT ( 'NONE',  ( 127.1040286383415889, 37.49395136275129659, -19.95267234602065898 ) ) ;
#19916=CARTESIAN_POINT ( 'NONE',  ( 22.15926701483431316, 7.796117250416240374, -12.20938565424666500 ) ) ;
#19917=CARTESIAN_POINT ( 'NONE',  ( 13.84704553156522167, 7.452804552247568992, 3.421577053668306334 ) ) ;
#19922=CARTESIAN_POINT ( 'NONE',  ( 129.1310456962234809, 39.80382822048400726, -49.36754109056038686 ) ) ;
#19926=CARTESIAN_POINT ( 'NONE',  ( 186.5979919519638486, 85.84756789133378163, -38.63534547958833798 ) ) ;
#19929=EDGE_CURVE ( 'NONE', #5910, #58406, #17070, .T. ) ;
#19930=CARTESIAN_POINT ( 'NONE',  ( -142.9730935922299295, 58.82921737386681826, -11.77770370840645420 ) ) ;
#19931=EDGE_CURVE ( 'NONE', #36547, #6792, #47341, .T. ) ;
#19935=CARTESIAN_POINT ( 'NONE',  ( 155.4893034622222672, 57.39280319106983796, 83.35853011262113910 ) ) ;
#19937=CARTESIAN_POINT ( 'NONE',  ( -58.97243502469717669, 16.81420332340175960, 17.37168708933159422 ) ) ;
#19941=DIRECTION ( 'NONE',  ( 0.000000000000000000, 0.000000000000000000, 1.000000000000000000 ) ) ;
#19946=ORIENTED_EDGE ( 'NONE', *, *, #21796, .T. ) ;
#19950=CARTESIAN_POINT ( 'NONE',  ( -168.1811549361197820, 83.25427431521137578, 5.828879898275340921 ) ) ;
#19952=CARTESIAN_POINT ( 'NONE',  ( -179.6470915626256897, 94.69856161161345653, -19.07391450275219924 ) ) ;
#19955=CARTESIAN_POINT ( 'NONE',  ( -130.5811943660945360, 50.88295841537573949, 59.08986182251942409 ) ) ;
#19957=CARTESIAN_POINT ( 'NONE',  ( -109.0191069781766657, 37.48620563201052391, 94.99999999999866418 ) ) ;
#19962=CARTESIAN_POINT ( 'NONE',  ( -62.49130718206700408, 16.80297926264071506, -16.86221752726308409 ) ) ;
#19964=CARTESIAN_POINT ( 'NONE',  ( -130.5811943660945076, 50.88295841537573239, -75.13289112979900608 ) ) ;
#19965=CARTESIAN_POINT ( 'NONE',  ( 117.6924004117966263, 33.61107268965020722, 36.09735895212963186 ) ) ;
#19967=CARTESIAN_POINT ( 'NONE',  ( 70.51522979775974420, 15.57935281015687323, -69.56303398768666568 ) ) ;
#19968=VERTEX_POINT ( 'NONE', #27101 ) ;
#19969=ORIENTED_EDGE ( 'NONE', *, *, #53551, .T. ) ;
#19970=CARTESIAN_POINT ( 'NONE',  ( -142.3260422482981085, 59.60034523324941347, -13.23360016362279090 ) ) ;
#19971=CARTESIAN_POINT ( 'NONE',  ( -167.1534554062404254, 80.72263015867909530, -37.66204370233266729 ) ) ;
#19973=CARTESIAN_POINT ( 'NONE',  ( -47.76873007799818538, 12.84869220385979460, -94.56435065590063971 ) ) ;
#19976=CARTESIAN_POINT ( 'NONE',  ( 63.01563776193091826, 12.67277567978500130, -35.72069083216973695 ) ) ;
#19978=CARTESIAN_POINT ( 'NONE',  ( -172.3057147739577317, 86.22480007276995195, -76.52359078706952289 ) ) ;
#19980=CARTESIAN_POINT ( 'NONE',  ( -104.7956873821848660, 35.21322275870666374, 30.94966216072465670 ) ) ;
#19982=CARTESIAN_POINT ( 'NONE',  ( 79.98183030723785691, 18.31194381986301778, -93.43937185863195793 ) ) ;
#19987=CARTESIAN_POINT ( 'NONE',  ( 36.77024545412685796, 9.095083943590521969, 3.541950953158858884 ) ) ;
#19988=CARTESIAN_POINT ( 'NONE',  ( 38.91493890549795509, 8.346224043800605230, 3.069283715499573351 ) ) ;
#19990=CARTESIAN_POINT ( 'NONE',  ( -34.74023699876257609, 11.17830703027882855, -22.72455885904352257 ) ) ;
#19996=CARTESIAN_POINT ( 'NONE',  ( 8.767814708128309320, 7.383611927972575373, -72.51365984521781627 ) ) ;
#19997=CARTESIAN_POINT ( 'NONE',  ( -189.5325095384513645, 107.4952257375067433, 13.70762090391955823 ) ) ;
#20000=CARTESIAN_POINT ( 'NONE',  ( -98.67723517640901321, 30.98797878696540309, -9.087774546891575156 ) ) ;
#20002=CARTESIAN_POINT ( 'NONE',  ( 157.2533363798600021, 58.75760182111577024, -51.12418429913766005 ) ) ;
#20003=AXIS2_PLACEMENT_3D ( 'NONE', #14300, #50884, #45258 ) ;
#20006=CYLINDRICAL_SURFACE ( 'NONE', #61035, 7.500000000000013323 ) ;
#20008=CARTESIAN_POINT ( 'NONE',  ( -122.3745688183166322, 44.21964839958061333, 44.75990178122122387 ) ) ;
#20011=CARTESIAN_POINT ( 'NONE',  ( -177.1514380519392944, 93.28180884530864603, -62.71624474115134262 ) ) ;
#20012=CARTESIAN_POINT ( 'NONE',  ( 127.7121523762017858, 38.99241938113798511, 94.99999999999866418 ) ) ;
#20013=CARTESIAN_POINT ( 'NONE',  ( 203.3979956051160229, 106.2714448901421633, -90.12122811341167505 ) ) ;
#20018=CARTESIAN_POINT ( 'NONE',  ( -123.6619986853277737, 45.04188181212062858, -62.09435052478287531 ) ) ;
#20019=ORIENTED_EDGE ( 'NONE', *, *, #14255, .F. ) ;
#20020=CARTESIAN_POINT ( 'NONE',  ( 197.3707490726350215, 96.80690576410106019, 38.34013995466353464 ) ) ;
#20021=CARTESIAN_POINT ( 'NONE',  ( 116.0773578185793582, 31.67580513411752463, -75.00610128316866110 ) ) ;
#20022=CARTESIAN_POINT ( 'NONE',  ( 184.3879440808140089, 83.47316703125159165, 43.54523204561664329 ) ) ;
#20023=B_SPLINE_CURVE_WITH_KNOTS ( 'NONE', 3,
 ( #21816, #16886, #22174, #27438, #48527, #15855, #32730, #48876, #53815, #21472, #54157, #21147, #48191, #10572, #37649, #38347, #361, #37300, #65086, #5980, #27795, #49584, #43615, #53473, #59789, #11605, #33080, #54508, #5304, #42916, #49234, #11968, #43259, #22519, #38706, #58752, #16547, #1069, #32391, #32039, #5638, #17232, #43961, #65438 ),
 .UNSPECIFIED., .F., .F.,
 ( 4, 2, 2, 2, 2, 2, 2, 2, 2, 2, 2, 2, 2, 2, 2, 2, 2, 2, 2, 2, 2, 4 ),
 ( 0.02432640572110343971, 0.02583721026359365666, 0.02659261253483874779, 0.02734801480608383545, 0.02885881934857404546, 0.02961422161981916434, 0.03036962389106428670, 0.03188042843355452099, 0.03339123297604475182, 0.03414663524728984989, 0.03490203751853494796, 0.03641284206102511634, 0.03716824433227021440, 0.03792364660351530553, 0.03943445114600549473, 0.04094525568849567698, 0.04245606023098587312, 0.04396686477347605537, 0.04472226704472114650, 0.04547766931596623763, 0.04698847385845637131, 0.04849927840094650500 ),
 .UNSPECIFIED. ) ;
#20024=CARTESIAN_POINT ( 'NONE',  ( 139.6150621148398727, 46.20856238844174158, 14.99708312333219595 ) ) ;
#20028=DIRECTION ( 'NONE',  ( -0.000000000000000000, 1.000000000000000000, -0.000000000000000000 ) ) ;
#20030=CARTESIAN_POINT ( 'NONE',  ( 68.63585058221465829, 15.08566240483131793, 59.16672110021340103 ) ) ;
#20031=CARTESIAN_POINT ( 'NONE',  ( 128.9313739248989918, 38.52897977562246723, 85.03336623935274474 ) ) ;
#20032=ADVANCED_FACE ( 'NONE', ( #17241 ), #38712, .F. ) ;
#20037=CARTESIAN_POINT ( 'NONE',  ( 117.4806398654733783, 33.50379325299404343, -45.45665458773512313 ) ) ;
#20038=ORIENTED_EDGE ( 'NONE', *, *, #4822, .F. ) ;
#20039=FACE_OUTER_BOUND ( 'NONE', #29408, .T. ) ;
#20043=CARTESIAN_POINT ( 'NONE',  ( 79.39764314491564789, 18.13166883367086157, -18.48108370271943102 ) ) ;
#20044=CARTESIAN_POINT ( 'NONE',  ( -165.9992860119575084, 79.53569239468049545, 35.95263399248825209 ) ) ;
#20045=CARTESIAN_POINT ( 'NONE',  ( 157.0336341255056425, 57.31169401067823088, 56.25401806271707272 ) ) ;
#20051=CARTESIAN_POINT ( 'NONE',  ( 153.8224167330182297, 56.12711234192239829, -10.22241626634837353 ) ) ;
#20052=CARTESIAN_POINT ( 'NONE',  ( 205.5049354810107900, 109.1776577097391225, -24.48138044215792775 ) ) ;
#20053=CARTESIAN_POINT ( 'NONE',  ( 103.1534365798308386, 26.83148826706846179, 39.61125415960676577 ) ) ;
#20055=CARTESIAN_POINT ( 'NONE',  ( 56.31946197080010563, 11.21858957927811495, 87.60745826581978690 ) ) ;
#20056=B_SPLINE_CURVE_WITH_KNOTS ( 'NONE', 3,
 ( #46635, #46982, #30462, #3721, #25201, #68109, #48329, #42731, #53275, #27592, #64539, #59942, #163, #42394, #53956, #15999, #54308, #59586, #58903, #870, #5785, #11065, #519, #20938, #17028, #10718, #64187, #26219, #21621, #22322, #32192, #53624, #5449, #63856, #11762, #37448, #43067, #69112, #32876, #48000, #15665, #58555, #43762, #21282, #10372 ),
 .UNSPECIFIED., .F., .F.,
 ( 4, 2, 2, 1, 2, 2, 2, 2, 2, 2, 2, 2, 2, 2, 2, 2, 2, 2, 2, 2, 2, 2, 4 ),
 ( 0.02345095402629352246, 0.02491692321306682514, 0.02564990780645347995, 0.02638289239984013129, 0.02711587699322678263, 0.02784886158661343744, 0.02931483077338673318, 0.03004781536677338799, 0.03078079996016004280, 0.03224676914693334895, 0.03297975374032000723, 0.03371273833370666551, 0.03517870752047992655, 0.03664467670725320148, 0.03737766130063985281, 0.03811064589402650415, 0.03957661508079982071, 0.04104258426757313033, 0.04250855345434643995, 0.04324153804773310517, 0.04397452264111975651, 0.04544049182789308000, 0.04690646101466640350 ),
 .UNSPECIFIED. ) ;
#20057=CARTESIAN_POINT ( 'NONE',  ( 181.5079096844946491, 80.47139261082470796, 2.464043515047716681 ) ) ;
#20058=CARTESIAN_POINT ( 'NONE',  ( 212.1983751099433846, 117.2326047784726910, -43.68460009809672329 ) ) ;
#20059=CARTESIAN_POINT ( 'NONE',  ( 173.9288990958750105, 71.66475105971929338, 12.28611953004625335 ) ) ;
#20063=CARTESIAN_POINT ( 'NONE',  ( -72.77296415263759854, 21.23032531836537018, 60.09768903209150182 ) ) ;
#20064=CARTESIAN_POINT ( 'NONE',  ( 55.90910788310615231, 11.13585330978401089, -67.61777098659958085 ) ) ;
#20065=CARTESIAN_POINT ( 'NONE',  ( -77.02372450489323796, 21.70271995013166233, 3.751895169942434993 ) ) ;
#20067=CARTESIAN_POINT ( 'NONE',  ( -7.181048525087159184, 6.849049514988890586, 83.80408853790447665 ) ) ;
#20068=CARTESIAN_POINT ( 'NONE',  ( -106.7004823116342180, 36.22460663120047286, -9.592053525173668049 ) ) ;
#20072=CARTESIAN_POINT ( 'NONE',  ( -74.17694007417657076, 20.66176641130875424, 70.79032727487506804 ) ) ;
#20073=CARTESIAN_POINT ( 'NONE',  ( 197.8053004231843772, 97.34590015073870006, -94.51308478323058182 ) ) ;
#20077=CARTESIAN_POINT ( 'NONE',  ( 58.47673920847984874, 11.66523265296355305, -49.21114976423752552 ) ) ;
#20084=CARTESIAN_POINT ( 'NONE',  ( 211.7451286015360949, 116.5372661580811524, 12.44640788307098767 ) ) ;
#20085=DIRECTION ( 'NONE',  ( -0.000000000000000000, 1.000000000000000000, -0.000000000000000000 ) ) ;
#20086=CARTESIAN_POINT ( 'NONE',  ( 209.6877167158270652, 113.4449353909247407, 42.31176391386135549 ) ) ;
#20087=CARTESIAN_POINT ( 'NONE',  ( 15.78827728214693416, 6.500811158483322139, -89.20804527961313113 ) ) ;
#20094=CARTESIAN_POINT ( 'NONE',  ( -118.4463605755664446, 42.96013650986014909, 92.75845490717212272 ) ) ;
#20095=CARTESIAN_POINT ( 'NONE',  ( -165.7699288023689803, 79.30174988963861438, -16.88298621586212889 ) ) ;
#20097=EDGE_CURVE ( 'NONE', #57426, #56594, #67673, .T. ) ;
#20098=CARTESIAN_POINT ( 'NONE',  ( 22.82910978135140212, 6.828162702325536237, 93.80883881146230863 ) ) ;
#20099=CARTESIAN_POINT ( 'NONE',  ( 23.10675661028717087, 7.853421165986156360, 92.87640639569337964 ) ) ;
#20103=CARTESIAN_POINT ( 'NONE',  ( -96.00016893459647349, 29.70347032303887858, 68.97150621174834839 ) ) ;
#20105=CARTESIAN_POINT ( 'NONE',  ( -86.15275984831841072, 25.31588180512565600, 11.59364235127147680 ) ) ;
#20106=ORIENTED_EDGE ( 'NONE', *, *, #60738, .F. ) ;
#20107=CARTESIAN_POINT ( 'NONE',  ( -56.73868929054667376, 16.18382781951278915, -8.559674830497424836 ) ) ;
#20113=CARTESIAN_POINT ( 'NONE',  ( -108.9643850519886001, 37.45603458068514158, -92.79426669927697446 ) ) ;
#20115=CARTESIAN_POINT ( 'NONE',  ( 22.30016284075436417, 6.796348835713779124, 14.42317800662865146 ) ) ;
#20116=EDGE_LOOP ( 'NONE', ( #47534, #5599, #14221, #65561 ) ) ;
#20117=CARTESIAN_POINT ( 'NONE',  ( -38.04017048906806053, 10.76841555971077469, 87.83049671292886273 ) ) ;
#20118=CARTESIAN_POINT ( 'NONE',  ( 174.9099402067542997, 73.96774984027643995, -66.30337972617925857 ) ) ;
#20120=CARTESIAN_POINT ( 'NONE',  ( 109.3047266816501235, 28.44977739115299897, -50.87832046748908965 ) ) ;
#20121=CARTESIAN_POINT ( 'NONE',  ( 85.68197636629479064, 20.16141071296263831, -50.77689019393022818 ) ) ;
#20125=CARTESIAN_POINT ( 'NONE',  ( -83.13046924527391468, 25.15778674529014936, -75.49169951200217099 ) ) ;
#20126=CARTESIAN_POINT ( 'NONE',  ( 174.4978817191264966, 73.57770570413210010, 6.365850984605415874 ) ) ;
#20128=CARTESIAN_POINT ( 'NONE',  ( 15.78827728214693416, 6.500811158483327468, -35.51894409868578606 ) ) ;
#20130=CARTESIAN_POINT ( 'NONE',  ( -154.6171773099879374, 68.63761944777704116, 16.87154224365831467 ) ) ;
#20131=CARTESIAN_POINT ( 'NONE',  ( -118.6727642982647239, 43.09863379477472733, -71.35525363643188257 ) ) ;
#20132=CARTESIAN_POINT ( 'NONE',  ( 204.6977192012829789, 108.0580384837235073, 44.20772073876944575 ) ) ;
#20133=CARTESIAN_POINT ( 'NONE',  ( -80.31482177285907653, 24.03632224640839254, 57.44225315143493305 ) ) ;
#20135=ORIENTED_EDGE ( 'NONE', *, *, #36037, .T. ) ;
#20136=CARTESIAN_POINT ( 'NONE',  ( -53.51212025488904800, 15.31378391224928315, 84.15964359628104319 ) ) ;
#20137=ORIENTED_EDGE ( 'NONE', *, *, #2103, .T. ) ;
#20139=EDGE_LOOP ( 'NONE', ( #48631, #29658, #17355, #59448 ) ) ;
#20141=B_SPLINE_CURVE_WITH_KNOTS ( 'NONE', 3,
 ( #9630, #31088, #52528, #4351, #41973, #54942, #23306, #11333, #32803, #65517, #38424, #59172, #50021, #32456, #28210, #21890, #43685, #10992, #27513, #1855, #59514, #18018, #54233, #17312, #38783, #48602, #439, #16615, #60230, #44392, #22248, #60575, #59868, #38072, #49657, #44033, #54593, #11684, #7113, #12043, #27165, #6054, #43342, #65161 ),
 .UNSPECIFIED., .F., .F.,
 ( 4, 2, 2, 2, 2, 2, 2, 2, 2, 2, 2, 2, 2, 2, 2, 2, 2, 2, 2, 2, 2, 4 ),
 ( 6.938893903907228378E-18, 0.001488594467279747650, 0.002232891700919627329, 0.002977188934559507009, 0.004465783401839248587, 0.005954377869118990599, 0.007442972336398733478, 0.008187269570038610556, 0.008931566803678486766, 0.01042016127095824786, 0.01190875573823800895, 0.01265305297187786955, 0.01339735020551772841, 0.01488594467279744440, 0.01563024190643729980, 0.01637453914007715866, 0.01786313360735687292, 0.01935172807463658370, 0.02009602530827643563, 0.02084032254191628408, 0.02232891700919596364, 0.02381751147647563627 ),
 .UNSPECIFIED. ) ;
#20142=CARTESIAN_POINT ( 'NONE',  ( 16.77104078056616743, 7.540619757007628543, -62.41212509805560416 ) ) ;
#20147=CARTESIAN_POINT ( 'NONE',  ( 141.3586046882815026, 47.34625111366350581, -44.03220709178651049 ) ) ;
#20148=CARTESIAN_POINT ( 'NONE',  ( 33.44983424733137412, 7.709709042132400825, -38.53006481374713843 ) ) ;
#20150=CARTESIAN_POINT ( 'NONE',  ( 8.679939806240508204, 7.383357464882124077, -40.61437127068128916 ) ) ;
#20152=CARTESIAN_POINT ( 'NONE',  ( -120.5002574492098972, 44.22930148497321312, -10.35167903076605000 ) ) ;
#20158=CARTESIAN_POINT ( 'NONE',  ( -31.43908319763709969, 9.591432048623762086, -62.16174795566551836 ) ) ;
#20159=AXIS2_PLACEMENT_3D ( 'NONE', #26012, #63977, #47439 ) ;
#20160=CARTESIAN_POINT ( 'NONE',  ( 8.336031647119268584, 6.376437040857334537, 11.64877837691457607 ) ) ;
#20161=CARTESIAN_POINT ( 'NONE',  ( 43.35536254672140188, 9.973606330917814233, -76.34245829030946595 ) ) ;
#20164=CARTESIAN_POINT ( 'NONE',  ( -177.5259994307673423, 92.16784265327252967, -48.30003138184611089 ) ) ;
#20166=CARTESIAN_POINT ( 'NONE',  ( -27.70185240367227664, 10.02491413133431131, 58.05382884042261082 ) ) ;
#20169=CARTESIAN_POINT ( 'NONE',  ( -51.35181696773308602, 13.72007042346227479, 58.12010125874579103 ) ) ;
#20170=EDGE_CURVE ( 'NONE', #20616, #29587, #5371, .T. ) ;
#20175=CARTESIAN_POINT ( 'NONE',  ( 156.5890478960376697, 58.24007662587948175, 71.21522256953024055 ) ) ;
#20176=CARTESIAN_POINT ( 'NONE',  ( -103.2164890789475606, 34.39030697009940951, -61.90300353352128582 ) ) ;
#20181=CARTESIAN_POINT ( 'NONE',  ( -61.38706483483509402, 16.47181058798476272, 68.68523971831442054 ) ) ;
#20188=AXIS2_PLACEMENT_3D ( 'NONE', #43013, #21236, #26514 ) ;
#20191=CARTESIAN_POINT ( 'NONE',  ( 60.63380853769237433, 13.16344960520421914, -50.33659022662053673 ) ) ;
#20193=CARTESIAN_POINT ( 'NONE',  ( -85.95621526752228192, 26.32462117888284681, 36.13660444380358427 ) ) ;
#20195=AXIS2_PLACEMENT_3D ( 'NONE', #56694, #45796, #61627 ) ;
#20196=CARTESIAN_POINT ( 'NONE',  ( -30.46002654261637588, 10.45132580906818021, -23.42440563520737129 ) ) ;
#20198=EDGE_CURVE ( 'NONE', #6856, #47821, #34839, .T. ) ;
#20201=CARTESIAN_POINT ( 'NONE',  ( 8.683531412707433006, 6.377173148747124820, 66.77437832024716613 ) ) ;
#20202=CARTESIAN_POINT ( 'NONE',  ( -24.95029760921699591, 9.631514785009935409, 33.94725700252100609 ) ) ;
#20203=CARTESIAN_POINT ( 'NONE',  ( 204.3091227790962989, 107.5190503136782638, 44.20772073876946706 ) ) ;
#20204=CARTESIAN_POINT ( 'NONE',  ( -71.35453793101461883, 20.73435672776740191, 89.90586990597532235 ) ) ;
#20205=DIRECTION ( 'NONE',  ( 0.000000000000000000, 0.000000000000000000, 1.000000000000000000 ) ) ;
#20207=CARTESIAN_POINT ( 'NONE',  ( 68.62997155117722059, 15.08415013720828668, 42.30982577549439583 ) ) ;
#20208=ORIENTED_EDGE ( 'NONE', *, *, #30117, .F. ) ;
#20211=CARTESIAN_POINT ( 'NONE',  ( 113.4402889550712956, 31.50582881646778333, -63.46592719120694426 ) ) ;
#20216=CARTESIAN_POINT ( 'NONE',  ( -85.36298448216592760, 26.07611629625833771, -12.35578000808629184 ) ) ;
#20218=CARTESIAN_POINT ( 'NONE',  ( -151.2410113808308552, 65.66338888995502998, -49.62284842420343978 ) ) ;
#20219=ORIENTED_EDGE ( 'NONE', *, *, #8191, .T. ) ;
#20223=CARTESIAN_POINT ( 'NONE',  ( 116.9223627093533509, 32.09655261207334576, 87.37230592524522876 ) ) ;
#20225=FACE_OUTER_BOUND ( 'NONE', #68492, .T. ) ;
#20234=CARTESIAN_POINT ( 'NONE',  ( 174.1355634792904254, 71.85737575453710235, -94.55186492391756303 ) ) ;
#20239=CARTESIAN_POINT ( 'NONE',  ( 184.3879440808139805, 83.47316703125162007, 70.38978263608034069 ) ) ;
#20240=CARTESIAN_POINT ( 'NONE',  ( 46.58610174774756985, 9.452965170565081010, 88.92390424605549981 ) ) ;
#20243=CARTESIAN_POINT ( 'NONE',  ( 22.51849650178395734, 7.817407610814552044, 13.98895852407905949 ) ) ;
#20247=CARTESIAN_POINT ( 'NONE',  ( 133.3990214534116774, 41.14886683286415803, -24.16826940798425838 ) ) ;
#20250=CARTESIAN_POINT ( 'NONE',  ( 11.20486344102687504, 7.403248964808827104, 16.62706366644169620 ) ) ;
#20252=B_SPLINE_CURVE_WITH_KNOTS ( 'NONE', 3,
 ( #38371, #5330, #42941, #64411, #10942, #44340, #38730, #1093, #16220, #22199, #64762, #32413, #59816, #386, #11631, #33105, #53838, #49609, #60174, #10590, #745, #5657, #27463, #27117, #6003, #54891, #27822, #48212, #54541, #37, #37674, #6368, #65825, #43287, #11995, #43637, #21842, #1442, #17258, #48907, #65114, #17619, #22895, #59121 ),
 .UNSPECIFIED., .F., .F.,
 ( 4, 2, 2, 2, 2, 2, 2, 2, 2, 2, 2, 2, 2, 2, 2, 2, 2, 2, 2, 2, 2, 4 ),
 ( 0.02908143158676655682, 0.03095422299093871302, 0.03282701439511086922, 0.03469980579928302888, 0.03657259720345518855, 0.03844538860762734822, 0.04031818001179950095, 0.04125457571388553568, 0.04219097141597157041, 0.04312736711805760514, 0.04359556496910062251, 0.04406376282014363988, 0.04500015852222963991, 0.04593655422431563301, 0.04687294992640163305, 0.04780934562848762615, 0.04968213703265959846, 0.05155492843683157078, 0.05342771984100353616, 0.05530051124517551542, 0.05717330264934748080, 0.05904609405351945312 ),
 .UNSPECIFIED. ) ;
#20255=CARTESIAN_POINT ( 'NONE',  ( 188.4937788906148626, 86.43336847120863808, 11.16285860195706547 ) ) ;
#20258=CARTESIAN_POINT ( 'NONE',  ( 181.0840389613909736, 78.60582251573003987, 44.30859410551141764 ) ) ;
#20260=CARTESIAN_POINT ( 'NONE',  ( 41.80536115778102868, 8.734184316430667394, -77.07306109708069641 ) ) ;
#20261=CARTESIAN_POINT ( 'NONE',  ( 187.8973304652193121, 87.27378997243174297, -46.87199284111774489 ) ) ;
#20264=CARTESIAN_POINT ( 'NONE',  ( -144.2029146819478456, 59.80706661873674790, -10.14434587346329941 ) ) ;
#20267=CARTESIAN_POINT ( 'NONE',  ( 113.4493678088378346, 30.39339414805073858, 70.75222796080394971 ) ) ;
#20269=LINE ( 'NONE', #31188, #42423 ) ;
#20274=CARTESIAN_POINT ( 'NONE',  ( -94.84390436305045569, 29.16104988397310649, 39.02940028697720010 ) ) ;
#20275=DIRECTION ( 'NONE',  ( -0.000000000000000000, 1.000000000000000000, -0.000000000000000000 ) ) ;
#20281=EDGE_LOOP ( 'NONE', ( #37278, #60625, #30752, #12668, #20539, #41970, #18810, #40398, #2655, #33761, #63561, #57088, #68848, #68555, #2199, #64811, #31459, #25249, #59345, #46386, #286, #58587, #63518, #7742, #50002, #34406, #13133, #11899, #54738, #31033, #27385, #13289, #199, #10105, #47474, #7792, #55812, #18357, #40839, #54854, #25541, #399, #12259, #67096, #11456, #17846, #6000, #328, #53511, #67037, #22984, #25385, #13119, #16307, #30866, #41677, #67961, #67914, #26810, #53976, #3980, #57386, #62090, #37072, #22605, #5589, #30235, #58414, #7781, #1438, #49355, #28087, #5216, #8343, #43184, #35787, #28207, #56033, #66348, #7999, #43612, #63451, #42804, #27688, #29484, #32087, #35128, #20038, #66450, #21606, #59894, #34253, #38893, #4818, #44610, #39374, #7954, #29111, #47637, #36139, #53897, #64557, #57727 ) ) ;
#20282=CARTESIAN_POINT ( 'NONE',  ( -123.4531143159639441, 44.90777521523904880, -22.66459338198712103 ) ) ;
#20284=CARTESIAN_POINT ( 'NONE',  ( -176.3896317155480062, 90.84057090619018027, -22.13191603966969012 ) ) ;
#20285=CARTESIAN_POINT ( 'NONE',  ( -133.3316503378477762, 52.82738260200863323, 63.86119459864413272 ) ) ;
#20287=CARTESIAN_POINT ( 'NONE',  ( -107.7144780656001330, 36.77195912774744357, 86.50315365870005735 ) ) ;
#20289=ORIENTED_EDGE ( 'NONE', *, *, #64654, .F. ) ;
#20291=CARTESIAN_POINT ( 'NONE',  ( -133.1640943168118554, 52.70734926280009347, -67.39673842532138792 ) ) ;
#20292=CARTESIAN_POINT ( 'NONE',  ( 60.23839536713451537, 12.04563565271882908, -89.93993854489507100 ) ) ;
#20294=CARTESIAN_POINT ( 'NONE',  ( 64.94098077424392557, 14.16208887966257102, -77.33007373951066654 ) ) ;
#20298=CARTESIAN_POINT ( 'NONE',  ( 181.9406741394861911, 79.47484497224795064, -63.10656098916969370 ) ) ;
#20299=CARTESIAN_POINT ( 'NONE',  ( -169.1005390226459326, 82.76152663947085841, -35.86510333151966279 ) ) ;
#20301=CARTESIAN_POINT ( 'NONE',  ( 103.1695711638930817, 26.83837309506524704, -72.81073785818523447 ) ) ;
#20302=CARTESIAN_POINT ( 'NONE',  ( -73.80418150970713498, 21.59712875466422588, 32.18635260252404606 ) ) ;
#20304=CARTESIAN_POINT ( 'NONE',  ( 66.73467315386238852, 14.60276727483218906, -36.68961546505575200 ) ) ;
#20306=CARTESIAN_POINT ( 'NONE',  ( -171.4867114763004281, 85.32693843184998173, -76.38800489763023904 ) ) ;
#20307=EDGE_CURVE ( 'NONE', #18940, #52822, #10498, .T. ) ;
#20309=CARTESIAN_POINT ( 'NONE',  ( -107.0584934212648420, 35.27493744466473657, -9.868436795408833007 ) ) ;
#20312=CARTESIAN_POINT ( 'NONE',  ( -180.5312359056721618, 95.77409857860999409, -94.70578744242111213 ) ) ;
#20314=CARTESIAN_POINT ( 'NONE',  ( 79.37778929114111293, 18.12554302172301490, 66.03557851574602466 ) ) ;
#20316=CARTESIAN_POINT ( 'NONE',  ( -189.2826425734429279, 107.1493800926106275, -68.08208096063634684 ) ) ;
#20320=FACE_OUTER_BOUND ( 'NONE', #47499, .T. ) ;
#20322=CARTESIAN_POINT ( 'NONE',  ( -38.92718193365331558, 11.96647478777219931, -15.48328760661300052 ) ) ;
#20328=CARTESIAN_POINT ( 'NONE',  ( -189.7334103489410495, 107.7745063523401257, 8.881755487159328055 ) ) ;
#20330=CARTESIAN_POINT ( 'NONE',  ( -14.55390976651257873, 7.422979442794215288, -73.08496616077771080 ) ) ;
#20331=CARTESIAN_POINT ( 'NONE',  ( -101.3492134984965531, 32.31003911421601060, -8.213220048528352635 ) ) ;
#20332=CARTESIAN_POINT ( 'NONE',  ( 156.5890478960376413, 58.24007662587944623, -36.16297979232447091 ) ) ;
#20333=EDGE_CURVE ( 'NONE', #55323, #39717, #29669, .T. ) ;
#20335=ORIENTED_EDGE ( 'NONE', *, *, #42565, .T. ) ;
#20338=CARTESIAN_POINT ( 'NONE',  ( 175.0696098417091378, 74.11936424544842339, -21.36851627469916082 ) ) ;
#20341=ORIENTED_EDGE ( 'NONE', *, *, #1502, .F. ) ;
#20342=CARTESIAN_POINT ( 'NONE',  ( -179.2128128997734962, 95.75254520622995358, -73.46006140737962653 ) ) ;
#20343=CARTESIAN_POINT ( 'NONE',  ( -2.355184675731021304, 6.596450510445342807, -21.21029824059963786 ) ) ;
#20344=CARTESIAN_POINT ( 'NONE',  ( 113.4351684956570523, 30.38657459074490319, 30.30815483564448343 ) ) ;
#20348=CARTESIAN_POINT ( 'NONE',  ( 199.7255144154428592, 99.76581417577200739, 31.07377068937141473 ) ) ;
#20349=CARTESIAN_POINT ( 'NONE',  ( 116.5096233816161941, 31.89062767870469983, -74.39514096115526343 ) ) ;
#20350=CARTESIAN_POINT ( 'NONE',  ( 188.5651904823862424, 88.01586411309099844, 37.41956129399849829 ) ) ;
#20356=CARTESIAN_POINT ( 'NONE',  ( 174.6307688320643479, 73.70327352127002030, 59.82234444106918403 ) ) ;
#20359=CARTESIAN_POINT ( 'NONE',  ( -109.3553681454883844, 36.52260784104392854, -45.05470719201598229 ) ) ;
#20360=CARTESIAN_POINT ( 'NONE',  ( 136.3708086338960470, 42.96321442892168818, 83.62629360459338557 ) ) ;
#20361=CARTESIAN_POINT ( 'NONE',  ( -62.53989795537026453, 16.81768094534200131, 38.32257745060478982 ) ) ;
#20362=CARTESIAN_POINT ( 'NONE',  ( 151.8005253678161921, 54.62151558044536159, 5.128849957095197531 ) ) ;
#20364=CARTESIAN_POINT ( 'NONE',  ( 160.9099843287285125, 61.67000084894969092, -50.30479636640266961 ) ) ;
#20366=DIRECTION ( 'NONE',  ( -0.000000000000000000, 1.000000000000000000, -0.000000000000000000 ) ) ;
#20370=CARTESIAN_POINT ( 'NONE',  ( -149.5074843970971301, 64.17983161892345834, -49.81283053149198992 ) ) ;
#20373=CARTESIAN_POINT ( 'NONE',  ( -180.6215424137752450, 97.48070480470856580, 38.62763768963357336 ) ) ;
#20374=CARTESIAN_POINT ( 'NONE',  ( 150.8925291903903769, 52.71218673668931132, 60.11153687441628080 ) ) ;
#20377=CARTESIAN_POINT ( 'NONE',  ( 45.89268866913128875, 10.36133864615985622, 14.33506431777695056 ) ) ;
#20378=ORIENTED_EDGE ( 'NONE', *, *, #19931, .F. ) ;
#20379=CARTESIAN_POINT ( 'NONE',  ( 154.0515132159917471, 56.29926936869308918, -23.47126196184992253 ) ) ;
#20380=ADVANCED_FACE ( 'NONE', ( #17509 ), #285, .F. ) ;
#20381=CARTESIAN_POINT ( 'NONE',  ( 210.9631450001600683, 117.1791136960929265, -21.14097324130973377 ) ) ;
#20382=CARTESIAN_POINT ( 'NONE',  ( 102.7446498997619955, 26.65764321315730001, 36.57460656155974021 ) ) ;
#20383=CARTESIAN_POINT ( 'NONE',  ( -156.0171627975467743, 69.90368824761765154, -65.42354838375587178 ) ) ;
#20385=CARTESIAN_POINT ( 'NONE',  ( 188.5653887627527752, 88.01608521313129074, 9.354702516507275689 ) ) ;
#20386=CARTESIAN_POINT ( 'NONE',  ( 211.5066273949819333, 116.1727691518061789, -47.01952303312400971 ) ) ;
#20393=CARTESIAN_POINT ( 'NONE',  ( -73.10086105983764071, 21.34631349770505082, 69.81410049433821996 ) ) ;
#20394=CARTESIAN_POINT ( 'NONE',  ( 61.33627421985469397, 12.28939706835343237, -62.75169496998579888 ) ) ;
#20397=EDGE_CURVE ( 'NONE', #20568, #27916, #32999, .T. ) ;
#20398=CARTESIAN_POINT ( 'NONE',  ( -0.4830416248186119588, 6.524023950717643849, 92.86839907411122397 ) ) ;
#20400=CARTESIAN_POINT ( 'NONE',  ( -109.7079446832838983, 37.86719386855315861, -16.74036298271016321 ) ) ;
#20401=VERTEX_POINT ( 'NONE', #44598 ) ;
#20403=CARTESIAN_POINT ( 'NONE',  ( -78.66644367742109978, 22.32174330031321574, 72.26275173013684139 ) ) ;
#20405=ORIENTED_EDGE ( 'NONE', *, *, #21832, .F. ) ;
#20407=CARTESIAN_POINT ( 'NONE',  ( -152.9119739516381458, 67.12135129037712034, 31.52259186888439046 ) ) ;
#20408=CARTESIAN_POINT ( 'NONE',  ( 56.19513604272050600, 11.19349063094192509, -40.09155741990996802 ) ) ;
#20413=LINE ( 'NONE', #53098, #1623 ) ;
#20417=CARTESIAN_POINT ( 'NONE',  ( -131.6253556217205016, 51.61436399519948282, 33.25658671114208431 ) ) ;
#20419=CARTESIAN_POINT ( 'NONE',  ( 212.1707951106656935, 117.1901534358505614, 10.52110880440418939 ) ) ;
#20420=CARTESIAN_POINT ( 'NONE',  ( -142.9843132609582597, 60.12226089556227748, 41.93116989061249456 ) ) ;
#20421=CARTESIAN_POINT ( 'NONE',  ( 209.6525588430077960, 113.3929734759396837, 31.07261694010716013 ) ) ;
#20426=CARTESIAN_POINT ( 'NONE',  ( -133.1325180892867479, 52.68453899796251250, 89.73671469607783990 ) ) ;
#20427=DIRECTION ( 'NONE',  ( 0.000000000000000000, 0.000000000000000000, 1.000000000000000000 ) ) ;
#20429=CARTESIAN_POINT ( 'NONE',  ( 20.62507889231323688, 6.703605479764012998, 85.46244512927005132 ) ) ;
#20430=CARTESIAN_POINT ( 'NONE',  ( 15.13717264782866145, 7.486582872045924653, 83.70339063347323361 ) ) ;
#20433=CARTESIAN_POINT ( 'NONE',  ( 203.1414537950835779, 105.9225671689748367, -36.47858528242302611 ) ) ;
#20435=CARTESIAN_POINT ( 'NONE',  ( -81.00507684688702170, 23.22613445438389235, 18.20370096348767319 ) ) ;
#20437=CARTESIAN_POINT ( 'NONE',  ( -125.8938041572051389, -170.0000000000000000, 30.61994787315706290 ) ) ;
#20438=EDGE_LOOP ( 'NONE', ( #53088, #33098, #33087, #38795 ) ) ;
#20441=CARTESIAN_POINT ( 'NONE',  ( -118.7011544766493500, 43.11604763363182968, 13.41670242813880876 ) ) ;
#20442=CARTESIAN_POINT ( 'NONE',  ( -180.0179082103088319, 95.14811732286298707, 68.12739521910877727 ) ) ;
#20443=CARTESIAN_POINT ( 'NONE',  ( 128.4224537826254675, 38.23837035195749223, 69.04676071552452754 ) ) ;
#20446=B_SPLINE_CURVE_WITH_KNOTS ( 'NONE', 3,
 ( #66085, #1347, #22801, #65727, #17876, #33716, #40370, #68156, #29127, #3430, #8722, #45295, #66780, #19605, #14340, #46680, #51961, #30508, #25244, #35092, #19965, #13637, #13305, #41416, #24556, #8015, #62163, #41066, #30172, #56544, #29818, #40707, #3772, #19253, #50577, #62525 ),
 .UNSPECIFIED., .F., .F.,
 ( 4, 2, 2, 2, 2, 2, 2, 2, 2, 2, 2, 2, 2, 2, 2, 2, 2, 4 ),
 ( 3.469446951953614189E-18, 0.001545474820159074576, 0.003090949640318145682, 0.004636424460477216354, 0.006181899280636287894, 0.007727374100795359434, 0.008500111510874878290, 0.009272848920954396279, 0.01081832374111341144, 0.01236379856127242660, 0.01390927338143144350, 0.01545474820159046039, 0.01700022302174947555, 0.01854569784190849072, 0.02009117266206750935, 0.02163664748222652451, 0.02318212230238554314, 0.02472759712254455483 ),
 .UNSPECIFIED. ) ;
#20450=CARTESIAN_POINT ( 'NONE',  ( -37.14089062983303080, 10.59660406339133942, 86.49034957900197185 ) ) ;
#20455=CARTESIAN_POINT ( 'NONE',  ( -24.33435124463266419, 8.532637995283112176, 40.13176205844700206 ) ) ;
#20456=CARTESIAN_POINT ( 'NONE',  ( -146.1201263095600780, 62.66021356509617135, -62.46206482111294633 ) ) ;
#20460=CARTESIAN_POINT ( 'NONE',  ( -83.51110947562230535, 25.31252704029285283, -75.19045686144863794 ) ) ;
#20461=CARTESIAN_POINT ( 'NONE',  ( -7.825402957745085430, 6.891034867348153625, -89.10717191287116634 ) ) ;
#20464=CARTESIAN_POINT ( 'NONE',  ( 130.7260704202055024, 39.56565398554880630, 3.334336834773580005 ) ) ;
#20465=CARTESIAN_POINT ( 'NONE',  ( 36.19799081159146681, 8.014391982702079531, -90.02455723444843727 ) ) ;
#20466=CARTESIAN_POINT ( 'NONE',  ( -120.5002574492099114, 44.22930148497321312, -64.04078021169341639 ) ) ;
#20468=CARTESIAN_POINT ( 'NONE',  ( 39.40195752203891999, 9.424259417798145577, 71.75838489642698903 ) ) ;
#20469=CARTESIAN_POINT ( 'NONE',  ( 164.3577270662354124, 63.21061577643033758, 7.084215918832702741 ) ) ;
#20470=CARTESIAN_POINT ( 'NONE',  ( -105.4589068214114178, 34.42476264325678414, 31.20975402820559808 ) ) ;
#20473=CARTESIAN_POINT ( 'NONE',  ( -47.88727290496198208, 13.91049128144765490, 93.81492665685888710 ) ) ;
#20477=CYLINDRICAL_SURFACE ( 'NONE', #7403, 7.500000000000020428 ) ;
#20479=CARTESIAN_POINT ( 'NONE',  ( -168.7329347389695897, 83.83901812802763232, 32.22089368191161185 ) ) ;
#20482=CARTESIAN_POINT ( 'NONE',  ( 140.9141742510256563, 47.05414327990549594, -46.11397078288850082 ) ) ;
#20483=CARTESIAN_POINT ( 'NONE',  ( 34.83825437341841535, 7.859462995505741567, -49.09150060942670990 ) ) ;
#20491=CARTESIAN_POINT ( 'NONE',  ( -170.2951623264597458, 85.51757001115473145, -8.407365705316680149 ) ) ;
#20492=ADVANCED_FACE ( 'NONE', ( #27362 ), #59375, .F. ) ;
#20499=CARTESIAN_POINT ( 'NONE',  ( 177.2011275744679324, 74.76848439756734876, -76.99017118353420130 ) ) ;
#20502=CARTESIAN_POINT ( 'NONE',  ( -178.2427210808090479, 93.01567669683340966, -47.69625270927920013 ) ) ;
#20512=FACE_OUTER_BOUND ( 'NONE', #21296, .T. ) ;
#20513=CARTESIAN_POINT ( 'NONE',  ( -0.3234390959946896738, 7.525307474706613320, 91.58024944812166268 ) ) ;
#20514=ORIENTED_EDGE ( 'NONE', *, *, #61635, .T. ) ;
#20519=CARTESIAN_POINT ( 'NONE',  ( 38.76018190153303067, 9.341091693823624809, 83.62323164182360813 ) ) ;
#20520=CARTESIAN_POINT ( 'NONE',  ( 39.40195752203892710, -170.0000000000000000, 64.25838489642696061 ) ) ;
#20525=CARTESIAN_POINT ( 'NONE',  ( 35.65685430025423841, 7.951642554322390311, -9.758845964438441101 ) ) ;
#20528=CARTESIAN_POINT ( 'NONE',  ( 93.09528872995971938, 21.72934119836186184, 41.04433854226019918 ) ) ;
#20533=CARTESIAN_POINT ( 'NONE',  ( 13.84120792123769128, 6.445822122644895735, 57.09985721401838532 ) ) ;
#20535=CARTESIAN_POINT ( 'NONE',  ( 197.4121679705848180, 98.46451029407253941, 34.92010124187357434 ) ) ;
#20536=CARTESIAN_POINT ( 'NONE',  ( -71.21425542757401672, 20.68582981242713359, 92.51412664241122741 ) ) ;
#20539=ORIENTED_EDGE ( 'NONE', *, *, #21591, .F. ) ;
#20543=CARTESIAN_POINT ( 'NONE',  ( 116.5100763992442836, 33.01539745157281658, -66.13966895617740249 ) ) ;
#20544=CARTESIAN_POINT ( 'NONE',  ( 8.000000000000007105, 249.8719672152120381, 94.99999999999866418 ) ) ;
#20545=CARTESIAN_POINT ( 'NONE',  ( 203.9181091394788155, 105.2759068139671683, -63.17048162308529413 ) ) ;
#20549=EDGE_CURVE ( 'NONE', #31339, #29832, #12859, .T. ) ;
#20550=CARTESIAN_POINT ( 'NONE',  ( 204.6977192012829789, -170.0000000000000000, -16.98138044215791354 ) ) ;
#20552=CARTESIAN_POINT ( 'NONE',  ( 21.64175105888077510, 7.766279958615638357, -92.00052844524886098 ) ) ;
#20554=CARTESIAN_POINT ( 'NONE',  ( -154.0718453320783681, 68.14976693162391541, -48.26858095381671632 ) ) ;
#20559=CARTESIAN_POINT ( 'NONE',  ( -85.95621526752229613, 26.32462117888285746, -44.39704732758743688 ) ) ;
#20561=CARTESIAN_POINT ( 'NONE',  ( 105.4886448962878660, 26.74369472770962020, 84.99022211379437408 ) ) ;
#20563=CARTESIAN_POINT ( 'NONE',  ( -156.1477286774994298, 71.38742644140636173, 14.87326405071225111 ) ) ;
#20568=VERTEX_POINT ( 'NONE', #27194 ) ;
#20580=CARTESIAN_POINT ( 'NONE',  ( 10.13846145460683168, 6.385368868491634764, -11.21767487839372279 ) ) ;
#20581=CARTESIAN_POINT ( 'NONE',  ( 20.35964562795320276, 7.697260051881319676, 16.63611903121913826 ) ) ;
#20582=CARTESIAN_POINT ( 'NONE',  ( 186.6054783416232112, 84.37128553200973613, 58.55262771499806718 ) ) ;
#20583=CARTESIAN_POINT ( 'NONE',  ( -118.9468627709229196, 42.08677365399179848, 14.11409130223153774 ) ) ;
#20584=CARTESIAN_POINT ( 'NONE',  ( 70.11438327604405174, 14.43198353181101368, -67.63221911897893790 ) ) ;
#20586=CARTESIAN_POINT ( 'NONE',  ( 23.04797191264876588, 7.849755664016359269, -18.12056745251717871 ) ) ;
#20590=CARTESIAN_POINT ( 'NONE',  ( 188.2988323915788840, 86.21831227955483712, 12.03370908765665170 ) ) ;
#20592=CARTESIAN_POINT ( 'NONE',  ( 174.6127059037622189, 72.30368563770912260, 32.97823390021704881 ) ) ;
#20594=CARTESIAN_POINT ( 'NONE',  ( -104.1225399044495816, 34.86084180570099278, -49.78854814781668381 ) ) ;
#20595=CARTESIAN_POINT ( 'NONE',  ( 182.7745872728868335, 81.77554423487160307, -36.36768213514671544 ) ) ;
#20597=VECTOR ( 'NONE', #32601, 1000.000000000000000 ) ;
#20601=CARTESIAN_POINT ( 'NONE',  ( 175.0857681883884140, 72.74906374897946648, 94.99999999999866418 ) ) ;
#20604=CARTESIAN_POINT ( 'NONE',  ( 112.1012908502484464, 29.75117929736500955, 56.68578264432271396 ) ) ;
#20607=PLANE ( 'NONE',  #64326 ) ;
#20611=CARTESIAN_POINT ( 'NONE',  ( 158.2025576483179066, 58.22064626730321635, -89.81328548006500512 ) ) ;
#20612=CARTESIAN_POINT ( 'NONE',  ( 86.62931800182293784, 19.42108912189597092, -50.82156419891174437 ) ) ;
#20616=VERTEX_POINT ( 'NONE', #67798 ) ;
#20618=CARTESIAN_POINT ( 'NONE',  ( -119.6995109608660783, 42.54844499216735443, -19.80530726453818957 ) ) ;
#20619=ADVANCED_FACE ( 'NONE', ( #35789 ), #19597, .F. ) ;
#20621=CARTESIAN_POINT ( 'NONE',  ( -180.4654253355436992, 95.69358270527510513, -16.91796665578175052 ) ) ;
#20627=B_SPLINE_CURVE_WITH_KNOTS ( 'NONE', 3,
 ( #10260, #48560, #47532, #5339, #394, #26794, #48220, #45, #57771, #4310, #47201, #64419, #68659, #15202, #16230, #20469, #9930, #52817, #68995, #20820, #42279, #54549, #28887, #39098, #2157, #6012, #1811, #27472, #22208, #23610, #55253, #54899, #33116, #43997, #6723, #48915, #65475, #23265, #6376, #32762, #753, #11639, #28168, #27830 ),
 .UNSPECIFIED., .F., .F.,
 ( 4, 2, 2, 2, 2, 2, 2, 2, 2, 2, 2, 2, 2, 2, 2, 2, 2, 2, 2, 2, 2, 4 ),
 ( 0.02638217555535139064, 0.02805347641364862310, 0.02972477727194585209, 0.03139607813024308108, 0.03306737898854031354, 0.03390302941768895406, 0.03473867984683759458, 0.03640998070513487561, 0.03724563113428349531, 0.03808128156343210807, 0.03891693199258072083, 0.03975258242172934053, 0.04058823285087795329, 0.04142388328002657299, 0.04225953370917518576, 0.04309518413832380546, 0.04476648499662103098, 0.04643778585491824956, 0.04810908671321547508, 0.04978038757151270061, 0.05145168842980992613, 0.05312298928810715165 ),
 .UNSPECIFIED. ) ;
#20628=CARTESIAN_POINT ( 'NONE',  ( -59.36813706141739289, 15.88103696331960890, -9.732856487797739931 ) ) ;
#20632=CARTESIAN_POINT ( 'NONE',  ( -128.9843070188473177, 49.78011598923035308, -76.10710841746416122 ) ) ;
#20633=VECTOR ( 'NONE', #17576, 1000.000000000000000 ) ;
#20635=CARTESIAN_POINT ( 'NONE',  ( -131.6399667378751133, 51.62465701391629835, 16.12153412855955636 ) ) ;
#20636=CARTESIAN_POINT ( 'NONE',  ( -96.76159256735191150, 30.06445763698411255, -64.25652613276936620 ) ) ;
#20637=ORIENTED_EDGE ( 'NONE', *, *, #23312, .F. ) ;
#20638=ORIENTED_EDGE ( 'NONE', *, *, #60121, .T. ) ;
#20641=CARTESIAN_POINT ( 'NONE',  ( 185.1802655733641245, 82.84606286178498635, -64.27098958697960995 ) ) ;
#20642=CARTESIAN_POINT ( 'NONE',  ( -166.2028193222419077, 79.74385139484274987, -45.12230103603525322 ) ) ;
#20643=CARTESIAN_POINT ( 'NONE',  ( -125.8938041572051389, -170.0000000000000000, -42.41370389823394760 ) ) ;
#20646=CARTESIAN_POINT ( 'NONE',  ( 105.2529848321548229, 27.73895015262023023, -75.87138210954954332 ) ) ;
#20647=CARTESIAN_POINT ( 'NONE',  ( -72.77296415263764118, 21.23032531836537018, 33.25313844162783283 ) ) ;
#20648=CARTESIAN_POINT ( 'NONE',  ( 79.38459371357853911, 17.07499996355401350, 39.21690604770069655 ) ) ;
#20649=CARTESIAN_POINT ( 'NONE',  ( 64.69738688745236743, 14.10375742873388027, -35.90769066738622683 ) ) ;
#20650=VECTOR ( 'NONE', #12538, 1000.000000000000000 ) ;
#20651=CARTESIAN_POINT ( 'NONE',  ( -118.4106078162223525, 42.93830006159888057, 38.68969896642374096 ) ) ;
#20655=CARTESIAN_POINT ( 'NONE',  ( -108.6909373351217454, 36.15835109565441741, -19.59438147849856549 ) ) ;
#20657=CARTESIAN_POINT ( 'NONE',  ( 85.05043445648591671, 19.94792874060193100, -89.63462324852685015 ) ) ;
#20659=CARTESIAN_POINT ( 'NONE',  ( 81.04027388895740103, 18.64386073872848115, 69.08189960584093114 ) ) ;
#20664=CARTESIAN_POINT ( 'NONE',  ( 31.90217595456442368, 7.552213897210514837, -69.47029962155583860 ) ) ;
#20668=EDGE_CURVE ( 'NONE', #49023, #52035, #29494, .T. ) ;
#20672=CARTESIAN_POINT ( 'NONE',  ( 55.91133443650747381, 12.16263767238153726, 61.70338409828477921 ) ) ;
#20673=CARTESIAN_POINT ( 'NONE',  ( 14.81290967676422454, 7.477658233646010011, -77.31609961694144317 ) ) ;
#20675=EDGE_CURVE ( 'NONE', #40831, #988, #63182, .T. ) ;
#20678=CARTESIAN_POINT ( 'NONE',  ( -55.90340863576495423, 14.91086451836061677, -88.94171492579830840 ) ) ;
#20680=CARTESIAN_POINT ( 'NONE',  ( 150.2941978382489197, 53.52137138947629325, -45.82117147580458294 ) ) ;
#20683=CARTESIAN_POINT ( 'NONE',  ( -149.9475539515598825, 65.87716206616011050, 72.56537183036279259 ) ) ;
#20686=CARTESIAN_POINT ( 'NONE',  ( -129.3970594949620079, 50.06339481638098476, -49.06162375837405420 ) ) ;
#20688=DIRECTION ( 'NONE',  ( -0.000000000000000000, 1.000000000000000000, -0.000000000000000000 ) ) ;
#20689=CARTESIAN_POINT ( 'NONE',  ( 94.02921784728462740, 22.08005910033070762, 65.30351108513647773 ) ) ;
#20690=CARTESIAN_POINT ( 'NONE',  ( 200.8303160266298732, 102.8412051751308667, -10.54118182323272634 ) ) ;
#20691=CARTESIAN_POINT ( 'NONE',  ( -146.9398925983290951, 62.03096887829646988, 84.84101267915092137 ) ) ;
#20695=CARTESIAN_POINT ( 'NONE',  ( 198.2545923567585362, 97.90679023593578734, 32.85835692444881317 ) ) ;
#20698=CARTESIAN_POINT ( 'NONE',  ( 188.4920037102894526, 87.93425473911918289, 38.01812594245322430 ) ) ;
#20699=CARTESIAN_POINT ( 'NONE',  ( 164.0105905242218398, 64.23277447906893656, 6.384859283288245813 ) ) ;
#20700=CARTESIAN_POINT ( 'NONE',  ( -101.8140949286062238, 33.67224128592400945, 45.51907450641512298 ) ) ;
#20706=CARTESIAN_POINT ( 'NONE',  ( 173.8623159076319382, 72.97967239795016781, 61.60855493920503534 ) ) ;
#20709=CARTESIAN_POINT ( 'NONE',  ( -109.6660553119435377, 36.69391917620600196, -41.18609763443000560 ) ) ;
#20710=ADVANCED_FACE ( 'NONE', ( #50667 ), #40121, .F. ) ;
#20711=CARTESIAN_POINT ( 'NONE',  ( 64.69649025047539226, 13.06878919510322312, -77.37851346046119261 ) ) ;
#20713=DIRECTION ( 'NONE',  ( 0.000000000000000000, 0.000000000000000000, 1.000000000000000000 ) ) ;
#20716=CARTESIAN_POINT ( 'NONE',  ( -174.7800083645696532, 88.99302808536934606, 30.99548995540544638 ) ) ;
#20718=CARTESIAN_POINT ( 'NONE',  ( 114.6659427952414347, 32.10199811723106933, -37.34674998934434598 ) ) ;
#20720=B_SPLINE_CURVE_WITH_KNOTS ( 'NONE', 3,
 ( #67513, #43173, #37559, #58319, #57988, #64650, #69222, #52694, #37211, #16105, #53379, #10138, #4861, #15764, #48431, #63952, #25650, #59012, #9807, #42154, #31597, #68544, #10828, #268, #53727, #58662, #36884, #32297, #15077, #10479, #5549, #27002, #31267, #21723, #16457, #37912, #36539, #53037, #68869, #4521, #41814, #25984, #59357 ),
 .UNSPECIFIED., .F., .F.,
 ( 4, 2, 2, 2, 2, 2, 2, 2, 2, 2, 2, 1, 2, 2, 2, 2, 2, 2, 2, 2, 2, 4 ),
 ( 0.02515559250233026511, 0.02674001423437960545, 0.02753222510040427562, 0.02832443596642894579, 0.02990885769847835204, 0.03149327943052775830, 0.03307770116257716109, 0.03386991202860185901, 0.03466212289462655693, 0.03624654462667591809, 0.03703875549270058826, 0.03783096635872525842, 0.03862317722474992859, 0.03941538809077459876, 0.04099980982282395992, 0.04258423155487331413, 0.04337644242089799818, 0.04416865328692266834, 0.04575307501897196011, 0.04733749675102125187, 0.04892191848307053670, 0.05050634021511982846 ),
 .UNSPECIFIED. ) ;
#20724=CARTESIAN_POINT ( 'NONE',  ( 140.9169160367233076, 45.85398962664667977, 66.43883726660729394 ) ) ;
#20725=CARTESIAN_POINT ( 'NONE',  ( -171.0758681675584683, 84.87997360100517596, 45.54985601431179276 ) ) ;
#20726=CARTESIAN_POINT ( 'NONE',  ( -31.43908319763709969, 9.591432048623762086, -62.16174795566551836 ) ) ;
#20728=CARTESIAN_POINT ( 'NONE',  ( 87.11239765416381431, 20.65008247340817604, 44.71208757247934074 ) ) ;
#20731=EDGE_CURVE ( 'NONE', #48266, #33282, #246, .T. ) ;
#20734=CARTESIAN_POINT ( 'NONE',  ( -57.54234552050026963, 15.36296824409563477, 84.42464098905453795 ) ) ;
#20736=CARTESIAN_POINT ( 'NONE',  ( -156.9910258076866114, 70.79617246506502681, -69.73103036517183284 ) ) ;
#20739=CARTESIAN_POINT ( 'NONE',  ( 206.7099580236350107, 109.1417833474364585, -36.58928946998770471 ) ) ;
#20746=CARTESIAN_POINT ( 'NONE',  ( 205.5004956747122833, 107.4493581495447785, -78.13833085385769550 ) ) ;
#20747=CARTESIAN_POINT ( 'NONE',  ( 55.76298701799386492, 11.10663440745151398, -68.09037621486923797 ) ) ;
#20750=FACE_OUTER_BOUND ( 'NONE', #38432, .T. ) ;
#20751=CARTESIAN_POINT ( 'NONE',  ( 161.1112535418156710, 61.83422628788726882, -63.90774190170210289 ) ) ;
#20752=ORIENTED_EDGE ( 'NONE', *, *, #8743, .T. ) ;
#20757=VERTEX_POINT ( 'NONE', #26362 ) ;
#20760=FACE_OUTER_BOUND ( 'NONE', #16623, .T. ) ;
#20761=DIRECTION ( 'NONE',  ( -0.000000000000000000, 0.000000000000000000, -1.000000000000000000 ) ) ;
#20768=CARTESIAN_POINT ( 'NONE',  ( 205.0999694062793992, 106.8955893716604919, 2.363170148305747009 ) ) ;
#20769=DIRECTION ( 'NONE',  ( 0.000000000000000000, -0.000000000000000000, -1.000000000000000000 ) ) ;
#20770=CARTESIAN_POINT ( 'NONE',  ( -3.255961059272213465, 7.643453059677441708, 70.42757466837964841 ) ) ;
#20772=B_SPLINE_CURVE_WITH_KNOTS ( 'NONE', 3,
 ( #63677, #36601, #19727, #67930, #41185, #62647, #41875, #14454, #30289, #57362, #58383, #68933, #53093, #15491, #14103, #42217, #35909, #36943, #25367, #51738, #58049, #30633, #41529, #10192, #8839, #69287, #3543, #40832, #52079, #62291, #3899, #68271, #35563, #57022, #47139, #57708, #62981, #20407, #9521, #36252, #52427, #4250, #25710, #68601 ),
 .UNSPECIFIED., .F., .F.,
 ( 4, 2, 2, 2, 2, 2, 2, 2, 2, 2, 2, 2, 2, 2, 2, 2, 2, 2, 2, 2, 2, 4 ),
 ( 1.387778780781445676E-17, 0.003433139681083872442, 0.004291424601354786560, 0.005149709521625698942, 0.006866279362167435237, 0.007724564282438299914, 0.008582849202709161990, 0.009441134122980024065, 0.01029941904325088614, 0.01201598888379266233, 0.01373255872433443679, 0.01459084364460531621, 0.01544912856487619217, 0.01630741348514706812, 0.01716569840541794581, 0.01888226824595971506, 0.02059883808650148432, 0.02145712300677240711, 0.02231540792704332990, 0.02403197776758510262, 0.02574854760812687188, 0.02746511744866864460 ),
 .UNSPECIFIED. ) ;
#20774=EDGE_LOOP ( 'NONE', ( #6609, #50155, #54092, #64691 ) ) ;
#20776=CARTESIAN_POINT ( 'NONE',  ( -120.2269354400981598, 44.05870085693242544, 86.88615135046399018 ) ) ;
#20777=CARTESIAN_POINT ( 'NONE',  ( -78.66644367742111399, -170.0000000000000000, -61.96000122218157458 ) ) ;
#20780=CARTESIAN_POINT ( 'NONE',  ( 17.10503398861595770, 7.553194056991637595, 83.81298706601685922 ) ) ;
#20782=CARTESIAN_POINT ( 'NONE',  ( -86.05211524933166345, 26.36495896184001708, -95.00000000000133582 ) ) ;
#20783=CARTESIAN_POINT ( 'NONE',  ( -94.78109144324895396, 29.13179392050636807, 64.57839755988879915 ) ) ;
#20785=ORIENTED_EDGE ( 'NONE', *, *, #29169, .T. ) ;
#20786=CARTESIAN_POINT ( 'NONE',  ( -86.10361028793437299, 25.29528064050657576, 10.07196939449881512 ) ) ;
#20787=ORIENTED_EDGE ( 'NONE', *, *, #25121, .T. ) ;
#20793=ORIENTED_EDGE ( 'NONE', *, *, #53042, .T. ) ;
#20794=CARTESIAN_POINT ( 'NONE',  ( 8.670103207226933506, 6.377073801252349128, -45.43205147905846530 ) ) ;
#20795=CARTESIAN_POINT ( 'NONE',  ( -173.5394735271661375, 87.59446374803708579, 57.66624519710470054 ) ) ;
#20796=CARTESIAN_POINT ( 'NONE',  ( 22.53041628628729498, 6.810083298012986397, 13.99219147001824126 ) ) ;
#20801=CARTESIAN_POINT ( 'NONE',  ( -36.44526830929234507, 10.46676546085014969, 85.81153421141065962 ) ) ;
#20805=EDGE_CURVE ( 'NONE', #2387, #50015, #54446, .T. ) ;
#20806=CARTESIAN_POINT ( 'NONE',  ( 103.1567541746301941, 25.73937982110323119, -45.93086059415202982 ) ) ;
#20807=CARTESIAN_POINT ( 'NONE',  ( 138.5684226926155702, 45.53585076428269218, -64.51278046548689815 ) ) ;
#20808=CARTESIAN_POINT ( 'NONE',  ( -142.0860844253782886, 59.41107357617637064, -70.27677374158945156 ) ) ;
#20812=CARTESIAN_POINT ( 'NONE',  ( -83.69370847062539553, 25.38703975185371675, -75.03095722555288205 ) ) ;
#20813=CARTESIAN_POINT ( 'NONE',  ( 173.9405361758639117, 73.05302209498822208, 12.26640283032960532 ) ) ;
#20814=CARTESIAN_POINT ( 'NONE',  ( -118.5151419614604436, 43.00218563933588456, -41.04416846843501787 ) ) ;
#20815=CARTESIAN_POINT ( 'NONE',  ( -79.61235761536667610, 23.76245710489569518, 3.618273565636886069 ) ) ;
#20817=CARTESIAN_POINT ( 'NONE',  ( 33.34472344659697285, 7.698735568503753512, -92.36667317427755108 ) ) ;
#20818=CARTESIAN_POINT ( 'NONE',  ( 197.3914575603701280, 98.43856781875066986, 92.14791230178799708 ) ) ;
#20819=CARTESIAN_POINT ( 'NONE',  ( 70.45466089417031696, 14.52203022703029056, 11.45482948366315945 ) ) ;
#20820=CARTESIAN_POINT ( 'NONE',  ( 164.8407099662995563, 63.61629583487395223, 8.649268911586283082 ) ) ;
#20821=B_SPLINE_CURVE_WITH_KNOTS ( 'NONE', 3,
 ( #39325, #1337, #34410, #28774, #60767, #12592, #61475, #23499, #11883, #34048, #43878, #7672, #33707, #66425, #54791, #55853, #55489, #55135, #17505, #2731, #38621, #28060, #65363, #61122, #50917, #38981, #50567, #18217, #22791, #17146, #34750, #60064, #23847, #6613, #60428, #12244, #13294, #56186, #44231, #45286, #33361, #66769, #18560, #49499, #6960 ),
 .UNSPECIFIED., .F., .F.,
 ( 4, 2, 2, 1, 2, 2, 2, 2, 2, 2, 2, 2, 2, 2, 2, 2, 2, 2, 2, 2, 2, 2, 4 ),
 ( 0.02346464386237015476, 0.02493212228186624663, 0.02566586149161429603, 0.02639960070136234196, 0.02713333991111039137, 0.02786707912085843730, 0.02933455754035455693, 0.03006829675010262021, 0.03080203595985067655, 0.03226951437934676148, 0.03300325358909482476, 0.03373699279884288804, 0.03520447121833901460, 0.03667194963783514117, 0.03740568884758317669, 0.03813942805733121916, 0.03960690647682733878, 0.04107438489632345840, 0.04254186331581957803, 0.04327560252556764131, 0.04400934173531570459, 0.04547682015481182422, 0.04694429857430794384 ),
 .UNSPECIFIED. ) ;
#20823=ORIENTED_EDGE ( 'NONE', *, *, #2613, .F. ) ;
#20825=CARTESIAN_POINT ( 'NONE',  ( -52.90268453104089730, 15.15480697857591252, 84.31435017214288052 ) ) ;
#20829=CARTESIAN_POINT ( 'NONE',  ( 23.03546163277112768, 7.848986635155163150, -67.91707449678644082 ) ) ;
#20832=CARTESIAN_POINT ( 'NONE',  ( 66.72974708835175761, 13.56459745268606554, -22.91045958329191734 ) ) ;
#20834=CARTESIAN_POINT ( 'NONE',  ( -50.53243683205840853, 14.55237037207940531, -63.55645086763099272 ) ) ;
#20835=CARTESIAN_POINT ( 'NONE',  ( 154.4550750032601627, 55.34393534448157226, -36.75316982753754758 ) ) ;
#20837=CARTESIAN_POINT ( 'NONE',  ( -118.9668643994984052, 43.27909474462862960, -12.68187660284936413 ) ) ;
#20838=ORIENTED_EDGE ( 'NONE', *, *, #36474, .T. ) ;
#20841=DIRECTION ( 'NONE',  ( 0.4112000000000004540, 0.9115451497320358198, -0.000000000000000000 ) ) ;
#20847=VECTOR ( 'NONE', #50536, 1000.000000000000000 ) ;
#20849=CARTESIAN_POINT ( 'NONE',  ( 184.3879440808140657, 83.47316703125159165, -10.14386913531070711 ) ) ;
#20850=CARTESIAN_POINT ( 'NONE',  ( 174.1364721914477514, 71.85829564941447245, -73.40901879464566093 ) ) ;
#20853=B_SPLINE_CURVE_WITH_KNOTS ( 'NONE', 3,
 ( #68452, #69473, #21292, #57894, #42739, #20260, #31179, #52606, #49740, #32202, #174, #54678, #60314, #38154, #32885, #21630, #26913, #43077, #17038, #28301, #23038, #1570, #53633, #6506, #11772, #48339, #64550, #22679, #17396, #44484, #55027, #33597, #65964, #59594, #17762, #65603, #16699, #16358, #39216, #27600, #11073, #64902, #27954, #49041, #5796 ),
 .UNSPECIFIED., .F., .F.,
 ( 4, 2, 2, 2, 2, 2, 2, 2, 2, 2, 2, 2, 2, 1, 2, 2, 2, 2, 2, 2, 2, 2, 4 ),
 ( 0.02352719711393053484, 0.02499986300757012572, 0.02573619595438991076, 0.02647252890120969232, 0.02794519479484923810, 0.02941786068848878388, 0.03015419363530857239, 0.03089052658212835742, 0.03236319247576796565, 0.03309952542258779579, 0.03383585836940762592, 0.03530852426304727926, 0.03604485720986710939, 0.03678119015668693953, 0.03751752310350676967, 0.03825385605032659980, 0.03972652194396622538, 0.04119918783760584402, 0.04267185373124546266, 0.04340818667806528586, 0.04414451962488510905, 0.04561718551852474157, 0.04708985141216438797 ),
 .UNSPECIFIED. ) ;
#20861=CARTESIAN_POINT ( 'NONE',  ( -173.1211646369891355, 87.12891641440857882, 72.66624519710475738 ) ) ;
#20863=CARTESIAN_POINT ( 'NONE',  ( 154.4435090467313785, 56.59612921827832110, 70.61996015326239728 ) ) ;
#20864=CARTESIAN_POINT ( 'NONE',  ( -142.6736406357357794, 59.87555372585265445, 94.99999999999866418 ) ) ;
#20865=DIRECTION ( 'NONE',  ( -0.000000000000000000, 1.000000000000000000, -0.000000000000000000 ) ) ;
#20866=CARTESIAN_POINT ( 'NONE',  ( -0.7847733590455667763, 7.541558926123923534, 88.69980130832604459 ) ) ;
#20873=CARTESIAN_POINT ( 'NONE',  ( 46.86855270197328593, 10.51779196975806840, 91.88407132189860249 ) ) ;
#20876=CARTESIAN_POINT ( 'NONE',  ( 135.3597199823648225, 43.52062712031425207, -89.85493311428349728 ) ) ;
#20878=B_SPLINE_CURVE_WITH_KNOTS ( 'NONE', 3,
 ( #3566, #61273, #13097, #45790, #18713, #40857, #30308, #18361, #8509, #40165, #29960, #51422, #62309, #67598, #34563, #7478, #46470, #66918, #57044, #67949, #19394, #29266, #8858, #39468, #2534, #12744, #66570, #28928, #39818, #50714, #58073, #10564, #9891, #25729, #36624, #19745, #48182, #63003, #26066, #68955, #9192, #36967, #47494, #31002, #57381 ),
 .UNSPECIFIED., .F., .F.,
 ( 4, 2, 2, 2, 2, 2, 2, 2, 2, 2, 2, 2, 2, 1, 2, 2, 2, 2, 2, 2, 2, 2, 4 ),
 ( 0.02356759485890611364, 0.02503765354686408873, 0.02577268289084306413, 0.02650771223482203606, 0.02797777092277998687, 0.02944782961073793767, 0.03018285895471693736, 0.03091788829869593358, 0.03238794698665397459, 0.03312297633063299857, 0.03385800567461202254, 0.03532806436257011212, 0.03606309370654915691, 0.03679812305052820171, 0.03753315239450724650, 0.03826818173848629129, 0.03973824042644441557, 0.04120829911440254678, 0.04267835780236067800, 0.04341338714633974361, 0.04414841649031881615, 0.04561847517827696125, 0.04708853386623510634 ),
 .UNSPECIFIED. ) ;
#20880=CARTESIAN_POINT ( 'NONE',  ( -5.401648928593173693, 6.744888135494081283, 17.88536589262118071 ) ) ;
#20882=CARTESIAN_POINT ( 'NONE',  ( 34.84173759613683075, 7.859847277726514925, -10.30082682987506715 ) ) ;
#20883=CARTESIAN_POINT ( 'NONE',  ( 174.1348882614952629, 73.23561817543362906, -40.88960443691671998 ) ) ;
#20884=CARTESIAN_POINT ( 'NONE',  ( 164.2089238023960718, 63.08603653844363635, 87.28623637339566699 ) ) ;
#20889=AXIS2_PLACEMENT_3D ( 'NONE', #67985, #52812, #31379 ) ;
#20891=B_SPLINE_CURVE_WITH_KNOTS ( 'NONE', 3,
 ( #58434, #47882, #69346, #35623, #57075, #27464, #59817, #11632, #10591, #43288, #32063, #16912, #65115, #38 ),
 .UNSPECIFIED., .F., .F.,
 ( 4, 2, 2, 2, 2, 2, 4 ),
 ( 0.000000000000000000, 0.001279364114800584686, 0.002558728229601169371, 0.003838092344401753623, 0.005117456459202338742, 0.007676184688803516787, 0.01023491291840469483 ),
 .UNSPECIFIED. ) ;
#20892=CARTESIAN_POINT ( 'NONE',  ( 11.21312910819262676, 7.403355431336992254, 31.55132192236441568 ) ) ;
#20894=CARTESIAN_POINT ( 'NONE',  ( 198.2581645178918279, 99.52881771501679964, 40.56300693318002715 ) ) ;
#20895=CARTESIAN_POINT ( 'NONE',  ( -85.31879956968585077, 26.05747381080316316, 88.08442089185827228 ) ) ;
#20902=CARTESIAN_POINT ( 'NONE',  ( 117.7442255600443133, 33.63739995216997158, -70.76590447690840335 ) ) ;
#20907=CARTESIAN_POINT ( 'NONE',  ( -190.6985136298602015, 109.1272424661243434, -10.81538671745452795 ) ) ;
#20908=CARTESIAN_POINT ( 'NONE',  ( -8.810383862755523765, 7.965311326754778598, -8.622074896589690951 ) ) ;
#20912=CARTESIAN_POINT ( 'NONE',  ( -190.6985136298602015, 109.1272424661243434, -64.50448789838189612 ) ) ;
#20915=CARTESIAN_POINT ( 'NONE',  ( 70.51583798635768119, 15.57951509147424041, -16.61804899806768532 ) ) ;
#20916=CARTESIAN_POINT ( 'NONE',  ( -83.13046924527391468, 25.15778674529016357, -48.64714892153850201 ) ) ;
#20917=CARTESIAN_POINT ( 'NONE',  ( 107.7734915886500460, 27.75592479571297488, 83.71111518197675139 ) ) ;
#20918=CARTESIAN_POINT ( 'NONE',  ( -156.0209085498132140, 71.27066046086522988, 7.619205632352728408 ) ) ;
#20921=CARTESIAN_POINT ( 'NONE',  ( -147.4686369529070191, 63.77742835114294451, 84.67161332027325216 ) ) ;
#20926=CARTESIAN_POINT ( 'NONE',  ( 34.45972925205163762, 8.830088223935224079, -48.78227442661408020 ) ) ;
#20927=CARTESIAN_POINT ( 'NONE',  ( 104.6432117441986520, 26.37618165085906341, -92.10548344321300362 ) ) ;
#20928=CARTESIAN_POINT ( 'NONE',  ( -36.37371824399144060, 10.45334302951138206, 58.89140364663110461 ) ) ;
#20929=CYLINDRICAL_SURFACE ( 'NONE', #19515, 7.500000000000020428 ) ;
#20931=CARTESIAN_POINT ( 'NONE',  ( 35.44781468922823109, 7.928097401423693569, 57.88074027180304881 ) ) ;
#20932=CARTESIAN_POINT ( 'NONE',  ( 12.46277766093406214, 6.416700641561363661, -9.434012564203385409 ) ) ;
#20933=ADVANCED_FACE ( 'NONE', ( #32329 ), #16485, .T. ) ;
#20935=CARTESIAN_POINT ( 'NONE',  ( 184.3941060377211443, 82.01604625189463604, 56.90855055168082544 ) ) ;
#20937=CARTESIAN_POINT ( 'NONE',  ( -81.23297981660238065, 23.31577157498399089, -35.56415816642201833 ) ) ;
#20938=CARTESIAN_POINT ( 'NONE',  ( 23.28785143291466042, 6.856621069835718174, 63.85807121681927612 ) ) ;
#20940=CARTESIAN_POINT ( 'NONE',  ( 8.767814708128309320, 7.383611927972575373, 8.019991926173236862 ) ) ;
#20945=CARTESIAN_POINT ( 'NONE',  ( 188.2076037774874635, 86.11782719225436722, 7.600624286963005183 ) ) ;
#20947=CARTESIAN_POINT ( 'NONE',  ( -190.6985136298601731, 109.1272424661242582, 94.99999999999866418 ) ) ;
#20950=CARTESIAN_POINT ( 'NONE',  ( 55.91494169499919309, 12.16343363043255543, -67.63797929442789325 ) ) ;
#20951=EDGE_LOOP ( 'NONE', ( #64924, #7459, #60403, #28308 ) ) ;
#20956=CARTESIAN_POINT ( 'NONE',  ( -28.13266652174640470, 9.071935854491409046, -9.236353854820380960 ) ) ;
#20957=CARTESIAN_POINT ( 'NONE',  ( 197.3756653044963230, 98.41886189307120958, 8.231045378275350544 ) ) ;
#20958=EDGE_CURVE ( 'NONE', #25468, #68538, #34766, .T. ) ;
#20964=CARTESIAN_POINT ( 'NONE',  ( 131.6005058089754982, 40.07838125795770168, 29.84241593357604216 ) ) ;
#20974=CARTESIAN_POINT ( 'NONE',  ( -119.2682179969168175, 42.28333404791700190, -12.01608118964443861 ) ) ;
#20977=CARTESIAN_POINT ( 'NONE',  ( -180.2252811616041868, 95.40045830523435200, -12.94562834876021107 ) ) ;
#20978=PLANE ( 'NONE',  #60062 ) ;
#20979=CARTESIAN_POINT ( 'NONE',  ( -142.6264002846223775, 58.55577336362199503, -45.30821067346655440 ) ) ;
#20980=VERTEX_POINT ( 'NONE', #50585 ) ;
#20981=CARTESIAN_POINT ( 'NONE',  ( -109.7058324133404454, 37.86601138638052788, 92.81177118499459766 ) ) ;
#20988=CARTESIAN_POINT ( 'NONE',  ( -95.05323930133205579, 30.36974142673411592, 66.93429615280686562 ) ) ;
#20990=CARTESIAN_POINT ( 'NONE',  ( -129.6079169496900931, 50.20899308323960497, -62.73827057211200753 ) ) ;
#20991=CARTESIAN_POINT ( 'NONE',  ( 55.86967469797618691, 11.12799771593089559, -94.59437614483285017 ) ) ;
#20992=CARTESIAN_POINT ( 'NONE',  ( -100.4262673593280226, 31.84860241619275101, 18.45695312107208252 ) ) ;
#20993=CARTESIAN_POINT ( 'NONE',  ( -98.46684543088107944, 30.88557736720390778, -62.89638174071533427 ) ) ;
#20999=CARTESIAN_POINT ( 'NONE',  ( -166.5704851812740515, 80.12110537694670143, -45.87459088847822386 ) ) ;
#21002=DIRECTION ( 'NONE',  ( 0.000000000000000000, 0.000000000000000000, 1.000000000000000000 ) ) ;
#21003=CARTESIAN_POINT ( 'NONE',  ( -78.19438069111009781, 23.21811806230640585, 30.41820113967310846 ) ) ;
#21004=CARTESIAN_POINT ( 'NONE',  ( -72.21889834709581635, 21.03534256744170960, -65.59680318578142533 ) ) ;
#21008=CARTESIAN_POINT ( 'NONE',  ( -120.1346137380982526, 44.00127440773568566, 33.30914571746500741 ) ) ;
#21009=CARTESIAN_POINT ( 'NONE',  ( 208.9781236209186659, 112.4006213943319636, 69.72746670309929584 ) ) ;
#21013=CARTESIAN_POINT ( 'NONE',  ( -14.94265033805046095, 7.459411036484911328, -45.33398552347500754 ) ) ;
#21015=DIRECTION ( 'NONE',  ( 0.000000000000000000, 0.000000000000000000, 1.000000000000000000 ) ) ;
#21016=CARTESIAN_POINT ( 'NONE',  ( 92.95016907945942819, 22.74936990452175678, 60.01214966832145592 ) ) ;
#21019=CARTESIAN_POINT ( 'NONE',  ( 34.45500533947588195, 7.817363290423888778, -64.30597072735039887 ) ) ;
#21020=CARTESIAN_POINT ( 'NONE',  ( -94.83091526606385457, 30.26550147229323073, -70.37511245693397655 ) ) ;
#21021=CARTESIAN_POINT ( 'NONE',  ( -32.41898580403140784, 10.77423026598439648, -8.520716206325841924 ) ) ;
#21027=CARTESIAN_POINT ( 'NONE',  ( 12.47451846520757002, 7.423604437114563304, -76.59618454708339641 ) ) ;
#21028=CARTESIAN_POINT ( 'NONE',  ( -190.3061188229049208, 108.5745819235681751, 15.45852572812942327 ) ) ;
#21030=CARTESIAN_POINT ( 'NONE',  ( -1.857619870843140619, 6.575690665396233925, 42.18455459037815558 ) ) ;
#21031=CARTESIAN_POINT ( 'NONE',  ( 210.6189312023034574, 116.6550319566545539, 94.99999999999866418 ) ) ;
#21032=CARTESIAN_POINT ( 'NONE',  ( 151.6178224291901131, 54.48737267587416966, -38.92713886945099233 ) ) ;
#21033=EDGE_CURVE ( 'NONE', #45819, #37504, #60081, .T. ) ;
#21036=CARTESIAN_POINT ( 'NONE',  ( -189.4248691432192970, 107.3461292335514656, -16.99913809175565405 ) ) ;
#21037=CARTESIAN_POINT ( 'NONE',  ( 175.5498284945444709, 74.57669191966280664, -21.96822280477383060 ) ) ;
#21038=CARTESIAN_POINT ( 'NONE',  ( -108.5248383251030333, 37.21456094989614627, 60.70243158702523090 ) ) ;
#21043=CARTESIAN_POINT ( 'NONE',  ( -2.866724795119724778, 6.618578306599219196, -10.42539455610338806 ) ) ;
#21046=CARTESIAN_POINT ( 'NONE',  ( 197.9868529032975744, 99.18611233336805810, -20.34206310618822755 ) ) ;
#21047=CARTESIAN_POINT ( 'NONE',  ( -142.0345488537072072, 58.09133413710082294, 91.24922763633107081 ) ) ;
#21048=EDGE_CURVE ( 'NONE', #14098, #13609, #35526, .T. ) ;
#21054=CARTESIAN_POINT ( 'NONE',  ( 80.16761386260783695, 18.37011649821945269, 6.527426858061783577 ) ) ;
#21056=CARTESIAN_POINT ( 'NONE',  ( 164.8433205901839358, 64.93586312665800619, 11.46758294457424654 ) ) ;
#21061=B_SPLINE_CURVE_WITH_KNOTS ( 'NONE', 3,
 ( #59930, #27933, #49722, #1550, #6485, #39880, #38852, #49372, #1204, #61341, #13161, #55004, #39537, #66631, #18427, #45150, #23709, #22657, #44098, #23011, #17015, #55715, #65581, #17743, #55357, #17374, #43747, #60296, #33580, #44464, #50440, #28274, #12114, #34626, #7541, #7879, #39200, #33918, #65224, #60990, #6826, #12812, #65945, #29329 ),
 .UNSPECIFIED., .F., .F.,
 ( 4, 2, 2, 2, 2, 2, 2, 2, 2, 2, 2, 2, 2, 2, 2, 2, 2, 2, 2, 2, 2, 4 ),
 ( 1.440969542111313559E-17, 0.001482469635030006592, 0.002223704452545002298, 0.002964939270059997571, 0.004447408905089988117, 0.005929878540119976928, 0.007412348175149966606, 0.008153582992664965348, 0.008894817810179967560, 0.01037728744520997198, 0.01185975708023997814, 0.01260099189775498556, 0.01334222671526999297, 0.01482469635030000607, 0.01556593116781501175, 0.01630716598533001743, 0.01778963562036001839, 0.01927210525539002628, 0.02001334007290502676, 0.02075457489042003070, 0.02223704452545005247, 0.02371951416048007424 ),
 .UNSPECIFIED. ) ;
#21062=CARTESIAN_POINT ( 'NONE',  ( 174.1348882614952629, 73.23561817543360064, 66.48859792493803411 ) ) ;
#21065=CARTESIAN_POINT ( 'NONE',  ( -105.8879439778144445, 34.65133284149107595, -49.10708695906607346 ) ) ;
#21066=CARTESIAN_POINT ( 'NONE',  ( 69.08240197259638649, 14.16210831900840716, -74.48173343371692567 ) ) ;
#21068=CARTESIAN_POINT ( 'NONE',  ( 151.1700480242206197, 54.15904440870136938, 14.14223021667874569 ) ) ;
#21070=CARTESIAN_POINT ( 'NONE',  ( -178.0633751203918393, 92.80295726428047942, 43.96776513697549404 ) ) ;
#21072=EDGE_CURVE ( 'NONE', #47842, #60292, #25934, .T. ) ;
#21073=EDGE_CURVE ( 'NONE', #55324, #10027, #45209, .T. ) ;
#21074=CARTESIAN_POINT ( 'NONE',  ( 117.4711568421289627, 33.49899443629671936, -41.35662267546008763 ) ) ;
#21078=CARTESIAN_POINT ( 'NONE',  ( 137.4117721579687554, 43.61242559081432546, 70.47591696582985321 ) ) ;
#21079=CARTESIAN_POINT ( 'NONE',  ( -166.5686015187718283, 80.11916873959171426, 41.98092334962779404 ) ) ;
#21080=CARTESIAN_POINT ( 'NONE',  ( -37.38781680082736614, 10.64362327909142181, -74.25552192898616966 ) ) ;
#21083=CARTESIAN_POINT ( 'NONE',  ( 45.35621884287174765, 10.27694987765648271, 5.982729125893944122 ) ) ;
#21085=EDGE_LOOP ( 'NONE', ( #29214, #27170, #33901, #48224 ) ) ;
#21087=CARTESIAN_POINT ( 'NONE',  ( 212.1488570093001726, 119.0116247937291405, -17.85290917965843605 ) ) ;
#21089=CARTESIAN_POINT ( 'NONE',  ( -157.0077369422017739, 70.81157624963286423, -69.43848245219707849 ) ) ;
#21091=CARTESIAN_POINT ( 'NONE',  ( -109.2503638244981232, 36.46497529133068127, 88.92031527522445344 ) ) ;
#21093=CARTESIAN_POINT ( 'NONE',  ( 207.8675797643809631, 110.7908513421271977, -37.01557826710286037 ) ) ;
#21098=VERTEX_POINT ( 'NONE', #36143 ) ;
#21099=CARTESIAN_POINT ( 'NONE',  ( -71.17984086584780812, 20.67393782512345624, 65.27769819161431997 ) ) ;
#21101=CARTESIAN_POINT ( 'NONE',  ( 188.2950202724320263, 86.21411212788220269, 34.72575518757594182 ) ) ;
#21104=CARTESIAN_POINT ( 'NONE',  ( -76.78936026062118003, 21.61552955137052479, 3.808395977436665358 ) ) ;
#21105=CARTESIAN_POINT ( 'NONE',  ( -33.12535873119978191, 9.874205581139028354, -89.19521348031341290 ) ) ;
#21106=CARTESIAN_POINT ( 'NONE',  ( 21.43750346857338229, 7.754771113113082315, 42.47208553991309543 ) ) ;
#21107=CARTESIAN_POINT ( 'NONE',  ( 197.5213143501814272, 96.99325216816036743, 88.17819802051872102 ) ) ;
#21111=CARTESIAN_POINT ( 'NONE',  ( -76.10397364431022993, 21.36211154336727702, 57.71004732640698620 ) ) ;
#21114=ORIENTED_EDGE ( 'NONE', *, *, #31124, .F. ) ;
#21116=CARTESIAN_POINT ( 'NONE',  ( 57.39674746172462250, 11.43903079040058834, -38.22885664779096970 ) ) ;
#21118=LINE ( 'NONE', #26733, #23790 ) ;
#21124=CARTESIAN_POINT ( 'NONE',  ( -125.8938041572051389, 47.69968343338778283, 30.61994787315706290 ) ) ;
#21128=CARTESIAN_POINT ( 'NONE',  ( 59.72526569420001152, 11.93313563009888689, 70.91484602205103727 ) ) ;
#21133=EDGE_CURVE ( 'NONE', #40777, #18538, #27267, .T. ) ;
#21139=CARTESIAN_POINT ( 'NONE',  ( -165.9992860119575084, 79.53569239468046703, -17.73646718843910008 ) ) ;
#21140=CARTESIAN_POINT ( 'NONE',  ( 135.6651581599209919, 42.52720121194706593, -77.65019136801915067 ) ) ;
#21141=CARTESIAN_POINT ( 'NONE',  ( 204.6977192012829789, 106.3443248447423599, 56.05227132923312183 ) ) ;
#21142=CARTESIAN_POINT ( 'NONE',  ( -189.7334103489410211, 107.7745063523401114, -71.65189628423172508 ) ) ;
#21144=CARTESIAN_POINT ( 'NONE',  ( -95.52163045714284806, 29.47808868198295329, 61.60217047910855825 ) ) ;
#21146=AXIS2_PLACEMENT_3D ( 'NONE', #12651, #39039, #18620 ) ;
#21147=CARTESIAN_POINT ( 'NONE',  ( -73.81689110552360944, 20.53332132481498462, 32.19181849619675972 ) ) ;
#21150=ORIENTED_EDGE ( 'NONE', *, *, #7309, .T. ) ;
#21151=CARTESIAN_POINT ( 'NONE',  ( -119.6801029354224681, 43.71909921132878907, 7.067823973529548276 ) ) ;
#21152=CARTESIAN_POINT ( 'NONE',  ( -179.8996803435689174, 95.00451760716447325, 68.38766948947770175 ) ) ;
#21154=CARTESIAN_POINT ( 'NONE',  ( 126.4324872316703363, 37.11876756822026380, 64.95086461873292194 ) ) ;
#21157=CARTESIAN_POINT ( 'NONE',  ( 63.01563776193091826, 13.70579113808096849, 17.96841034875761878 ) ) ;
#21158=CARTESIAN_POINT ( 'NONE',  ( 152.8558173410469578, 54.14978343559394602, 42.84179159303089790 ) ) ;
#21160=FACE_OUTER_BOUND ( 'NONE', #5536, .T. ) ;
#21161=CARTESIAN_POINT ( 'NONE',  ( -26.88245755577923291, 8.887394979218516511, 31.73890780661882971 ) ) ;
#21164=FACE_BOUND ( 'NONE', #31960, .T. ) ;
#21166=CARTESIAN_POINT ( 'NONE',  ( -79.62207341875657107, 23.76621716825509623, -62.00572262374755894 ) ) ;
#21167=CARTESIAN_POINT ( 'NONE',  ( 174.4912080999799002, 73.57140295268877139, 13.55010776019312679 ) ) ;
#21169=CARTESIAN_POINT ( 'NONE',  ( -85.89078989036968892, 26.29712602777652464, 9.043151598351821363 ) ) ;
#21171=CARTESIAN_POINT ( 'NONE',  ( 37.36225457415450535, 8.152725941243264884, -89.57965209093477199 ) ) ;
#21172=CARTESIAN_POINT ( 'NONE',  ( -118.4709174626548531, 42.97515378817185905, -68.15209134257274570 ) ) ;
#21173=CARTESIAN_POINT ( 'NONE',  ( 63.98009977735162579, 12.89803120691695959, 3.014776002286982948 ) ) ;
#21174=CARTESIAN_POINT ( 'NONE',  ( -85.66184035008924980, 26.20110535976566624, 67.47910982318403228 ) ) ;
#21175=CARTESIAN_POINT ( 'NONE',  ( 93.32228019177713918, 22.88890999585039410, -19.87069863458034291 ) ) ;
#21181=CARTESIAN_POINT ( 'NONE',  ( 22.28700331106866983, 7.803633676228379557, -66.11158134317128088 ) ) ;
#21183=CARTESIAN_POINT ( 'NONE',  ( -144.7530445311634821, 61.54314312182903990, 59.25981816036905059 ) ) ;
#21185=LINE ( 'NONE', #26805, #50842 ) ;
#21186=CARTESIAN_POINT ( 'NONE',  ( -52.00092620775817664, 14.92276858858357436, -76.41618673138754048 ) ) ;
#21188=CARTESIAN_POINT ( 'NONE',  ( -122.3994536713185539, 45.42826354555015911, -8.928800194678888857 ) ) ;
#21191=ORIENTED_EDGE ( 'NONE', *, *, #57402, .F. ) ;
#21194=CARTESIAN_POINT ( 'NONE',  ( -306.1215797690288696, 161.1948386903797825, 0.000000000000000000 ) ) ;
#21197=CARTESIAN_POINT ( 'NONE',  ( 128.0786479395874267, 39.20070012600677956, -92.41263896547152967 ) ) ;
#21200=CARTESIAN_POINT ( 'NONE',  ( 89.88147981065577596, 21.62466191578948127, 17.14297335626316254 ) ) ;
#21201=CARTESIAN_POINT ( 'NONE',  ( -15.08468253268399728, 7.472949889606720575, 62.51227595438552243 ) ) ;
#21202=CARTESIAN_POINT ( 'NONE',  ( 210.0055645826032844, 115.7254585628714239, 4.541385688506491825 ) ) ;
#21204=CARTESIAN_POINT ( 'NONE',  ( -85.85317205159077503, 26.28128351165222298, -94.11325662453201346 ) ) ;
#21205=CARTESIAN_POINT ( 'NONE',  ( 46.76970795284345428, 9.482505412758889918, -14.81013751142722867 ) ) ;
#21206=CARTESIAN_POINT ( 'NONE',  ( 205.0999694062793424, 106.8955893716604777, -24.48138044215792064 ) ) ;
#21209=CARTESIAN_POINT ( 'NONE',  ( 157.4703587214989398, 58.92748579479259519, 71.25401806271709404 ) ) ;
#21211=VERTEX_POINT ( 'NONE', #45997 ) ;
#21214=CARTESIAN_POINT ( 'NONE',  ( 92.52113039222224700, 22.58921125235803729, -38.65466082921378188 ) ) ;
#21217=CARTESIAN_POINT ( 'NONE',  ( 150.4544126017350720, 52.39556706174411715, 7.400449090205046154 ) ) ;
#21218=CARTESIAN_POINT ( 'NONE',  ( -3.540478021920604679, 7.657046766457612286, 85.14064472492238167 ) ) ;
#21220=ORIENTED_EDGE ( 'NONE', *, *, #58272, .F. ) ;
#21222=CARTESIAN_POINT ( 'NONE',  ( -62.45176220516618315, 16.79101814080731714, 65.91410335926558162 ) ) ;
#21224=ORIENTED_EDGE ( 'NONE', *, *, #25519, .T. ) ;
#21225=CARTESIAN_POINT ( 'NONE',  ( 41.05177318205839754, 9.645271888559822315, 83.77932428570838397 ) ) ;
#21227=CARTESIAN_POINT ( 'NONE',  ( 137.8343364920582133, 45.06871843100040564, -90.84222727415109944 ) ) ;
#21229=CARTESIAN_POINT ( 'NONE',  ( -59.56523643198715234, 15.93788386494078502, -63.56521738332754268 ) ) ;
#21230=CARTESIAN_POINT ( 'NONE',  ( 39.40195752203892710, 8.409560354027385998, -8.775266874964067654 ) ) ;
#21231=CARTESIAN_POINT ( 'NONE',  ( 175.0696098417091662, 74.11936424544846602, -48.21306686516284401 ) ) ;
#21233=CARTESIAN_POINT ( 'NONE',  ( 88.52345267551655184, 20.07594890262053866, 29.95123874579921619 ) ) ;
#21236=DIRECTION ( 'NONE',  ( -0.000000000000000000, 1.000000000000000000, -0.000000000000000000 ) ) ;
#21237=FACE_OUTER_BOUND ( 'NONE', #41375, .T. ) ;
#21238=CARTESIAN_POINT ( 'NONE',  ( 198.7123879174244223, 100.1053816708572555, 32.18029401982719406 ) ) ;
#21239=VECTOR ( 'NONE', #47346, 1000.000000000000000 ) ;
#21240=CARTESIAN_POINT ( 'NONE',  ( -83.27963540317796287, 25.21826204940221317, 85.68556430999879581 ) ) ;
#21241=DIRECTION ( 'NONE',  ( 0.000000000000000000, 0.000000000000000000, 1.000000000000000000 ) ) ;
#21245=CARTESIAN_POINT ( 'NONE',  ( 116.0822834687217266, 32.80169113915576418, -65.53445419630700997 ) ) ;
#21248=CARTESIAN_POINT ( 'NONE',  ( -36.89224332184166855, 11.57404295377975956, 59.40614351394950177 ) ) ;
#21249=CARTESIAN_POINT ( 'NONE',  ( -10.23531775138760480, 8.068923942586298637, -23.18003092887482453 ) ) ;
#21250=CARTESIAN_POINT ( 'NONE',  ( 152.6560521232696033, 54.00248515670894989, -76.22471660518338865 ) ) ;
#21251=CARTESIAN_POINT ( 'NONE',  ( -24.09190246691234805, 9.515371887976103338, -95.00000000000133582 ) ) ;
#21252=DIRECTION ( 'NONE',  ( -0.000000000000000000, 1.000000000000000000, -0.000000000000000000 ) ) ;
#21257=CARTESIAN_POINT ( 'NONE',  ( 107.1706323048065599, 27.48610522718908911, 83.95080517049565572 ) ) ;
#21258=CARTESIAN_POINT ( 'NONE',  ( 115.7612476187724013, 32.64200929566222698, -11.47492610996905782 ) ) ;
#21259=ADVANCED_FACE ( 'NONE', ( #47713 ), #16407, .F. ) ;
#21262=CARTESIAN_POINT ( 'NONE',  ( -190.6985136298602015, 109.1272424661243434, -91.34903848884556510 ) ) ;
#21267=CARTESIAN_POINT ( 'NONE',  ( -151.2511071212631748, 67.00426547928871912, -8.160532014092686026 ) ) ;
#21269=CARTESIAN_POINT ( 'NONE',  ( 33.75794032130627187, 8.754084575552404601, -38.15644254858585782 ) ) ;
#21274=CARTESIAN_POINT ( 'NONE',  ( 203.9228889538745193, 106.9879579748728702, 56.08195001833964710 ) ) ;
#21276=CARTESIAN_POINT ( 'NONE',  ( 183.1873354889583538, 82.20882912211250471, 56.44120003221799209 ) ) ;
#21277=CARTESIAN_POINT ( 'NONE',  ( -156.0300823189602113, 69.91528270335481920, 61.32471221532804861 ) ) ;
#21278=CARTESIAN_POINT ( 'NONE',  ( -7.825402957745087207, 6.891034867348159842, -35.41807073194381417 ) ) ;
#21279=CARTESIAN_POINT ( 'NONE',  ( 184.3994103300443328, 82.02159554764423888, 70.39554651480847269 ) ) ;
#21281=CARTESIAN_POINT ( 'NONE',  ( -86.15441609607631790, 25.31657638323081727, -43.11050758368907054 ) ) ;
#21282=CARTESIAN_POINT ( 'NONE',  ( 16.28371206594635368, 6.516665886438621769, 71.85925826316893961 ) ) ;
#21284=CARTESIAN_POINT ( 'NONE',  ( 8.848532605049241440, 6.377649401037235322, -66.98796475424842356 ) ) ;
#21286=AXIS2_PLACEMENT_3D ( 'NONE', #50484, #12158, #57152 ) ;
#21288=CARTESIAN_POINT ( 'NONE',  ( -31.43908319763710679, -170.0000000000000000, 37.71645440618917888 ) ) ;
#21290=CARTESIAN_POINT ( 'NONE',  ( 176.6258282025055166, 74.21441092921637050, 30.77301370930646840 ) ) ;
#21291=DIRECTION ( 'NONE',  ( -0.000000000000000000, 1.000000000000000000, -0.000000000000000000 ) ) ;
#21292=CARTESIAN_POINT ( 'NONE',  ( 40.37438610703016906, 8.537526699166111399, -77.41724195684747656 ) ) ;
#21296=EDGE_LOOP ( 'NONE', ( #63587, #24238, #110, #66143 ) ) ;
#21298=CARTESIAN_POINT ( 'NONE',  ( 174.6746562023443801, 72.36198225676386642, 94.41010371319214300 ) ) ;
#21300=CARTESIAN_POINT ( 'NONE',  ( 116.1021807117072058, 31.68810634233422974, 68.66407567072008078 ) ) ;
#21302=CARTESIAN_POINT ( 'NONE',  ( 132.9453095272139649, 42.04754713161464252, -62.86786152285933582 ) ) ;
#21303=CARTESIAN_POINT ( 'NONE',  ( 128.0568017572569488, 38.03085713813911184, 32.22834714527665056 ) ) ;
#21305=CARTESIAN_POINT ( 'NONE',  ( 84.66625268040917263, 18.76025835477234693, -89.76113623899809113 ) ) ;
#21306=CARTESIAN_POINT ( 'NONE',  ( -119.1064753703575718, -170.0000000000000000, 94.99999999999866418 ) ) ;
#21307=DIRECTION ( 'NONE',  ( 0.000000000000000000, 0.000000000000000000, 1.000000000000000000 ) ) ;
#21308=B_SPLINE_CURVE_WITH_KNOTS ( 'NONE', 3,
 ( #13544, #46930, #62420, #34666, #29717, #68393, #51860, #19156, #14574, #56103, #40610, #2640, #35698, #8264, #8621, #14237, #25144, #45542, #51179, #67025, #18816, #24453, #35343, #56802, #45894, #67365, #459, #52877, #10321, #9648, #43007, #58174, #52546, #53567, #5046, #63803, #20884, #47947, #32475, #48279, #11011, #21913, #15266, #4705, #26853, #64483, #41993, #58851, #43362, #69416, #107, #36729 ),
 .UNSPECIFIED., .F., .F.,
 ( 4, 2, 2, 2, 2, 2, 2, 2, 2, 2, 2, 2, 2, 2, 2, 2, 2, 2, 2, 2, 2, 2, 2, 2, 2, 4 ),
 ( 0.000000000000000000, 0.002274976238400359084, 0.004549952476800718168, 0.005687440596000920695, 0.006824928715201121487, 0.007962416834401324015, 0.009099904953601524807, 0.01023739307280172733, 0.01137488119200192986, 0.01364985743040229675, 0.01592483366880266538, 0.01706232178800288005, 0.01819980990720309125, 0.02047478614560356569, 0.02274976238400404360, 0.02388725050320428950, 0.02502473862240453192, 0.02729971486080498902, 0.02843720298000524879, 0.02957469109920550163, 0.03071217921840575446, 0.03184966733760600383, 0.03298715545680625666, 0.03412464357600650949, 0.03526213169520676233, 0.03639961981440701516 ),
 .UNSPECIFIED. ) ;
#21313=CARTESIAN_POINT ( 'NONE',  ( -149.5074843970970733, 65.50121172469319220, -34.81283053149196149 ) ) ;
#21314=CARTESIAN_POINT ( 'NONE',  ( -169.1116812882276861, 84.24296059722695418, -62.70237070590246731 ) ) ;
#21315=CARTESIAN_POINT ( 'NONE',  ( -144.2188519266539970, 59.82027639618911508, -47.63651262692244615 ) ) ;
#21317=CARTESIAN_POINT ( 'NONE',  ( -7.825402957745087207, -170.0000000000000000, -8.573520141480127421 ) ) ;
#21323=CARTESIAN_POINT ( 'NONE',  ( 80.17205177205136124, 17.31791394718354837, -20.30016712999428918 ) ) ;
#21324=CARTESIAN_POINT ( 'NONE',  ( -128.9863978264384627, 49.78205252558956317, -62.42159899320021310 ) ) ;
#21326=CARTESIAN_POINT ( 'NONE',  ( -95.50384525802328994, 29.46973564057716999, 14.39913645707428280 ) ) ;
#21327=CARTESIAN_POINT ( 'NONE',  ( -95.21430597939259144, 29.33390900154318004, -71.92457073492782627 ) ) ;
#21330=CARTESIAN_POINT ( 'NONE',  ( 181.0840389613909736, 78.60582251573003987, -78.06960825634331513 ) ) ;
#21332=CARTESIAN_POINT ( 'NONE',  ( -165.7689197919845014, 79.30072199592278537, -40.70117905480101683 ) ) ;
#21335=CARTESIAN_POINT ( 'NONE',  ( 109.7782172510783454, 29.77507867835874933, -77.76698815611737814 ) ) ;
#21336=CARTESIAN_POINT ( 'NONE',  ( -78.18897186942402300, 23.21604822208489338, 45.41820113967314398 ) ) ;
#21337=CARTESIAN_POINT ( 'NONE',  ( 82.14449817946434962, 17.93919511903895625, 43.22844623160558086 ) ) ;
#21339=CARTESIAN_POINT ( 'NONE',  ( 42.71680114082827373, 9.880016734137544887, -36.37429557171203243 ) ) ;
#21342=CARTESIAN_POINT ( 'NONE',  ( 204.6977192012829789, 108.0580384837234931, -9.481380442157895772 ) ) ;
#21345=CARTESIAN_POINT ( 'NONE',  ( -9.525868120571905351, 7.007646177566255297, -35.60930802222527092 ) ) ;
#21347=CARTESIAN_POINT ( 'NONE',  ( 88.53025347111699261, 21.14438024052374132, 56.78577616652550830 ) ) ;
#21348=CARTESIAN_POINT ( 'NONE',  ( 110.2429982417149432, 29.99119854320847267, 2.766663615273645682 ) ) ;
#21350=CARTESIAN_POINT ( 'NONE',  ( 31.95008798096003844, 7.556925044648910905, -68.98185651406271290 ) ) ;
#21351=CARTESIAN_POINT ( 'NONE',  ( 15.78827728214693416, 7.507518794609589818, -50.51894409868581448 ) ) ;
#21359=CARTESIAN_POINT ( 'NONE',  ( 8.540564391411901823, 7.383006541823028179, -71.80808571654557682 ) ) ;
#21362=CARTESIAN_POINT ( 'NONE',  ( -4.955782654901479845, 6.720825733572404204, 30.67341288399633115 ) ) ;
#21363=CARTESIAN_POINT ( 'NONE',  ( -97.47339919287394139, 30.40512551257286944, -9.891953464162076770 ) ) ;
#21364=CARTESIAN_POINT ( 'NONE',  ( 93.47266763748514506, 22.94549330578766089, 87.81307861244059154 ) ) ;
#21368=AXIS2_PLACEMENT_3D ( 'NONE', #14186, #51127, #51478 ) ;
#21370=CARTESIAN_POINT ( 'NONE',  ( -133.3149301983942507, 51.57857650535024163, 12.39399621277310004 ) ) ;
#21373=CARTESIAN_POINT ( 'NONE',  ( -105.8683518445188980, 35.77995342500074827, 58.26050255926607235 ) ) ;
#21375=CARTESIAN_POINT ( 'NONE',  ( -133.3220917939969752, 52.82057604964900577, -41.34405810791972868 ) ) ;
#21378=CARTESIAN_POINT ( 'NONE',  ( 92.21267147730743829, 21.40196534721317434, 69.08802095801497956 ) ) ;
#21380=CARTESIAN_POINT ( 'NONE',  ( -145.9244519207070141, 61.19885883688223771, 85.31486399595573289 ) ) ;
#21382=ORIENTED_EDGE ( 'NONE', *, *, #8011, .T. ) ;
#21384=CARTESIAN_POINT ( 'NONE',  ( 79.33384730094452664, 18.11203072455030849, 8.609877271889105899 ) ) ;
#21386=CARTESIAN_POINT ( 'NONE',  ( -125.8938041572051389, -170.0000000000000000, -23.06915330777029638 ) ) ;
#21387=VECTOR ( 'NONE', #3411, 1000.000000000000000 ) ;
#21389=CARTESIAN_POINT ( 'NONE',  ( -149.5074843970970733, 65.50121172469317798, -61.65738112195564469 ) ) ;
#21392=CARTESIAN_POINT ( 'NONE',  ( 66.72974708835175761, 13.56459745268607087, -76.59956076421927662 ) ) ;
#21394=B_SPLINE_CURVE_WITH_KNOTS ( 'NONE', 3,
 ( #6959, #49857, #60766, #50222, #1688, #27710, #991, #12591, #55487, #65361, #33359, #6612, #12949, #51950, #2730, #14327, #46671, #13972, #3763, #40011, #61472, #50915 ),
 .UNSPECIFIED., .F., .F.,
 ( 4, 2, 2, 2, 2, 2, 2, 2, 2, 2, 4 ),
 ( 0.000000000000000000, 0.001288289306256240390, 0.002576578612512480781, 0.003864867918768720954, 0.005153157225024961562, 0.006441446531281201301, 0.007085591184409312064, 0.007729735837537421092, 0.009018025143793640883, 0.009662169796921762921, 0.01030631445004988149 ),
 .UNSPECIFIED. ) ;
#21397=CARTESIAN_POINT ( 'NONE',  ( -177.1540936177023298, 91.73126115633628785, 31.98316566157747332 ) ) ;
#21407=CARTESIAN_POINT ( 'NONE',  ( -173.1211646369891355, 88.63826465341151106, 30.82169460664101734 ) ) ;
#21408=CARTESIAN_POINT ( 'NONE',  ( 126.4318266066171930, 38.27072266789465971, 62.76314339832654809 ) ) ;
#21409=ORIENTED_EDGE ( 'NONE', *, *, #18655, .F. ) ;
#21411=EDGE_LOOP ( 'NONE', ( #55505, #18773 ) ) ;
#21414=CARTESIAN_POINT ( 'NONE',  ( -47.66823188586783289, 12.82507252420411881, 92.85681623549952235 ) ) ;
#21417=CARTESIAN_POINT ( 'NONE',  ( 69.97872708500212013, 14.39620413031757629, 93.80885834994377603 ) ) ;
#21420=CARTESIAN_POINT ( 'NONE',  ( -132.2199390322348336, 50.80243550247265460, 69.02423031754652527 ) ) ;
#21423=EDGE_LOOP ( 'NONE', ( #45279, #34765 ) ) ;
#21424=CARTESIAN_POINT ( 'NONE',  ( -100.6199109870225641, 33.06995330681461098, -88.87768113824378702 ) ) ;
#21426=CARTESIAN_POINT ( 'NONE',  ( -78.18897186942403721, 23.21604822208489338, 72.26275173013684139 ) ) ;
#21427=CARTESIAN_POINT ( 'NONE',  ( 212.1962110267000128, 117.2292732107321171, -71.04714369557829912 ) ) ;
#21429=CARTESIAN_POINT ( 'NONE',  ( 56.19211641164837800, 11.19288081156168602, -73.18788659422385479 ) ) ;
#21430=CARTESIAN_POINT ( 'NONE',  ( -76.31381168750409927, 21.43908608416555239, 18.21112609344433864 ) ) ;
#21434=DIRECTION ( 'NONE',  ( 0.000000000000000000, 0.000000000000000000, 1.000000000000000000 ) ) ;
#21435=ORIENTED_EDGE ( 'NONE', *, *, #47078, .F. ) ;
#21439=ORIENTED_EDGE ( 'NONE', *, *, #25240, .T. ) ;
#21440=CARTESIAN_POINT ( 'NONE',  ( -24.61094659556678010, 9.585225265507407499, -66.54939687623127043 ) ) ;
#21441=CARTESIAN_POINT ( 'NONE',  ( 56.53635105806414174, 11.26263375223564012, -47.00625827598132389 ) ) ;
#21444=ADVANCED_FACE ( 'NONE', ( #7253 ), #6895, .F. ) ;
#21452=EDGE_LOOP ( 'NONE', ( #19400, #29325 ) ) ;
#21454=CARTESIAN_POINT ( 'NONE',  ( -145.5195986658808920, 62.16746116576786818, 31.86476147939222514 ) ) ;
#21457=CARTESIAN_POINT ( 'NONE',  ( -6.843910203392214342, 7.836697961436722260, 71.91164237052761621 ) ) ;
#21465=CYLINDRICAL_SURFACE ( 'NONE', #64682, 7.500000000000013323 ) ;
#21468=CARTESIAN_POINT ( 'NONE',  ( -189.8071159312682710, 107.8771087123619736, -71.83549201025891762 ) ) ;
#21470=CARTESIAN_POINT ( 'NONE',  ( -98.46684543088103680, 30.88557736720386515, 71.32637121160307458 ) ) ;
#21471=ORIENTED_EDGE ( 'NONE', *, *, #26592, .F. ) ;
#21472=CARTESIAN_POINT ( 'NONE',  ( -74.40004226286974642, 20.74218500375952345, 31.74512071546088521 ) ) ;
#21473=ORIENTED_EDGE ( 'NONE', *, *, #45094, .F. ) ;
#21475=CARTESIAN_POINT ( 'NONE',  ( -118.8392474096542628, 43.20060570451235549, 8.676164318946312903 ) ) ;
#21476=CARTESIAN_POINT ( 'NONE',  ( -180.6213815675304488, 95.88446356933842196, 64.85668927554371521 ) ) ;
#21477=CARTESIAN_POINT ( 'NONE',  ( 126.4754729582248416, 37.14269484129876275, 65.21006343432689789 ) ) ;
#21482=CARTESIAN_POINT ( 'NONE',  ( 69.83617901654358207, 15.39919709983075258, 34.18378910825896355 ) ) ;
#21486=CARTESIAN_POINT ( 'NONE',  ( -27.48703802937315288, 8.975952825337598640, 44.09546302086310732 ) ) ;
#21487=CARTESIAN_POINT ( 'NONE',  ( -143.2587158300142107, 60.34092810886537706, -65.00150092923556144 ) ) ;
#21490=FACE_BOUND ( 'NONE', #63417, .T. ) ;
#21500=CARTESIAN_POINT ( 'NONE',  ( -119.6801029354225108, 43.71909921132878907, -73.46582779786149331 ) ) ;
#21504=CARTESIAN_POINT ( 'NONE',  ( -83.15209219203885027, 25.16621997697721724, 70.79312038800895834 ) ) ;
#21505=CARTESIAN_POINT ( 'NONE',  ( 42.03341093683043539, 9.782505851509640138, -89.78263700018763416 ) ) ;
#21509=DIRECTION ( 'NONE',  ( -0.000000000000000000, 1.000000000000000000, -0.000000000000000000 ) ) ;
#21511=B_SPLINE_CURVE_WITH_KNOTS ( 'NONE', 3,
 ( #65156, #60223, #18965, #40762, #39131, #61860, #48947, #60570, #22241, #43680, #22941, #16950, #27862, #38414, #46037, #59859, #11679, #54936, #33151, #33508, #28565, #29868, #1846, #54587, #23302, #6412, #49304, #44748, #22588, #17305, #56593, #40413, #44028, #3147, #13685, #44383, #65873, #35141, #8415, #12039, #24604, #67504, #65507, #6756, #1480, #30558, #31260 ),
 .UNSPECIFIED., .F., .F.,
 ( 4, 2, 2, 2, 2, 2, 2, 2, 2, 2, 2, 2, 1, 2, 2, 2, 2, 2, 2, 2, 2, 2, 2, 4 ),
 ( 0.000000000000000000, 0.001493793014771564818, 0.002240689522157346576, 0.002987586029543128335, 0.004481379044314701826, 0.005228275551700484018, 0.005975172059086265343, 0.007468965073857845340, 0.008215861581243648348, 0.008962758088629452224, 0.01045655110340105130, 0.01120344761078684304, 0.01195034411817263130, 0.01269724062555842130, 0.01344413713294421130, 0.01493793014771577221, 0.01568482665510154486, 0.01643172316248732098, 0.01792551617725886975, 0.01941930919203041853, 0.02016620569941620159, 0.02091310220680198464, 0.02240689522157354036, 0.02390068823634509954 ),
 .UNSPECIFIED. ) ;
#21513=CARTESIAN_POINT ( 'NONE',  ( 39.40195752203892710, -170.0000000000000000, 44.91383430596327742 ) ) ;
#21514=CARTESIAN_POINT ( 'NONE',  ( 112.4855833589208629, 31.04769103621673310, 83.63625584413014735 ) ) ;
#21516=CARTESIAN_POINT ( 'NONE',  ( 70.46452034227870342, 14.52462608639673292, -17.38126288549829113 ) ) ;
#21518=CARTESIAN_POINT ( 'NONE',  ( 135.0005116824454490, 43.29964618809726318, -50.93914690418067437 ) ) ;
#21519=CARTESIAN_POINT ( 'NONE',  ( -47.55316895016325418, 13.83165595246917157, -69.05820636316589400 ) ) ;
#21524=CARTESIAN_POINT ( 'NONE',  ( 37.70910994512002645, 9.209110272746707793, 56.94781516157431156 ) ) ;
#21525=CARTESIAN_POINT ( 'NONE',  ( 184.0270137565624964, 83.08990924474782958, 83.57409603390661346 ) ) ;
#21526=LINE ( 'NONE', #15912, #7203 ) ;
#21530=CARTESIAN_POINT ( 'NONE',  ( 91.67776154311745529, 22.27748043241296472, 15.91940090679946174 ) ) ;
#21531=CARTESIAN_POINT ( 'NONE',  ( -10.46803069297985900, 7.077485182625207649, 71.48343882395781179 ) ) ;
#21532=CARTESIAN_POINT ( 'NONE',  ( 212.0075063341774069, 118.7912820769029594, 8.154294459840707887 ) ) ;
#21534=CARTESIAN_POINT ( 'NONE',  ( 46.90222083990963142, 9.503928413859229707, -16.03507805835512556 ) ) ;
#21540=CARTESIAN_POINT ( 'NONE',  ( 129.1052153257904251, 39.78893484542955861, 15.98927307743317350 ) ) ;
#21541=CARTESIAN_POINT ( 'NONE',  ( 91.67776154311745529, 22.27748043241296472, -37.76970027412789932 ) ) ;
#21545=CARTESIAN_POINT ( 'NONE',  ( 150.7926588734435427, 52.63999027731879465, 13.48961824798760745 ) ) ;
#21546=CARTESIAN_POINT ( 'NONE',  ( -14.86245480583235690, 8.462548703819992468, 88.69022230593746770 ) ) ;
#21549=CARTESIAN_POINT ( 'NONE',  ( 62.04664474957769471, 12.44961624115901522, 17.92119150936918004 ) ) ;
#21557=CARTESIAN_POINT ( 'NONE',  ( 90.91356992076214283, 21.99794663086830937, -64.00549692677411429 ) ) ;
#21558=ORIENTED_EDGE ( 'NONE', *, *, #15706, .F. ) ;
#21560=CARTESIAN_POINT ( 'NONE',  ( -56.96214175905167565, 15.20165595797839586, -62.30395517612640077 ) ) ;
#21562=CARTESIAN_POINT ( 'NONE',  ( -0.5178428571329638519, 7.532057582089302095, 12.47706993293499522 ) ) ;
#21563=CARTESIAN_POINT ( 'NONE',  ( 174.2468109002382732, 73.34092405459590225, -40.63028982688571489 ) ) ;
#21567=ORIENTED_EDGE ( 'NONE', *, *, #25102, .T. ) ;
#21568=CARTESIAN_POINT ( 'NONE',  ( -47.94960849910474110, 13.92522873833625141, -40.25875785308206645 ) ) ;
#21571=CARTESIAN_POINT ( 'NONE',  ( 8.336237313193160858, 7.382629160459399209, 38.49233202133056864 ) ) ;
#21576=ORIENTED_EDGE ( 'NONE', *, *, #47700, .F. ) ;
#21579=CARTESIAN_POINT ( 'NONE',  ( -51.99406906667273631, 13.88268392809765217, 44.66953586812910260 ) ) ;
#21583=CARTESIAN_POINT ( 'NONE',  ( -62.54086041493278714, 17.86944394914986489, -42.22520487807840084 ) ) ;
#21585=CARTESIAN_POINT ( 'NONE',  ( 149.9838583332407893, 52.05699766415858676, -70.99723250371756933 ) ) ;
#21586=CARTESIAN_POINT ( 'NONE',  ( 19.75784582661440680, 6.660183274347839522, -9.806260835590238756 ) ) ;
#21588=CARTESIAN_POINT ( 'NONE',  ( -156.6819053601226415, 70.51177710383656461, -40.05411599417865176 ) ) ;
#21591=EDGE_CURVE ( 'NONE', #45287, #13481, #27777, .T. ) ;
#21596=CARTESIAN_POINT ( 'NONE',  ( -82.33596576276353574, 24.83688096733770934, -36.05641134141605164 ) ) ;
#21597=CARTESIAN_POINT ( 'NONE',  ( -24.07713913638673731, 9.513388522963451166, 92.87435816855477810 ) ) ;
#21598=CARTESIAN_POINT ( 'NONE',  ( -153.6994314938756077, 69.16570456337670691, 17.61204298921591516 ) ) ;
#21602=CARTESIAN_POINT ( 'NONE',  ( 22.29513692215318343, 6.796052026456514739, 33.75287157804441307 ) ) ;
#21606=ORIENTED_EDGE ( 'NONE', *, *, #46598, .F. ) ;
#21608=CARTESIAN_POINT ( 'NONE',  ( -152.9143627383494959, 68.46626892668653852, -8.771231553591714913 ) ) ;
#21609=CARTESIAN_POINT ( 'NONE',  ( 32.66883187925819954, 8.640402022338109944, -46.46001169007210763 ) ) ;
#21611=CARTESIAN_POINT ( 'NONE',  ( -34.51918258780366955, 10.11719938103012417, 57.71828778730281329 ) ) ;
#21614=CARTESIAN_POINT ( 'NONE',  ( 181.5079096844946491, 80.47139261082472217, 56.15314469597509373 ) ) ;
#21617=CARTESIAN_POINT ( 'NONE',  ( 23.28809538736928531, 7.864824219997530008, 11.16234900110744732 ) ) ;
#21618=CARTESIAN_POINT ( 'NONE',  ( 106.0171289417044136, 26.97542621030656207, 16.46741202603713816 ) ) ;
#21620=CARTESIAN_POINT ( 'NONE',  ( -85.35127931077731489, 24.98147633333001494, -46.02518267684259001 ) ) ;
#21621=CARTESIAN_POINT ( 'NONE',  ( 22.89634831467700593, 6.832298124325686395, 66.76462710434758208 ) ) ;
#21622=ADVANCED_FACE ( 'NONE', ( #20225 ), #67392, .F. ) ;
#21624=CARTESIAN_POINT ( 'NONE',  ( 8.288104306525687193, 6.376394648992966374, -70.35007307862180426 ) ) ;
#21625=ORIENTED_EDGE ( 'NONE', *, *, #19695, .T. ) ;
#21628=CARTESIAN_POINT ( 'NONE',  ( 173.5843421840238250, 71.34465141434345981, 37.11183576288200925 ) ) ;
#21629=DIRECTION ( 'NONE',  ( -0.000000000000000000, 1.000000000000000000, -0.000000000000000000 ) ) ;
#21630=CARTESIAN_POINT ( 'NONE',  ( 45.90128843543705983, 9.343910238294478532, -73.73932652712356628 ) ) ;
#21631=CARTESIAN_POINT ( 'NONE',  ( 56.29445224195347919, 12.24017809212661767, -73.42969269962038936 ) ) ;
#21635=CARTESIAN_POINT ( 'NONE',  ( 198.7129816317746815, 100.1061386900356354, 14.39133888418318463 ) ) ;
#21638=CARTESIAN_POINT ( 'NONE',  ( 115.7561705820728832, 31.51689401996054940, 58.84795663990033177 ) ) ;
#21640=CARTESIAN_POINT ( 'NONE',  ( 116.6436511186860798, 33.08230081168869674, 67.87302575006638961 ) ) ;
#21642=CARTESIAN_POINT ( 'NONE',  ( 134.3135005523731706, 42.87884033955813834, 56.36529494589373712 ) ) ;
#21645=CARTESIAN_POINT ( 'NONE',  ( 161.0127366078917532, 60.45848280706938738, -90.69197953650788691 ) ) ;
#21646=ADVANCED_FACE ( 'NONE', ( #62452 ), #51209, .F. ) ;
#21647=CARTESIAN_POINT ( 'NONE',  ( 91.11342358617756076, 21.00000175105273570, -49.33836006142978903 ) ) ;
#21653=ORIENTED_EDGE ( 'NONE', *, *, #59283, .F. ) ;
#21655=ADVANCED_FACE ( 'NONE', ( #62096 ), #30438, .F. ) ;
#21657=CARTESIAN_POINT ( 'NONE',  ( 8.000000000000007105, 249.8719672152120381, -95.00000000000133582 ) ) ;
#21658=CARTESIAN_POINT ( 'NONE',  ( 39.88971011078924533, 8.472992116645412963, -50.61981746542778637 ) ) ;
#21659=CARTESIAN_POINT ( 'NONE',  ( -165.9121868482145885, 80.88751546905562861, -71.14685045223694715 ) ) ;
#21660=CARTESIAN_POINT ( 'NONE',  ( -144.2029146819478171, 59.80706661873674079, -36.98889646392695596 ) ) ;
#21661=ORIENTED_EDGE ( 'NONE', *, *, #728, .F. ) ;
#21662=CARTESIAN_POINT ( 'NONE',  ( 55.52751777340359496, 12.08567914268658683, 10.95808945309540405 ) ) ;
#21666=CARTESIAN_POINT ( 'NONE',  ( -131.2803255164624829, 50.14412978403780841, 43.34457761225254302 ) ) ;
#21668=CARTESIAN_POINT ( 'NONE',  ( 81.76092782665034520, 17.81692437267513895, -10.76658827783151118 ) ) ;
#21669=CARTESIAN_POINT ( 'NONE',  ( 87.10668362745094839, 19.58396519288861981, -77.66611478937539914 ) ) ;
#21670=DIRECTION ( 'NONE',  ( -1.000000000000000000, 0.000000000000000000, 0.000000000000000000 ) ) ;
#21671=CARTESIAN_POINT ( 'NONE',  ( -96.45845418068302024, 29.92035703021963755, 6.419777494690062980 ) ) ;
#21672=CARTESIAN_POINT ( 'NONE',  ( -155.3953402213948038, 69.33856625680883212, -91.33370433575318259 ) ) ;
#21676=CARTESIAN_POINT ( 'NONE',  ( 187.2465631085773339, 85.06582225041682932, -66.26497931038906586 ) ) ;
#21677=CARTESIAN_POINT ( 'NONE',  ( 15.78827728214693416, 7.507518794609576496, -35.51894409868578606 ) ) ;
#21680=CARTESIAN_POINT ( 'NONE',  ( 107.0447263249841399, 28.53200276018955606, -63.47887945344969296 ) ) ;
#21681=CARTESIAN_POINT ( 'NONE',  ( 83.37786665291103816, 18.33670623396829313, 43.98793584344309693 ) ) ;
#21683=CARTESIAN_POINT ( 'NONE',  ( 45.35146934743632841, 10.27620685439441850, -38.52673262789923569 ) ) ;
#21684=CARTESIAN_POINT ( 'NONE',  ( 212.0850679406002826, 117.0583048437721629, 64.89170834392957943 ) ) ;
#21686=CARTESIAN_POINT ( 'NONE',  ( -109.7793173546317291, 36.75648380851388453, -15.38638933786221763 ) ) ;
#21688=CARTESIAN_POINT ( 'NONE',  ( -15.13254930056756820, 7.477527548005404867, -41.21022013649527338 ) ) ;
#21690=CARTESIAN_POINT ( 'NONE',  ( -85.86555129592289859, 25.19562892552701783, 93.80983709230186207 ) ) ;
#21691=CARTESIAN_POINT ( 'NONE',  ( 87.59078297315399197, 20.81577753000345865, 56.60314402004118506 ) ) ;
#21692=CARTESIAN_POINT ( 'NONE',  ( 154.0401952541423611, 55.03227529428313147, -10.10604738963787419 ) ) ;
#21694=CARTESIAN_POINT ( 'NONE',  ( -95.04371414958065145, 30.36527049547257562, -71.39807560214309490 ) ) ;
#21698=AXIS2_PLACEMENT_3D ( 'NONE', #3021, #41346, #8993 ) ;
#21699=CARTESIAN_POINT ( 'NONE',  ( 211.5481110227417503, 116.2365999939639920, 93.47554241977024958 ) ) ;
#21705=CARTESIAN_POINT ( 'NONE',  ( 39.40195752203891999, 9.424259417798142024, -62.46436805589144114 ) ) ;
#21706=CARTESIAN_POINT ( 'NONE',  ( -6.126800896373027605, 6.786243985899686137, 30.30631899384127692 ) ) ;
#21709=CARTESIAN_POINT ( 'NONE',  ( -102.2801239173131052, 33.91021738430207222, -50.01457726497594081 ) ) ;
#21714=CARTESIAN_POINT ( 'NONE',  ( -189.7334103489410495, 107.7745063523401114, -17.96279510330434448 ) ) ;
#21716=CARTESIAN_POINT ( 'NONE',  ( -166.3205068063721512, 81.30869308872871670, -45.38659965827987008 ) ) ;
#21717=CARTESIAN_POINT ( 'NONE',  ( -180.6286109613758981, 95.89331854612689199, 92.18987725550799439 ) ) ;
#21721=CARTESIAN_POINT ( 'NONE',  ( 201.5876148766342908, 103.8397408698164952, -10.14323620147940908 ) ) ;
#21722=CARTESIAN_POINT ( 'NONE',  ( -146.1757827157406666, 61.40416249728257725, 85.18476316236196055 ) ) ;
#21723=CARTESIAN_POINT ( 'NONE',  ( 139.1353280997809634, 44.70436000187871173, 42.34369417666323443 ) ) ;
#21727=CARTESIAN_POINT ( 'NONE',  ( 164.6598737201887559, 64.78038692612517480, 7.858682584642552094 ) ) ;
#21730=CARTESIAN_POINT ( 'NONE',  ( 176.6156959113758660, 75.60152827082542615, 69.69554617303106170 ) ) ;
#21732=ORIENTED_EDGE ( 'NONE', *, *, #1181, .T. ) ;
#21733=CARTESIAN_POINT ( 'NONE',  ( -71.67841390531691559, 19.78168466957075822, -18.50581070427913843 ) ) ;
#21735=CARTESIAN_POINT ( 'NONE',  ( 9.319975126229035567, 6.379801983805998944, 94.99999999999866418 ) ) ;
#21739=LINE ( 'NONE', #23149, #19591 ) ;
#21740=EDGE_CURVE ( 'NONE', #31531, #40675, #37871, .T. ) ;
#21741=CARTESIAN_POINT ( 'NONE',  ( 150.3360255159550150, 53.55172128635252449, -95.00000000000133582 ) ) ;
#21747=VECTOR ( 'NONE', #26834, 1000.000000000000000 ) ;
#21749=CARTESIAN_POINT ( 'NONE',  ( -180.2188652555596775, 96.98354576637426305, 35.88108729135068842 ) ) ;
#21751=CARTESIAN_POINT ( 'NONE',  ( -38.16002576456688899, 10.79155573432543669, -72.99943442513966829 ) ) ;
#21752=EDGE_CURVE ( 'NONE', #27576, #564, #31170, .T. ) ;
#21761=CARTESIAN_POINT ( 'NONE',  ( -107.0206060416819014, 35.25485366694522327, 85.88817087773396963 ) ) ;
#21764=CARTESIAN_POINT ( 'NONE',  ( 8.000000000000007105, 249.8719672152120381, -95.00000000000133582 ) ) ;
#21770=CARTESIAN_POINT ( 'NONE',  ( 187.2354698746856627, 85.05376776489249835, 32.48870243768265453 ) ) ;
#21772=CARTESIAN_POINT ( 'NONE',  ( -7.825402957745085430, -170.0000000000000000, 30.11558103944718923 ) ) ;
#21773=CARTESIAN_POINT ( 'NONE',  ( -37.61622737004960015, 10.68719896441377237, -92.24730381973596138 ) ) ;
#21774=CARTESIAN_POINT ( 'NONE',  ( -190.6985136298601731, 109.1272424661242582, 94.99999999999866418 ) ) ;
#21775=CARTESIAN_POINT ( 'NONE',  ( 197.2089704088280087, 96.60702177658571088, 89.92753103993992170 ) ) ;
#21776=DIRECTION ( 'NONE',  ( -0.000000000000000000, 1.000000000000000000, -0.000000000000000000 ) ) ;
#21784=CARTESIAN_POINT ( 'NONE',  ( 40.38495044702527537, 9.554194848483444247, 29.96251898938304592 ) ) ;
#21786=AXIS2_PLACEMENT_3D ( 'NONE', #55283, #39812, #66910 ) ;
#21787=CARTESIAN_POINT ( 'NONE',  ( -142.1381007084227122, 58.17237452544245002, 9.955516383538055791 ) ) ;
#21791=CARTESIAN_POINT ( 'NONE',  ( -132.4776673493542773, 52.21763813822160216, 34.51875723904359461 ) ) ;
#21795=LINE ( 'NONE', #10551, #9403 ) ;
#21796=EDGE_CURVE ( 'NONE', #19003, #30189, #18077, .T. ) ;
#21804=ORIENTED_EDGE ( 'NONE', *, *, #45424, .F. ) ;
#21810=CARTESIAN_POINT ( 'NONE',  ( 65.40032188136233060, 13.23841673691966569, 30.19802725762940554 ) ) ;
#21814=ORIENTED_EDGE ( 'NONE', *, *, #63859, .T. ) ;
#21816=CARTESIAN_POINT ( 'NONE',  ( -78.66644367742109978, 22.32174330031319442, 30.41820113967310490 ) ) ;
#21819=CARTESIAN_POINT ( 'NONE',  ( -142.1381007084227122, 58.17237452544243581, -70.57813538785298135 ) ) ;
#21822=CARTESIAN_POINT ( 'NONE',  ( -149.5074843970971301, -170.0000000000000000, 11.37627064943538890 ) ) ;
#21823=VERTEX_POINT ( 'NONE', #39526 ) ;
#21826=CARTESIAN_POINT ( 'NONE',  ( 153.2282895792479849, 54.42637815496162546, 30.71980616472758996 ) ) ;
#21832=EDGE_CURVE ( 'NONE', #43301, #31528, #51348, .T. ) ;
#21833=CARTESIAN_POINT ( 'NONE',  ( -24.70911172866235361, 8.583078995053023519, 34.36983212919319897 ) ) ;
#21834=DIRECTION ( 'NONE',  ( 0.9115451497320358198, -0.4112000000000002875, 0.000000000000000000 ) ) ;
#21838=FACE_BOUND ( 'NONE', #46301, .T. ) ;
#21839=ADVANCED_FACE ( 'NONE', ( #39870 ), #47462, .F. ) ;
#21840=CARTESIAN_POINT ( 'NONE',  ( -0.5158933718595631879, 6.525180340836110204, -68.06532982274359256 ) ) ;
#21842=CARTESIAN_POINT ( 'NONE',  ( -177.1514380519393512, 93.28180884530867445, 71.50650821116707334 ) ) ;
#21845=CARTESIAN_POINT ( 'NONE',  ( -85.36298448216592760, 26.07611629625833416, 14.48877058237737181 ) ) ;
#21848=CARTESIAN_POINT ( 'NONE',  ( -152.9119739516381458, 67.12135129037712034, 4.678041278420704607 ) ) ;
#21849=CARTESIAN_POINT ( 'NONE',  ( -72.69566972648141245, 20.13629716597854369, -91.74463633560024789 ) ) ;
#21850=VECTOR ( 'NONE', #65405, 1000.000000000000000 ) ;
#21851=CARTESIAN_POINT ( 'NONE',  ( 69.49862690228273721, 14.27023134440513630, 6.665126176731966723 ) ) ;
#21852=CARTESIAN_POINT ( 'NONE',  ( -79.14638003838379632, 23.58242782405879012, 72.26275173013684139 ) ) ;
#21853=CARTESIAN_POINT ( 'NONE',  ( 44.63883881567345213, 10.16630920665935278, -91.43600144160676280 ) ) ;
#21855=CARTESIAN_POINT ( 'NONE',  ( -34.52542994698666945, 11.14027065218092183, 17.71174954528721202 ) ) ;
#21858=CARTESIAN_POINT ( 'NONE',  ( 109.3079614081140676, 28.45126415661779973, -62.81087680795587147 ) ) ;
#21860=CARTESIAN_POINT ( 'NONE',  ( 86.14890207173840508, 20.31981596387580069, -62.66611478937539204 ) ) ;
#21861=CARTESIAN_POINT ( 'NONE',  ( 103.3565118956568938, 26.91828102196332750, 93.79128338615151961 ) ) ;
#21862=CARTESIAN_POINT ( 'NONE',  ( -142.3260422482980516, 59.60034523324940636, 67.30005160776828177 ) ) ;
#21863=CARTESIAN_POINT ( 'NONE',  ( 66.94779593213118574, 13.61918177102165828, -9.984881045247117726 ) ) ;
#21864=CARTESIAN_POINT ( 'NONE',  ( -24.71645982722742119, 9.599558729461495687, -39.48295160479800359 ) ) ;
#21865=CARTESIAN_POINT ( 'NONE',  ( -47.61402178322637724, 13.84598486314982146, -70.54967370588845199 ) ) ;
#21867=CARTESIAN_POINT ( 'NONE',  ( -119.5404913382139824, 43.63271406506957106, -19.56318599381059897 ) ) ;
#21870=CARTESIAN_POINT ( 'NONE',  ( 32.15613847490628530, 8.588587416860169910, 62.30661714676169538 ) ) ;
#21871=CARTESIAN_POINT ( 'NONE',  ( -167.1619226259398943, 82.18315278115414912, 60.60531548443081817 ) ) ;
#21872=CARTESIAN_POINT ( 'NONE',  ( 128.9266876467504233, 39.68626248249439215, -91.54607739640439945 ) ) ;
#21874=CARTESIAN_POINT ( 'NONE',  ( 69.47389377197907834, 15.30385359588022709, -93.07428216817731936 ) ) ;
#21877=CARTESIAN_POINT ( 'NONE',  ( 186.6075385349484179, 85.85749512876286360, -21.97869164680669840 ) ) ;
#21878=CARTESIAN_POINT ( 'NONE',  ( 211.7318474105134669, 118.3631723164074856, 7.243756357567826321 ) ) ;
#21880=DIRECTION ( 'NONE',  ( -0.000000000000000000, 1.000000000000000000, -0.000000000000000000 ) ) ;
#21882=DIRECTION ( 'NONE',  ( -0.000000000000000000, 1.000000000000000000, -0.000000000000000000 ) ) ;
#21883=CARTESIAN_POINT ( 'NONE',  ( 164.1338586910085837, 64.33646242148853389, 67.20636812611378730 ) ) ;
#21886=ORIENTED_EDGE ( 'NONE', *, *, #15426, .F. ) ;
#21887=DIRECTION ( 'NONE',  ( -1.000000000000000000, 0.000000000000000000, 0.000000000000000000 ) ) ;
#21888=CARTESIAN_POINT ( 'NONE',  ( 92.20490818459943227, 22.47175429302964034, -38.28145556619914913 ) ) ;
#21890=CARTESIAN_POINT ( 'NONE',  ( -48.34500911884042296, 14.01939034823941910, 68.02609795225436073 ) ) ;
#21893=DIRECTION ( 'NONE',  ( 0.000000000000000000, 0.000000000000000000, 1.000000000000000000 ) ) ;
#21895=AXIS2_PLACEMENT_3D ( 'NONE', #24423, #30378, #25464 ) ;
#21896=ORIENTED_EDGE ( 'NONE', *, *, #7722, .T. ) ;
#21898=EDGE_CURVE ( 'NONE', #7404, #47113, #18767, .T. ) ;
#21899=EDGE_CURVE ( 'NONE', #57172, #54901, #36590, .T. ) ;
#21907=CARTESIAN_POINT ( 'NONE',  ( 93.08174259058945665, 22.79847752828721141, -66.31129219526786756 ) ) ;
#21908=VERTEX_POINT ( 'NONE', #62010 ) ;
#21909=EDGE_CURVE ( 'NONE', #4017, #30296, #9350, .T. ) ;
#21910=CARTESIAN_POINT ( 'NONE',  ( -55.53469534616547065, 14.81076603075805664, -77.06087458892359621 ) ) ;
#21911=CARTESIAN_POINT ( 'NONE',  ( 36.76746179515744473, 8.081433644308896547, -9.248917121289487397 ) ) ;
#21912=CARTESIAN_POINT ( 'NONE',  ( 177.0027897064244371, 75.97676392242546228, -37.41656822527980353 ) ) ;
#21913=CARTESIAN_POINT ( 'NONE',  ( 164.9657042191946061, 63.72163127919190373, 90.13840011216286996 ) ) ;
#21916=CARTESIAN_POINT ( 'NONE',  ( -49.13048465129993048, 14.20828170588045758, -38.08805284523984369 ) ) ;
#21918=CARTESIAN_POINT ( 'NONE',  ( 11.82929895397812992, 7.412564870773605818, 31.13995448514249631 ) ) ;
#21923=ORIENTED_EDGE ( 'NONE', *, *, #1936, .T. ) ;
#21924=EDGE_CURVE ( 'NONE', #7404, #23453, #48808, .T. ) ;
#21927=CARTESIAN_POINT ( 'NONE',  ( -11.57808265946729875, 7.164483090579918390, -22.57181510547873771 ) ) ;
#21928=CARTESIAN_POINT ( 'NONE',  ( -54.56693200831792723, 14.55131601960338905, 45.31732777293116499 ) ) ;
#21932=CARTESIAN_POINT ( 'NONE',  ( -38.17232309348613484, 11.81874355808867350, 67.90144012224213554 ) ) ;
#21933=CARTESIAN_POINT ( 'NONE',  ( -11.78188048797445475, 8.190559674012728664, -22.44981765585516698 ) ) ;
#21934=CARTESIAN_POINT ( 'NONE',  ( 153.2384531768736053, 54.43344429203624202, -64.25936496073454407 ) ) ;
#21943=CARTESIAN_POINT ( 'NONE',  ( -61.26061298622803974, 17.48391647823794059, -92.17393543469286499 ) ) ;
#21944=CARTESIAN_POINT ( 'NONE',  ( 117.7395339318602652, 32.50726632670704674, 90.38096001386408318 ) ) ;
#21945=CARTESIAN_POINT ( 'NONE',  ( -151.2511071212632032, 67.00426547928871912, 18.68401857637098473 ) ) ;
#21955=VERTEX_POINT ( 'NONE', #18592 ) ;
#21957=CARTESIAN_POINT ( 'NONE',  ( -156.9262190792699698, 72.10659547035872663, -14.32972382511977116 ) ) ;
#21958=CARTESIAN_POINT ( 'NONE',  ( 32.30062460741315533, 8.603096374765343057, -45.54517555199483070 ) ) ;
#21962=CARTESIAN_POINT ( 'NONE',  ( 86.62931800182293784, 20.48449268398422873, -50.82156419891174437 ) ) ;
#21963=CARTESIAN_POINT ( 'NONE',  ( -156.0171627975467743, 69.90368824761766575, 68.79920456856257260 ) ) ;
#21964=CARTESIAN_POINT ( 'NONE',  ( -1.328627985309864590, 7.561890325089884790, -46.67342399825810162 ) ) ;
#21965=CARTESIAN_POINT ( 'NONE',  ( 105.2506154496929582, 26.63995206619728506, 15.86906671377738576 ) ) ;
#21967=CARTESIAN_POINT ( 'NONE',  ( -83.52505811737955810, 24.23179517241434411, -48.35018627393339585 ) ) ;
#21970=CARTESIAN_POINT ( 'NONE',  ( 8.951900209438534262, 6.378066731449594684, -72.95773463900229672 ) ) ;
#21975=CARTESIAN_POINT ( 'NONE',  ( 179.0096185093687779, 76.53352131383243773, 29.58811944080985512 ) ) ;
#21981=B_SPLINE_CURVE_WITH_KNOTS ( 'NONE', 3,
 ( #23247, #6354, #60858, #12681, #34147, #7416, #49247, #43971, #49954, #55945, #22884, #54527, #28868, #1080, #7760, #50319, #54880, #22532, #6702, #39760, #16898, #2137, #23589, #65453, #65099, #17247, #66510, #38716, #65813, #60162, #13043, #33453, #29209, #11982, #28148, #17608, #49595, #1427, #44327, #39074, #33790, #7051, #28510, #41494, #8449 ),
 .UNSPECIFIED., .F., .F.,
 ( 4, 2, 2, 2, 2, 2, 2, 2, 2, 2, 2, 2, 2, 1, 2, 2, 2, 2, 2, 2, 2, 2, 4 ),
 ( 0.02356759485890610670, 0.02503765354686417546, 0.02577268289084322372, 0.02650771223482226852, 0.02797777092278037545, 0.02944782961073848238, 0.03018285895471753758, 0.03091788829869659277, 0.03238794698665466848, 0.03312297633063371327, 0.03385800567461275806, 0.03532806436257082683, 0.03606309370654985080, 0.03679812305052886784, 0.03753315239450789181, 0.03826818173848690885, 0.03973824042644495680, 0.04120829911440300475, 0.04267835780236105270, 0.04341338714634006279, 0.04414841649031907983, 0.04561847517827709309, 0.04708853386623509940 ),
 .UNSPECIFIED. ) ;
#21982=VERTEX_POINT ( 'NONE', #61157 ) ;
#21983=CARTESIAN_POINT ( 'NONE',  ( -126.3071720906782076, 46.76607039798766863, -88.60280507916129977 ) ) ;
#21985=CARTESIAN_POINT ( 'NONE',  ( 184.0196598574194411, 81.62390236021667533, 83.58993435411535700 ) ) ;
#21994=CARTESIAN_POINT ( 'NONE',  ( 105.2147050270618820, 27.72205961956172260, -91.53208825577468133 ) ) ;
#21997=CARTESIAN_POINT ( 'NONE',  ( 141.2361973397653117, 47.26569015399784490, 65.21956349169761324 ) ) ;
#21998=CARTESIAN_POINT ( 'NONE',  ( -75.43044859198177221, 21.11535168543637297, -35.84517485573555007 ) ) ;
#22000=CARTESIAN_POINT ( 'NONE',  ( -96.00016893459647349, 29.70347032303887502, 42.12695562128465099 ) ) ;
#22003=CARTESIAN_POINT ( 'NONE',  ( -189.2352924136013996, 107.0839554967701304, 37.97586783404467070 ) ) ;
#22009=CIRCLE ( 'NONE', #63601, 242.4895526022646379 ) ;
#22011=CARTESIAN_POINT ( 'NONE',  ( 42.70988075781784943, 8.862408058333471672, -49.86848500202146539 ) ) ;
#22013=CARTESIAN_POINT ( 'NONE',  ( -142.9730935922300148, 58.82921737386682537, -38.62225429887013917 ) ) ;
#22015=CARTESIAN_POINT ( 'NONE',  ( -173.1211646369891355, -170.0000000000000000, 72.66624519710475738 ) ) ;
#22016=EDGE_LOOP ( 'NONE', ( #61763, #57213 ) ) ;
#22017=CARTESIAN_POINT ( 'NONE',  ( -31.43908319763710679, -170.0000000000000000, -42.81719736520184938 ) ) ;
#22021=DIRECTION ( 'NONE',  ( 0.000000000000000000, -1.000000000000000000, 0.000000000000000000 ) ) ;
#22022=CARTESIAN_POINT ( 'NONE',  ( 89.88695630745282017, 20.55793566325393584, -63.39359200686787688 ) ) ;
#22024=CARTESIAN_POINT ( 'NONE',  ( -97.49219489034497599, 30.41416107059307805, 5.381099477080671711 ) ) ;
#22027=ORIENTED_EDGE ( 'NONE', *, *, #44042, .T. ) ;
#22028=CARTESIAN_POINT ( 'NONE',  ( 45.02738683369922512, 9.207938468499239804, 32.44741314349040806 ) ) ;
#22029=CARTESIAN_POINT ( 'NONE',  ( 12.46704290855393360, 6.417105965824392300, 30.78567100710504789 ) ) ;
#22030=CARTESIAN_POINT ( 'NONE',  ( 63.01563776193091826, -170.0000000000000000, -70.06524142263343435 ) ) ;
#22032=CARTESIAN_POINT ( 'NONE',  ( 210.9608386442062624, 117.1762372255316365, -39.69180030939477888 ) ) ;
#22034=CARTESIAN_POINT ( 'NONE',  ( -190.6985136298602015, 109.1272424661243434, 16.02916387300914280 ) ) ;
#22035=CARTESIAN_POINT ( 'NONE',  ( 44.34689728705970424, 10.12166135033765357, -37.45970703709721050 ) ) ;
#22038=CARTESIAN_POINT ( 'NONE',  ( -27.70115495247213033, 10.02455692117573882, 17.39240037915121206 ) ) ;
#22041=CARTESIAN_POINT ( 'NONE',  ( -11.57808265946730586, 7.164483090579920166, -49.41636569594241024 ) ) ;
#22045=CARTESIAN_POINT ( 'NONE',  ( 31.91383250562745388, 8.564461488296998937, 11.05764693793517139 ) ) ;
#22047=CARTESIAN_POINT ( 'NONE',  ( -96.77705718164442317, 31.18700926299569787, -64.23949498694426552 ) ) ;
#22048=CARTESIAN_POINT ( 'NONE',  ( 116.7923802250937371, 33.15684512294094333, -93.43283724407298507 ) ) ;
#22056=CARTESIAN_POINT ( 'NONE',  ( -8.800520192024523070, 7.964629484975262130, 3.318412053709786758 ) ) ;
#22058=CARTESIAN_POINT ( 'NONE',  ( 41.33434189587761409, 9.684413566891873160, -62.71343792220747559 ) ) ;
#22059=CARTESIAN_POINT ( 'NONE',  ( -5.401648928593166588, 6.744888135494082171, 44.72991648308484258 ) ) ;
#22062=CARTESIAN_POINT ( 'NONE',  ( 93.28147497731882254, 22.87326625539070335, 94.43110130039434580 ) ) ;
#22063=AXIS2_PLACEMENT_3D ( 'NONE', #48394, #57611, #53340 ) ;
#22069=CARTESIAN_POINT ( 'NONE',  ( -168.1839487819771364, 83.25723186408067988, -36.56132926469148003 ) ) ;
#22071=CARTESIAN_POINT ( 'NONE',  ( -173.1211646369891355, 87.12891641440857882, -61.55650775521367279 ) ) ;
#22074=B_SPLINE_CURVE_WITH_KNOTS ( 'NONE', 3,
 ( #31380, #30688, #8548, #26098, #41582, #24729, #8891, #52138, #62352, #40891, #14165, #47197, #35964, #30344, #9580, #58108, #35627, #30000, #25423, #46863, #46506, #9925, #61993, #19786, #14844, #63391, #36311, #40542, #41249, #57766, #13809, #31039, #52813, #35273, #52483, #4306, #25768, #68654, #20464, #41927, #15198, #37329, #54545, #43291, #26448, #49264 ),
 .UNSPECIFIED., .F., .F.,
 ( 4, 2, 2, 2, 2, 2, 2, 2, 2, 2, 2, 2, 2, 2, 2, 2, 2, 2, 2, 2, 2, 2, 4 ),
 ( 3.122502256758252770E-17, 0.001572224531395700550, 0.003144449062791369875, 0.004716673594187039201, 0.006288898125582708526, 0.007861122656978377851, 0.009433347188374047176, 0.01021945945407186709, 0.01100557171976968875, 0.01179168398546750866, 0.01257779625116533032, 0.01415002078256097189, 0.01493613304825880048, 0.01572224531395662733, 0.01650835757965446113, 0.01729446984535228798, 0.01886669437674788966, 0.01965280664244568876, 0.02043891890814348439, 0.02201114343953908259, 0.02358336797093467732, 0.02436948023663247295, 0.02515559250233026511 ),
 .UNSPECIFIED. ) ;
#22075=CARTESIAN_POINT ( 'NONE',  ( -4.725257700476006129, 6.708862164351558910, -9.239876348931433725 ) ) ;
#22076=CARTESIAN_POINT ( 'NONE',  ( 197.2199569260504006, 98.22436319491366419, -16.31760007026884551 ) ) ;
#22077=CARTESIAN_POINT ( 'NONE',  ( -145.4293260530172631, 60.79600197597825684, 85.60900646559132099 ) ) ;
#22078=EDGE_CURVE ( 'NONE', #21823, #23678, #54264, .T. ) ;
#22081=CARTESIAN_POINT ( 'NONE',  ( -190.6985136298601731, 109.1272424661242582, 94.99999999999866418 ) ) ;
#22082=CARTESIAN_POINT ( 'NONE',  ( 84.26390409839197559, 19.68678207880320841, 17.50091665772310989 ) ) ;
#22084=CARTESIAN_POINT ( 'NONE',  ( -97.88021438939451002, 31.71889184683103480, 44.11149307090948213 ) ) ;
#22085=CARTESIAN_POINT ( 'NONE',  ( -0.4996266546846072631, -170.0000000000000000, -95.00000000000133582 ) ) ;
#22089=VERTEX_POINT ( 'NONE', #67480 ) ;
#22091=CARTESIAN_POINT ( 'NONE',  ( -121.9166680696882850, 43.93013778640997202, -89.72953050740939318 ) ) ;
#22094=CARTESIAN_POINT ( 'NONE',  ( 150.0980941434704619, 53.37942190380064034, 8.659987245234894715 ) ) ;
#22096=CARTESIAN_POINT ( 'NONE',  ( 164.8942204024298235, 63.66138186734713855, 38.01188527962676034 ) ) ;
#22097=DIRECTION ( 'NONE',  ( -0.8160245890732938934, -0.5780171883497599028, 0.000000000000000000 ) ) ;
#22099=AXIS2_PLACEMENT_3D ( 'NONE', #13100, #65165, #38427 ) ;
#22104=CARTESIAN_POINT ( 'NONE',  ( 153.6158476725599371, 54.71469178023152580, -90.86794399618655405 ) ) ;
#22105=CARTESIAN_POINT ( 'NONE',  ( 129.5225439633634608, 40.02995148249141266, 57.71575578625421343 ) ) ;
#22106=ORIENTED_EDGE ( 'NONE', *, *, #43705, .T. ) ;
#22110=CARTESIAN_POINT ( 'NONE',  ( -47.81209834363054512, 12.85890427894798727, 93.48825161138802287 ) ) ;
#22113=CARTESIAN_POINT ( 'NONE',  ( 70.10607374715122830, 14.42976827319814426, 88.53455713664466487 ) ) ;
#22119=CARTESIAN_POINT ( 'NONE',  ( -101.4485769343308021, 33.48710798375949338, -88.73808582770939779 ) ) ;
#22122=CARTESIAN_POINT ( 'NONE',  ( 212.0047492081761504, 116.9348962082588770, -72.39146962302672250 ) ) ;
#22123=B_SPLINE_CURVE_WITH_KNOTS ( 'NONE', 3,
 ( #61119, #23842, #34748, #67793, #3082, #56184, #62152, #8000, #45639, #67116, #18909, #40355, #35081, #56531, #67448, #8358, #51271, #24545, #45981, #19239, #13969, #35431, #51609, #56894, #8709, #30162, #14660, #41740, #10756, #32223, #25231, #5136, #52965, #63201, #42426, #47016, #19950, #36121, #42759, #62859, #42080, #46668, #57582, #68475, #9388, #25916 ),
 .UNSPECIFIED., .F., .F.,
 ( 4, 2, 2, 2, 2, 2, 2, 2, 2, 2, 2, 2, 2, 2, 2, 2, 2, 2, 2, 2, 2, 2, 4 ),
 ( 0.000000000000000000, 0.003635178948345819169, 0.005452768422518699913, 0.007270357896691580224, 0.008179152633778006068, 0.009087947370864431912, 0.01090553684503732870, 0.01181433158212378404, 0.01272312631921023764, 0.01363192105629669297, 0.01454071579338314830, 0.01544951053046960364, 0.01635830526755605724, 0.01726710000464251257, 0.01817589474172896791, 0.01908468947881542324, 0.01999348421590187511, 0.02090227895298833391, 0.02181107369007478577, 0.02362866316424774155, 0.02544625263842069732, 0.02726384211259364962, 0.02908143158676660539 ),
 .UNSPECIFIED. ) ;
#22126=CARTESIAN_POINT ( 'NONE',  ( -35.29220329090401975, 10.25561257217314726, -90.06824336686142374 ) ) ;
#22127=CARTESIAN_POINT ( 'NONE',  ( 18.88468164817598449, 7.626722602998420975, 30.67930430767540173 ) ) ;
#22137=CARTESIAN_POINT ( 'NONE',  ( -86.06489347855098515, 25.27905598459107495, 36.66192029063178381 ) ) ;
#22138=CARTESIAN_POINT ( 'NONE',  ( -24.03640295269301319, 9.507963273819777683, -70.89105126548017211 ) ) ;
#22146=VERTEX_POINT ( 'NONE', #41088 ) ;
#22153=CARTESIAN_POINT ( 'NONE',  ( 181.7858281697336054, 80.75685888198293583, -89.93877274835493552 ) ) ;
#22155=CARTESIAN_POINT ( 'NONE',  ( 55.76298701799387914, 11.10663440745151753, 66.13237673744916378 ) ) ;
#22156=CARTESIAN_POINT ( 'NONE',  ( 141.2794969024892850, 47.29417766120044320, 89.56677758534438283 ) ) ;
#22158=CARTESIAN_POINT ( 'NONE',  ( -30.58934775954355345, 10.47225103507684452, -89.04256022645139979 ) ) ;
#22165=ORIENTED_EDGE ( 'NONE', *, *, #9627, .T. ) ;
#22172=CARTESIAN_POINT ( 'NONE',  ( 82.34195123877069022, 18.00239921638038965, 16.52602691977476113 ) ) ;
#22174=CARTESIAN_POINT ( 'NONE',  ( -77.72491324796695267, 21.96482567905607652, 30.46232876248773636 ) ) ;
#22176=LINE ( 'NONE', #16889, #49928 ) ;
#22178=CARTESIAN_POINT ( 'NONE',  ( -124.9970785861868166, 47.10847819093960709, 3.825783188233985666 ) ) ;
#22179=CARTESIAN_POINT ( 'NONE',  ( 88.30010642107259855, 19.99780058782974734, 17.68303557786764912 ) ) ;
#22186=CARTESIAN_POINT ( 'NONE',  ( -173.1211646369891355, -170.0000000000000000, -95.90105834567735599 ) ) ;
#22187=CARTESIAN_POINT ( 'NONE',  ( -179.5186635612084558, 96.12511541314940189, -38.25937866299342716 ) ) ;
#22190=FACE_OUTER_BOUND ( 'NONE', #52027, .T. ) ;
#22192=CARTESIAN_POINT ( 'NONE',  ( 139.6326990672751265, 46.22017155708128655, -75.15836175618863990 ) ) ;
#22196=FACE_BOUND ( 'NONE', #59707, .T. ) ;
#22199=CARTESIAN_POINT ( 'NONE',  ( -178.2328124332055665, 94.56955476227568624, 59.65814836521386155 ) ) ;
#22200=CARTESIAN_POINT ( 'NONE',  ( -145.3233446620410518, 62.00659513626053609, -9.226959667183525227 ) ) ;
#22201=CARTESIAN_POINT ( 'NONE',  ( -118.6727642982647239, 43.09863379477474155, -44.51070304596819227 ) ) ;
#22206=CARTESIAN_POINT ( 'NONE',  ( -122.3759299995709853, 45.41285412136511468, -75.89897174332118368 ) ) ;
#22207=CARTESIAN_POINT ( 'NONE',  ( 64.94794467308302899, 13.12874966082105033, 17.73165300221493723 ) ) ;
#22208=CARTESIAN_POINT ( 'NONE',  ( 164.6499013411308852, 63.45576988183551492, 12.25078358121806232 ) ) ;
#22209=CARTESIAN_POINT ( 'NONE',  ( 94.02861641584118502, 23.15570573563316259, -17.72789564107222304 ) ) ;
#22212=CARTESIAN_POINT ( 'NONE',  ( -36.00304714721388422, 11.40794940913598943, 16.84363149277759675 ) ) ;
#22215=CARTESIAN_POINT ( 'NONE',  ( 86.15454111412297777, 20.32174891186170029, -77.66611478937542756 ) ) ;
#22216=CARTESIAN_POINT ( 'NONE',  ( 117.4733638683028545, 33.50010943445380462, 92.82365936243014914 ) ) ;
#22217=CARTESIAN_POINT ( 'NONE',  ( -143.3980294393558950, 60.45217072626397226, 60.70765849063186437 ) ) ;
#22218=CARTESIAN_POINT ( 'NONE',  ( 66.08620257826613908, 13.40585338179127461, -9.529234331028934690 ) ) ;
#22220=CARTESIAN_POINT ( 'NONE',  ( -53.38065169970957413, 15.27943072477081365, -62.24569998015859085 ) ) ;
#22221=CARTESIAN_POINT ( 'NONE',  ( -74.09606306030876510, 21.70217968620899285, -90.35397259367368861 ) ) ;
#22225=CARTESIAN_POINT ( 'NONE',  ( 34.45158752686798209, 8.829194381141995507, 69.91381216925195474 ) ) ;
#22227=CARTESIAN_POINT ( 'NONE',  ( 174.6127059037623042, 72.30368563770916523, 59.82278449068079595 ) ) ;
#22228=CARTESIAN_POINT ( 'NONE',  ( -167.4844853368928455, 82.52074065752736942, 60.21220728262811406 ) ) ;
#22233=CARTESIAN_POINT ( 'NONE',  ( 102.7983318509014765, 26.68040613344514611, -44.46865102779961632 ) ) ;
#22234=CARTESIAN_POINT ( 'NONE',  ( -14.19447842053094533, 7.389800932646229725, 68.42821250095973085 ) ) ;
#22235=CARTESIAN_POINT ( 'NONE',  ( 211.5034924207028268, 118.0100795718635283, 13.02898940588344345 ) ) ;
#22237=CARTESIAN_POINT ( 'NONE',  ( -84.05936786797155946, 25.53661143797981126, -91.07400105329199391 ) ) ;
#22238=CARTESIAN_POINT ( 'NONE',  ( 43.97326221476410524, 9.047815246749987494, -10.30912291823035787 ) ) ;
#22240=FACE_BOUND ( 'NONE', #13769, .T. ) ;
#22241=CARTESIAN_POINT ( 'NONE',  ( -58.76005811686685831, 15.70653557534867240, -36.17866631179933279 ) ) ;
#22242=AXIS2_PLACEMENT_3D ( 'NONE', #33060, #53105, #5282 ) ;
#22243=EDGE_CURVE ( 'NONE', #21908, #18538, #40368, .T. ) ;
#22244=ORIENTED_EDGE ( 'NONE', *, *, #60527, .T. ) ;
#22246=CARTESIAN_POINT ( 'NONE',  ( 128.3889472838589256, 39.37765603157608041, 15.32265653812712891 ) ) ;
#22248=CARTESIAN_POINT ( 'NONE',  ( -48.70883077256303295, 14.10659259062419224, 60.65374130472434899 ) ) ;
#22250=CARTESIAN_POINT ( 'NONE',  ( 153.8366942494330942, 54.87992279068317458, 16.62999931596239378 ) ) ;
#22252=EDGE_CURVE ( 'NONE', #51410, #63684, #4371, .T. ) ;
#22253=CARTESIAN_POINT ( 'NONE',  ( -14.13685348404360731, 8.394908291011505597, 87.24003644221730269 ) ) ;
#22255=EDGE_LOOP ( 'NONE', ( #67700, #24767 ) ) ;
#22257=CARTESIAN_POINT ( 'NONE',  ( -59.95707852844800101, 16.05120821151901822, 58.96607362597248425 ) ) ;
#22260=ORIENTED_EDGE ( 'NONE', *, *, #23821, .F. ) ;
#22263=CARTESIAN_POINT ( 'NONE',  ( 105.8203563788590458, 26.88901185006198347, 43.17332345044523123 ) ) ;
#22265=ORIENTED_EDGE ( 'NONE', *, *, #52180, .T. ) ;
#22266=FACE_OUTER_BOUND ( 'NONE', #26736, .T. ) ;
#22267=CARTESIAN_POINT ( 'NONE',  ( 161.7006237583814539, 62.31514460450500792, 30.69927748893351449 ) ) ;
#22268=CARTESIAN_POINT ( 'NONE',  ( 107.0555969502564579, 28.53646637607230474, 3.461266515144562295 ) ) ;
#22269=CARTESIAN_POINT ( 'NONE',  ( 67.55199883153193241, 14.80832170058782005, 4.476120955455310302 ) ) ;
#22271=CARTESIAN_POINT ( 'NONE',  ( 103.8055367708241334, 27.11070767929350822, -12.69745074032687882 ) ) ;
#22273=CARTESIAN_POINT ( 'NONE',  ( 8.537735592981553268, 7.383000420390736451, 39.44863563677944995 ) ) ;
#22275=CARTESIAN_POINT ( 'NONE',  ( 79.97490006123518924, 17.25652566631320539, 94.42763666094869279 ) ) ;
#22280=CARTESIAN_POINT ( 'NONE',  ( 86.62931800182293784, 20.48449268398423229, 56.55663816294300261 ) ) ;
#22281=CARTESIAN_POINT ( 'NONE',  ( -165.7966693951447610, 80.76873405560772312, 93.63453536631139684 ) ) ;
#22282=DIRECTION ( 'NONE',  ( 0.000000000000000000, 0.000000000000000000, 1.000000000000000000 ) ) ;
#22284=CARTESIAN_POINT ( 'NONE',  ( -125.8938041572051389, 46.49392987655491538, 18.77539728269342945 ) ) ;
#22285=CARTESIAN_POINT ( 'NONE',  ( -56.72676045871359207, 16.18052435693491375, -50.03113401488633372 ) ) ;
#22286=CARTESIAN_POINT ( 'NONE',  ( -14.93280618462406828, 8.469244267267910686, -13.66615899223535280 ) ) ;
#22289=CARTESIAN_POINT ( 'NONE',  ( 22.89634831467701304, 6.832298124325687283, -13.76902466704347638 ) ) ;
#22290=EDGE_CURVE ( 'NONE', #55679, #49668, #59324, .T. ) ;
#22292=CARTESIAN_POINT ( 'NONE',  ( -31.43908319763710679, -170.0000000000000000, -35.31719736520183517 ) ) ;
#22295=AXIS2_PLACEMENT_3D ( 'NONE', #16791, #66409, #59693 ) ;
#22298=CARTESIAN_POINT ( 'NONE',  ( -28.03757796776831057, 10.07506086180835503, 84.71353597014326908 ) ) ;
#22299=CARTESIAN_POINT ( 'NONE',  ( -95.88718821240196633, 29.65015105908825888, -46.44459427566074083 ) ) ;
#22301=CARTESIAN_POINT ( 'NONE',  ( -109.7793173546317007, 36.75648380851387742, 11.45816125260146556 ) ) ;
#22302=CARTESIAN_POINT ( 'NONE',  ( 23.09784929786603414, 6.844738137842330872, 39.21172352895144542 ) ) ;
#22303=CARTESIAN_POINT ( 'NONE',  ( 134.7720294983483313, 43.15885542353188953, -9.221000502456890402 ) ) ;
#22304=VERTEX_POINT ( 'NONE', #48755 ) ;
#22306=ORIENTED_EDGE ( 'NONE', *, *, #52096, .F. ) ;
#22310=CARTESIAN_POINT ( 'NONE',  ( 110.2429982417149432, 28.88204397445228722, -62.76698815611734972 ) ) ;
#22312=EDGE_CURVE ( 'NONE', #31650, #44375, #50520, .T. ) ;
#22314=CARTESIAN_POINT ( 'NONE',  ( -38.69577193929645631, 10.89562623693159793, 62.60268121862340251 ) ) ;
#22315=CARTESIAN_POINT ( 'NONE',  ( 201.5876148766343476, 103.8397408698165520, 70.39041556991163873 ) ) ;
#22317=CARTESIAN_POINT ( 'NONE',  ( 182.7686108735401262, 81.77235358504609053, 56.33239625640001691 ) ) ;
#22318=CARTESIAN_POINT ( 'NONE',  ( 133.8566784816069344, -170.0000000000000000, -36.02331093239566684 ) ) ;
#22319=CARTESIAN_POINT ( 'NONE',  ( -2.869721780807576561, 7.625909776230885839, -37.26733688883847151 ) ) ;
#22321=DIRECTION ( 'NONE',  ( 0.000000000000000000, 0.000000000000000000, 1.000000000000000000 ) ) ;
#22322=CARTESIAN_POINT ( 'NONE',  ( 22.81270948571148338, 6.827178363529886163, 66.99894383605555959 ) ) ;
#22324=CARTESIAN_POINT ( 'NONE',  ( 12.68603346975294066, 7.427591953486039067, 17.50285206886463030 ) ) ;
#22329=CARTESIAN_POINT ( 'NONE',  ( -133.3392045760936924, 51.59583146030207246, -43.46796065370383388 ) ) ;
#22335=B_SPLINE_CURVE_WITH_KNOTS ( 'NONE', 3,
 ( #45627, #3746, #55835, #8694, #13955, #50552, #2370, #24863, #19577, #51931, #57219, #35769, #30481, #40341, #25219, #67780, #18892, #39997, #46652, #29790, #13275, #67101, #30149, #51258, #7987, #34733, #62500, #68130, #29439, #56516, #41390, #19935, #3068, #45967, #29104, #41035, #9034, #14310, #19223, #61788, #62844, #7655, #23827, #66751, #13610, #50898, #61454, #62138, #56881, #56171, #8345, #51597, #2715, #35066, #24177, #67431, #3405, #26244, #32212, #14646, #52278, #41728 ),
 .UNSPECIFIED., .F., .F.,
 ( 4, 2, 2, 2, 2, 2, 2, 2, 2, 2, 2, 2, 2, 2, 2, 2, 2, 2, 2, 2, 2, 2, 2, 2, 2, 2, 2, 2, 2, 2, 4 ),
 ( 0.000000000000000000, 0.002279643572853625681, 0.003419465359280425294, 0.004559287145707224473, 0.005699108932134024086, 0.006269019825347425627, 0.006838930718560828036, 0.007978752504987699640, 0.009118574291414570376, 0.01025839607784144285, 0.01139821786426831358, 0.01367786143712207934, 0.01481768322354893794, 0.01595750500997579827, 0.01823714858282953280, 0.02051679215568326387, 0.02165661394211009644, 0.02279643572853692554, 0.02393625751496376158, 0.02507607930139059416, 0.02621590108781742673, 0.02735572287424425930, 0.02849554466067109534, 0.02963536644709792445, 0.03077518823352475702, 0.03191501001995159653, 0.03305483180637842217, 0.03362474269959182110, 0.03419465359280521310, 0.03533447537923198323, 0.03647429716565874641 ),
 .UNSPECIFIED. ) ;
#22338=CARTESIAN_POINT ( 'NONE',  ( -133.2386639184428248, 51.52423002108237426, -94.50477388902842790 ) ) ;
#22340=ORIENTED_EDGE ( 'NONE', *, *, #46795, .T. ) ;
#22347=CARTESIAN_POINT ( 'NONE',  ( 139.2794027252094224, 45.99190465195506761, 69.05840653717436339 ) ) ;
#22352=DIRECTION ( 'NONE',  ( -0.000000000000000000, 1.000000000000000000, -0.000000000000000000 ) ) ;
#22353=CARTESIAN_POINT ( 'NONE',  ( -49.44484229820457699, 14.28460989390479519, -10.86759184043735260 ) ) ;
#22355=CARTESIAN_POINT ( 'NONE',  ( 112.5554747942046276, 29.96654954475020460, -50.56094890218214033 ) ) ;
#22357=CARTESIAN_POINT ( 'NONE',  ( -143.7133518487517279, 60.70463114991424902, -37.54395651202641204 ) ) ;
#22359=CARTESIAN_POINT ( 'NONE',  ( -133.1138189109049392, 51.43538799925376992, 89.75153789939945170 ) ) ;
#22361=CARTESIAN_POINT ( 'NONE',  ( 55.56634333706182360, 12.09342294753929181, 9.466922162906941551 ) ) ;
#22363=CARTESIAN_POINT ( 'NONE',  ( -146.5341851369306028, 61.69744206542950593, 58.16577801895916622 ) ) ;
#22366=CARTESIAN_POINT ( 'NONE',  ( 182.5617509987553433, 80.11195108039726165, -24.23659823810514169 ) ) ;
#22367=CARTESIAN_POINT ( 'NONE',  ( 79.52861599156696570, 17.11914630560288941, -18.94279912049138304 ) ) ;
#22371=CARTESIAN_POINT ( 'NONE',  ( -102.2801239173131194, 32.78103895658057354, 18.67452391595144334 ) ) ;
#22372=CARTESIAN_POINT ( 'NONE',  ( -156.0525065694671696, 69.93592087802322510, -92.33156131024371405 ) ) ;
#22376=CARTESIAN_POINT ( 'NONE',  ( 157.4703587214989398, -170.0000000000000000, 10.06491688178970456 ) ) ;
#22382=CARTESIAN_POINT ( 'NONE',  ( 46.90208227351340042, 10.52324439420451263, -43.36172691416860658 ) ) ;
#22383=CARTESIAN_POINT ( 'NONE',  ( 161.7048274740120632, 61.01946783654761930, -76.67637307521195567 ) ) ;
#22386=CARTESIAN_POINT ( 'NONE',  ( -27.49195330402088899, 9.993776132065301354, 4.489922646395196004 ) ) ;
#22388=CARTESIAN_POINT ( 'NONE',  ( -37.38781680082739456, 10.64362327909143069, 6.278129842404852390 ) ) ;
#22389=CARTESIAN_POINT ( 'NONE',  ( -86.17326876353082810, 25.32448302420862163, 91.54163727806503914 ) ) ;
#22392=B_SPLINE_CURVE_WITH_KNOTS ( 'NONE', 3,
 ( #21209, #9967, #26827, #53190, #4672, #16609, #42655, #27161, #36702, #5019, #68692, #31419, #26138, #48595, #47572, #15923, #21883, #47921, #37039, #10634, #64113, #43334, #37366, #64809, #58824, #53543, #48254, #85, #42983, #64456, #37719, #59167, #27508, #50011, #6050, #19301, #33845, #32795, #12387, #55286, #789, #49652, #1137, #7107 ),
 .UNSPECIFIED., .F., .F.,
 ( 4, 2, 2, 2, 2, 2, 2, 2, 2, 2, 2, 2, 2, 2, 2, 2, 2, 2, 2, 2, 2, 4 ),
 ( 1.387778780781445676E-17, 0.003360573201437459107, 0.004200716501796845567, 0.005040859802156232028, 0.006721146402874958112, 0.007561289703234315950, 0.008401433003593675522, 0.009241576303953032492, 0.01008171960431239120, 0.01176200620503115718, 0.01260214950539055231, 0.01344229280574994398, 0.01428243610610933738, 0.01512257940646873078, 0.01680286600718748982, 0.01764300930754687108, 0.01848315260790624887, 0.02016343920862502526, 0.02184372580934380165, 0.02352401241006257804, 0.02520429901078135443, 0.02688458561150013082 ),
 .UNSPECIFIED. ) ;
#22393=CARTESIAN_POINT ( 'NONE',  ( 126.6464677212869532, 38.39096133771043640, 34.87906214376891967 ) ) ;
#22394=CARTESIAN_POINT ( 'NONE',  ( 31.90170717962884694, 8.563261373066634263, 10.80943639421792746 ) ) ;
#22397=CARTESIAN_POINT ( 'NONE',  ( 86.62931800182292363, 19.42108912189597092, -35.82156419891171595 ) ) ;
#22406=CARTESIAN_POINT ( 'NONE',  ( -12.77550690612892126, 8.273784096785060882, 5.115475724758070442 ) ) ;
#22408=CARTESIAN_POINT ( 'NONE',  ( -1.083610669212419220, 6.545642299653495755, 40.93835893625630717 ) ) ;
#22409=CARTESIAN_POINT ( 'NONE',  ( -108.6634958860518338, 36.14357436892402831, -65.41376181801383893 ) ) ;
#22410=CARTESIAN_POINT ( 'NONE',  ( 93.57136411925270636, 22.98262485654570142, 93.82112078936462751 ) ) ;
#22411=ORIENTED_EDGE ( 'NONE', *, *, #45495, .T. ) ;
#22415=CARTESIAN_POINT ( 'NONE',  ( -130.1964689553233256, 49.39217932424207191, 17.43607221889983094 ) ) ;
#22416=EDGE_CURVE ( 'NONE', #40691, #39142, #32756, .T. ) ;
#22417=CARTESIAN_POINT ( 'NONE',  ( -171.5023337025455135, 86.83681590836891928, -49.54666913844562259 ) ) ;
#22418=CARTESIAN_POINT ( 'NONE',  ( -133.3799602664182373, 52.86209125874979264, -41.88354727973125335 ) ) ;
#22420=CARTESIAN_POINT ( 'NONE',  ( -118.8689810167775960, 42.03922634358562505, -45.05399606991056061 ) ) ;
#22421=CARTESIAN_POINT ( 'NONE',  ( -4.504169684898449155, 6.697401007565304099, -9.344495963075038603 ) ) ;
#22424=CARTESIAN_POINT ( 'NONE',  ( -1.327237339235002311, 7.561837009978236601, -66.00973041474892966 ) ) ;
#22428=CARTESIAN_POINT ( 'NONE',  ( -15.15117926080556465, 8.490099586177995761, -95.00000000000133582 ) ) ;
#22429=CARTESIAN_POINT ( 'NONE',  ( 197.6316695787931224, 97.13022718399025734, -41.29383634472684861 ) ) ;
#22430=CARTESIAN_POINT ( 'NONE',  ( -151.2428028786328014, 66.99705074331122034, 30.91134539836198059 ) ) ;
#22433=LINE ( 'NONE', #66757, #12986 ) ;
#22435=CARTESIAN_POINT ( 'NONE',  ( 178.1888264190354221, 77.13727704498026583, 70.58518440423399909 ) ) ;
#22438=CARTESIAN_POINT ( 'NONE',  ( -71.17819443284076897, 19.60909329639481413, -15.27992725511833427 ) ) ;
#22440=CARTESIAN_POINT ( 'NONE',  ( 150.2060369882285045, 53.45752899907539302, 11.95053698778202467 ) ) ;
#22442=CARTESIAN_POINT ( 'NONE',  ( 162.0835148203877054, 61.32844276806159201, 30.97683732797539946 ) ) ;
#22444=VECTOR ( 'NONE', #9548, 1000.000000000000000 ) ;
#22447=EDGE_LOOP ( 'NONE', ( #32856, #42222, #41834, #29931 ) ) ;
#22448=CARTESIAN_POINT ( 'NONE',  ( -142.6105148419746911, 59.82538670924427038, -93.01220556088156854 ) ) ;
#22449=EDGE_CURVE ( 'NONE', #34501, #48145, #4248, .T. ) ;
#22452=CARTESIAN_POINT ( 'NONE',  ( 150.4747435624740604, 52.41018979694876379, -94.57218390293165555 ) ) ;
#22453=CARTESIAN_POINT ( 'NONE',  ( -38.87848244732138170, 10.93141945332449616, -70.64516419336318620 ) ) ;
#22454=CARTESIAN_POINT ( 'NONE',  ( 23.24047374271773236, 7.861801299833791390, 65.33839104122442620 ) ) ;
#22455=VERTEX_POINT ( 'NONE', #14613 ) ;
#22461=CARTESIAN_POINT ( 'NONE',  ( -38.92726670956012214, 10.94099576009806718, -43.30594718313987102 ) ) ;
#22462=DIRECTION ( 'NONE',  ( -0.8118923937861950435, -0.5838071093367415143, 0.000000000000000000 ) ) ;
#22464=CARTESIAN_POINT ( 'NONE',  ( -129.3963145237380843, 48.84337839101546308, 71.60049605309630749 ) ) ;
#22465=CARTESIAN_POINT ( 'NONE',  ( -50.89515345785970624, 14.64311186056398384, 85.25617531740348909 ) ) ;
#22467=CARTESIAN_POINT ( 'NONE',  ( 83.38067517854670996, 18.33799117207140128, 57.29236275353452612 ) ) ;
#22470=FACE_OUTER_BOUND ( 'NONE', #6508, .T. ) ;
#22472=ORIENTED_EDGE ( 'NONE', *, *, #36619, .F. ) ;
#22473=CARTESIAN_POINT ( 'NONE',  ( 186.6054783416232112, 84.37128553200977876, 31.70807712453434846 ) ) ;
#22475=EDGE_CURVE ( 'NONE', #53864, #64948, #45350, .T. ) ;
#22478=CARTESIAN_POINT ( 'NONE',  ( -55.05276343752909440, 14.68156374112637508, 18.47277718246750311 ) ) ;
#22480=CARTESIAN_POINT ( 'NONE',  ( 152.8558173410470147, 54.14978343559395313, -37.69186017836011615 ) ) ;
#22481=CARTESIAN_POINT ( 'NONE',  ( 164.1352994389932576, 64.33767534192696758, -73.91823402297541179 ) ) ;
#22488=VERTEX_POINT ( 'NONE', #42380 ) ;
#22489=CARTESIAN_POINT ( 'NONE',  ( -85.90441187606242579, 25.21188850826091254, 39.94801297243609639 ) ) ;
#22490=CARTESIAN_POINT ( 'NONE',  ( -26.50207385662996273, 9.849226639603653410, -75.32933197546118720 ) ) ;
#22491=CARTESIAN_POINT ( 'NONE',  ( 46.12582897016704209, 10.39833982076225283, 40.74553764170175185 ) ) ;
#22492=CARTESIAN_POINT ( 'NONE',  ( -24.19091603582231897, 8.513464105188679909, 66.50394091260255891 ) ) ;
#22493=PLANE ( 'NONE',  #63386 ) ;
#22495=B_SPLINE_CURVE_WITH_KNOTS ( 'NONE', 3,
 ( #42543, #21426, #62969, #15128, #25698, #14774, #68259, #68919, #36929, #4566, #36589, #52069, #25355, #20393, #36240, #58035, #37253, #57697, #10522, #69274, #16149, #21099, #31994, #42868, #42205, #46787, #64338, #4910, #9507, #47126, #63666, #52415, #20063, #37602, #31313, #26716, #26029, #63997, #48146, #4232, #26374, #47814, #58705, #5256, #59056 ),
 .UNSPECIFIED., .F., .F.,
 ( 4, 2, 2, 2, 2, 2, 2, 2, 2, 2, 2, 1, 2, 2, 2, 2, 2, 2, 2, 2, 2, 2, 4 ),
 ( 0.000000000000000000, 0.001512548138464654733, 0.002268822207696980040, 0.003025096276929305564, 0.004537644415393922784, 0.005293918484626250476, 0.006050192553858578168, 0.007562740692323231817, 0.009075288830787885466, 0.01058783696925254258, 0.01134411103848488936, 0.01210038510771723613, 0.01285665917694958464, 0.01361293324618193142, 0.01512548138464657639, 0.01588175545387889021, 0.01663802952311120575, 0.01815057766157582991, 0.01966312580004045407, 0.02041939986927276962, 0.02117567393850508517, 0.02268822207696974402, 0.02420077021543440635 ),
 .UNSPECIFIED. ) ;
#22496=VERTEX_POINT ( 'NONE', #5438 ) ;
#22500=CARTESIAN_POINT ( 'NONE',  ( 33.75794032130628608, 8.754084575552406378, -11.31189195812216397 ) ) ;
#22502=CARTESIAN_POINT ( 'NONE',  ( 55.76066037845576062, 11.10616952318089368, 62.19232937580554221 ) ) ;
#22513=CARTESIAN_POINT ( 'NONE',  ( 138.6020257460770040, 44.36414356192210562, -64.53975052502872245 ) ) ;
#22517=CARTESIAN_POINT ( 'NONE',  ( 79.19132716134490124, 17.01584750883626995, 9.372603967536683456 ) ) ;
#22519=CARTESIAN_POINT ( 'NONE',  ( -73.79615177260656367, 20.52570924097573624, 43.64279597580159731 ) ) ;
#22521=CARTESIAN_POINT ( 'NONE',  ( -118.4753258120605466, 42.97785158603420541, -95.00000000000133582 ) ) ;
#22523=CARTESIAN_POINT ( 'NONE',  ( -146.5341851369306028, 61.69744206542950593, -76.05697493335925685 ) ) ;
#22525=CARTESIAN_POINT ( 'NONE',  ( 94.11746922806585758, 22.11341285603783291, 10.85955068103982057 ) ) ;
#22528=EDGE_LOOP ( 'NONE', ( #415, #27881 ) ) ;
#22529=DIRECTION ( 'NONE',  ( -0.000000000000000000, 1.000000000000000000, -0.000000000000000000 ) ) ;
#22532=CARTESIAN_POINT ( 'NONE',  ( 32.38493285958205092, 8.611594965040675120, 34.75454220440185082 ) ) ;
#22533=CARTESIAN_POINT ( 'NONE',  ( -177.5100621450480105, 93.70693725195826573, -48.31160080727584472 ) ) ;
#22534=EDGE_CURVE ( 'NONE', #44530, #52688, #49565, .T. ) ;
#22535=CARTESIAN_POINT ( 'NONE',  ( -128.9925397612932727, 48.56800623462827815, -22.40303128747859063 ) ) ;
#22540=CARTESIAN_POINT ( 'NONE',  ( -148.0058283997321098, 64.22864592525515093, -76.50871507917976544 ) ) ;
#22542=EDGE_CURVE ( 'NONE', #50285, #45819, #21061, .T. ) ;
#22543=FACE_BOUND ( 'NONE', #52066, .T. ) ;
#22544=CARTESIAN_POINT ( 'NONE',  ( -4.955782747743210592, 6.720825863997140992, -76.70478924277563237 ) ) ;
#22545=CARTESIAN_POINT ( 'NONE',  ( -31.43908319763709969, 10.61114334766716105, 30.21645440618916112 ) ) ;
#22548=CARTESIAN_POINT ( 'NONE',  ( -4.071369321747702053, 7.682719369516286534, 44.12691017724150555 ) ) ;
#22551=CARTESIAN_POINT ( 'NONE',  ( -7.825402957745083654, 7.899365992529244984, -8.573520141480125645 ) ) ;
#22552=CARTESIAN_POINT ( 'NONE',  ( -11.56945424397728139, 8.173256823723107800, 31.11234499143955645 ) ) ;
#22553=CARTESIAN_POINT ( 'NONE',  ( 116.6457744947906860, 31.95847117670279403, 6.352866292760225519 ) ) ;
#22554=CARTESIAN_POINT ( 'NONE',  ( 44.78501478287838466, 10.18870581198737391, -91.58250997119135661 ) ) ;
#22556=CARTESIAN_POINT ( 'NONE',  ( -33.12994257348896099, 10.89587983539684402, 3.560888656335561731 ) ) ;
#22557=VERTEX_POINT ( 'NONE', #28998 ) ;
#22560=DIRECTION ( 'NONE',  ( -0.000000000000000000, 1.000000000000000000, -0.000000000000000000 ) ) ;
#22561=CARTESIAN_POINT ( 'NONE',  ( 116.5839788410853544, 33.05236809212184568, 86.78057374190305495 ) ) ;
#22562=CARTESIAN_POINT ( 'NONE',  ( 181.0840389613909736, -170.0000000000000000, -63.06960825634327961 ) ) ;
#22563=CARTESIAN_POINT ( 'NONE',  ( 68.63487067129261732, 14.04635751989138903, -11.38481879685736153 ) ) ;
#22565=CARTESIAN_POINT ( 'NONE',  ( -26.50207385662994852, 9.849226639603649858, -48.48478138499748979 ) ) ;
#22566=CARTESIAN_POINT ( 'NONE',  ( -190.6985136298601731, 109.1272424661242582, -95.00000000000133582 ) ) ;
#22569=CARTESIAN_POINT ( 'NONE',  ( -125.8938041572051389, 47.69968343338778283, 3.775397282693376155 ) ) ;
#22573=CARTESIAN_POINT ( 'NONE',  ( 174.2469308602414912, 71.96142024047682639, 60.55816399741460287 ) ) ;
#22581=CARTESIAN_POINT ( 'NONE',  ( 102.7414208686707866, 26.65627265923299660, -42.93303738452352292 ) ) ;
#22582=CARTESIAN_POINT ( 'NONE',  ( 188.4918087359956758, 87.93403732562657638, -18.09163806308507461 ) ) ;
#22583=CARTESIAN_POINT ( 'NONE',  ( -85.45399718454963534, 25.02415453493131281, -12.57056528233159298 ) ) ;
#22585=CARTESIAN_POINT ( 'NONE',  ( 45.36109889487609337, 9.259412558041139718, -11.69495450463035446 ) ) ;
#22586=CARTESIAN_POINT ( 'NONE',  ( 206.3125232506203020, 108.5822159704961933, -9.646018633704194656 ) ) ;
#22587=FACE_BOUND ( 'NONE', #66886, .T. ) ;
#22588=CARTESIAN_POINT ( 'NONE',  ( -62.30463872474476261, 16.74658165105248386, -44.69399102852965200 ) ) ;
#22591=CARTESIAN_POINT ( 'NONE',  ( 92.95016907945944240, 22.74936990452174967, -47.36605269353328396 ) ) ;
#22596=EDGE_CURVE ( 'NONE', #63625, #65931, #56065, .T. ) ;
#22597=ORIENTED_EDGE ( 'NONE', *, *, #36771, .T. ) ;
#22602=LINE ( 'NONE', #28219, #22924 ) ;
#22604=CARTESIAN_POINT ( 'NONE',  ( 108.3906473026529511, 28.03385344351497110, 44.39384328560462478 ) ) ;
#22605=ORIENTED_EDGE ( 'NONE', *, *, #25898, .F. ) ;
#22606=VECTOR ( 'NONE', #31175, 1000.000000000000000 ) ;
#22609=CARTESIAN_POINT ( 'NONE',  ( 164.8444104055694481, 64.93678790243656351, 35.51303964267133750 ) ) ;
#22610=CARTESIAN_POINT ( 'NONE',  ( -156.9900125991011066, 72.16580261738675972, -69.74404362362140830 ) ) ;
#22618=CARTESIAN_POINT ( 'NONE',  ( 109.3047140914111850, 29.55674059952506738, -9.121791405023586208 ) ) ;
#22619=FACE_OUTER_BOUND ( 'NONE', #30603, .T. ) ;
#22620=CARTESIAN_POINT ( 'NONE',  ( -131.6253556217205016, 51.61436399519948282, -20.43251446978527852 ) ) ;
#22621=CARTESIAN_POINT ( 'NONE',  ( -153.4120976477049965, 68.90960692040326308, -89.59491812855455350 ) ) ;
#22628=VECTOR ( 'NONE', #41595, 1000.000000000000000 ) ;
#22630=CARTESIAN_POINT ( 'NONE',  ( -11.14445507968271265, 7.129894202659272651, -22.80362678214407168 ) ) ;
#22631=CARTESIAN_POINT ( 'NONE',  ( -165.8387952943256778, 80.81203372455925660, 93.81362447417453154 ) ) ;
#22634=CARTESIAN_POINT ( 'NONE',  ( -55.53456145826331181, 15.85318253404851419, -50.21632399845988459 ) ) ;
#22636=FACE_OUTER_BOUND ( 'NONE', #67647, .T. ) ;
#22640=EDGE_LOOP ( 'NONE', ( #23964, #29233, #64608, #64688 ) ) ;
#22642=EDGE_CURVE ( 'NONE', #4373, #10658, #1754, .T. ) ;
#22650=CARTESIAN_POINT ( 'NONE',  ( 141.3400002717722828, 47.33399859146518907, -16.11108315197586194 ) ) ;
#22652=ORIENTED_EDGE ( 'NONE', *, *, #21924, .T. ) ;
#22653=ORIENTED_EDGE ( 'NONE', *, *, #69545, .T. ) ;
#22655=CARTESIAN_POINT ( 'NONE',  ( -156.9919426121902575, 72.16759471857101005, -14.90541269196195451 ) ) ;
#22657=CARTESIAN_POINT ( 'NONE',  ( 55.90910788310615231, 11.13585330978403576, -13.92866980567223756 ) ) ;
#22659=AXIS2_PLACEMENT_3D ( 'NONE', #61621, #51068, #13096 ) ;
#22660=CARTESIAN_POINT ( 'NONE',  ( -102.2801239173131194, 32.78103895658057354, 45.51907450641513009 ) ) ;
#22663=CARTESIAN_POINT ( 'NONE',  ( 181.0840389613909736, 80.03940679743416808, 56.15314469597509373 ) ) ;
#22664=CARTESIAN_POINT ( 'NONE',  ( -156.7487895666416762, 70.57327586518566420, 63.09231583114617337 ) ) ;
#22667=CARTESIAN_POINT ( 'NONE',  ( -0.7076388175553602888, 7.538734751903869657, -45.33243332686139127 ) ) ;
#22668=CARTESIAN_POINT ( 'NONE',  ( 105.4375968828853729, 26.72149058755205786, 16.03008684478035661 ) ) ;
#22669=CARTESIAN_POINT ( 'NONE',  ( -167.9399687280718751, 81.54040755612503233, -90.45838053675130652 ) ) ;
#22671=FACE_BOUND ( 'NONE', #30482, .T. ) ;
#22673=CARTESIAN_POINT ( 'NONE',  ( 10.83046137699561484, 6.392429922561257527, -64.21464171610804783 ) ) ;
#22678=CARTESIAN_POINT ( 'NONE',  ( -132.4951995226844872, 50.99687809989499243, -45.98269415215550993 ) ) ;
#22679=CARTESIAN_POINT ( 'NONE',  ( 46.65037935242578016, 9.463293687292242851, -68.02239084012497017 ) ) ;
#22683=VERTEX_POINT ( 'NONE', #30369 ) ;
#22685=CARTESIAN_POINT ( 'NONE',  ( 180.9522142081943059, 78.47222086051785084, 82.99343427934738315 ) ) ;
#22687=ADVANCED_FACE ( 'NONE', ( #51821 ), #3628, .T. ) ;
#22688=EDGE_LOOP ( 'NONE', ( #46218, #57249, #4689, #56444 ) ) ;
#22689=CARTESIAN_POINT ( 'NONE',  ( 180.2473887773227545, 77.76029175826236894, -36.22505766587961773 ) ) ;
#22690=CARTESIAN_POINT ( 'NONE',  ( -78.66644367742111399, 22.32174330031318021, -23.27090004125422595 ) ) ;
#22694=CARTESIAN_POINT ( 'NONE',  ( -77.72491324796695267, 21.96482567905607297, -50.07132300890329901 ) ) ;
#22696=CARTESIAN_POINT ( 'NONE',  ( 90.31682503704257670, 20.71196693118262289, -36.77252112897771497 ) ) ;
#22697=CARTESIAN_POINT ( 'NONE',  ( -50.52615126106341847, 14.55080735582893148, -21.87146891271175875 ) ) ;
#22699=ORIENTED_EDGE ( 'NONE', *, *, #54445, .F. ) ;
#22700=EDGE_CURVE ( 'NONE', #25068, #52964, #21526, .T. ) ;
#22703=CARTESIAN_POINT ( 'NONE',  ( -142.5087559769085033, 59.74468185400780129, -39.56408865608762682 ) ) ;
#22705=CARTESIAN_POINT ( 'NONE',  ( -171.5023337025454850, 86.83681590836890507, -76.39121972890930579 ) ) ;
#22706=CARTESIAN_POINT ( 'NONE',  ( -132.6405077585060042, 51.09958558523505445, 88.51731180315442771 ) ) ;
#22707=ORIENTED_EDGE ( 'NONE', *, *, #15906, .T. ) ;
#22708=DIRECTION ( 'NONE',  ( 0.000000000000000000, 0.000000000000000000, 1.000000000000000000 ) ) ;
#22710=EDGE_CURVE ( 'NONE', #24054, #10586, #29403, .T. ) ;
#22714=CARTESIAN_POINT ( 'NONE',  ( -146.1260528621668016, 61.36307454672304829, 58.35490513784959887 ) ) ;
#22719=CARTESIAN_POINT ( 'NONE',  ( 82.94943325692328528, 18.19803534719806137, -23.01670398887183921 ) ) ;
#22721=DIRECTION ( 'NONE',  ( -0.000000000000000000, 1.000000000000000000, -0.000000000000000000 ) ) ;
#22722=CARTESIAN_POINT ( 'NONE',  ( -25.50819575705322606, 8.692660622847146357, -91.89581271472285096 ) ) ;
#22723=CARTESIAN_POINT ( 'NONE',  ( -55.05276343752909440, 15.72344139423348430, 45.31732777293115788 ) ) ;
#22727=CARTESIAN_POINT ( 'NONE',  ( 46.50207827473962396, 9.439498081273459462, 34.98490145612715452 ) ) ;
#22728=CARTESIAN_POINT ( 'NONE',  ( -173.1211646369891355, 88.63826465341152527, 72.66624519710475738 ) ) ;
#22729=LINE ( 'NONE', #43127, #48048 ) ;
#22734=CARTESIAN_POINT ( 'NONE',  ( 210.0055645826033981, 115.7254585628714096, -49.14771549242088611 ) ) ;
#22735=CARTESIAN_POINT ( 'NONE',  ( -71.15374617000811952, 20.66492714610676273, -69.44983854139488244 ) ) ;
#22736=CARTESIAN_POINT ( 'NONE',  ( -109.7290872258107299, 36.72869630780160577, 63.84435436436351807 ) ) ;
#22737=CARTESIAN_POINT ( 'NONE',  ( -29.49620345460273185, 9.280093073089044964, -35.55655680868790114 ) ) ;
#22738=CARTESIAN_POINT ( 'NONE',  ( 162.7921669283191761, 61.91024532638674316, -75.75915507580972985 ) ) ;
#22739=ORIENTED_EDGE ( 'NONE', *, *, #42584, .T. ) ;
#22743=CARTESIAN_POINT ( 'NONE',  ( -86.07006026987795622, 25.28121476708071924, 92.84969470335587971 ) ) ;
#22744=CARTESIAN_POINT ( 'NONE',  ( -82.93267503967652488, 23.99263498936122119, 70.93582899126512586 ) ) ;
#22745=CARTESIAN_POINT ( 'NONE',  ( 130.3281282802763315, 40.49854652972196334, 30.37535463369031774 ) ) ;
#22748=CARTESIAN_POINT ( 'NONE',  ( 117.3187069485358620, 33.42192264892479869, -94.58789033624162812 ) ) ;
#22750=CARTESIAN_POINT ( 'NONE',  ( 212.1666685067961566, 117.1838024370489109, 89.67890646288726941 ) ) ;
#22754=CARTESIAN_POINT ( 'NONE',  ( -13.92109095214679648, 8.375243258322930373, 6.394640106076189490 ) ) ;
#22757=B_SPLINE_CURVE_WITH_KNOTS ( 'NONE', 3,
 ( #61434, #40319, #7633, #45596, #19911, #56150, #62113, #41366, #8321, #24840, #29085, #35393, #67756, #56853, #67081, #23804, #18871, #51910, #50532, #13590, #29765, #45942, #19200, #3717, #8671, #45245, #30125, #55814, #41015, #51576, #62470, #62819, #7967, #14286, #29422, #35746, #50872, #9015, #25196, #14623, #2352, #2690, #10037, #31165, #21278 ),
 .UNSPECIFIED., .F., .F.,
 ( 4, 2, 2, 1, 2, 2, 2, 2, 2, 2, 2, 2, 2, 2, 2, 2, 2, 2, 2, 2, 2, 2, 4 ),
 ( 0.02348395315094739880, 0.02495010856601295388, 0.02568318627354573142, 0.02641626398107850549, 0.02714934168861128302, 0.02788241939614406056, 0.02934857481120962605, 0.03008165251874241747, 0.03081473022627520542, 0.03228088564134076743, 0.03301396334887356232, 0.03374704105640635721, 0.03521319647147194004, 0.03667935188653752288, 0.03741242959407032470, 0.03814550730160312653, 0.03961166271666873018, 0.04107781813173433383, 0.04254397354679993748, 0.04327705125433273931, 0.04401012896186554113, 0.04547628437693114478, 0.04694243979199674843 ),
 .UNSPECIFIED. ) ;
#22761=CARTESIAN_POINT ( 'NONE',  ( -189.4223925288096666, 107.3427006758676470, -13.54568499105593382 ) ) ;
#22762=CARTESIAN_POINT ( 'NONE',  ( -133.3926783185151521, 51.63401075114365568, 11.57669413790383572 ) ) ;
#22763=CARTESIAN_POINT ( 'NONE',  ( -171.4943428135322847, 86.82484920477509149, -34.84193120942898503 ) ) ;
#22764=CARTESIAN_POINT ( 'NONE',  ( -128.7724923851857000, 49.63576597317771189, -35.48433415201512275 ) ) ;
#22767=AXIS2_PLACEMENT_3D ( 'NONE', #11198, #45660, #33381 ) ;
#22770=CARTESIAN_POINT ( 'NONE',  ( -0.5783162822156577842, 7.534184941292929594, -67.81582771104294238 ) ) ;
#22772=VECTOR ( 'NONE', #1471, 1000.000000000000000 ) ;
#22773=FACE_OUTER_BOUND ( 'NONE', #26487, .T. ) ;
#22775=CARTESIAN_POINT ( 'NONE',  ( 157.8370895073805684, 59.21456076921543143, -89.81328548006499091 ) ) ;
#22776=CARTESIAN_POINT ( 'NONE',  ( 200.8298320869470217, 101.1869877914233342, -50.26595701390404969 ) ) ;
#22777=CARTESIAN_POINT ( 'NONE',  ( -94.83794676023109105, 30.26879337035745365, 39.08187224689461203 ) ) ;
#22779=CARTESIAN_POINT ( 'NONE',  ( 21.25987915030396636, 6.737472588634930482, -48.15424469599262380 ) ) ;
#22783=CARTESIAN_POINT ( 'NONE',  ( 177.7886308167536242, 76.74396398590876345, 70.40547167736322365 ) ) ;
#22784=EDGE_CURVE ( 'NONE', #62313, #3776, #61297, .T. ) ;
#22788=CARTESIAN_POINT ( 'NONE',  ( 181.0840389613909736, 80.03940679743416808, 29.30859410551139277 ) ) ;
#22791=CARTESIAN_POINT ( 'NONE',  ( -14.93280618462407006, 8.469244267267917792, -67.35526017316270497 ) ) ;
#22793=CARTESIAN_POINT ( 'NONE',  ( 160.9241720448059709, 60.38677655937337363, 43.58305608898694317 ) ) ;
#22801=CARTESIAN_POINT ( 'NONE',  ( 111.1829448509513014, 30.43012797723691065, 44.56673546540911701 ) ) ;
#22803=CARTESIAN_POINT ( 'NONE',  ( 20.36233635256088093, 7.697399815318435756, 58.39548332934419506 ) ) ;
#22807=CARTESIAN_POINT ( 'NONE',  ( 208.9381799476942660, 112.3426042533246658, -91.31812090025519524 ) ) ;
#22812=CARTESIAN_POINT ( 'NONE',  ( -33.13098007862451055, 9.875138601866705557, -35.50648902819412456 ) ) ;
#22813=CARTESIAN_POINT ( 'NONE',  ( -102.3225989298749141, 32.80186750033362841, 84.19102271607455634 ) ) ;
#22817=CARTESIAN_POINT ( 'NONE',  ( -61.97459043553174496, 17.69799435201358051, 94.41227228605326616 ) ) ;
#22819=CARTESIAN_POINT ( 'NONE',  ( 81.76092782665033099, 17.81692437267514251, 69.76706349355957570 ) ) ;
#22820=ORIENTED_EDGE ( 'NONE', *, *, #67276, .F. ) ;
#22821=CARTESIAN_POINT ( 'NONE',  ( 34.84173759613681653, 7.859847277726516701, 43.38827435105228147 ) ) ;
#22823=DIRECTION ( 'NONE',  ( -0.000000000000000000, 1.000000000000000000, -0.000000000000000000 ) ) ;
#22827=CARTESIAN_POINT ( 'NONE',  ( -71.96390573417174608, 19.88067451234327265, 14.47695953071579922 ) ) ;
#22828=CARTESIAN_POINT ( 'NONE',  ( -125.8938041572051389, 47.69968343338778993, 57.46449846362076386 ) ) ;
#22829=CARTESIAN_POINT ( 'NONE',  ( -51.13073217147957905, 13.66490163179656925, 17.37025274476010495 ) ) ;
#22831=CARTESIAN_POINT ( 'NONE',  ( 151.3309484205704791, 53.03078371058069962, -39.30893049917887794 ) ) ;
#22835=ORIENTED_EDGE ( 'NONE', *, *, #35041, .F. ) ;
#22838=ORIENTED_EDGE ( 'NONE', *, *, #791, .T. ) ;
#22840=CARTESIAN_POINT ( 'NONE',  ( 154.0515132159917471, 56.29926936869308918, -77.16036314277725694 ) ) ;
#22842=CARTESIAN_POINT ( 'NONE',  ( -25.50312845906834269, 8.692070753302665764, 59.97022089822687008 ) ) ;
#22844=ORIENTED_EDGE ( 'NONE', *, *, #21740, .T. ) ;
#22848=CARTESIAN_POINT ( 'NONE',  ( 183.3913492984167704, 80.96922346472078402, 2.824542694585014502 ) ) ;
#22849=CARTESIAN_POINT ( 'NONE',  ( -0.3252226420479318314, 7.525368746738508641, 63.97339285451934643 ) ) ;
#22850=CARTESIAN_POINT ( 'NONE',  ( -25.13974312463025029, 9.657576844361820179, -92.43015382880602715 ) ) ;
#22854=CARTESIAN_POINT ( 'NONE',  ( -118.7011677090247304, 41.93687969120207981, -71.39957740465628433 ) ) ;
#22859=AXIS2_PLACEMENT_3D ( 'NONE', #55169, #65038, #23183 ) ;
#22860=CARTESIAN_POINT ( 'NONE',  ( -172.7116702014379257, 86.67317892691252723, -7.867406574286299303 ) ) ;
#22861=CARTESIAN_POINT ( 'NONE',  ( -130.2340355668706309, 50.64168009053632602, -89.97067613245286566 ) ) ;
#22866=ADVANCED_FACE ( 'NONE', ( #18003 ), #12375, .F. ) ;
#22867=CARTESIAN_POINT ( 'NONE',  ( 79.52861599156696570, 17.11914630560288941, 7.901751469972297492 ) ) ;
#22874=EDGE_CURVE ( 'NONE', #29587, #37010, #56322, .T. ) ;
#22877=CARTESIAN_POINT ( 'NONE',  ( -143.8794621588508846, 59.54894433207191895, -74.12090710118032177 ) ) ;
#22883=CARTESIAN_POINT ( 'NONE',  ( 58.17717674717528809, 12.63051673829130550, 85.26196710955888136 ) ) ;
#22884=CARTESIAN_POINT ( 'NONE',  ( 34.45972925205164472, 8.830088223935229408, 31.75137734477696938 ) ) ;
#22885=CARTESIAN_POINT ( 'NONE',  ( -180.2243452982808378, 96.99029284948632323, -39.78723934564764875 ) ) ;
#22886=CARTESIAN_POINT ( 'NONE',  ( -128.7650348665116837, 48.41336321950709731, -8.636724289455223413 ) ) ;
#22887=CARTESIAN_POINT ( 'NONE',  ( 32.12337157895397866, 8.585320123189577046, -95.00000000000133582 ) ) ;
#22888=CARTESIAN_POINT ( 'NONE',  ( 126.3737790127712515, 37.08609730334947585, -69.79690750847547065 ) ) ;
#22890=DIRECTION ( 'NONE',  ( -0.000000000000000000, 1.000000000000000000, -0.000000000000000000 ) ) ;
#22891=CARTESIAN_POINT ( 'NONE',  ( -144.9417090887490360, 61.69631066549397502, -75.11214843033646105 ) ) ;
#22893=CARTESIAN_POINT ( 'NONE',  ( -154.0833774771448930, 69.51012195447349029, -36.35145225699776006 ) ) ;
#22894=CARTESIAN_POINT ( 'NONE',  ( -0.5751131641471395328, 6.527254166626919485, -67.82773600439074357 ) ) ;
#22895=CARTESIAN_POINT ( 'NONE',  ( -173.5422248620771484, 89.11126078969411424, 72.66624519710472896 ) ) ;
#22896=CARTESIAN_POINT ( 'NONE',  ( -142.9843132609582312, 60.12226089556225617, -11.75793129031485051 ) ) ;
#22897=CYLINDRICAL_SURFACE ( 'NONE', #53627, 7.500000000000020428 ) ;
#22898=CARTESIAN_POINT ( 'NONE',  ( -55.05276343752910151, -170.0000000000000000, -15.87177340799618364 ) ) ;
#22904=CARTESIAN_POINT ( 'NONE',  ( 117.3110050642447817, 32.29133253383015756, 7.707881950449412933 ) ) ;
#22905=CARTESIAN_POINT ( 'NONE',  ( -48.72990440218273989, 14.11167693102101950, -92.36568283827145365 ) ) ;
#22908=CARTESIAN_POINT ( 'NONE',  ( -33.36965723649377935, 10.93726715887723877, 3.620524580207087340 ) ) ;
#22911=CARTESIAN_POINT ( 'NONE',  ( 79.33384730094455506, 18.11203072455035823, -71.92377449950194546 ) ) ;
#22912=AXIS2_PLACEMENT_3D ( 'NONE', #45933, #19189, #17821 ) ;
#22915=CARTESIAN_POINT ( 'NONE',  ( -24.95010104166214759, 9.631487977190600347, -39.04838185491376379 ) ) ;
#22918=CARTESIAN_POINT ( 'NONE',  ( -173.1211646369891071, 87.12891641440857882, 57.66624519710472185 ) ) ;
#22923=B_SPLINE_CURVE_WITH_KNOTS ( 'NONE', 3,
 ( #63963, #53049, #37575, #20711, #26683, #48114, #26341, #15777, #21392, #59023, #47777, #58332, #42838, #52706, #21066, #10150, #10839, #42512, #32311, #53738, #37223, #58674, #5560, #58003, #9822, #31280, #20584, #4081, #3386, #31168, #68108, #46634, #24843, #25546, #42046, #40663, #62822, #30461, #30128, #46282, #67759, #52259, #46981 ),
 .UNSPECIFIED., .F., .F.,
 ( 4, 2, 2, 2, 2, 2, 2, 2, 2, 2, 2, 2, 1, 2, 2, 2, 2, 2, 2, 2, 2, 4 ),
 ( 0.02371951416048009159, 0.02520633211177537858, 0.02594974108742300126, 0.02669315006307062393, 0.02817996801436589011, 0.02966678596566115281, 0.03041019494130878589, 0.03115360391695641898, 0.03264042186825171638, 0.03412723981954701724, 0.03561405777084231117, 0.03635746674648995813, 0.03710087572213760509, 0.03784428469778525900, 0.03858769367343290596, 0.04007451162472822070, 0.04156132957602352851, 0.04304814752731883631, 0.04379155650296651103, 0.04453496547861417187, 0.04602178342990950743, 0.04750860138120484299 ),
 .UNSPECIFIED. ) ;
#22924=VECTOR ( 'NONE', #38082, 1000.000000000000000 ) ;
#22926=CARTESIAN_POINT ( 'NONE',  ( 175.8963338753314360, 73.51705463274396379, 69.07525203059798002 ) ) ;
#22930=CARTESIAN_POINT ( 'NONE',  ( -171.0950923142953854, 86.38958441093222973, -22.60122060940205202 ) ) ;
#22932=CARTESIAN_POINT ( 'NONE',  ( 8.000000000000007105, 249.8719672152120381, 94.99999999999866418 ) ) ;
#22934=CARTESIAN_POINT ( 'NONE',  ( 89.65730223173018487, 21.54473673261222899, 3.501741773472330621 ) ) ;
#22937=CARTESIAN_POINT ( 'NONE',  ( -82.71271320792514814, 24.98855420139966199, -89.97510010486354304 ) ) ;
#22939=CARTESIAN_POINT ( 'NONE',  ( 210.6741002223296846, 114.9147155784838503, -12.44257081975957746 ) ) ;
#22940=FACE_BOUND ( 'NONE', #46141, .T. ) ;
#22941=CARTESIAN_POINT ( 'NONE',  ( -59.56523643198717366, 15.93788386494078857, -36.72066679286387370 ) ) ;
#22946=CARTESIAN_POINT ( 'NONE',  ( -55.05276343752909440, 14.68156374112637863, -62.06087458892354647 ) ) ;
#22947=EDGE_CURVE ( 'NONE', #47361, #10179, #24675, .T. ) ;
#22948=CARTESIAN_POINT ( 'NONE',  ( -7.825402957745087207, -170.0000000000000000, -89.10717191287116634 ) ) ;
#22950=CARTESIAN_POINT ( 'NONE',  ( 204.6977192012829789, 108.0580384837234931, 71.05227132923315025 ) ) ;
#22953=CARTESIAN_POINT ( 'NONE',  ( 63.01563776193091826, 12.67277567978500308, 2.968410348757589023 ) ) ;
#22955=ORIENTED_EDGE ( 'NONE', *, *, #20549, .T. ) ;
#22959=CARTESIAN_POINT ( 'NONE',  ( -62.55320287144887459, 17.87319849854531384, -15.63420304729892152 ) ) ;
#22960=CARTESIAN_POINT ( 'NONE',  ( 109.3047266816501377, 28.44977739115299187, 29.65533130390193151 ) ) ;
#22966=CARTESIAN_POINT ( 'NONE',  ( -15.15117926080556465, 7.479311051197340632, -95.00000000000133582 ) ) ;
#22967=CARTESIAN_POINT ( 'NONE',  ( 163.7403496014744633, 64.00600007368879574, 32.78579552523091678 ) ) ;
#22969=CARTESIAN_POINT ( 'NONE',  ( 69.72564955710446100, 15.37006465677306721, 13.82808010939183596 ) ) ;
#22971=CARTESIAN_POINT ( 'NONE',  ( 92.53566308513170213, 21.52138666710685300, 41.86074465914231979 ) ) ;
#22974=CARTESIAN_POINT ( 'NONE',  ( 108.3753929817421664, 29.13179266688724312, -9.298753174311741532 ) ) ;
#22975=CARTESIAN_POINT ( 'NONE',  ( -49.12372073857198274, 14.20664392157176081, 6.353358384741189191 ) ) ;
#22977=CARTESIAN_POINT ( 'NONE',  ( -126.7944042662569046, 48.29830493043728978, -23.02871842506080213 ) ) ;
#22980=CARTESIAN_POINT ( 'NONE',  ( 86.98834118549886796, 19.54364583620759532, 83.40280743883631942 ) ) ;
#22982=ORIENTED_EDGE ( 'NONE', *, *, #59019, .F. ) ;
#22984=ORIENTED_EDGE ( 'NONE', *, *, #43163, .T. ) ;
#22985=CARTESIAN_POINT ( 'NONE',  ( 157.4703587214989398, -170.0000000000000000, 44.40946747225338953 ) ) ;
#22986=CARTESIAN_POINT ( 'NONE',  ( -165.6851864275418507, 80.65423768630888901, 91.01486207682364693 ) ) ;
#22987=CARTESIAN_POINT ( 'NONE',  ( -47.60396279792517760, 12.80997843568595052, -16.87800407465863373 ) ) ;
#22988=CARTESIAN_POINT ( 'NONE',  ( 102.8066580714140628, 25.59117171227001819, -17.58622140034226788 ) ) ;
#22989=CARTESIAN_POINT ( 'NONE',  ( -62.30163634902122993, 17.79682011226254446, -44.70441580692872208 ) ) ;
#22992=CARTESIAN_POINT ( 'NONE',  ( -15.07200981767290848, 7.471751903425211339, 39.56416694737108486 ) ) ;
#22997=CARTESIAN_POINT ( 'NONE',  ( -142.6736406357357794, -170.0000000000000000, 94.99999999999866418 ) ) ;
#22998=CARTESIAN_POINT ( 'NONE',  ( -58.35358059297030309, 16.63726411742650413, -89.66742083260719198 ) ) ;
#22999=CARTESIAN_POINT ( 'NONE',  ( -165.7140086129056442, 80.68381997492572566, 37.10624841604320068 ) ) ;
#23000=CARTESIAN_POINT ( 'NONE',  ( 112.5612011511790342, 31.08353758940340228, -23.72632233143615466 ) ) ;
#23003=CARTESIAN_POINT ( 'NONE',  ( 135.0005116824454205, 43.29964618809724897, -24.09459631371699118 ) ) ;
#23004=ORIENTED_EDGE ( 'NONE', *, *, #32865, .T. ) ;
#23009=CARTESIAN_POINT ( 'NONE',  ( -15.08468253268400083, 7.472949889606720575, 8.823174773458156039 ) ) ;
#23010=FACE_OUTER_BOUND ( 'NONE', #60637, .T. ) ;
#23011=CARTESIAN_POINT ( 'NONE',  ( 55.56474667084420815, 11.06706367715631778, -15.38353893648206849 ) ) ;
#23014=DIRECTION ( 'NONE',  ( 0.000000000000000000, -1.000000000000000000, 0.000000000000000000 ) ) ;
#23015=VERTEX_POINT ( 'NONE', #50701 ) ;
#23018=CARTESIAN_POINT ( 'NONE',  ( -55.54036735998997898, 15.85474597822064702, -62.06087458892358200 ) ) ;
#23019=CARTESIAN_POINT ( 'NONE',  ( 197.1979149960398274, 98.19687999751999996, -71.00583573180291808 ) ) ;
#23021=CARTESIAN_POINT ( 'NONE',  ( -0.8863173716723027340, 7.545240407187534970, -40.04092009748728032 ) ) ;
#23023=CARTESIAN_POINT ( 'NONE',  ( -47.68562151781910785, -170.0000000000000000, -95.00000000000133582 ) ) ;
#23026=FACE_BOUND ( 'NONE', #67774, .T. ) ;
#23038=CARTESIAN_POINT ( 'NONE',  ( 46.70715146412976537, 9.472433765547007667, -71.68030912521341236 ) ) ;
#23040=ORIENTED_EDGE ( 'NONE', *, *, #21133, .F. ) ;
#23041=ORIENTED_EDGE ( 'NONE', *, *, #5920, .F. ) ;
#23042=CARTESIAN_POINT ( 'NONE',  ( -130.2299182487217024, 49.41538973246969846, -89.96770515742747421 ) ) ;
#23043=CARTESIAN_POINT ( 'NONE',  ( 188.5747655895476100, 86.52284255640786625, 89.95077014674320992 ) ) ;
#23044=ORIENTED_EDGE ( 'NONE', *, *, #18986, .T. ) ;
#23045=ORIENTED_EDGE ( 'NONE', *, *, #17864, .T. ) ;
#23046=CARTESIAN_POINT ( 'NONE',  ( 174.2469308602415197, 71.96142024047681218, -46.82003836444015121 ) ) ;
#23050=VERTEX_POINT ( 'NONE', #52085 ) ;
#23051=DIRECTION ( 'NONE',  ( 0.000000000000000000, 0.000000000000000000, 1.000000000000000000 ) ) ;
#23052=CARTESIAN_POINT ( 'NONE',  ( -177.5259994307673708, 92.16784265327251546, 5.389069799081259049 ) ) ;
#23053=CARTESIAN_POINT ( 'NONE',  ( -77.71448999903257970, 21.96089801565736721, -35.16068627303630478 ) ) ;
#23054=CARTESIAN_POINT ( 'NONE',  ( 80.01789329971975917, 17.27008742253428153, -93.44501639533700654 ) ) ;
#23056=CARTESIAN_POINT ( 'NONE',  ( -190.0468231512976161, 108.2116162189845170, 35.02347016645559563 ) ) ;
#23060=CARTESIAN_POINT ( 'NONE',  ( -73.10086105983761229, 21.34631349770504372, 16.12499931341085002 ) ) ;
#23061=CARTESIAN_POINT ( 'NONE',  ( 41.33692564073608366, 8.668977654195479943, -50.37004257708993293 ) ) ;
#23064=CARTESIAN_POINT ( 'NONE',  ( -118.5237170689549941, 41.82886034450997670, 90.37931702170654091 ) ) ;
#23066=CARTESIAN_POINT ( 'NONE',  ( 86.62931800182293784, 19.42108912189597092, -50.82156419891174437 ) ) ;
#23068=CARTESIAN_POINT ( 'NONE',  ( -143.8794621588507994, 59.54894433207190474, 60.10184585113807287 ) ) ;
#23069=CARTESIAN_POINT ( 'NONE',  ( 83.59652366361571296, 19.46709838196857945, 44.07574043631387184 ) ) ;
#23075=CARTESIAN_POINT ( 'NONE',  ( 140.1999945597799524, 45.38880890490935371, -20.68848176573018094 ) ) ;
#23076=CARTESIAN_POINT ( 'NONE',  ( 39.88975917505624835, 9.487965272711651465, 3.069283715499572907 ) ) ;
#23077=CARTESIAN_POINT ( 'NONE',  ( 87.59061758233886508, 19.75077892934019985, -62.71238299196379984 ) ) ;
#23083=CARTESIAN_POINT ( 'NONE',  ( 43.14356474118746831, 8.925336319666905993, 30.89513714664620281 ) ) ;
#23084=CARTESIAN_POINT ( 'NONE',  ( 197.2197025888161761, 96.62026035493815357, -17.64164879660345164 ) ) ;
#23087=CARTESIAN_POINT ( 'NONE',  ( 209.6698611676811197, 115.2210955123518517, -38.19286268395692474 ) ) ;
#23088=B_SPLINE_CURVE_WITH_KNOTS ( 'NONE', 3,
 ( #1793, #6704, #28150, #23249, #44694, #66173, #7419, #50321, #68236, #3511, #51364, #30597, #29546, #8804, #24638, #46072, #2824, #36218, #52049, #9489, #51015, #62251, #8452, #67543 ),
 .UNSPECIFIED., .F., .F.,
 ( 4, 2, 2, 2, 2, 2, 2, 2, 2, 2, 2, 4 ),
 ( 0.000000000000000000, 0.001774223329494980465, 0.002661334994242444893, 0.003548446658989908888, 0.004435558323737373750, 0.005322669988484837744, 0.007096893317979765733, 0.007984004982727195901, 0.008871116647474627803, 0.01064533997696948987, 0.01241956330646435194, 0.01419378663595921401 ),
 .UNSPECIFIED. ) ;
#23090=CARTESIAN_POINT ( 'NONE',  ( -78.66644367742109978, 23.39876645725288284, -76.96000122218160300 ) ) ;
#23091=CARTESIAN_POINT ( 'NONE',  ( -149.5074843970971301, -170.0000000000000000, 18.87627064943540134 ) ) ;
#23092=CARTESIAN_POINT ( 'NONE',  ( -24.07146890348362689, 8.497559956800399661, -41.35130633274434331 ) ) ;
#23093=CARTESIAN_POINT ( 'NONE',  ( 163.2886151008987952, 62.32020850087171482, -75.20809123641221561 ) ) ;
#23101=DIRECTION ( 'NONE',  ( 0.000000000000000000, 0.000000000000000000, 1.000000000000000000 ) ) ;
#23107=CARTESIAN_POINT ( 'NONE',  ( 57.07246224906427301, 12.39953617563784860, 68.75870423085009975 ) ) ;
#23108=CARTESIAN_POINT ( 'NONE',  ( -13.47517652744367567, 8.334971000693556675, 15.72779575785819972 ) ) ;
#23113=CARTESIAN_POINT ( 'NONE',  ( 127.2358066117906787, 38.72257733469225371, -20.23951017382307782 ) ) ;
#23120=CARTESIAN_POINT ( 'NONE',  ( -31.92572261726339633, 10.69135962481465008, -50.31719736520186359 ) ) ;
#23121=DIRECTION ( 'NONE',  ( -0.000000000000000000, 1.000000000000000000, -0.000000000000000000 ) ) ;
#23125=CARTESIAN_POINT ( 'NONE',  ( -119.1795380581000074, 42.22910606512925114, -45.76561242440763522 ) ) ;
#23127=CARTESIAN_POINT ( 'NONE',  ( -147.3641864666714980, 62.38213854487954535, -22.66905609602007132 ) ) ;
#23133=CARTESIAN_POINT ( 'NONE',  ( -62.15063206372444427, 17.75106610013994768, 8.499825761613776010 ) ) ;
#23134=CARTESIAN_POINT ( 'NONE',  ( 197.8572563162090887, 97.41072138832262794, -40.73584554935744251 ) ) ;
#23135=CARTESIAN_POINT ( 'NONE',  ( -95.21085197937820510, 30.44372064875428663, 40.57601684981261059 ) ) ;
#23139=CARTESIAN_POINT ( 'NONE',  ( 18.21423326326596737, 6.590134686181412960, -35.90535394282123605 ) ) ;
#23145=CARTESIAN_POINT ( 'NONE',  ( -122.6739428120618953, 44.40980909172365898, -89.31540991285331188 ) ) ;
#23149=CARTESIAN_POINT ( 'NONE',  ( 15.78827728214693416, -170.0000000000000000, -77.36349468914950478 ) ) ;
#23154=CARTESIAN_POINT ( 'NONE',  ( -144.0702036543480631, 60.99138314440749298, -90.83095804928598227 ) ) ;
#23155=AXIS2_PLACEMENT_3D ( 'NONE', #10253, #31715, #53147 ) ;
#23156=CARTESIAN_POINT ( 'NONE',  ( -35.38560449531983920, 10.27249159032101389, -22.35498971822604375 ) ) ;
#23157=CARTESIAN_POINT ( 'NONE',  ( -180.3161328724958139, 97.10341277064809162, 40.46042418554912956 ) ) ;
#23158=CARTESIAN_POINT ( 'NONE',  ( -132.0738857626834601, 51.93126104279141941, 7.018657644745633029 ) ) ;
#23159=CARTESIAN_POINT ( 'NONE',  ( 16.77104078056616387, 7.540619757007627655, 71.81062785426281891 ) ) ;
#23160=EDGE_LOOP ( 'NONE', ( #5459, #42688 ) ) ;
#23161=EDGE_LOOP ( 'NONE', ( #61212, #65227, #61787, #23598 ) ) ;
#23166=VECTOR ( 'NONE', #47668, 1000.000000000000000 ) ;
#23169=CARTESIAN_POINT ( 'NONE',  ( -35.17686701826947626, 10.23452050416468317, -36.29668785629766603 ) ) ;
#23171=CARTESIAN_POINT ( 'NONE',  ( -94.81181312526928195, 29.14610013485190265, 92.47439075634365224 ) ) ;
#23174=CARTESIAN_POINT ( 'NONE',  ( -126.3458714439410784, 46.79154809309477514, 57.46449846362074965 ) ) ;
#23178=CARTESIAN_POINT ( 'NONE',  ( 85.67452303415197434, 19.09699411916384548, 71.51082955247741779 ) ) ;
#23181=CARTESIAN_POINT ( 'NONE',  ( 32.09567473596477782, 7.571373529017937365, 39.12545751119512261 ) ) ;
#23183=DIRECTION ( 'NONE',  ( 0.000000000000000000, 0.000000000000000000, 1.000000000000000000 ) ) ;
#23188=CARTESIAN_POINT ( 'NONE',  ( -51.78153763344962357, 13.82841714689605617, 4.206538418488238840 ) ) ;
#23190=CARTESIAN_POINT ( 'NONE',  ( 164.0105905242218398, 64.23277447906893656, -74.14879248810279933 ) ) ;
#23193=CARTESIAN_POINT ( 'NONE',  ( -188.7743570271016722, 108.2592512368506306, 92.51026036494342009 ) ) ;
#23194=ORIENTED_EDGE ( 'NONE', *, *, #5572, .T. ) ;
#23199=EDGE_CURVE ( 'NONE', #17554, #41847, #20413, .T. ) ;
#23200=CARTESIAN_POINT ( 'NONE',  ( -80.31691774066412393, 22.95709084517032750, 45.23817464378598885 ) ) ;
#23202=CARTESIAN_POINT ( 'NONE',  ( 43.35536254672140188, 9.973606330917817786, 31.03574407154524195 ) ) ;
#23204=CARTESIAN_POINT ( 'NONE',  ( 136.9798231265810387, 43.34196232604179500, -50.35791885916582089 ) ) ;
#23211=CARTESIAN_POINT ( 'NONE',  ( 32.09610685027467980, 8.582590950734818591, -17.98836414960963737 ) ) ;
#23213=CARTESIAN_POINT ( 'NONE',  ( -1.298947065946362001, 6.553849421084473548, 94.99999999999866418 ) ) ;
#23214=CARTESIAN_POINT ( 'NONE',  ( -7.336630171688594437, 7.867399454768211342, 56.96013162991088308 ) ) ;
#23216=FACE_OUTER_BOUND ( 'NONE', #39194, .T. ) ;
#23219=EDGE_LOOP ( 'NONE', ( #21435, #35487, #1864, #44697 ) ) ;
#23222=CARTESIAN_POINT ( 'NONE',  ( 164.8407099662994995, 63.61629583487393802, -18.19528167887739656 ) ) ;
#23223=CARTESIAN_POINT ( 'NONE',  ( 32.99392442438140449, 7.662387294680161887, 94.99999999999866418 ) ) ;
#23226=CARTESIAN_POINT ( 'NONE',  ( 141.3707934840545022, 46.15056991286792965, -70.39752903070149159 ) ) ;
#23228=EDGE_CURVE ( 'NONE', #27330, #19842, #10948, .T. ) ;
#23229=EDGE_CURVE ( 'NONE', #23453, #51654, #3050, .T. ) ;
#23235=CARTESIAN_POINT ( 'NONE',  ( 8.683531412707429453, 6.377173148747125708, 39.92982772978346162 ) ) ;
#23238=CARTESIAN_POINT ( 'NONE',  ( -62.56514071794335052, 16.82532503654672240, -69.55340720332647209 ) ) ;
#23239=CARTESIAN_POINT ( 'NONE',  ( 126.8191975983342132, 37.33444841723056840, -94.58288091666166508 ) ) ;
#23242=CARTESIAN_POINT ( 'NONE',  ( 89.87518614971253328, 20.55373388674512114, 3.589420107556450912 ) ) ;
#23246=CARTESIAN_POINT ( 'NONE',  ( 57.23886567152862881, 12.43405960935903565, 86.20712845614353625 ) ) ;
#23247=CARTESIAN_POINT ( 'NONE',  ( 39.40195752203892710, 9.424259417798134919, 29.91383430596324899 ) ) ;
#23248=CARTESIAN_POINT ( 'NONE',  ( 79.40386128751609363, -170.0000000000000000, -95.00000000000133582 ) ) ;
#23249=CARTESIAN_POINT ( 'NONE',  ( -180.0765937259068323, 96.80858110077558365, -93.08190667287861686 ) ) ;
#23250=CARTESIAN_POINT ( 'NONE',  ( 155.7262569076171985, 56.30477153194511430, 71.10411761268670716 ) ) ;
#23253=CARTESIAN_POINT ( 'NONE',  ( 135.0005116824453921, 43.29964618809727028, -77.78369749464437177 ) ) ;
#23254=CARTESIAN_POINT ( 'NONE',  ( -143.8634661037141598, 60.82480701605705065, -74.12280952559889613 ) ) ;
#23256=CARTESIAN_POINT ( 'NONE',  ( -153.1031717208031750, 68.63449618039562949, -48.89866867094185920 ) ) ;
#23258=CARTESIAN_POINT ( 'NONE',  ( -38.80621516088652356, 11.94263260276895089, 39.18500952932296855 ) ) ;
#23261=CARTESIAN_POINT ( 'NONE',  ( -15.15117926080556465, 7.479311051197340632, -95.00000000000133582 ) ) ;
#23264=CARTESIAN_POINT ( 'NONE',  ( -9.765753193741726790, 8.033970690975921869, 30.36677245833251959 ) ) ;
#23265=CARTESIAN_POINT ( 'NONE',  ( 160.9241720448059141, 60.38677655937336652, 16.73850549852324576 ) ) ;
#23268=VECTOR ( 'NONE', #40825, 1000.000000000000000 ) ;
#23270=CARTESIAN_POINT ( 'NONE',  ( -101.8187363387487494, 33.67461140603123226, -50.01457726497595502 ) ) ;
#23271=ORIENTED_EDGE ( 'NONE', *, *, #68056, .T. ) ;
#23275=CARTESIAN_POINT ( 'NONE',  ( 45.90128843543707404, 9.343910238294480308, 60.48342642519485679 ) ) ;
#23280=DIRECTION ( 'NONE',  ( -0.000000000000000000, 1.000000000000000000, -0.000000000000000000 ) ) ;
#23282=CARTESIAN_POINT ( 'NONE',  ( -119.2804658695887952, 43.47213805166349943, -19.11607275521528848 ) ) ;
#23283=ORIENTED_EDGE ( 'NONE', *, *, #29208, .F. ) ;
#23284=VERTEX_POINT ( 'NONE', #2694 ) ;
#23287=CARTESIAN_POINT ( 'NONE',  ( 180.2572128312847326, 77.77323980479698662, 56.18701387320973595 ) ) ;
#23289=CARTESIAN_POINT ( 'NONE',  ( -165.6208371326873987, 80.58821715390999429, 64.86840870663141345 ) ) ;
#23291=CARTESIAN_POINT ( 'NONE',  ( -171.5023337025455135, 86.83681590836889086, -22.70211854798193940 ) ) ;
#23293=ADVANCED_FACE ( 'NONE', ( #40322 ), #22493, .T. ) ;
#23294=LINE ( 'NONE', #49643, #22772 ) ;
#23295=ORIENTED_EDGE ( 'NONE', *, *, #11980, .T. ) ;
#23297=CARTESIAN_POINT ( 'NONE',  ( -14.19493007850031674, 7.389842975086043708, 60.49290409118579248 ) ) ;
#23299=FACE_OUTER_BOUND ( 'NONE', #57499, .T. ) ;
#23301=FACE_OUTER_BOUND ( 'NONE', #20281, .T. ) ;
#23302=CARTESIAN_POINT ( 'NONE',  ( -62.56514138729678365, 16.82532522382519247, -42.70885660030685216 ) ) ;
#23303=ORIENTED_EDGE ( 'NONE', *, *, #6348, .T. ) ;
#23306=CARTESIAN_POINT ( 'NONE',  ( -52.45048892661851170, 15.03803514841138345, 71.70015838030094812 ) ) ;
#23307=CYLINDRICAL_SURFACE ( 'NONE', #48939, 7.500000000000020428 ) ;
#23308=CARTESIAN_POINT ( 'NONE',  ( 211.3757499519976477, 117.8130818709823444, 66.97729077751435511 ) ) ;
#23312=EDGE_CURVE ( 'NONE', #15400, #37405, #14206, .T. ) ;
#23313=CARTESIAN_POINT ( 'NONE',  ( 55.90536342106780410, 11.13510150712953362, 8.031316846378679486 ) ) ;
#23317=CARTESIAN_POINT ( 'NONE',  ( 105.5230584365412909, 27.85718471813526165, -91.26905600704951382 ) ) ;
#23320=CARTESIAN_POINT ( 'NONE',  ( -61.77164219855453098, 17.63686644795249592, -12.50187732388345552 ) ) ;
#23321=CARTESIAN_POINT ( 'NONE',  ( 157.4703587214989398, -170.0000000000000000, -97.31328548006501933 ) ) ;
#23326=CARTESIAN_POINT ( 'NONE',  ( 163.5944155533005926, 63.88379440759437955, 32.57248427008062208 ) ) ;
#23328=CARTESIAN_POINT ( 'NONE',  ( -149.9475539515598541, 65.87716206616011050, -61.65738112195565890 ) ) ;
#23329=CARTESIAN_POINT ( 'NONE',  ( 69.72789637502503979, 15.37065610545703898, 7.113218370438198157 ) ) ;
#23330=CARTESIAN_POINT ( 'NONE',  ( 89.88695630745277754, 20.55793566325391097, 43.98461035498685590 ) ) ;
#23335=CARTESIAN_POINT ( 'NONE',  ( -126.3453033442920344, 47.99870040347946798, -23.06915330777029283 ) ) ;
#23337=CARTESIAN_POINT ( 'NONE',  ( 113.8568724296587646, 30.58972477291343495, -23.16725636275993239 ) ) ;
#23339=DIRECTION ( 'NONE',  ( 0.000000000000000000, 0.000000000000000000, 1.000000000000000000 ) ) ;
#23345=CARTESIAN_POINT ( 'NONE',  ( 177.7964363391244831, 76.75162026635256041, 3.207951730180587546 ) ) ;
#23346=CARTESIAN_POINT ( 'NONE',  ( -50.13771638889893723, 13.41835215703894235, -10.18558108554858421 ) ) ;
#23347=CARTESIAN_POINT ( 'NONE',  ( 106.4107271020440209, 27.14892220304137993, -23.02936651802438206 ) ) ;
#23348=CARTESIAN_POINT ( 'NONE',  ( 197.3059626281005876, 96.72682679064189415, 11.17401084065080674 ) ) ;
#23349=CARTESIAN_POINT ( 'NONE',  ( 210.3652912788962510, 116.2694780445520450, 85.47466341958396185 ) ) ;
#23353=CARTESIAN_POINT ( 'NONE',  ( -10.91976120871577649, 7.112268444252506150, 30.77925799739722379 ) ) ;
#23359=DIRECTION ( 'NONE',  ( -0.000000000000000000, 1.000000000000000000, -0.000000000000000000 ) ) ;
#23360=CARTESIAN_POINT ( 'NONE',  ( -57.15783124718920760, 16.30010385357887159, -89.19421615593020647 ) ) ;
#23361=CARTESIAN_POINT ( 'NONE',  ( -167.0073208999199323, 82.02183861952778443, 33.96945047750333657 ) ) ;
#23364=CARTESIAN_POINT ( 'NONE',  ( -105.8768181937898731, 34.64545164169051361, 17.77285717464364367 ) ) ;
#23365=B_SPLINE_CURVE_WITH_KNOTS ( 'NONE', 3,
 ( #21124, #52437, #42895, #36608, #336, #4932, #42568, #5613, #58389, #64715, #63685, #47834, #20417, #53103, #4256, #21791, #43239, #10199, #4586, #30990, #37277, #41881, #15501, #26055, #63338, #15150, #69296, #64025, #16172, #15833, #31668, #25716, #68940, #9880, #42223, #59077, #31333, #10894, #7518, #16526, #58727, #32366, #37981, #10546, #47147, #52760, #32021, #47482 ),
 .UNSPECIFIED., .F., .F.,
 ( 4, 2, 2, 2, 2, 2, 2, 2, 2, 2, 2, 2, 2, 2, 2, 2, 2, 2, 2, 2, 2, 2, 2, 4 ),
 ( 0.02554216173022672010, 0.02715505844859240209, 0.02796150680777521533, 0.02876795516695802857, 0.03038085188532359260, 0.03199374860368916357, 0.03360664532205472760, 0.03441309368123751655, 0.03521954204042029857, 0.03602599039960308752, 0.03683243875878587648, 0.03844533547715142663, 0.03925178383633420170, 0.04005823219551697678, 0.04086468055469975880, 0.04167112891388254081, 0.04247757727306530895, 0.04328402563224809096, 0.04489692235061371051, 0.04650981906897933005, 0.04731626742816215370, 0.04812271578734497735, 0.04973561250571069403, 0.05134850922407641072 ),
 .UNSPECIFIED. ) ;
#23367=CARTESIAN_POINT ( 'NONE',  ( 140.2200249818744737, 46.60103563593123255, -20.65665471008218290 ) ) ;
#23368=ORIENTED_EDGE ( 'NONE', *, *, #4434, .F. ) ;
#23369=VERTEX_POINT ( 'NONE', #47310 ) ;
#23371=AXIS2_PLACEMENT_3D ( 'NONE', #46192, #15231, #41276 ) ;
#23381=CARTESIAN_POINT ( 'NONE',  ( -53.38256734720886243, 14.24001356352782643, 30.50165874791065335 ) ) ;
#23382=CARTESIAN_POINT ( 'NONE',  ( 199.2049631873262570, 100.7347227143600321, 68.66534253790618436 ) ) ;
#23386=CARTESIAN_POINT ( 'NONE',  ( 197.3119541548906568, 98.33923235143194574, -71.98455133656509020 ) ) ;
#23388=CARTESIAN_POINT ( 'NONE',  ( -4.731197926646205865, 7.716745361328039898, -49.75446812449514766 ) ) ;
#23389=CARTESIAN_POINT ( 'NONE',  ( -171.2055437419722352, 85.02094814279229240, -88.63902259587010235 ) ) ;
#23392=CARTESIAN_POINT ( 'NONE',  ( -31.43908319763710679, -170.0000000000000000, -62.16174795566551836 ) ) ;
#23397=CARTESIAN_POINT ( 'NONE',  ( -133.1093894320205493, 51.43221067881453479, -71.37503833356859673 ) ) ;
#23403=CARTESIAN_POINT ( 'NONE',  ( 188.2509234269329852, 86.16546166485385072, 92.74063656379689746 ) ) ;
#23406=CARTESIAN_POINT ( 'NONE',  ( 176.4367926094705297, 74.03315361639849357, -49.61664505837055827 ) ) ;
#23407=CARTESIAN_POINT ( 'NONE',  ( -178.5790738944853615, 93.41591512785083751, -63.90684885259965853 ) ) ;
#23408=B_SPLINE_CURVE_WITH_KNOTS ( 'NONE', 3,
 ( #2232, #51455, #67301, #61990, #66605, #56728, #23345, #66269, #23681, #7151, #28612, #44788, #45124, #18395, #20126, #41578, #46503, #10251, #15195, #41924, #14502, #57415, #26094, #31036, #63034, #62702, #30685, #4631, #20813, #19783, #36655, #21167, #47194, #47524, #35961, #57763, #25765, #4976, #52478, #52810, #25420, #31713, #9577, #9230 ),
 .UNSPECIFIED., .F., .F.,
 ( 4, 2, 2, 2, 2, 2, 2, 2, 2, 2, 2, 2, 2, 2, 2, 2, 2, 2, 2, 2, 2, 4 ),
 ( 0.02895403260893137515, 0.03071603688922227085, 0.03247804116951316655, 0.03424004544980405879, 0.03600204973009495796, 0.03776405401038585019, 0.03864505615053129284, 0.03952605829067672161, 0.04040706043082216425, 0.04128806257096759996, 0.04216906471111303567, 0.04305006685125847138, 0.04393106899140390709, 0.04481207113154934280, 0.04569307327169477850, 0.04657407541184021421, 0.04745507755198564992, 0.04833607969213108563, 0.05009808397242195011, 0.05186008825271282152, 0.05362209253300369294, 0.05714610109358540802 ),
 .UNSPECIFIED. ) ;
#23415=CARTESIAN_POINT ( 'NONE',  ( 15.78827728214693416, 6.500811158483322139, -89.20804527961313113 ) ) ;
#23416=CARTESIAN_POINT ( 'NONE',  ( -52.45048892661851880, 15.03803514841137989, -8.833493391090108560 ) ) ;
#23419=CARTESIAN_POINT ( 'NONE',  ( 111.1868021579656585, 29.32055685204858975, -35.96702300233707916 ) ) ;
#23420=CARTESIAN_POINT ( 'NONE',  ( -77.02112161466367013, 22.77583432622784798, 18.39477498643213238 ) ) ;
#23421=CARTESIAN_POINT ( 'NONE',  ( 45.04360969585142982, 9.210232288266707812, -38.15382515615639392 ) ) ;
#23423=CARTESIAN_POINT ( 'NONE',  ( -133.1633009596832835, 51.47055553769570935, 93.77542264256487670 ) ) ;
#23425=CARTESIAN_POINT ( 'NONE',  ( 84.97343609940689646, 18.86260005312943733, -36.00277291887266529 ) ) ;
#23429=CARTESIAN_POINT ( 'NONE',  ( -142.5211356634642073, 58.47296527616907724, 62.32377730571725749 ) ) ;
#23432=CARTESIAN_POINT ( 'NONE',  ( 93.32228019177715339, 22.88890999585040475, 33.81840254634702347 ) ) ;
#23434=CARTESIAN_POINT ( 'NONE',  ( 141.3707934840545022, 46.15056991286794386, -16.70842784977412521 ) ) ;
#23436=CARTESIAN_POINT ( 'NONE',  ( -178.5750994113944898, 94.98114813978523330, -20.53983915495086165 ) ) ;
#23437=EDGE_CURVE ( 'NONE', #48053, #29969, #20056, .T. ) ;
#23442=CARTESIAN_POINT ( 'NONE',  ( 46.65037935242577305, 9.463293687292226863, 39.35581152172980524 ) ) ;
#23446=DIRECTION ( 'NONE',  ( -0.000000000000000000, 1.000000000000000000, -0.000000000000000000 ) ) ;
#23447=CARTESIAN_POINT ( 'NONE',  ( -75.43495400358861502, 22.18831810339352018, -76.23245966557912823 ) ) ;
#23448=CARTESIAN_POINT ( 'NONE',  ( -104.1244073710069955, 33.72720758483610126, 72.14810588085583731 ) ) ;
#23449=FACE_OUTER_BOUND ( 'NONE', #31547, .T. ) ;
#23453=VERTEX_POINT ( 'NONE', #26903 ) ;
#23455=CARTESIAN_POINT ( 'NONE',  ( -173.1211646369891355, -170.0000000000000000, 92.01079578756841215 ) ) ;
#23456=CARTESIAN_POINT ( 'NONE',  ( -83.51052366780672287, 24.22613130369187573, 70.49372462622615387 ) ) ;
#23460=CARTESIAN_POINT ( 'NONE',  ( -102.2801239173131052, 33.91021738430207932, -76.85912785543962400 ) ) ;
#23462=CARTESIAN_POINT ( 'NONE',  ( 57.09527843067914432, 12.40436368789086785, 32.70209107450780550 ) ) ;
#23469=LINE ( 'NONE', #39633, #20847 ) ;
#23470=CARTESIAN_POINT ( 'NONE',  ( 200.4600337307565212, 100.7087439352120981, 69.75767833949197438 ) ) ;
#23471=CARTESIAN_POINT ( 'NONE',  ( -97.21582058037952834, 30.28155166330514803, -90.65436857541234872 ) ) ;
#23476=CARTESIAN_POINT ( 'NONE',  ( -37.37206033059242571, 11.66494618096613323, -47.41181603092942254 ) ) ;
#23480=CARTESIAN_POINT ( 'NONE',  ( -165.7109829243804029, 79.24174252277771302, 90.83868518818385951 ) ) ;
#23483=CARTESIAN_POINT ( 'NONE',  ( -142.2626321327577159, 58.26997216742665131, -17.42748240704912988 ) ) ;
#23484=CARTESIAN_POINT ( 'NONE',  ( -1.454841858088669948, 7.566772088227306625, -73.72818962830181988 ) ) ;
#23486=ORIENTED_EDGE ( 'NONE', *, *, #28494, .F. ) ;
#23487=CARTESIAN_POINT ( 'NONE',  ( 164.6046919270428930, 64.73376589608267295, -95.00000000000133582 ) ) ;
#23488=CARTESIAN_POINT ( 'NONE',  ( 198.4017331595409246, 98.09114638179335088, -47.91029365316073552 ) ) ;
#23489=CARTESIAN_POINT ( 'NONE',  ( -97.48179118242300945, 31.52606332398819688, 32.23367912195875817 ) ) ;
#23490=CARTESIAN_POINT ( 'NONE',  ( 23.03864809957654813, 6.841061756139156458, -41.08436505523182092 ) ) ;
#23491=CARTESIAN_POINT ( 'NONE',  ( 116.0822834687217409, 32.80169113915574286, 14.99919757508403606 ) ) ;
#23497=CARTESIAN_POINT ( 'NONE',  ( -71.16584859396994034, 19.60484997908768179, -15.53593528491745879 ) ) ;
#23499=CARTESIAN_POINT ( 'NONE',  ( -11.13714165684778656, 8.138643170880696331, -76.49629683574410421 ) ) ;
#23504=CARTESIAN_POINT ( 'NONE',  ( -72.21889834709583056, 21.03534256744171316, -38.75225259531774213 ) ) ;
#23506=CARTESIAN_POINT ( 'NONE',  ( 179.3667785869576221, 78.30612312851273771, -90.10490419269625306 ) ) ;
#23508=CARTESIAN_POINT ( 'NONE',  ( 135.6647932137617545, 43.70902528961477174, 44.30326689254214045 ) ) ;
#23509=CARTESIAN_POINT ( 'NONE',  ( 154.6343438497236775, 55.47873774496031274, -90.35998153076583606 ) ) ;
#23520=CARTESIAN_POINT ( 'NONE',  ( -173.1211646369891355, -170.0000000000000000, -76.55650775521370122 ) ) ;
#23521=CARTESIAN_POINT ( 'NONE',  ( -142.1381007084227122, 58.17237452544241449, 36.80006697400171589 ) ) ;
#23525=CARTESIAN_POINT ( 'NONE',  ( 82.95057496836383848, 18.19812356106674045, 70.61033162475500546 ) ) ;
#23527=CARTESIAN_POINT ( 'NONE',  ( -95.93275853296375999, 30.78481241411489577, -92.20198253166996949 ) ) ;
#23532=DIRECTION ( 'NONE',  ( 0.000000000000000000, 0.000000000000000000, 1.000000000000000000 ) ) ;
#23535=CARTESIAN_POINT ( 'NONE',  ( -49.45858366215607305, 13.25262207532076175, 5.971190123746847433 ) ) ;
#23539=ADVANCED_FACE ( 'NONE', ( #44110, #65956, #23722, #18441, #2275, #34640, #33933, #49734, #23026, #22671, #50103, #1218, #6838, #66644, #45165, #50455, #27943, #12468, #1933, #39896, #39550, #44829, #28293, #49386, #54669, #6497, #1563, #61004, #65593, #12828, #7894, #61353, #66311, #60655, #38865, #60305, #12127, #17754, #34282, #29012, #33590, #39210, #55371, #13174, #55731, #7192, #28652, #56077, #11280, #17256, #16566, #49257, #16909, #5655, #15875, #64760, #54889, #38025, #59470, #54539, #33466, #59119, #32060, #21838, #32411, #27115, #48549, #69342, #21490, #32750, #6366, #6712, #65112, #53836, #54180, #22543, #6001, #37322, #16218, #53496, #27460, #65464, #22196, #59814, #384, #35, #43285, #48904, #743, #43635, #38369, #11629, #33102, #27819, #47879, #1091, #38727, #43984, #60172, #11993, #21164, #42609, #64064 ), #58774, .F. ) ;
#23543=CARTESIAN_POINT ( 'NONE',  ( -152.5046761101291963, 66.76407727525179325, -8.589501201676744913 ) ) ;
#23546=CARTESIAN_POINT ( 'NONE',  ( -55.53456145826332602, 15.85318253404849642, 57.16187836339481976 ) ) ;
#23550=CARTESIAN_POINT ( 'NONE',  ( 152.6804161981488335, 55.27286404993341762, -76.24495480003128023 ) ) ;
#23551=CARTESIAN_POINT ( 'NONE',  ( -98.69283175933883001, 30.99524616306737812, -22.27381787311723116 ) ) ;
#23552=CARTESIAN_POINT ( 'NONE',  ( 140.9169160367233360, 45.85398962664670108, -40.93936509524743173 ) ) ;
#23559=CARTESIAN_POINT ( 'NONE',  ( -3.255961059272218350, 7.643453059677440820, 16.73847348745228913 ) ) ;
#23560=CARTESIAN_POINT ( 'NONE',  ( 140.3960818782622368, 46.71517501795715788, 94.43580953081790597 ) ) ;
#23561=CARTESIAN_POINT ( 'NONE',  ( 181.0840389613909736, -170.0000000000000000, -70.56960825634330092 ) ) ;
#23568=CARTESIAN_POINT ( 'NONE',  ( -130.9162414595584494, 51.11675657752020641, -90.51570049338198487 ) ) ;
#23573=CARTESIAN_POINT ( 'NONE',  ( 157.4703587214989113, 58.92748579479258808, -24.27963370867398396 ) ) ;
#23574=CARTESIAN_POINT ( 'NONE',  ( 8.951900209438530709, 6.378066731449591131, 34.42046772285240763 ) ) ;
#23577=CARTESIAN_POINT ( 'NONE',  ( 66.30636076182547356, 14.49616748423541424, 70.91462538568637797 ) ) ;
#23579=ORIENTED_EDGE ( 'NONE', *, *, #20397, .T. ) ;
#23580=CARTESIAN_POINT ( 'NONE',  ( 162.7963212667073378, 63.21900188423068556, -38.33791397036713988 ) ) ;
#23583=CARTESIAN_POINT ( 'NONE',  ( 159.2389084450350083, 59.03884018680376755, -36.32203399312435721 ) ) ;
#23584=EDGE_LOOP ( 'NONE', ( #34728, #57310, #52120, #58584 ) ) ;
#23585=CARTESIAN_POINT ( 'NONE',  ( -95.60805465865864505, 30.63099276904602419, 7.711323492103204558 ) ) ;
#23586=ADVANCED_FACE ( 'NONE', ( #50270 ), #8049, .F. ) ;
#23587=EDGE_CURVE ( 'NONE', #52584, #31501, #3132, .T. ) ;
#23589=CARTESIAN_POINT ( 'NONE',  ( 31.90247004928963648, 8.563336936370818719, 36.91044412156482224 ) ) ;
#23590=CARTESIAN_POINT ( 'NONE',  ( 66.73431804020511038, 14.60294556126670784, 30.79520888878160179 ) ) ;
#23591=CARTESIAN_POINT ( 'NONE',  ( -128.1219934350341703, 47.97781708504714970, -8.393129055976467967 ) ) ;
#23593=CARTESIAN_POINT ( 'NONE',  ( 126.3580543567275072, 37.07735301062817257, -70.06395634770694869 ) ) ;
#23597=CARTESIAN_POINT ( 'NONE',  ( -12.39770133248888939, 8.241491894828994802, 58.49459516380375845 ) ) ;
#23598=ORIENTED_EDGE ( 'NONE', *, *, #33376, .F. ) ;
#23600=VECTOR ( 'NONE', #60978, 1000.000000000000000 ) ;
#23601=CARTESIAN_POINT ( 'NONE',  ( -154.8006992380339000, 70.15733562427992354, -36.97816043303905786 ) ) ;
#23603=CARTESIAN_POINT ( 'NONE',  ( -35.38962320578852427, 11.29584325137385292, 44.09638843715468681 ) ) ;
#23604=CARTESIAN_POINT ( 'NONE',  ( -167.6413528428655866, 81.22881971256911982, -47.35830433886697932 ) ) ;
#23605=DIRECTION ( 'NONE',  ( -0.000000000000000000, 1.000000000000000000, -0.000000000000000000 ) ) ;
#23607=CARTESIAN_POINT ( 'NONE',  ( -54.09522495088364735, 14.42642983673692392, -77.01522855835996495 ) ) ;
#23608=CARTESIAN_POINT ( 'NONE',  ( 208.9507214515059843, 112.3605999017434982, -50.01955735436095551 ) ) ;
#23609=CARTESIAN_POINT ( 'NONE',  ( -10.23531775138760658, 8.068923942586302189, 30.50907025205252410 ) ) ;
#23610=CARTESIAN_POINT ( 'NONE',  ( 164.4728833318993111, 63.30716077995680990, 12.76463807767628644 ) ) ;
#23612=CARTESIAN_POINT ( 'NONE',  ( -99.10674985723794350, 32.31836975419496838, -49.32651561662824236 ) ) ;
#23617=CARTESIAN_POINT ( 'NONE',  ( 45.02738683369923223, 9.207938468499236251, 59.29196373395410546 ) ) ;
#23620=ADVANCED_FACE ( 'NONE', ( #23887 ), #2776, .F. ) ;
#23624=CARTESIAN_POINT ( 'NONE',  ( -78.19460645047364267, 22.14203592077027238, 57.26275173013679876 ) ) ;
#23628=DIRECTION ( 'NONE',  ( -0.000000000000000000, 1.000000000000000000, -0.000000000000000000 ) ) ;
#23629=CARTESIAN_POINT ( 'NONE',  ( 173.7227242028391174, 71.47307702680409136, 62.18859588645529612 ) ) ;
#23632=CARTESIAN_POINT ( 'NONE',  ( -165.7149569557575433, 80.68479365246973600, -14.14659806419673416 ) ) ;
#23633=VECTOR ( 'NONE', #49800, 1000.000000000000000 ) ;
#23636=CARTESIAN_POINT ( 'NONE',  ( 103.0004140566503139, 26.76634862952792560, -41.40820395346565164 ) ) ;
#23637=DIRECTION ( 'NONE',  ( 0.000000000000000000, 0.000000000000000000, 1.000000000000000000 ) ) ;
#23640=DIRECTION ( 'NONE',  ( -0.8160245890732938934, -0.5780171883497599028, 0.000000000000000000 ) ) ;
#23641=FACE_BOUND ( 'NONE', #11196, .T. ) ;
#23646=CARTESIAN_POINT ( 'NONE',  ( -176.3763474213711220, 92.36993073950279154, 4.706365262177376607 ) ) ;
#23647=CARTESIAN_POINT ( 'NONE',  ( 157.4703587214989113, 57.65129005721576760, 2.564916881789689018 ) ) ;
#23651=LINE ( 'NONE', #65348, #3379 ) ;
#23652=CARTESIAN_POINT ( 'NONE',  ( 197.8588046850312878, 99.02485934465610740, -40.73259020836108846 ) ) ;
#23657=CARTESIAN_POINT ( 'NONE',  ( -86.15275984831842493, 25.31588180512566311, -68.94000942011957989 ) ) ;
#23658=CARTESIAN_POINT ( 'NONE',  ( -57.42826130032240428, 16.37596353166459906, -22.98975030771917361 ) ) ;
#23659=CARTESIAN_POINT ( 'NONE',  ( 89.87840278991590992, 21.62393877508912254, -76.93015269146556534 ) ) ;
#23661=ORIENTED_EDGE ( 'NONE', *, *, #66589, .T. ) ;
#23662=CARTESIAN_POINT ( 'NONE',  ( 45.89268866913130296, 10.36133864615983313, 68.02416549870430629 ) ) ;
#23665=CARTESIAN_POINT ( 'NONE',  ( 70.26639875985993910, 15.51307715494296602, 12.45038511837332074 ) ) ;
#23668=CARTESIAN_POINT ( 'NONE',  ( -47.60266343315662141, 13.84328785304052900, 11.97199953281541340 ) ) ;
#23669=CARTESIAN_POINT ( 'NONE',  ( -125.8938041572051389, 47.69968343338778283, -23.06915330777029638 ) ) ;
#23671=CARTESIAN_POINT ( 'NONE',  ( 115.2288739107204378, 31.25773204386717552, -22.18589349865573013 ) ) ;
#23673=CARTESIAN_POINT ( 'NONE',  ( 80.86807176260094820, 17.53499872637983259, 86.08745821396813369 ) ) ;
#23678=VERTEX_POINT ( 'NONE', #18257 ) ;
#23679=CARTESIAN_POINT ( 'NONE',  ( 45.90128843543707404, 9.343910238294474979, 6.794325244267485964 ) ) ;
#23681=CARTESIAN_POINT ( 'NONE',  ( 176.6238742729555042, 75.60943990211367804, 3.915602851659322869 ) ) ;
#23683=CARTESIAN_POINT ( 'NONE',  ( 105.8022841538863901, 26.88074187880707910, -22.64102311982845706 ) ) ;
#23684=CARTESIAN_POINT ( 'NONE',  ( 201.9869293910474823, 102.6997661182766990, 16.86785852109921180 ) ) ;
#23685=CARTESIAN_POINT ( 'NONE',  ( 200.4927459033473554, 102.4002847909967358, 84.17857932545575750 ) ) ;
#23689=CARTESIAN_POINT ( 'NONE',  ( -11.14445507968271265, 7.129894202659277092, 30.88547439878327694 ) ) ;
#23690=ORIENTED_EDGE ( 'NONE', *, *, #59197, .T. ) ;
#23691=CARTESIAN_POINT ( 'NONE',  ( 15.78827728214693060, 7.507518794609574719, -8.674393508222097537 ) ) ;
#23693=EDGE_LOOP ( 'NONE', ( #45373, #33222, #3210, #54673 ) ) ;
#23694=CARTESIAN_POINT ( 'NONE',  ( -144.2155061717026001, 61.10843690942979833, 16.69664983447127682 ) ) ;
#23695=CARTESIAN_POINT ( 'NONE',  ( 188.2950976467626560, 87.71503060978555766, -68.48684010819242474 ) ) ;
#23696=CARTESIAN_POINT ( 'NONE',  ( -33.66581254962768810, 10.98864113404396825, 84.23646623808619438 ) ) ;
#23698=CARTESIAN_POINT ( 'NONE',  ( -101.3602137809054682, 32.31558061113913993, -49.97243961166241633 ) ) ;
#23703=CARTESIAN_POINT ( 'NONE',  ( 141.1220430186941996, 47.19066702031172866, -14.79883838647629446 ) ) ;
#23705=ORIENTED_EDGE ( 'NONE', *, *, #28738, .T. ) ;
#23706=CARTESIAN_POINT ( 'NONE',  ( 187.2885369019321615, 86.60256649394396788, 94.72525040610283042 ) ) ;
#23707=CARTESIAN_POINT ( 'NONE',  ( -102.2801239173131194, -170.0000000000000000, -15.67002667451224163 ) ) ;
#23709=CARTESIAN_POINT ( 'NONE',  ( 56.19513604272051310, 11.19349063094194996, -13.24700682944630259 ) ) ;
#23711=CARTESIAN_POINT ( 'NONE',  ( -188.6739852773920347, 108.2139733222100517, 36.71694418889097022 ) ) ;
#23712=CARTESIAN_POINT ( 'NONE',  ( 201.9721407532275066, 104.3507814346148308, 70.55148779649883295 ) ) ;
#23713=ORIENTED_EDGE ( 'NONE', *, *, #15494, .F. ) ;
#23715=CARTESIAN_POINT ( 'NONE',  ( -59.96408504033279030, 17.10126854471815605, -63.87159806579914800 ) ) ;
#23716=CARTESIAN_POINT ( 'NONE',  ( 201.5876148766343476, 103.8397408698165378, -63.83233738240677724 ) ) ;
#23720=CARTESIAN_POINT ( 'NONE',  ( -166.9982296371934467, 80.56207291422407479, 7.137779597826984457 ) ) ;
#23721=CARTESIAN_POINT ( 'NONE',  ( -78.66644367742109978, 22.32174330031318732, -50.11545063171791270 ) ) ;
#23722=FACE_BOUND ( 'NONE', #69418, .T. ) ;
#23724=CARTESIAN_POINT ( 'NONE',  ( -0.5158933718595627438, 6.525180340836106652, 66.15742312957483762 ) ) ;
#23728=CARTESIAN_POINT ( 'NONE',  ( 150.2060369882285613, 53.45752899907545697, 65.63963816870943901 ) ) ;
#23729=FACE_OUTER_BOUND ( 'NONE', #64704, .T. ) ;
#23731=DIRECTION ( 'NONE',  ( -0.000000000000000000, 1.000000000000000000, -0.000000000000000000 ) ) ;
#23732=VECTOR ( 'NONE', #41300, 1000.000000000000000 ) ;
#23742=CARTESIAN_POINT ( 'NONE',  ( 150.0980941434705187, 53.37942190380064034, 35.50453783569854238 ) ) ;
#23746=CARTESIAN_POINT ( 'NONE',  ( -180.5231752320737542, 95.76423526868920533, 12.72482689812798640 ) ) ;
#23747=CARTESIAN_POINT ( 'NONE',  ( -0.8055628312658252854, 6.535476276302840226, 8.119209976128034967 ) ) ;
#23750=CARTESIAN_POINT ( 'NONE',  ( -25.80443741485378695, 9.749985135376006085, -10.99864234085158010 ) ) ;
#23751=CARTESIAN_POINT ( 'NONE',  ( 157.4703587214989113, 57.65129005721576050, 17.56491688178971700 ) ) ;
#23756=ADVANCED_FACE ( 'NONE', ( #29853 ), #66127, .F. ) ;
#23761=CARTESIAN_POINT ( 'NONE',  ( -118.7818591202210570, 41.98604392202508251, 89.40455488510173154 ) ) ;
#23763=CARTESIAN_POINT ( 'NONE',  ( 82.95057496836383848, 18.19812356106674045, -36.76787073709972731 ) ) ;
#23764=ORIENTED_EDGE ( 'NONE', *, *, #67591, .T. ) ;
#23765=FACE_OUTER_BOUND ( 'NONE', #56839, .T. ) ;
#23766=CARTESIAN_POINT ( 'NONE',  ( 85.67165909753200026, 20.15791549876377076, 44.66629182770078899 ) ) ;
#23768=CARTESIAN_POINT ( 'NONE',  ( 184.0013086981203116, 81.60415045669145684, -9.957762043733517032 ) ) ;
#23771=CARTESIAN_POINT ( 'NONE',  ( -175.1968289912785224, 90.99944698359495021, -8.147980974625541606 ) ) ;
#23777=CARTESIAN_POINT ( 'NONE',  ( 158.3595886390532144, 58.34525996025799088, 56.29374580151184659 ) ) ;
#23782=CARTESIAN_POINT ( 'NONE',  ( -107.0584934212648420, 35.27493744466470105, 70.66521497598225210 ) ) ;
#23784=EDGE_CURVE ( 'NONE', #27023, #14111, #38479, .T. ) ;
#23785=CARTESIAN_POINT ( 'NONE',  ( 8.000000000000007105, 249.8719672152120381, 94.99999999999866418 ) ) ;
#23786=EDGE_LOOP ( 'NONE', ( #2513, #20289 ) ) ;
#23790=VECTOR ( 'NONE', #5606, 1000.000000000000000 ) ;
#23792=CARTESIAN_POINT ( 'NONE',  ( -71.19538519667726462, 19.61500601486861584, 90.87246897265434598 ) ) ;
#23794=B_SPLINE_CURVE_WITH_KNOTS ( 'NONE', 3,
 ( #58039, #46439, #40823, #54465, #21105, #58709, #53773, #27746, #42873, #22126, #27049, #64341, #1027, #64696, #42547, #37607, #10877, #21773, #38302, #15814, #33033, #59742 ),
 .UNSPECIFIED., .F., .F.,
 ( 4, 2, 2, 2, 2, 2, 2, 2, 2, 2, 4 ),
 ( 0.01028001298432954305, 0.01156964999863937214, 0.01221446850579429276, 0.01285928701294921338, 0.01414892402725907369, 0.01479374253441401513, 0.01543856104156895483, 0.01672819805587879086, 0.01737301656303372882, 0.01801783507018866332, 0.02059710909880842558 ),
 .UNSPECIFIED. ) ;
#23795=CARTESIAN_POINT ( 'NONE',  ( 129.1052153257903683, 39.78893484542955861, 42.83382366789680162 ) ) ;
#23797=LINE ( 'NONE', #33663, #65958 ) ;
#23799=CARTESIAN_POINT ( 'NONE',  ( -96.76336539645315327, 31.18045094643428783, -20.77494314902249783 ) ) ;
#23800=CARTESIAN_POINT ( 'NONE',  ( 56.28782924480458405, 12.23883190161851431, 40.66469570347511819 ) ) ;
#23801=CARTESIAN_POINT ( 'NONE',  ( 44.50274518366926912, 9.127743804123598537, 85.59476506304760335 ) ) ;
#23804=CARTESIAN_POINT ( 'NONE',  ( -1.728570918131775880, 6.570609986804655023, -47.29287092331269093 ) ) ;
#23806=CARTESIAN_POINT ( 'NONE',  ( -15.27733754929849930, 8.502213909106950851, 11.74977910805278292 ) ) ;
#23807=CARTESIAN_POINT ( 'NONE',  ( -148.6409722988649946, 63.44808865916660778, 18.82920403144292720 ) ) ;
#23808=CARTESIAN_POINT ( 'NONE',  ( -102.2801239173131194, -170.0000000000000000, -8.170026674512227416 ) ) ;
#23809=CARTESIAN_POINT ( 'NONE',  ( 197.1980152960109933, 96.59350208824302797, 63.88959311545310271 ) ) ;
#23810=B_SPLINE_CURVE_WITH_KNOTS ( 'NONE', 3,
 ( #36737, #22275, #43372, #64844, #32829, #43018, #54258, #48984, #31794, #63465, #15275, #26517, #7142, #28961, #39846, #65907, #6450, #23673, #59892, #1516, #54623, #60952, #7508, #54972, #2225, #61303, #50055, #22980, #50406, #11714, #33187, #34594, #18049, #17340, #44064, #56030, #66262, #44424, #39505, #7844, #27901, #60606, #45116, #49337, #65544, #38812, #12773, #34235, #13127, #55677, #12425, #43712, #33883, #1169 ),
 .UNSPECIFIED., .F., .F.,
 ( 4, 2, 2, 2, 2, 2, 2, 2, 2, 2, 2, 2, 2, 2, 2, 2, 2, 2, 2, 2, 2, 2, 2, 2, 2, 2, 4 ),
 ( 0.000000000000000000, 0.002050985862343569343, 0.003076478793515368109, 0.004101971724687166442, 0.005127464655858964340, 0.006152957587030763106, 0.007178450518202561005, 0.008203943449374360639, 0.009229436380546157670, 0.01025492931171795470, 0.01230591517406149152, 0.01435690103640502834, 0.01538239396757682190, 0.01640788689874861372, 0.01743337982992040555, 0.01845887276109219738, 0.01948436569226398921, 0.02050985862343578103, 0.02256084448577935081, 0.02358633741695114958, 0.02461183034812294834, 0.02563732327929474711, 0.02666281621046654587, 0.02768830914163834464, 0.02871380207281014341, 0.03076478793515374094, 0.03281577379749733153 ),
 .UNSPECIFIED. ) ;
#23811=CARTESIAN_POINT ( 'NONE',  ( 126.8114659053431410, 38.48351437375811201, -19.30170971946317948 ) ) ;
#23814=CARTESIAN_POINT ( 'NONE',  ( -190.3061188229048923, 108.5745819235681893, -11.38602486233425282 ) ) ;
#23815=CARTESIAN_POINT ( 'NONE',  ( -35.99414836699284592, 11.40630460607620478, -48.79583236974338689 ) ) ;
#23817=ADVANCED_FACE ( 'NONE', ( #56940 ), #8759, .T. ) ;
#23818=CARTESIAN_POINT ( 'NONE',  ( -177.1350677909553610, 91.70863480978455584, 85.65203958319301591 ) ) ;
#23820=DIRECTION ( 'NONE',  ( -0.000000000000000000, 1.000000000000000000, -0.000000000000000000 ) ) ;
#23821=EDGE_CURVE ( 'NONE', #30571, #38092, #55297, .T. ) ;
#23825=CARTESIAN_POINT ( 'NONE',  ( -0.3252226420479320534, 7.525368746738510417, -70.24936009779905532 ) ) ;
#23826=EDGE_CURVE ( 'NONE', #52549, #1174, #953, .T. ) ;
#23827=CARTESIAN_POINT ( 'NONE',  ( 151.3114175117524098, 54.26246727166002870, 86.30372711477225778 ) ) ;
#23832=CARTESIAN_POINT ( 'NONE',  ( -149.9475539515598257, 65.87716206616006787, 45.72082123989907387 ) ) ;
#23834=CARTESIAN_POINT ( 'NONE',  ( 21.73827885904430346, 6.764046335627705631, -47.59151161415723408 ) ) ;
#23836=CARTESIAN_POINT ( 'NONE',  ( 117.6853163455685234, 33.60747889659834442, 11.32768630793334452 ) ) ;
#23838=CARTESIAN_POINT ( 'NONE',  ( 62.04664474957770892, 12.44961624115901699, 44.76574209983286323 ) ) ;
#23842=CARTESIAN_POINT ( 'NONE',  ( -172.3038663181179402, 87.72015621195185986, 18.97714401617737678 ) ) ;
#23845=CARTESIAN_POINT ( 'NONE',  ( 23.28869764673362752, 6.856674305776599532, -69.37513493160868450 ) ) ;
#23847=CARTESIAN_POINT ( 'NONE',  ( -13.79190010541704225, 8.363435739308565431, -65.19196453362162913 ) ) ;
#23852=CARTESIAN_POINT ( 'NONE',  ( -74.20136529587823304, 21.74007521413448529, -36.58445878614914903 ) ) ;
#23854=CARTESIAN_POINT ( 'NONE',  ( 212.1913428512247322, 119.0779339498137972, -71.02503579638820952 ) ) ;
#23855=CARTESIAN_POINT ( 'NONE',  ( 137.5911612413395630, 44.91497189902067078, 43.51869277555784521 ) ) ;
#23857=CYLINDRICAL_SURFACE ( 'NONE', #50462, 7.500000000000013323 ) ;
#23858=CARTESIAN_POINT ( 'NONE',  ( -71.97767679134960872, -170.0000000000000000, 94.99999999999866418 ) ) ;
#23860=EDGE_LOOP ( 'NONE', ( #49909, #10331, #44622, #49877 ) ) ;
#23863=CARTESIAN_POINT ( 'NONE',  ( -31.92580063159128301, 9.671320706097198183, -50.31719736520185648 ) ) ;
#23864=CARTESIAN_POINT ( 'NONE',  ( -99.41031881471059251, 31.34608289732367226, 84.75242236955884323 ) ) ;
#23869=CARTESIAN_POINT ( 'NONE',  ( -106.7004823116342322, 36.22460663120047997, 44.09704765575368413 ) ) ;
#23871=CARTESIAN_POINT ( 'NONE',  ( 38.91493890549798351, 8.346224043800607006, 29.91383430596325255 ) ) ;
#23876=CARTESIAN_POINT ( 'NONE',  ( -125.6703656163502245, 47.55170550253213690, 57.46449846362074254 ) ) ;
#23877=CARTESIAN_POINT ( 'NONE',  ( -11.56945424397727962, 8.173256823723109576, -49.42130677995150023 ) ) ;
#23879=CARTESIAN_POINT ( 'NONE',  ( 157.0336341255055856, 57.31169401067816693, -51.12418429913763873 ) ) ;
#23882=CARTESIAN_POINT ( 'NONE',  ( -106.8349332276852977, 35.15552157736319572, -90.24117577083924857 ) ) ;
#23883=CARTESIAN_POINT ( 'NONE',  ( -157.0077369422017739, 70.81157624963285002, -15.74938127126972098 ) ) ;
#23884=ORIENTED_EDGE ( 'NONE', *, *, #28368, .F. ) ;
#23886=CARTESIAN_POINT ( 'NONE',  ( -55.54036735998996477, 15.85474597822063636, 72.16187836339486239 ) ) ;
#23887=FACE_OUTER_BOUND ( 'NONE', #38020, .T. ) ;
#23888=ORIENTED_EDGE ( 'NONE', *, *, #6157, .T. ) ;
#23890=CARTESIAN_POINT ( 'NONE',  ( 150.9128604434958163, 53.97103482421773180, -74.14689824430200815 ) ) ;
#23891=CARTESIAN_POINT ( 'NONE',  ( -31.92580063159127590, 9.671320706097196407, 30.21645440618916467 ) ) ;
#23893=CARTESIAN_POINT ( 'NONE',  ( -24.33435124463267130, 8.532637995283112176, 66.97631264891070657 ) ) ;
#23899=CARTESIAN_POINT ( 'NONE',  ( 33.31166872005965729, 8.707041209322236242, -20.65919876726036719 ) ) ;
#23900=CARTESIAN_POINT ( 'NONE',  ( 181.9295719569814764, 79.46350097013164770, 2.499600187509602112 ) ) ;
#23902=CARTESIAN_POINT ( 'NONE',  ( 127.0101228374496998, 38.59541841538369056, 87.63242888966352950 ) ) ;
#23904=ADVANCED_FACE ( 'NONE', ( #53357 ), #48764, .F. ) ;
#23905=CARTESIAN_POINT ( 'NONE',  ( -120.4586945679390482, 43.01762219615314109, -64.06711385159694316 ) ) ;
#23907=CARTESIAN_POINT ( 'NONE',  ( 164.8471526211110927, 63.62172173173269130, -15.39771934190674330 ) ) ;
#23909=CARTESIAN_POINT ( 'NONE',  ( 67.93926590385571274, 13.86859831467925197, 69.83615169925958810 ) ) ;
#23910=CARTESIAN_POINT ( 'NONE',  ( 137.4117721579686986, 43.61242559081429704, -63.74683598648854854 ) ) ;
#23918=CARTESIAN_POINT ( 'NONE',  ( -109.0191069781766657, -170.0000000000000000, 94.99999999999866418 ) ) ;
#23919=EDGE_CURVE ( 'NONE', #8726, #36296, #10825, .T. ) ;
#23922=CARTESIAN_POINT ( 'NONE',  ( 160.4986104110022609, 61.33701824525267199, -36.75893793876068827 ) ) ;
#23925=CARTESIAN_POINT ( 'NONE',  ( 161.7048274740120917, 61.01946783654761219, -49.83182248474824405 ) ) ;
#23926=AXIS2_PLACEMENT_3D ( 'NONE', #36408, #24130, #14943 ) ;
#23928=CARTESIAN_POINT ( 'NONE',  ( -98.67557579989343708, 32.10670856967968945, 4.580045852397571338 ) ) ;
#23930=CARTESIAN_POINT ( 'NONE',  ( 64.66746655423649770, 14.09646650629620979, 83.67892219932799946 ) ) ;
#23932=CARTESIAN_POINT ( 'NONE',  ( 82.94816950786172072, 19.25538918181906567, -9.938066344431240040 ) ) ;
#23933=CARTESIAN_POINT ( 'NONE',  ( -131.3154845336012215, 50.16828105866952114, -20.77399769732809531 ) ) ;
#23935=CARTESIAN_POINT ( 'NONE',  ( 152.1327777395850376, 53.61712543276776444, 69.02866056097568048 ) ) ;
#23936=CARTESIAN_POINT ( 'NONE',  ( 132.9485794245231602, 40.87843215479637138, -62.90929565402166190 ) ) ;
#23939=CARTESIAN_POINT ( 'NONE',  ( -119.1064753703575718, 43.36500113374746945, 94.99999999999866418 ) ) ;
#23942=CARTESIAN_POINT ( 'NONE',  ( -151.2428028786328014, 66.99705074331122034, -49.62230637302906899 ) ) ;
#23944=CARTESIAN_POINT ( 'NONE',  ( 15.78827728214693771, 7.507518794609574719, 71.85925826316895382 ) ) ;
#23945=CARTESIAN_POINT ( 'NONE',  ( -1.095583923122880332, 7.553030873957007785, 40.93520185086673280 ) ) ;
#23946=CARTESIAN_POINT ( 'NONE',  ( -7.825402957745085430, 6.891034867348153625, -89.10717191287116634 ) ) ;
#23947=CARTESIAN_POINT ( 'NONE',  ( -47.55235941796723864, 12.79790236059690400, -69.32320573674819286 ) ) ;
#23948=CARTESIAN_POINT ( 'NONE',  ( -0.5658006089934850547, 7.533733779014708531, -18.02006150488200831 ) ) ;
#23950=CARTESIAN_POINT ( 'NONE',  ( -60.97727891098335817, 16.35024395194894709, 6.347587653709224398 ) ) ;
#23954=CARTESIAN_POINT ( 'NONE',  ( 103.1567541746301657, 25.73937982110324540, -72.77541118461569170 ) ) ;
#23955=CARTESIAN_POINT ( 'NONE',  ( 45.04506994399702080, 10.22854084020123722, -21.24017278588418378 ) ) ;
#23956=CARTESIAN_POINT ( 'NONE',  ( 42.71504753277075395, 8.863481902720391048, 70.99139177545366408 ) ) ;
#23961=CYLINDRICAL_SURFACE ( 'NONE', #54375, 7.500000000000013323 ) ;
#23962=DIRECTION ( 'NONE',  ( -0.000000000000000000, 1.000000000000000000, -0.000000000000000000 ) ) ;
#23964=ORIENTED_EDGE ( 'NONE', *, *, #50890, .F. ) ;
#23969=CARTESIAN_POINT ( 'NONE',  ( 108.3942953861066485, 29.14039925067522674, 56.67208651439320732 ) ) ;
#23973=CARTESIAN_POINT ( 'NONE',  ( 59.29474530993688575, 12.86968658439548996, -9.859655179614705389 ) ) ;
#23976=CARTESIAN_POINT ( 'NONE',  ( 22.89270809252618832, 7.840160460323050806, -40.60289454668881604 ) ) ;
#23977=CARTESIAN_POINT ( 'NONE',  ( -86.15275984831841072, 25.31588180512570574, -15.25090823919218153 ) ) ;
#23980=CARTESIAN_POINT ( 'NONE',  ( 209.6877167158270652, 113.4449353909247407, -11.37733726706599491 ) ) ;
#23981=FACE_BOUND ( 'NONE', #5624, .T. ) ;
#23983=EDGE_CURVE ( 'NONE', #52549, #10264, #26773, .T. ) ;
#23992=CARTESIAN_POINT ( 'NONE',  ( -180.4614954900548298, 97.28277348252829881, 9.908402751631699701 ) ) ;
#23994=CARTESIAN_POINT ( 'NONE',  ( 210.6592759200687794, 116.7161312026394029, 68.11051040608630558 ) ) ;
#23995=CARTESIAN_POINT ( 'NONE',  ( -173.1211646369891355, 87.12891641440857882, 30.82169460664101734 ) ) ;
#24001=ORIENTED_EDGE ( 'NONE', *, *, #21033, .T. ) ;
#24003=CARTESIAN_POINT ( 'NONE',  ( -56.01329802674225533, 15.98369420723829570, -23.32578036508402519 ) ) ;
#24004=CARTESIAN_POINT ( 'NONE',  ( 94.14197848494937659, 23.19876128416616368, -70.15589403930768242 ) ) ;
#24008=CARTESIAN_POINT ( 'NONE',  ( 46.23304607317101045, 10.41544405387738692, 61.15242819165885635 ) ) ;
#24012=EDGE_CURVE ( 'NONE', #32175, #44993, #18442, .T. ) ;
#24013=CARTESIAN_POINT ( 'NONE',  ( 16.76400266940279238, 6.533513613209218640, 3.217594506424259482 ) ) ;
#24015=B_SPLINE_CURVE_WITH_KNOTS ( 'NONE', 3,
 ( #42462, #33313, #1291, #34705, #29077, #44180, #55089, #34360, #22745, #6913, #28724, #50522, #56141, #28364, #39621, #50173, #22393, #943, #60722, #60017, #65669, #49811, #34002, #2002, #38936, #54742, #7626, #11837, #39965, #60383, #12197, #23795, #43832, #17457, #12542, #28013, #18170, #44549 ),
 .UNSPECIFIED., .F., .F.,
 ( 4, 2, 2, 2, 2, 2, 2, 2, 2, 2, 2, 2, 2, 2, 2, 2, 2, 2, 4 ),
 ( 0.02546424207107602852, 0.02703543426729208138, 0.02782103036540014424, 0.02860662646350820362, 0.03017781865972439526, 0.03174901085594058342, 0.03332020305215677852, 0.03489139524837296669, 0.03646258744458916179, 0.03724818354269725240, 0.03803377964080534995, 0.03881937573891344750, 0.03960497183702154506, 0.04117616403323773322, 0.04274735622945392832, 0.04431854842567012343, 0.04588974062188631853, 0.04746093281810250669, 0.05060331721053488996 ),
 .UNSPECIFIED. ) ;
#24017=CARTESIAN_POINT ( 'NONE',  ( 58.46823952472683317, 12.69204591816733263, -37.23638717655476427 ) ) ;
#24019=CARTESIAN_POINT ( 'NONE',  ( -13.18921082026369618, 8.309042481534840263, -91.29599530343861602 ) ) ;
#24028=CARTESIAN_POINT ( 'NONE',  ( 46.64694836521740484, 9.462741877720631578, 8.614408483111491321 ) ) ;
#24030=CARTESIAN_POINT ( 'NONE',  ( -51.34325167237332010, 13.71819364263221530, -9.348823597919418305 ) ) ;
#24031=CARTESIAN_POINT ( 'NONE',  ( 103.8093541423578614, 26.01745837747064272, -20.46464144355324422 ) ) ;
#24034=CARTESIAN_POINT ( 'NONE',  ( 209.2537571925653026, 114.6008442271929226, 84.43188915064283151 ) ) ;
#24035=AXIS2_PLACEMENT_3D ( 'NONE', #20947, #37812, #5109 ) ;
#24038=CARTESIAN_POINT ( 'NONE',  ( -8.320652113663530969, 6.923290556636832349, 45.11558103944723541 ) ) ;
#24041=CARTESIAN_POINT ( 'NONE',  ( 9.050324533885206080, 7.384616180193987134, -19.50471979745130469 ) ) ;
#24042=ORIENTED_EDGE ( 'NONE', *, *, #8595, .F. ) ;
#24047=CARTESIAN_POINT ( 'NONE',  ( -38.46365568132284807, 11.87544203234370066, 88.69750035019276879 ) ) ;
#24052=CARTESIAN_POINT ( 'NONE',  ( 126.5880720616306121, 37.20544379858409911, -41.65621509857714955 ) ) ;
#24054=VERTEX_POINT ( 'NONE', #43413 ) ;
#24058=CARTESIAN_POINT ( 'NONE',  ( -14.55425570676091773, 7.423011834016144839, 14.09261391691513765 ) ) ;
#24060=CARTESIAN_POINT ( 'NONE',  ( -23.99924996210628692, 8.487987924059021694, -68.68209970087039551 ) ) ;
#24062=CARTESIAN_POINT ( 'NONE',  ( 12.46704290855393360, 6.417105965824391411, 3.941120416641372692 ) ) ;
#24065=CARTESIAN_POINT ( 'NONE',  ( -62.50103539982529099, 17.85731685071835528, -70.57177136977581711 ) ) ;
#24066=CARTESIAN_POINT ( 'NONE',  ( 201.5987353083854998, 103.8544727311226836, -77.51376041726710753 ) ) ;
#24069=CARTESIAN_POINT ( 'NONE',  ( -167.1540252468942072, 80.72321878831102993, 6.926423838769506958 ) ) ;
#24072=CARTESIAN_POINT ( 'NONE',  ( -47.55360235114366674, 12.79819361309568571, 64.14926665824262386 ) ) ;
#24081=CARTESIAN_POINT ( 'NONE',  ( 150.4542242713869484, 53.63744268572192198, 66.41804297856887729 ) ) ;
#24082=CARTESIAN_POINT ( 'NONE',  ( 204.6977192012829505, 108.0580384837234931, 29.20772073876942088 ) ) ;
#24083=B_SPLINE_CURVE_WITH_KNOTS ( 'NONE', 3,
 ( #51581, #41020, #9704, #29770, #31171, #3051, #63171, #51234, #61768, #67414, #3388, #14965, #68771, #19916, #9020, #46284, #41371, #30463, #14291, #67761, #3722, #24513, #57202, #51915, #20586, #35054, #35752, #25202, #62825, #52599, #14628, #36091, #57547, #30815, #9351, #8326, #45947, #19205, #13937, #47312, #41708, #13594, #52261 ),
 .UNSPECIFIED., .F., .F.,
 ( 4, 2, 2, 2, 2, 2, 2, 2, 1, 2, 2, 2, 2, 2, 2, 2, 2, 2, 2, 2, 2, 4 ),
 ( 3.469446951953614189E-18, 0.001466285743483493852, 0.002199428615225239910, 0.002932571486966985535, 0.004398857230450466810, 0.005865142973933949386, 0.007331428717417431094, 0.008064571589159175852, 0.008797714460900918007, 0.009530857332642663632, 0.01026400020438440752, 0.01173028594786789183, 0.01319657169135137788, 0.01466285743483486219, 0.01539600030657660261, 0.01612914317831834130, 0.01759542892180181173, 0.01906171466528528563, 0.01979485753702702258, 0.02052800040876875606, 0.02199428615225222650, 0.02346057189573569693 ),
 .UNSPECIFIED. ) ;
#24092=ORIENTED_EDGE ( 'NONE', *, *, #38853, .T. ) ;
#24093=VECTOR ( 'NONE', #18291, 1000.000000000000000 ) ;
#24095=CARTESIAN_POINT ( 'NONE',  ( 152.1381498073140790, 54.87048121475574192, 31.61318467975951663 ) ) ;
#24097=ORIENTED_EDGE ( 'NONE', *, *, #63202, .T. ) ;
#24099=CARTESIAN_POINT ( 'NONE',  ( -178.7483298110139458, 93.61800926271536127, 6.512559139046779855 ) ) ;
#24100=CARTESIAN_POINT ( 'NONE',  ( -2.190131154568199179, 6.589492063460817839, 5.815768188893855495 ) ) ;
#24101=CARTESIAN_POINT ( 'NONE',  ( 55.56634333706183781, 12.09342294753929892, -44.22217901802044082 ) ) ;
#24103=CARTESIAN_POINT ( 'NONE',  ( -83.13046924527392889, 25.15778674529016357, 31.88650284985251915 ) ) ;
#24109=CARTESIAN_POINT ( 'NONE',  ( 117.3110050642448101, 32.29133253383016466, -45.98121923047796145 ) ) ;
#24110=CARTESIAN_POINT ( 'NONE',  ( -77.71490760329790248, 23.03637365463981723, 3.619075319522604417 ) ) ;
#24111=CARTESIAN_POINT ( 'NONE',  ( 41.81982603358023454, 8.735900550613184379, -36.00357662167354533 ) ) ;
#24120=CARTESIAN_POINT ( 'NONE',  ( 185.1802655733641529, 82.84606286178492951, -10.58188840605224534 ) ) ;
#24121=CARTESIAN_POINT ( 'NONE',  ( -124.1094910780272329, 45.33021696310841975, 57.67627168393939741 ) ) ;
#24122=DIRECTION ( 'NONE',  ( -0.000000000000000000, 1.000000000000000000, -0.000000000000000000 ) ) ;
#24123=CARTESIAN_POINT ( 'NONE',  ( -177.1381400275772080, 93.26609858452818003, -21.71591573839441125 ) ) ;
#24125=CARTESIAN_POINT ( 'NONE',  ( -47.79955240516189008, 13.88975739862082648, 35.84505809694404377 ) ) ;
#24128=CARTESIAN_POINT ( 'NONE',  ( 104.7034219878852070, 26.40210929103716353, 58.87558030574008683 ) ) ;
#24130=DIRECTION ( 'NONE',  ( -0.000000000000000000, 1.000000000000000000, -0.000000000000000000 ) ) ;
#24131=AXIS2_PLACEMENT_3D ( 'NONE', #67493, #28821, #62203 ) ;
#24132=CARTESIAN_POINT ( 'NONE',  ( 185.5415406465189676, 83.23025870924411151, -49.77515318378037534 ) ) ;
#24133=CARTESIAN_POINT ( 'NONE',  ( -109.0297561673456386, 36.34391931706014134, 68.14367124605330162 ) ) ;
#24135=CARTESIAN_POINT ( 'NONE',  ( -25.35398647985413945, 8.671412257862215256, -47.20835425011359376 ) ) ;
#24136=CARTESIAN_POINT ( 'NONE',  ( 164.7250737226290482, 63.51898362052163804, -68.54626621448289825 ) ) ;
#24138=ORIENTED_EDGE ( 'NONE', *, *, #20958, .F. ) ;
#24140=ORIENTED_EDGE ( 'NONE', *, *, #24190, .T. ) ;
#24144=CARTESIAN_POINT ( 'NONE',  ( -73.15403579853486349, 20.29791129869458643, 86.51172062028520315 ) ) ;
#24146=FACE_OUTER_BOUND ( 'NONE', #52858, .T. ) ;
#24148=CARTESIAN_POINT ( 'NONE',  ( -60.66101049381763488, 17.30588917955501316, 42.82097766060025634 ) ) ;
#24149=CARTESIAN_POINT ( 'NONE',  ( -96.02159028238561689, 30.82695531378848841, -11.52968351012710180 ) ) ;
#24151=CARTESIAN_POINT ( 'NONE',  ( 31.91416675805597336, 7.553393781468399126, 90.55988232731206722 ) ) ;
#24156=CARTESIAN_POINT ( 'NONE',  ( -189.2826425734428994, 107.1493800926106275, -41.23753037017266365 ) ) ;
#24157=CARTESIAN_POINT ( 'NONE',  ( 181.0840389613909736, -170.0000000000000000, 44.30859410551141764 ) ) ;
#24158=ADVANCED_FACE ( 'NONE', ( #32874 ), #49029, .F. ) ;
#24160=CARTESIAN_POINT ( 'NONE',  ( -106.6940984894958007, 35.07986071359378855, -75.44142825345944914 ) ) ;
#24161=CARTESIAN_POINT ( 'NONE',  ( 126.3681350380370958, 38.23508791628618297, -16.18615085686329991 ) ) ;
#24167=CARTESIAN_POINT ( 'NONE',  ( -38.93847286785603501, 11.96870349976818027, -43.32391969549294686 ) ) ;
#24170=CARTESIAN_POINT ( 'NONE',  ( -178.4330126279765523, 93.24097428920383379, 86.68317579884340773 ) ) ;
#24172=CARTESIAN_POINT ( 'NONE',  ( -125.8938041572051105, 46.49392987655494380, -34.91370389823391918 ) ) ;
#24173=CARTESIAN_POINT ( 'NONE',  ( -148.4259959918497600, 63.26767374754767559, -8.043489788822235198 ) ) ;
#24174=CARTESIAN_POINT ( 'NONE',  ( 198.8752826725511227, 100.3130050945023299, 5.128836562248959119 ) ) ;
#24175=ORIENTED_EDGE ( 'NONE', *, *, #54937, .T. ) ;
#24177=CARTESIAN_POINT ( 'NONE',  ( 150.1779365646289932, 53.43719151385364086, 92.36095605438667633 ) ) ;
#24179=CARTESIAN_POINT ( 'NONE',  ( -58.32502757340554211, 16.62877055630753631, 4.207105285353801349 ) ) ;
#24180=CARTESIAN_POINT ( 'NONE',  ( 126.3580543567275640, 37.07735301062818678, 37.31424601414773434 ) ) ;
#24183=DIRECTION ( 'NONE',  ( -0.000000000000000000, 1.000000000000000000, -0.000000000000000000 ) ) ;
#24185=CIRCLE ( 'NONE', #12988, 243.4957430088094839 ) ;
#24190=EDGE_CURVE ( 'NONE', #62155, #8631, #2273, .T. ) ;
#24191=CARTESIAN_POINT ( 'NONE',  ( 55.52750043885184539, 11.05966813607792787, 36.82308146611499211 ) ) ;
#24197=CARTESIAN_POINT ( 'NONE',  ( 18.66025561752210038, 6.609375019058819412, -76.80469486127859113 ) ) ;
#24198=CARTESIAN_POINT ( 'NONE',  ( -133.3799602664182657, 52.86209125874979975, 65.49465508212347231 ) ) ;
#24204=CARTESIAN_POINT ( 'NONE',  ( 211.5034924207028268, 118.0100795718634998, -67.50466236550761323 ) ) ;
#24205=B_SPLINE_CURVE_WITH_KNOTS ( 'NONE', 3,
 ( #39247, #49070, #23423, #909, #39930, #7232, #6171, #33966, #28689, #22359, #59979, #44862, #22706, #44516, #65990, #49774, #45204, #50487, #65272, #1600, #60690, #17063, #33278, #65632, #54707, #6875, #7591, #18135, #6534, #12866, #66347, #61040, #34321, #28327, #49423, #1253, #33626, #55769, #17420, #38899, #61388, #55056, #2310, #23761, #13210, #23064, #25155, #14246, #7926, #56110, #46237, #45551, #8278, #3340, #51188, #51534 ),
 .UNSPECIFIED., .F., .F.,
 ( 4, 2, 2, 2, 2, 2, 2, 2, 2, 2, 2, 2, 2, 2, 2, 2, 2, 2, 2, 2, 2, 2, 2, 2, 2, 2, 2, 4 ),
 ( 0.000000000000000000, 0.002031929280119430282, 0.003047893920179118102, 0.004063858560238805921, 0.005079823200298493741, 0.006095787840358182427, 0.007111752480417870247, 0.008127717120477558066, 0.009143681760537246753, 0.01015964640059693370, 0.01117561104065662239, 0.01219157568071631108, 0.01320754032077599803, 0.01422350496083568498, 0.01625543424095507103, 0.01828736352107445534, 0.02031929280119383271, 0.02133525744125350579, 0.02235122208131317192, 0.02336718672137284153, 0.02438315136143250766, 0.02641508064155189198, 0.02743104528161158240, 0.02844700992167126935, 0.02946297456173096324, 0.03047893920179065019, 0.03149490384185034408, 0.03251086848191003104 ),
 .UNSPECIFIED. ) ;
#24206=CARTESIAN_POINT ( 'NONE',  ( 140.7888851157410102, 46.97220912571250295, 39.88480869005077523 ) ) ;
#24207=DIRECTION ( 'NONE',  ( -0.000000000000000000, 1.000000000000000000, -0.000000000000000000 ) ) ;
#24208=CARTESIAN_POINT ( 'NONE',  ( -132.8150886319751862, 52.45790550853842404, 8.374808787430902512 ) ) ;
#24209=CARTESIAN_POINT ( 'NONE',  ( 66.30230369578305272, 14.49551544185123220, -76.81116625487784688 ) ) ;
#24213=CARTESIAN_POINT ( 'NONE',  ( 210.9044300540503514, 115.2613339746486076, -93.29905180977844736 ) ) ;
#24217=EDGE_CURVE ( 'NONE', #6748, #56804, #52795, .T. ) ;
#24219=CARTESIAN_POINT ( 'NONE',  ( -72.21947956767112942, 21.03570528348185320, -19.61146733724643099 ) ) ;
#24220=EDGE_CURVE ( 'NONE', #11797, #11917, #24306, .T. ) ;
#24222=CARTESIAN_POINT ( 'NONE',  ( -104.1393288135077313, 34.86912007524089319, 45.30014082762043159 ) ) ;
#24223=ORIENTED_EDGE ( 'NONE', *, *, #57908, .T. ) ;
#24225=CARTESIAN_POINT ( 'NONE',  ( 33.03621582719334526, 7.666716336587123592, 33.44051306690047909 ) ) ;
#24227=CARTESIAN_POINT ( 'NONE',  ( 86.15454111412294935, 20.32174891186170029, 56.55663816294301682 ) ) ;
#24228=ORIENTED_EDGE ( 'NONE', *, *, #29845, .F. ) ;
#24234=CYLINDRICAL_SURFACE ( 'NONE', #68207, 7.500000000000020428 ) ;
#24235=CARTESIAN_POINT ( 'NONE',  ( 152.6560521232695748, 54.00248515670892147, -49.38016601471965572 ) ) ;
#24237=AXIS2_PLACEMENT_3D ( 'NONE', #68373, #30385, #51837 ) ;
#24238=ORIENTED_EDGE ( 'NONE', *, *, #56787, .T. ) ;
#24246=ORIENTED_EDGE ( 'NONE', *, *, #53019, .F. ) ;
#24249=CARTESIAN_POINT ( 'NONE',  ( 149.9683128897950155, 53.28564708287393614, -69.93847851234227164 ) ) ;
#24250=CARTESIAN_POINT ( 'NONE',  ( -37.38781680082738745, 10.64362327909142714, 33.12268043286852759 ) ) ;
#24251=CARTESIAN_POINT ( 'NONE',  ( -26.49516976694650339, 8.831756547364859600, 70.22208721445005608 ) ) ;
#24253=EDGE_CURVE ( 'NONE', #62112, #168, #35374, .T. ) ;
#24256=CARTESIAN_POINT ( 'NONE',  ( -151.2428028786327729, 66.99705074331122034, 57.75589598882568509 ) ) ;
#24257=CARTESIAN_POINT ( 'NONE',  ( -119.5267374018686724, 42.44190186039717361, 42.11622477189887803 ) ) ;
#24258=ORIENTED_EDGE ( 'NONE', *, *, #38422, .F. ) ;
#24260=CARTESIAN_POINT ( 'NONE',  ( 93.32502112557678231, 21.81526022999040038, 60.64118160440343530 ) ) ;
#24262=CARTESIAN_POINT ( 'NONE',  ( -118.3960663196801022, 41.75130200162921312, -69.82620201183787856 ) ) ;
#24264=CARTESIAN_POINT ( 'NONE',  ( 163.1265310614426483, 62.18610413911354584, -21.71095227450152620 ) ) ;
#24266=CARTESIAN_POINT ( 'NONE',  ( 64.69649025047540647, 13.06878919510321957, 56.84423949185725178 ) ) ;
#24267=CARTESIAN_POINT ( 'NONE',  ( 140.2200249818743885, 46.60103563593123255, 6.187895880381468317 ) ) ;
#24270=CARTESIAN_POINT ( 'NONE',  ( 163.7379901688712778, 64.00402364591245430, -12.65244977937952875 ) ) ;
#24274=CARTESIAN_POINT ( 'NONE',  ( 66.30230369578303851, 14.49551544185124818, 57.41158669744056908 ) ) ;
#24275=CARTESIAN_POINT ( 'NONE',  ( 126.6419157458061022, 37.23544530986323053, 92.77959788058313961 ) ) ;
#24276=B_SPLINE_CURVE_WITH_KNOTS ( 'NONE', 3,
 ( #16681, #5775, #38135, #11392, #37104, #153, #58545, #43406, #32867, #26554, #37794, #59932, #54299, #58893, #27582, #32516, #48666, #33229, #54659, #507, #49021, #861, #65225, #42720, #38489, #22314, #26892, #53613, #17017, #10363, #53263, #69453, #11750, #20928, #6487, #47988, #64177, #48320, #21611, #15990, #27934, #11056, #37438, #63847 ),
 .UNSPECIFIED., .F., .F.,
 ( 4, 2, 2, 2, 2, 2, 2, 2, 2, 2, 2, 2, 2, 2, 2, 2, 2, 2, 2, 2, 2, 4 ),
 ( 7.152448122690996019E-18, 0.001476829494128784797, 0.002215244241193187278, 0.002953658988257589543, 0.004430488482386393638, 0.005907317976515197300, 0.007384147470644000961, 0.008122562217708420573, 0.008860976964772839318, 0.01033780645890166987, 0.01181463595303050042, 0.01255305070009489314, 0.01329146544715928933, 0.01476829494128811815, 0.01550670968835254557, 0.01624512443541697645, 0.01772195392954585905, 0.01919878342367474511, 0.01993719817073917946, 0.02067561291780361729, 0.02215244241193247560, 0.02362927190606133043 ),
 .UNSPECIFIED. ) ;
#24278=CARTESIAN_POINT ( 'NONE',  ( 162.0812592823604916, 62.62783216273700049, -37.68953501586388910 ) ) ;
#24291=AXIS2_PLACEMENT_3D ( 'NONE', #58030, #53765, #42864 ) ;
#24293=CARTESIAN_POINT ( 'NONE',  ( -149.5074843970971017, 64.17983161892348676, -61.65738112195564469 ) ) ;
#24294=CARTESIAN_POINT ( 'NONE',  ( -144.5499722824449691, 60.08555854030711174, -90.35693536357965172 ) ) ;
#24295=CARTESIAN_POINT ( 'NONE',  ( 127.4750938923429402, 37.70245908594341699, -74.31642906583816455 ) ) ;
#24296=ORIENTED_EDGE ( 'NONE', *, *, #3724, .F. ) ;
#24297=CARTESIAN_POINT ( 'NONE',  ( -95.04371414958066566, 30.36527049547257562, 62.82467735017532817 ) ) ;
#24298=CARTESIAN_POINT ( 'NONE',  ( -7.825402957745081878, 7.899365992529270741, 56.96013162991089018 ) ) ;
#24300=CARTESIAN_POINT ( 'NONE',  ( -156.6862310659955142, 71.88416263379565407, -40.06925897084124699 ) ) ;
#24301=EDGE_CURVE ( 'NONE', #42183, #30648, #41967, .T. ) ;
#24304=CARTESIAN_POINT ( 'NONE',  ( -154.6171773099879658, 68.63761944777706958, -63.66210952773269582 ) ) ;
#24305=CARTESIAN_POINT ( 'NONE',  ( 55.50964472539083516, 11.05611641653240440, 90.85181882182600077 ) ) ;
#24306=B_SPLINE_CURVE_WITH_KNOTS ( 'NONE', 3,
 ( #40245, #49732, #29010, #12826, #12466, #34280, #61351, #55729, #33931, #66642, #45163, #24069, #23720, #18439, #54667, #44827, #45513, #60303, #18786, #27941, #39893, #66309, #13172, #29339, #6836, #49384, #34638, #7190, #39208, #56075, #44108, #55015, #28291, #7892, #1561, #50791, #65954, #17752, #62390, #14204, #19125, #35662, #40930, #68023, #52519, #31082 ),
 .UNSPECIFIED., .F., .F.,
 ( 4, 2, 2, 2, 2, 2, 2, 2, 2, 2, 2, 2, 2, 2, 2, 2, 2, 2, 2, 2, 2, 2, 4 ),
 ( 0.02989107162308296539, 0.03170280136394040132, 0.03351453110479783726, 0.03532626084565526625, 0.03713799058651270218, 0.03894972032737013812, 0.03985558519779883180, 0.04076145006822753242, 0.04166731493865623304, 0.04257317980908492672, 0.04347904467951362040, 0.04438490954994231408, 0.04529077442037101470, 0.04619663929079970838, 0.04710250416122840206, 0.04800836903165709574, 0.04891423390208579636, 0.04982009877251449004, 0.05163182851337182189, 0.05344355825422915374, 0.05525528799508648559, 0.05706701773594381744, 0.05887874747680114235 ),
 .UNSPECIFIED. ) ;
#24307=CARTESIAN_POINT ( 'NONE',  ( -53.38256734720888375, 14.24001356352780334, -76.87654361394403679 ) ) ;
#24308=CARTESIAN_POINT ( 'NONE',  ( -4.502148936856955608, 7.704491846230413721, -9.332046380200495150 ) ) ;
#24309=EDGE_CURVE ( 'NONE', #29362, #44986, #57802, .T. ) ;
#24310=CARTESIAN_POINT ( 'NONE',  ( 173.5843421840238250, 71.34465141434343138, 10.26728517241832250 ) ) ;
#24311=CARTESIAN_POINT ( 'NONE',  ( -62.56514071794336473, 16.82532503654673306, 10.98024456806455618 ) ) ;
#24312=ORIENTED_EDGE ( 'NONE', *, *, #35735, .F. ) ;
#24313=CARTESIAN_POINT ( 'NONE',  ( 198.7765072002625288, 100.1872738704526427, 94.99999999999866418 ) ) ;
#24315=ORIENTED_EDGE ( 'NONE', *, *, #43666, .T. ) ;
#24316=CARTESIAN_POINT ( 'NONE',  ( 105.4193882736796297, 26.71329717705292239, -76.03135858187803819 ) ) ;
#24317=CARTESIAN_POINT ( 'NONE',  ( 46.12582897016703498, 10.39833982076227414, -12.94356353922558611 ) ) ;
#24318=CARTESIAN_POINT ( 'NONE',  ( 43.96465529479667111, 9.046527005589350523, 58.28554417598712689 ) ) ;
#24320=EDGE_CURVE ( 'NONE', #49272, #44530, #83, .T. ) ;
#24325=EDGE_LOOP ( 'NONE', ( #9113, #54378 ) ) ;
#24327=FACE_OUTER_BOUND ( 'NONE', #63524, .T. ) ;
#24329=CARTESIAN_POINT ( 'NONE',  ( 180.6710448012268273, 78.18844465372406205, -24.38050707541595230 ) ) ;
#24331=CARTESIAN_POINT ( 'NONE',  ( 103.5589117581614715, 27.00490790413961761, 67.39597877340914067 ) ) ;
#24332=DIRECTION ( 'NONE',  ( -0.000000000000000000, 1.000000000000000000, -0.000000000000000000 ) ) ;
#24341=FACE_BOUND ( 'NONE', #39931, .T. ) ;
#24344=ORIENTED_EDGE ( 'NONE', *, *, #48961, .F. ) ;
#24350=CARTESIAN_POINT ( 'NONE',  ( 8.306098662352679796, 6.376413070772140479, 90.59040921272263347 ) ) ;
#24352=VERTEX_POINT ( 'NONE', #432 ) ;
#24354=CARTESIAN_POINT ( 'NONE',  ( -125.8938041572051389, 47.69968343338778283, -49.91370389823397602 ) ) ;
#24358=CARTESIAN_POINT ( 'NONE',  ( -86.15441609607630369, 25.31657638323078530, -69.95505817415272531 ) ) ;
#24360=CARTESIAN_POINT ( 'NONE',  ( 86.62931800182293784, 20.48449268398423939, -77.66611478937542756 ) ) ;
#24362=ORIENTED_EDGE ( 'NONE', *, *, #59441, .T. ) ;
#24363=CARTESIAN_POINT ( 'NONE',  ( 46.12611922993085045, 10.39838587005582227, 60.92721693493930246 ) ) ;
#24365=CARTESIAN_POINT ( 'NONE',  ( 23.28869764673362397, 6.856674305776598644, 11.15851683978236686 ) ) ;
#24372=CARTESIAN_POINT ( 'NONE',  ( 114.6632852039171127, 30.98120524556723510, -22.64169526929315879 ) ) ;
#24373=CARTESIAN_POINT ( 'NONE',  ( 80.71682498289317209, 18.54204664833076421, -38.68071917220413525 ) ) ;
#24374=AXIS2_PLACEMENT_3D ( 'NONE', #37539, #48084, #9098 ) ;
#24375=CARTESIAN_POINT ( 'NONE',  ( -170.0946319916217533, 85.30045104993550353, -89.02616900977504599 ) ) ;
#24376=EDGE_LOOP ( 'NONE', ( #8826, #12180 ) ) ;
#24380=LINE ( 'NONE', #13806, #6866 ) ;
#24381=CARTESIAN_POINT ( 'NONE',  ( -51.99406906667273631, 13.88268392809765572, -9.019565312798222934 ) ) ;
#24385=CARTESIAN_POINT ( 'NONE',  ( -27.04746142609647208, 8.911459164085380635, -90.41129225940227343 ) ) ;
#24386=CARTESIAN_POINT ( 'NONE',  ( 212.1956890233897752, 119.0847181231351470, 90.11100298095867345 ) ) ;
#24387=ADVANCED_FACE ( 'NONE', ( #9964 ), #43330, .F. ) ;
#24389=CARTESIAN_POINT ( 'NONE',  ( -75.43044859198181484, 21.11535168543635876, -62.68972544619923326 ) ) ;
#24390=CARTESIAN_POINT ( 'NONE',  ( -11.57808265946729875, 7.164483090579920166, 31.11728607544860381 ) ) ;
#24396=B_SPLINE_CURVE_WITH_KNOTS ( 'NONE', 3,
 ( #62125, #35057, #25210, #67419, #13262, #46988, #41024, #46641, #67768, #57206, #19922, #30824, #67092, #56865, #19214, #51920, #68117, #40670, #41378, #45608, #34723, #56502, #14298, #8684, #40329, #62481, #8333, #25555, #62833, #14634, #18533, #50882, #39985, #56161, #29430, #37121, #59259, #58563 ),
 .UNSPECIFIED., .F., .F.,
 ( 4, 2, 2, 2, 2, 2, 2, 2, 2, 2, 2, 2, 2, 2, 2, 2, 2, 2, 4 ),
 ( 0.02546424207107603199, 0.02703543426729210220, 0.02782103036540017199, 0.02860662646350824179, 0.03017781865972445424, 0.03174901085594066669, 0.03332020305215688261, 0.03489139524837309159, 0.03646258744458930751, 0.03724818354269739118, 0.03803377964080548179, 0.03881937573891357240, 0.03960497183702166302, 0.04117616403323783036, 0.04274735622945401159, 0.04431854842567018588, 0.04588974062188636016, 0.04746093281810253445, 0.05060331721053489690 ),
 .UNSPECIFIED. ) ;
#24398=CARTESIAN_POINT ( 'NONE',  ( 187.5165082312810227, 86.85340440641661530, -74.43517852492631448 ) ) ;
#24399=CARTESIAN_POINT ( 'NONE',  ( -165.6215009671260816, 80.58889799860443759, 38.63580300477691765 ) ) ;
#24402=CARTESIAN_POINT ( 'NONE',  ( -24.60892750534350171, 9.584951112520226246, 7.763877395040260865 ) ) ;
#24404=CARTESIAN_POINT ( 'NONE',  ( 11.82929895397813524, 7.412564870773604930, -49.39369728624853195 ) ) ;
#24405=CARTESIAN_POINT ( 'NONE',  ( 126.3737790127712515, 37.08609730334947585, -42.95235691801180167 ) ) ;
#24409=CARTESIAN_POINT ( 'NONE',  ( -8.314575874103551811, 6.922894809783095127, 3.271030448983516692 ) ) ;
#24413=ADVANCED_FACE ( 'NONE', ( #38066 ), #63775, .F. ) ;
#24414=CARTESIAN_POINT ( 'NONE',  ( 9.290502160020464473, 6.379616279862540651, 6.916542375528051956 ) ) ;
#24418=CARTESIAN_POINT ( 'NONE',  ( -62.06231780744543869, 17.72446026058425517, -66.88159662817442097 ) ) ;
#24421=CARTESIAN_POINT ( 'NONE',  ( -178.2381786520593892, 93.01028335822118720, -36.72343023615520963 ) ) ;
#24423=CARTESIAN_POINT ( 'NONE',  ( 8.000000000000007105, 249.8719672152120381, 94.99999999999866418 ) ) ;
#24425=CARTESIAN_POINT ( 'NONE',  ( -48.32993240732259466, 12.98137013984324817, 68.02384498338118135 ) ) ;
#24428=CARTESIAN_POINT ( 'NONE',  ( -0.5751131641471390887, 6.527254166626920373, 66.39501694792768660 ) ) ;
#24434=CARTESIAN_POINT ( 'NONE',  ( -50.14771795543004629, 13.42081263859818030, -48.41097516278959034 ) ) ;
#24445=CARTESIAN_POINT ( 'NONE',  ( 149.9714610887121466, 53.28792066194168342, 36.60205868149071762 ) ) ;
#24449=CARTESIAN_POINT ( 'NONE',  ( -180.6009936245623635, 95.85948119829090786, 12.10851691733632407 ) ) ;
#24450=CARTESIAN_POINT ( 'NONE',  ( -4.504169684898447379, 6.697401007565304099, 17.50005462738863926 ) ) ;
#24451=CARTESIAN_POINT ( 'NONE',  ( 55.99998955208978657, 12.18058389017405396, -40.55750410589438104 ) ) ;
#24452=CARTESIAN_POINT ( 'NONE',  ( -85.73740570227381852, 26.23277384689409431, 35.40511533989044324 ) ) ;
#24453=CARTESIAN_POINT ( 'NONE',  ( 156.0703099390621276, 56.57038975554689131, 83.22409554701557965 ) ) ;
#24454=CARTESIAN_POINT ( 'NONE',  ( 138.2204650371259333, 44.12203217345473405, 16.28412638663770196 ) ) ;
#24455=EDGE_CURVE ( 'NONE', #62594, #40284, #69385, .T. ) ;
#24458=EDGE_CURVE ( 'NONE', #56740, #35856, #63659, .T. ) ;
#24459=LINE ( 'NONE', #60339, #8953 ) ;
#24460=CARTESIAN_POINT ( 'NONE',  ( 43.14712943604300932, 8.926114770663666320, -36.61723071961753817 ) ) ;
#24462=DIRECTION ( 'NONE',  ( -0.000000000000000000, 1.000000000000000000, -0.000000000000000000 ) ) ;
#24465=EDGE_LOOP ( 'NONE', ( #15103, #38057 ) ) ;
#24466=CARTESIAN_POINT ( 'NONE',  ( -143.3925773749112409, 59.16144459815140522, 69.41541250540224439 ) ) ;
#24468=CARTESIAN_POINT ( 'NONE',  ( 82.12277968641507186, 18.98848723477812683, 43.22702714516130840 ) ) ;
#24471=CARTESIAN_POINT ( 'NONE',  ( 182.7789203043889188, 80.33475476315291530, -9.562155104270011918 ) ) ;
#24474=CARTESIAN_POINT ( 'NONE',  ( -120.4816138481825050, 43.03185659245511374, 59.74961932001716747 ) ) ;
#24476=CARTESIAN_POINT ( 'NONE',  ( -79.61235761536670452, 23.76245710489567742, -23.22627702482678913 ) ) ;
#24477=CARTESIAN_POINT ( 'NONE',  ( -180.5234362879040191, 97.35934147644938719, -14.11989895273327456 ) ) ;
#24478=CARTESIAN_POINT ( 'NONE',  ( -47.61402178322637724, 13.84598486314981791, 36.82852865596623104 ) ) ;
#24484=CARTESIAN_POINT ( 'NONE',  ( 104.3931729003987243, 26.26823401847089912, 68.67546489303082069 ) ) ;
#24487=DIRECTION ( 'NONE',  ( 0.000000000000000000, 0.000000000000000000, 1.000000000000000000 ) ) ;
#24491=CARTESIAN_POINT ( 'NONE',  ( -142.0273276822220794, 59.36478176800545725, 91.25952348669476066 ) ) ;
#24492=ORIENTED_EDGE ( 'NONE', *, *, #12873, .F. ) ;
#24498=CARTESIAN_POINT ( 'NONE',  ( 68.45098769362918745, 13.99935947269948500, -48.39431334976815435 ) ) ;
#24500=CARTESIAN_POINT ( 'NONE',  ( -61.53550548562873246, 17.56596194025584978, 41.62090751969812885 ) ) ;
#24502=EDGE_CURVE ( 'NONE', #46532, #39310, #55995, .T. ) ;
#24504=CARTESIAN_POINT ( 'NONE',  ( 35.65685430025424552, 7.951642554322393863, 70.77480580695264223 ) ) ;
#24506=VERTEX_POINT ( 'NONE', #60219 ) ;
#24510=EDGE_CURVE ( 'NONE', #14354, #22557, #24185, .T. ) ;
#24512=CARTESIAN_POINT ( 'NONE',  ( 126.3541873520043737, 37.07520218256170352, -17.17827544387097305 ) ) ;
#24513=CARTESIAN_POINT ( 'NONE',  ( 23.28809538736928531, 7.864824219997530008, -15.68220158935621988 ) ) ;
#24514=CARTESIAN_POINT ( 'NONE',  ( -109.3432140528234839, 36.51591785955879743, -66.78469379273217044 ) ) ;
#24515=B_SPLINE_CURVE_WITH_KNOTS ( 'NONE', 3,
 ( #67426, #52274, #62133, #9368, #13952, #35409, #56874, #51927, #3740, #14643, #30830, #26238, #5800, #42743, #52611, #5462, #31183, #43431, #58919, #57898, #37464, #64909, #64202, #5115, #47671, #10736, #26578, #58571, #69126, #69477, #178, #48015, #10385, #16013, #47327, #25897, #20956, #68785, #31857, #32208, #16703, #15679, #26918 ),
 .UNSPECIFIED., .F., .F.,
 ( 4, 2, 2, 2, 2, 2, 2, 2, 2, 2, 2, 2, 1, 2, 2, 2, 2, 2, 2, 2, 2, 4 ),
 ( 0.02362927190606132349, 0.02510248541563191507, 0.02583909217041720913, 0.02657569892520249971, 0.02804891243477307741, 0.02952212594434365511, 0.03025873269912894223, 0.03099533945391422934, 0.03246855296348480358, 0.03394176647305537087, 0.03541497998262594510, 0.03615158673741123568, 0.03688819349219652627, 0.03762480024698181685, 0.03836140700176710744, 0.03983462051133769555, 0.04130783402090827672, 0.04278104753047885789, 0.04351765428526415541, 0.04425426104004945294, 0.04572747454962003411, 0.04720068805919061528 ),
 .UNSPECIFIED. ) ;
#24523=CARTESIAN_POINT ( 'NONE',  ( 126.3732561463888402, 38.23795180971325891, 9.601229107663494133 ) ) ;
#24531=CARTESIAN_POINT ( 'NONE',  ( 131.6115093721025175, 41.25402743071403933, -77.52764994514272701 ) ) ;
#24534=B_SPLINE_CURVE_WITH_KNOTS ( 'NONE', 3,
 ( #12824, #35309, #66640, #2961, #18094, #34636, #30376, #18437, #24421, #51827, #45863, #56768, #34278, #67335, #40928, #19123, #40577, #55727, #62032, #62388, #13170, #35660, #3637, #25112, #66307, #64108, #52845, #14543, #68688, #46544, #10285, #36346, #4667, #57454, #37034, #20502, #57798, #20164, #5367, #41280, #63075, #9266, #31751, #15919, #31080, #62739 ),
 .UNSPECIFIED., .F., .F.,
 ( 4, 2, 2, 2, 2, 2, 2, 2, 2, 2, 2, 2, 2, 2, 2, 2, 2, 2, 2, 2, 2, 2, 4 ),
 ( 0.000000000000000000, 0.003736383952885418379, 0.005604575929328127135, 0.007472767905770836758, 0.008406863893992191569, 0.009340959882213546381, 0.01120915185865624039, 0.01214324784687757092, 0.01307734383509889971, 0.01401143982332023023, 0.01494553581154155902, 0.01587963179976289302, 0.01681372778798422354, 0.01774782377620555407, 0.01868191976442688459, 0.01961601575264821859, 0.02055011174086954912, 0.02148420772909087964, 0.02241830371731221017, 0.02428649569375488856, 0.02615468767019756696, 0.02802287964664024883, 0.02989107162308292723 ),
 .UNSPECIFIED. ) ;
#24535=CARTESIAN_POINT ( 'NONE',  ( -154.0716379918897019, 69.49957566103795159, 32.25060227376270205 ) ) ;
#24541=CARTESIAN_POINT ( 'NONE',  ( 56.66438910147191166, 11.28870326331392882, 33.31645525201592051 ) ) ;
#24542=EDGE_LOOP ( 'NONE', ( #10181, #25657, #68460, #884 ) ) ;
#24545=CARTESIAN_POINT ( 'NONE',  ( -165.7713056973201731, 80.74264649718246289, 12.99982703628925407 ) ) ;
#24547=FACE_OUTER_BOUND ( 'NONE', #36938, .T. ) ;
#24551=CARTESIAN_POINT ( 'NONE',  ( -71.22896441287284119, 20.69091426169408621, -43.61454751274712294 ) ) ;
#24553=CARTESIAN_POINT ( 'NONE',  ( 174.7644348140981947, 73.82982812962299590, -93.36945622964188374 ) ) ;
#24555=CARTESIAN_POINT ( 'NONE',  ( 140.2200249818744453, 46.60103563593123255, 33.03244647084515861 ) ) ;
#24556=CARTESIAN_POINT ( 'NONE',  ( 116.6681538161788438, 33.09439081574000596, 33.21055421480799197 ) ) ;
#24557=CARTESIAN_POINT ( 'NONE',  ( -127.6894679065405711, 48.89973668460851997, 18.57123567224974536 ) ) ;
#24559=CARTESIAN_POINT ( 'NONE',  ( 66.07923263163412742, 14.44036440557998446, -76.91531762281159956 ) ) ;
#24563=CARTESIAN_POINT ( 'NONE',  ( -147.7925265216585444, 64.04960911618974251, -22.77289545559010264 ) ) ;
#24567=CARTESIAN_POINT ( 'NONE',  ( 46.57905527587767125, 10.47094344121033060, -94.59163972955721533 ) ) ;
#24569=CARTESIAN_POINT ( 'NONE',  ( -145.3279998500303236, 60.71393190715791377, 31.98882707624600030 ) ) ;
#24570=CARTESIAN_POINT ( 'NONE',  ( -120.6739978760426055, 44.33795494230363943, 43.51089096318784044 ) ) ;
#24571=CARTESIAN_POINT ( 'NONE',  ( -167.6413528428656150, 81.22881971256914824, -74.20285492933068383 ) ) ;
#24573=CARTESIAN_POINT ( 'NONE',  ( -108.9145525555662459, 37.42858360505774584, 34.51211213987539850 ) ) ;
#24576=CARTESIAN_POINT ( 'NONE',  ( -38.69577193929646342, 10.89562623693159615, 8.913580037696034353 ) ) ;
#24578=ORIENTED_EDGE ( 'NONE', *, *, #24455, .F. ) ;
#24580=CARTESIAN_POINT ( 'NONE',  ( -189.5325095384513077, 107.4952257375067290, -66.82603086747147358 ) ) ;
#24583=CARTESIAN_POINT ( 'NONE',  ( 32.15641333221390852, 7.577415570152256308, 12.52186555248743538 ) ) ;
#24584=CARTESIAN_POINT ( 'NONE',  ( -14.92860730136983882, 8.468845235798745819, -45.33787050070434788 ) ) ;
#24586=EDGE_CURVE ( 'NONE', #5113, #34356, #53542, .T. ) ;
#24588=B_SPLINE_CURVE_WITH_KNOTS ( 'NONE', 3,
 ( #28615, #50415, #18399, #39514, #34933, #51796, #68329, #57079, #4634, #63037, #46163, #68990, #62705, #67637, #51458, #14506 ),
 .UNSPECIFIED., .F., .F.,
 ( 4, 2, 2, 2, 2, 2, 2, 4 ),
 ( 0.000000000000000000, 0.001318014594730357791, 0.002636029189460715582, 0.003954043784191073156, 0.005272058378921431164, 0.006590072973651789172, 0.007908087568382146312, 0.01054411675784286233 ),
 .UNSPECIFIED. ) ;
#24589=CARTESIAN_POINT ( 'NONE',  ( -107.3439416623322842, 35.42826784730606704, -90.65402495570906183 ) ) ;
#24590=VERTEX_POINT ( 'NONE', #26993 ) ;
#24591=LINE ( 'NONE', #3810, #65410 ) ;
#24595=ORIENTED_EDGE ( 'NONE', *, *, #67074, .F. ) ;
#24597=CARTESIAN_POINT ( 'NONE',  ( -15.13254930056756287, 7.477527548005406643, -68.05477072695896368 ) ) ;
#24598=CARTESIAN_POINT ( 'NONE',  ( -35.17686701826947626, 10.23452050416468317, 44.23696391509336934 ) ) ;
#24599=CARTESIAN_POINT ( 'NONE',  ( -29.49620345460275317, 9.280093073089043187, 71.82164555316683163 ) ) ;
#24603=CARTESIAN_POINT ( 'NONE',  ( -119.1795380581000074, 42.22910606512925114, 34.76803934698340015 ) ) ;
#24604=CARTESIAN_POINT ( 'NONE',  ( -58.32860549785898030, 15.58423118879329294, -49.46749250328178960 ) ) ;
#24606=CARTESIAN_POINT ( 'NONE',  ( -177.5288247523079121, 93.72924674643513754, -62.97066215026593738 ) ) ;
#24607=CARTESIAN_POINT ( 'NONE',  ( 92.19920907511534836, 21.39700525884449434, 59.01058764121106748 ) ) ;
#24612=CARTESIAN_POINT ( 'NONE',  ( 197.9847015768255289, 97.56951352050452897, 40.06412533389060115 ) ) ;
#24614=CARTESIAN_POINT ( 'NONE',  ( 70.25990036603479894, 14.47042233282420298, 66.11517460769501042 ) ) ;
#24615=CARTESIAN_POINT ( 'NONE',  ( 187.4018290418642039, 85.23542003817890134, -93.36671599347617700 ) ) ;
#24617=EDGE_LOOP ( 'NONE', ( #13870, #22244, #7334 ) ) ;
#24619=CARTESIAN_POINT ( 'NONE',  ( 160.9097745014958036, 61.67033591969550343, -10.11087558020973987 ) ) ;
#24621=CARTESIAN_POINT ( 'NONE',  ( 70.12389542974192125, 15.47520081968151651, 61.71442529660797049 ) ) ;
#24623=CARTESIAN_POINT ( 'NONE',  ( 128.4441453432628180, 38.25093000060704895, 85.49679608215056703 ) ) ;
#24628=CARTESIAN_POINT ( 'NONE',  ( -143.8566410313463564, 59.53044870492033880, -64.19978731914612524 ) ) ;
#24632=B_SPLINE_CURVE_WITH_KNOTS ( 'NONE', 3,
 ( #53333, #21336, #36838, #9415, #64252, #4812, #25605, #36490, #58277, #41767, #30872, #16060, #52654, #26626, #9761, #42449, #48061, #47039, #52315, #10098, #31553, #63907, #69515, #14680, #63224, #47716, #42783, #52991, #37513, #15377, #36146, #4138, #20647, #63566, #20302, #15032, #10432, #42108, #57940, #4479, #15721, #25937, #68824, #21003, #37170 ),
 .UNSPECIFIED., .F., .F.,
 ( 4, 2, 2, 2, 2, 2, 2, 2, 2, 2, 2, 1, 2, 2, 2, 2, 2, 2, 2, 2, 2, 2, 4 ),
 ( 0.000000000000000000, 0.001512548138464682055, 0.002268822207697023408, 0.003025096276929364111, 0.004537644415394017326, 0.005293918484626359763, 0.006050192553858700466, 0.007562740692323367993, 0.009075288830788034652, 0.01058783696925270218, 0.01134411103848502640, 0.01210038510771735062, 0.01285665917694967485, 0.01361293324618199907, 0.01512548138464661802, 0.01588175545387892837, 0.01663802952311123351, 0.01815057766157585420, 0.01966312580004047489, 0.02041939986927278697, 0.02117567393850509905, 0.02268822207696975790, 0.02420077021543442022 ),
 .UNSPECIFIED. ) ;
#24633=CARTESIAN_POINT ( 'NONE',  ( -97.88021438939455265, 31.71889184683105611, 17.26694248044579538 ) ) ;
#24637=CARTESIAN_POINT ( 'NONE',  ( 83.38619203015947789, 19.39783821526630447, -23.25651540956177499 ) ) ;
#24638=CARTESIAN_POINT ( 'NONE',  ( -177.2783414347497626, 93.43285667108899872, -89.65509825100188834 ) ) ;
#24639=CARTESIAN_POINT ( 'NONE',  ( 150.5550643769628891, 52.46819381604269239, 60.83852809269659190 ) ) ;
#24642=ORIENTED_EDGE ( 'NONE', *, *, #59778, .T. ) ;
#24643=CARTESIAN_POINT ( 'NONE',  ( -95.20053778133913625, 30.43887292928078026, 62.33583445852484317 ) ) ;
#24644=DIRECTION ( 'NONE',  ( -0.000000000000000000, 1.000000000000000000, -0.000000000000000000 ) ) ;
#24646=ORIENTED_EDGE ( 'NONE', *, *, #58575, .T. ) ;
#24647=CARTESIAN_POINT ( 'NONE',  ( 155.2870855780214470, 57.23765125306420032, -9.590301590278679456 ) ) ;
#24648=CARTESIAN_POINT ( 'NONE',  ( 210.6592759200688079, 116.7161312026394171, -12.42314136530470670 ) ) ;
#24649=CARTESIAN_POINT ( 'NONE',  ( -4.072522659361689890, 7.683023425615342461, 31.11739723680042857 ) ) ;
#24651=CARTESIAN_POINT ( 'NONE',  ( -54.57280099357648595, 14.55288945003961310, -77.06087458892361042 ) ) ;
#24652=CARTESIAN_POINT ( 'NONE',  ( -1.096061481932294024, 7.553048580900440179, -19.39417165875558879 ) ) ;
#24653=CARTESIAN_POINT ( 'NONE',  ( 180.2473887773227545, 77.76029175826238315, 17.46404351504774510 ) ) ;
#24658=CARTESIAN_POINT ( 'NONE',  ( 110.2429982417149574, 29.99119854320846201, -50.92243756565370916 ) ) ;
#24662=CARTESIAN_POINT ( 'NONE',  ( 18.43272992546528144, 7.606837839440253823, 44.53733308803361979 ) ) ;
#24664=CARTESIAN_POINT ( 'NONE',  ( -109.6657532478350845, 37.84376708859253569, -17.00084428919926438 ) ) ;
#24669=EDGE_CURVE ( 'NONE', #44993, #32175, #5359, .T. ) ;
#24674=CARTESIAN_POINT ( 'NONE',  ( 104.7227067006896277, 27.50728936118536438, 58.85534883732941580 ) ) ;
#24675=LINE ( 'NONE', #34546, #54322 ) ;
#24676=VECTOR ( 'NONE', #15188, 1000.000000000000000 ) ;
#24677=CARTESIAN_POINT ( 'NONE',  ( 56.29445224195348629, 12.24017809212662122, -19.74059151869303719 ) ) ;
#24678=ORIENTED_EDGE ( 'NONE', *, *, #46371, .F. ) ;
#24681=ORIENTED_EDGE ( 'NONE', *, *, #25906, .T. ) ;
#24682=CARTESIAN_POINT ( 'NONE',  ( 206.6955592216989714, 109.1214665502617862, 2.622639889806200220 ) ) ;
#24684=CARTESIAN_POINT ( 'NONE',  ( 212.0047492081759799, 116.9348962082588059, 34.98673273882808132 ) ) ;
#24685=FACE_BOUND ( 'NONE', #14141, .T. ) ;
#24686=EDGE_LOOP ( 'NONE', ( #64659, #46445, #40296, #10701 ) ) ;
#24689=CARTESIAN_POINT ( 'NONE',  ( -118.4108695702138618, 42.93846248464117821, 92.41764988183072660 ) ) ;
#24694=CARTESIAN_POINT ( 'NONE',  ( 84.27368848767926579, 18.63026910897604083, -77.30289597407090696 ) ) ;
#24703=CARTESIAN_POINT ( 'NONE',  ( -79.14127775978546708, 22.50259208414362533, -76.96000122218161721 ) ) ;
#24709=EDGE_LOOP ( 'NONE', ( #45756, #38260 ) ) ;
#24710=CARTESIAN_POINT ( 'NONE',  ( 46.51377856795992471, 10.46037936279324221, 66.68987646718457540 ) ) ;
#24713=CARTESIAN_POINT ( 'NONE',  ( 17.72992212664810907, 6.570588738776103277, 3.421689050534150844 ) ) ;
#24718=EDGE_CURVE ( 'NONE', #59217, #889, #9609, .T. ) ;
#24719=CARTESIAN_POINT ( 'NONE',  ( 116.1021807117071916, 31.68810634233424395, -11.86957610067093860 ) ) ;
#24722=EDGE_LOOP ( 'NONE', ( #66709, #20208, #56368, #67953 ) ) ;
#24726=CARTESIAN_POINT ( 'NONE',  ( -175.7347375270319105, 91.62140458887586192, 84.96244202411565993 ) ) ;
#24729=CARTESIAN_POINT ( 'NONE',  ( 130.7531879853686405, 39.58149302537893988, 17.00924939245568623 ) ) ;
#24731=CARTESIAN_POINT ( 'NONE',  ( 199.2613222657365668, 100.8067368203101069, 85.21932682755294763 ) ) ;
#24732=CARTESIAN_POINT ( 'NONE',  ( 212.0104729185451049, 118.7959000526602864, 38.40396052458186205 ) ) ;
#24733=CARTESIAN_POINT ( 'NONE',  ( -75.00168449119588843, 20.95943092127967589, -62.91188405899502101 ) ) ;
#24736=CARTESIAN_POINT ( 'NONE',  ( 9.045716588192245666, 7.384596431530732197, -12.85322072703573859 ) ) ;
#24738=CARTESIAN_POINT ( 'NONE',  ( 201.9869293910475676, 102.6997661182766990, -9.976692069364466064 ) ) ;
#24740=CARTESIAN_POINT ( 'NONE',  ( -143.3980294393559234, 60.45217072626395094, 7.018557309704483771 ) ) ;
#24741=CARTESIAN_POINT ( 'NONE',  ( 187.5246323291926842, 86.86207184872515086, -66.68771993737131254 ) ) ;
#24742=CARTESIAN_POINT ( 'NONE',  ( -146.5309471467636229, 62.99917515507672050, 71.95316401501160897 ) ) ;
#24745=CARTESIAN_POINT ( 'NONE',  ( 35.44781468922821688, 7.928097401423690016, -49.49746209005169106 ) ) ;
#24748=CARTESIAN_POINT ( 'NONE',  ( 127.4750938923429544, 37.70245908594341699, -47.47187847537448135 ) ) ;
#24750=ORIENTED_EDGE ( 'NONE', *, *, #28646, .T. ) ;
#24751=CARTESIAN_POINT ( 'NONE',  ( 187.7216195934903169, 87.07953284547519957, 86.98655473364385671 ) ) ;
#24756=CARTESIAN_POINT ( 'NONE',  ( 14.80582440982707482, 6.470883766728820596, 18.12156665253656840 ) ) ;
#24759=CARTESIAN_POINT ( 'NONE',  ( 205.5130322755755401, 109.1888880665735684, 17.36317014830577676 ) ) ;
#24763=CARTESIAN_POINT ( 'NONE',  ( -24.32471770265757627, 9.546495606312140225, 62.13629395109772702 ) ) ;
#24765=CARTESIAN_POINT ( 'NONE',  ( -48.56549579811110817, 13.03742088415615541, 68.45772509223345992 ) ) ;
#24766=CARTESIAN_POINT ( 'NONE',  ( -7.825402957745083654, 6.891034867348165172, 56.96013162991089018 ) ) ;
#24767=ORIENTED_EDGE ( 'NONE', *, *, #61159, .F. ) ;
#24771=CARTESIAN_POINT ( 'NONE',  ( -52.45215874217870322, 13.99961488531757503, -49.75515071437175862 ) ) ;
#24773=VECTOR ( 'NONE', #66335, 1000.000000000000000 ) ;
#24779=ORIENTED_EDGE ( 'NONE', *, *, #17928, .F. ) ;
#24780=ORIENTED_EDGE ( 'NONE', *, *, #43666, .F. ) ;
#24782=CYLINDRICAL_SURFACE ( 'NONE', #62488, 7.500000000000020428 ) ;
#24783=CARTESIAN_POINT ( 'NONE',  ( 15.78827728214693060, 7.507518794609574719, -8.674393508222097537 ) ) ;
#24786=CARTESIAN_POINT ( 'NONE',  ( -55.05276343752910151, -170.0000000000000000, 91.50642895385851716 ) ) ;
#24787=LINE ( 'NONE', #19495, #62295 ) ;
#24790=CARTESIAN_POINT ( 'NONE',  ( 62.05396267233469132, 13.48332220860126540, -50.67464569965138566 ) ) ;
#24793=CARTESIAN_POINT ( 'NONE',  ( 140.4586216751744985, 45.55624550472995793, 6.597895794798392721 ) ) ;
#24795=CARTESIAN_POINT ( 'NONE',  ( 110.7164744784863757, 29.10110206241301611, -35.92243756565368784 ) ) ;
#24796=CARTESIAN_POINT ( 'NONE',  ( 10.83418588031599583, 6.392467435475929882, 58.70663493700131852 ) ) ;
#24797=ADVANCED_FACE ( 'NONE', ( #15673 ), #8685, .F. ) ;
#24798=CARTESIAN_POINT ( 'NONE',  ( 46.41758729921144777, 9.425975226414236019, -45.78279639359242026 ) ) ;
#24799=CARTESIAN_POINT ( 'NONE',  ( -77.48202330058325060, 22.94882077088976047, 84.19497686350740651 ) ) ;
#24801=VERTEX_POINT ( 'NONE', #42404 ) ;
#24807=CARTESIAN_POINT ( 'NONE',  ( -146.1142527948576060, 61.35394402951021675, 71.75774863290075700 ) ) ;
#24809=CARTESIAN_POINT ( 'NONE',  ( 197.1980152960109649, 96.59350208824301376, -70.33315983686533457 ) ) ;
#24812=CARTESIAN_POINT ( 'NONE',  ( -78.66644367742111399, 23.39876645725285798, -8.270900041254197532 ) ) ;
#24813=CARTESIAN_POINT ( 'NONE',  ( -176.3856149167965839, 92.38076834121986280, -8.600915367064782657 ) ) ;
#24814=CARTESIAN_POINT ( 'NONE',  ( -153.1121305730337383, 67.29834700374527756, -35.73192746080628268 ) ) ;
#24818=CARTESIAN_POINT ( 'NONE',  ( 102.8458551240039895, 25.60773946375957166, 62.69125674198833309 ) ) ;
#24819=CARTESIAN_POINT ( 'NONE',  ( 163.1265310614426767, 62.18610413911353874, 58.82269949688948429 ) ) ;
#24820=DIRECTION ( 'NONE',  ( -0.000000000000000000, 1.000000000000000000, -0.000000000000000000 ) ) ;
#24823=CARTESIAN_POINT ( 'NONE',  ( -31.43908319763710679, 9.591432048623762086, 72.06100499665289760 ) ) ;
#24827=CARTESIAN_POINT ( 'NONE',  ( -152.9008427825210958, 68.45483453645054794, -22.16050399148043226 ) ) ;
#24828=CARTESIAN_POINT ( 'NONE',  ( 39.40195752203892710, 9.424259417798134919, -50.61981746542779348 ) ) ;
#24829=CYLINDRICAL_SURFACE ( 'NONE', #69088, 7.500000000000013323 ) ;
#24830=CARTESIAN_POINT ( 'NONE',  ( 109.4667359685670078, 28.52415501392344410, -89.64184605405843342 ) ) ;
#24831=CARTESIAN_POINT ( 'NONE',  ( -57.89360549284270974, 16.50663738101750511, 44.77101158031961603 ) ) ;
#24833=CARTESIAN_POINT ( 'NONE',  ( -38.80621507254812741, 11.94263265896524473, -68.19319284720511121 ) ) ;
#24835=CARTESIAN_POINT ( 'NONE',  ( 11.21653854975268771, 6.397128675385706842, -10.20870010705862363 ) ) ;
#24837=B_SPLINE_CURVE_WITH_KNOTS ( 'NONE', 3,
 ( #63873, #10741, #5467, #36109, #20604, #10390, #10058, #57902, #63186, #42748, #48349, #9724, #36800, #21638, #182, #42066, #14988, #57563, #63526, #43092, #15342, #58242, #48019, #25564, #4774, #69480, #37472, #68462, #16019, #21300, #26922, #47002, #31518, #31186, #20267, #4102, #52952, #47674, #58923, #69132 ),
 .UNSPECIFIED., .F., .F.,
 ( 4, 2, 2, 2, 2, 2, 2, 2, 2, 2, 2, 2, 2, 2, 2, 2, 2, 2, 2, 4 ),
 ( 0.02454308262168998500, 0.02608670964102876785, 0.02685852315069817489, 0.02763033666036758540, 0.02917396367970639948, 0.02994577718937580652, 0.03071759069904521355, 0.03226121771838405539, 0.03303303122805349712, 0.03380484473772293885, 0.03534847175706178762, 0.03689209877640063640, 0.03843572579573948517, 0.03997935281507833394, 0.04152297983441718271, 0.04306660685375603148, 0.04461023387309488025, 0.04615386089243372902, 0.04769748791177257780, 0.04924111493111142657 ),
 .UNSPECIFIED. ) ;
#24840=CARTESIAN_POINT ( 'NONE',  ( -3.868882431147343315, 6.665575841812209745, -49.29435056024676953 ) ) ;
#24842=CARTESIAN_POINT ( 'NONE',  ( -121.5677746760273408, 43.71038933438990881, 17.42027109748232050 ) ) ;
#24843=CARTESIAN_POINT ( 'NONE',  ( 67.93926590385571274, 13.86859831467923954, -64.38660125305884208 ) ) ;
#24846=CARTESIAN_POINT ( 'NONE',  ( 197.3707490726349647, 96.80690576410100334, 65.18469054512721073 ) ) ;
#24849=ORIENTED_EDGE ( 'NONE', *, *, #46345, .F. ) ;
#24855=CARTESIAN_POINT ( 'NONE',  ( 186.0827296088607170, 85.28826835108066007, -38.12883777694066367 ) ) ;
#24857=ORIENTED_EDGE ( 'NONE', *, *, #17966, .F. ) ;
#24858=EDGE_CURVE ( 'NONE', #15369, #49352, #63177, .T. ) ;
#24863=CARTESIAN_POINT ( 'NONE',  ( 164.9799824490939670, 65.05186898783672689, 90.53880561405300398 ) ) ;
#24866=CARTESIAN_POINT ( 'NONE',  ( -57.43883374585515611, 16.37892664338858495, 18.08720956373479893 ) ) ;
#24867=CARTESIAN_POINT ( 'NONE',  ( 128.4224537826254107, 38.23837035195747092, 42.20221012506080172 ) ) ;
#24871=CARTESIAN_POINT ( 'NONE',  ( -102.2801239173131052, 32.78103895658057354, 30.51907450641510522 ) ) ;
#24875=CARTESIAN_POINT ( 'NONE',  ( 60.63507185982728487, 12.13307030573223599, 44.42928727059375404 ) ) ;
#24878=( BOUNDED_CURVE ( )  B_SPLINE_CURVE ( 3, ( #60199, #12020, #60551, #1119 ),
 .UNSPECIFIED., .F., .F. ) 
 B_SPLINE_CURVE_WITH_KNOTS ( ( 4, 4 ),
 ( 2.506209174768083692, 3.776976132411494103 ),
 .UNSPECIFIED. ) 
 CURVE ( )  GEOMETRIC_REPRESENTATION_ITEM ( )  RATIONAL_B_SPLINE_CURVE ( ( 1.000000000000000000, 0.8698961108463045822, 0.8698961108463045822, 1.000000000000000000 ) ) 
 REPRESENTATION_ITEM ( '' )  );
#24879=CARTESIAN_POINT ( 'NONE',  ( 174.1348882614952061, 73.23561817543357222, 39.64404733447431539 ) ) ;
#24881=CARTESIAN_POINT ( 'NONE',  ( 21.25987915030396636, 6.737472588634913606, -74.99879528645634252 ) ) ;
#24883=EDGE_LOOP ( 'NONE', ( #42467, #17899 ) ) ;
#24884=CARTESIAN_POINT ( 'NONE',  ( -99.98911906681071571, 32.75458865035245992, 84.54173588161988562 ) ) ;
#24886=EDGE_CURVE ( 'NONE', #14210, #55930, #60796, .T. ) ;
#24887=EDGE_CURVE ( 'NONE', #49789, #69259, #65241, .T. ) ;
#24888=CARTESIAN_POINT ( 'NONE',  ( -71.57025115638936086, 20.80908992785613165, -45.09462308011600129 ) ) ;
#24891=CARTESIAN_POINT ( 'NONE',  ( 212.1976655298228422, 119.0878071902807278, -70.84834327812836818 ) ) ;
#24894=CARTESIAN_POINT ( 'NONE',  ( 141.3400002717723396, 47.33399859146519617, 37.57801802895147603 ) ) ;
#24896=CARTESIAN_POINT ( 'NONE',  ( 15.78827728214693416, -170.0000000000000000, -50.51894409868581448 ) ) ;
#24897=CARTESIAN_POINT ( 'NONE',  ( 69.49112875363886133, 15.30845942322119768, -73.85730488686293427 ) ) ;
#24900=CARTESIAN_POINT ( 'NONE',  ( -145.5195986658808351, 62.16746116576787529, -21.82433970153511282 ) ) ;
#24902=CARTESIAN_POINT ( 'NONE',  ( -171.0814041607219451, 84.88598211196838861, -49.44167807983354379 ) ) ;
#24904=CARTESIAN_POINT ( 'NONE',  ( 133.8566784816069344, -170.0000000000000000, -70.36786152285935714 ) ) ;
#24908=CARTESIAN_POINT ( 'NONE',  ( -120.0051930351106364, 43.92079660368833061, 42.77160068737919829 ) ) ;
#24909=CARTESIAN_POINT ( 'NONE',  ( -168.7187482717114051, 82.35796501763488209, -75.14684098565754766 ) ) ;
#24911=CARTESIAN_POINT ( 'NONE',  ( -105.4487797565984124, 35.55724615608637862, 31.20524870816166896 ) ) ;
#24913=CARTESIAN_POINT ( 'NONE',  ( -178.9255766471344771, 93.82953196344688251, -91.12939640909104355 ) ) ;
#24915=CARTESIAN_POINT ( 'NONE',  ( -81.96040367003716653, 23.60340032034881830, -89.55302406663774661 ) ) ;
#24919=B_SPLINE_CURVE_WITH_KNOTS ( 'NONE', 3,
 ( #26409, #43607, #6329, #65077, #47844, #37640, #61195, #12660, #66489, #39389, #40085, #24264, #65788, #60839, #1763, #50629, #34817, #34121, #50295, #23222, #45709, #13018, #55560, #54856, #67187, #28128, #23907, #17585, #7388, #6681, #44672, #18975, #55211, #34478, #40426, #28843, #39051, #55922, #12311, #61869, #7735, #61541, #17936, #56254 ),
 .UNSPECIFIED., .F., .F.,
 ( 4, 2, 2, 2, 2, 2, 2, 2, 2, 2, 2, 2, 2, 2, 2, 2, 2, 2, 2, 2, 2, 4 ),
 ( 0.02638217555535137329, 0.02805347641364857800, 0.02972477727194578270, 0.03139607813024299088, 0.03306737898854019558, 0.03390302941768881528, 0.03473867984683744192, 0.03640998070513468826, 0.03724563113428332184, 0.03808128156343194848, 0.03891693199258058206, 0.03975258242172921563, 0.04058823285087784227, 0.04142388328002646891, 0.04225953370917509555, 0.04309518413832372219, 0.04476648499662096159, 0.04643778585491820099, 0.04810908671321544039, 0.04978038757151267979, 0.05145168842980991225, 0.05312298928810715165 ),
 .UNSPECIFIED. ) ;
#24920=CARTESIAN_POINT ( 'NONE',  ( 32.28603806442400526, 7.590310383548726669, 8.149296409025412302 ) ) ;
#24921=CARTESIAN_POINT ( 'NONE',  ( -13.77312480593389132, 8.361845410302544579, -47.49360053362800471 ) ) ;
#24927=CARTESIAN_POINT ( 'NONE',  ( -56.73868929054667376, 16.18382781951277138, 71.97397694089359277 ) ) ;
#24928=CARTESIAN_POINT ( 'NONE',  ( -24.94151142167917712, 8.614613465433007988, 7.093782003634580668 ) ) ;
#24931=CARTESIAN_POINT ( 'NONE',  ( -59.09409272559887683, 15.80233242102493918, -90.08371057033618001 ) ) ;
#24932=CARTESIAN_POINT ( 'NONE',  ( -38.15923928782687824, 10.79140400702259406, 41.05568229944667991 ) ) ;
#24934=ADVANCED_FACE ( 'NONE', ( #1225 ), #27953, .F. ) ;
#24938=CARTESIAN_POINT ( 'NONE',  ( -121.2008155373973892, 43.48033530165985638, 32.24946013892020602 ) ) ;
#24942=AXIS2_PLACEMENT_3D ( 'NONE', #42262, #41566, #32398 ) ;
#24943=CARTESIAN_POINT ( 'NONE',  ( 133.2949513180626298, 42.25961182073308464, 83.19458329861414825 ) ) ;
#24946=CARTESIAN_POINT ( 'NONE',  ( 116.6457744947906860, 31.95847117670278692, 33.19741688322386608 ) ) ;
#24948=B_SPLINE_CURVE_WITH_KNOTS ( 'NONE', 3,
 ( #37555, #53032, #68865, #10823, #68540, #10475, #42493, #42148, #26323, #5544, #26999, #63610, #20343, #48429, #57645, #15420, #36531, #263, #57985, #41468, #31945, #62922, #69218, #58316, #14722, #9802, #31263, #36186, #53373, #4516, #25979, #47411, #10135, #31592, #21043, #34028, #32631, #54765, #22421, #22075, #38246, #43515, #44210, #65695, #39304 ),
 .UNSPECIFIED., .F., .F.,
 ( 4, 2, 2, 1, 2, 2, 2, 2, 2, 2, 2, 2, 2, 2, 2, 2, 2, 2, 2, 2, 2, 2, 4 ),
 ( 0.02348395315094739533, 0.02495010856601299204, 0.02568318627354579040, 0.02641626398107858528, 0.02714934168861138364, 0.02788241939614417852, 0.02934857481120976483, 0.03008165251874255625, 0.03081473022627535113, 0.03228088564134094091, 0.03301396334887373579, 0.03374704105640652374, 0.03521319647147211351, 0.03667935188653769635, 0.03741242959407048430, 0.03814550730160327918, 0.03961166271666885508, 0.04107781813173443791, 0.04254397354680002075, 0.04327705125433280176, 0.04401012896186559664, 0.04547628437693117254, 0.04694243979199674843 ),
 .UNSPECIFIED. ) ;
#24953=CARTESIAN_POINT ( 'NONE',  ( -118.3927673406137586, 41.74929850983308199, -69.02033445283595370 ) ) ;
#24955=EDGE_CURVE ( 'NONE', #45299, #17268, #10380, .T. ) ;
#24956=ORIENTED_EDGE ( 'NONE', *, *, #60521, .T. ) ;
#24958=CARTESIAN_POINT ( 'NONE',  ( 111.1767565371974769, 29.31586421952252053, -77.72348245422179502 ) ) ;
#24960=CARTESIAN_POINT ( 'NONE',  ( 133.8566784816069060, 42.60093787723653236, 2.665790248531674678 ) ) ;
#24963=ORIENTED_EDGE ( 'NONE', *, *, #24320, .F. ) ;
#24966=CARTESIAN_POINT ( 'NONE',  ( 70.26936813788617542, 15.51386666370914824, 62.18728408539558217 ) ) ;
#24974=CARTESIAN_POINT ( 'NONE',  ( 162.8142581494936110, 61.92799983924231810, -38.34020306277995616 ) ) ;
#24975=ORIENTED_EDGE ( 'NONE', *, *, #62829, .T. ) ;
#24979=CARTESIAN_POINT ( 'NONE',  ( 150.9494776551346149, 53.99791200760193988, -93.60193293775073187 ) ) ;
#24980=FACE_OUTER_BOUND ( 'NONE', #13865, .T. ) ;
#24981=CARTESIAN_POINT ( 'NONE',  ( -167.9889421625799741, 81.59140042431236850, 32.83227558599013207 ) ) ;
#24984=CARTESIAN_POINT ( 'NONE',  ( 92.20490818459941806, 22.47175429302964744, 42.25219620519190755 ) ) ;
#24986=CARTESIAN_POINT ( 'NONE',  ( -102.2801239173131052, 33.91021738430207222, 57.36362509687880618 ) ) ;
#24987=CARTESIAN_POINT ( 'NONE',  ( -15.13211202216340823, 8.488266782358833140, 62.75077677020096445 ) ) ;
#24988=ORIENTED_EDGE ( 'NONE', *, *, #67667, .T. ) ;
#24990=CARTESIAN_POINT ( 'NONE',  ( 157.4703587214989113, 58.92748579479258808, -24.27963370867398396 ) ) ;
#24991=CARTESIAN_POINT ( 'NONE',  ( 212.1913428512247322, 119.0779339498138114, -17.33593461546083603 ) ) ;
#24992=CARTESIAN_POINT ( 'NONE',  ( 103.9685899589048290, 27.18106603025993095, 32.99486883808148008 ) ) ;
#24994=CARTESIAN_POINT ( 'NONE',  ( -6.840165690716691671, 7.836465889224642822, 30.16447760598867944 ) ) ;
#24995=CARTESIAN_POINT ( 'NONE',  ( 60.45761612245340899, 12.09376662961991578, 83.94407422121982165 ) ) ;
#24996=CARTESIAN_POINT ( 'NONE',  ( 187.2296622856351576, 86.53808614709456037, 5.657001796427024942 ) ) ;
#24997=CARTESIAN_POINT ( 'NONE',  ( 212.0047492081760936, 116.9348962082588343, -45.54691903256296115 ) ) ;
#24999=DIRECTION ( 'NONE',  ( 0.000000000000000000, 0.000000000000000000, 1.000000000000000000 ) ) ;
#25000=CARTESIAN_POINT ( 'NONE',  ( -61.52143283897137849, 16.51181063611436528, 7.169046980359220278 ) ) ;
#25003=ORIENTED_EDGE ( 'NONE', *, *, #21072, .F. ) ;
#25007=CARTESIAN_POINT ( 'NONE',  ( -3.544435206134087135, 6.649906604172325153, 85.13781338574963797 ) ) ;
#25010=ORIENTED_EDGE ( 'NONE', *, *, #24955, .T. ) ;
#25014=EDGE_LOOP ( 'NONE', ( #38138, #47832, #43400, #8505 ) ) ;
#25017=CARTESIAN_POINT ( 'NONE',  ( 173.5843421840238534, 71.34465141434344559, -16.57726541804536069 ) ) ;
#25018=CARTESIAN_POINT ( 'NONE',  ( -167.6524579626394598, 82.69702609844092933, 60.02780465990404934 ) ) ;
#25021=CARTESIAN_POINT ( 'NONE',  ( 59.08202327466404569, 12.82375733818951247, -9.985768006214025050 ) ) ;
#25025=CARTESIAN_POINT ( 'NONE',  ( 205.5004956747122264, 107.4493581495447927, 2.395320917533355409 ) ) ;
#25027=CARTESIAN_POINT ( 'NONE',  ( 206.6955592216991420, 109.1214665502618004, 29.46719048026987764 ) ) ;
#25028=CARTESIAN_POINT ( 'NONE',  ( 14.94784401874210822, 6.475021042546637240, -89.24363180946468788 ) ) ;
#25038=CYLINDRICAL_SURFACE ( 'NONE', #15230, 7.500000000000020428 ) ;
#25039=CARTESIAN_POINT ( 'NONE',  ( 22.84965234755525287, 6.829418951222932854, 88.65540587631463154 ) ) ;
#25040=CARTESIAN_POINT ( 'NONE',  ( 82.74007713545064746, 18.13042311233562032, -76.58347899170844642 ) ) ;
#25044=CARTESIAN_POINT ( 'NONE',  ( 197.2847860006354779, 98.30530166401518954, -44.97716114296652989 ) ) ;
#25047=CYLINDRICAL_SURFACE ( 'NONE', #47445, 7.500000000000020428 ) ;
#25049=CARTESIAN_POINT ( 'NONE',  ( -85.90441187606244000, 25.21188850826090899, -67.43018938941865770 ) ) ;
#25051=CIRCLE ( 'NONE', #57679, 242.4895526022646379 ) ;
#25054=VECTOR ( 'NONE', #14935, 1000.000000000000000 ) ;
#25055=VERTEX_POINT ( 'NONE', #24082 ) ;
#25056=CARTESIAN_POINT ( 'NONE',  ( 9.827939172326077610, 6.382931149346553923, -38.43989651470956659 ) ) ;
#25058=CARTESIAN_POINT ( 'NONE',  ( 20.36314374176837561, 6.689939636827347158, 4.706573874584005779 ) ) ;
#25062=CARTESIAN_POINT ( 'NONE',  ( 173.7225111622554721, 72.84868911716897344, -69.10599538675619158 ) ) ;
#25064=CARTESIAN_POINT ( 'NONE',  ( 103.9652201950894721, 26.08439499369982428, -39.31135386676266563 ) ) ;
#25065=CARTESIAN_POINT ( 'NONE',  ( 84.05289558242219528, 19.61733656419350069, -50.36921807815809160 ) ) ;
#25066=CARTESIAN_POINT ( 'NONE',  ( -165.7102224864505615, 80.67993370857061564, -94.71298376253034235 ) ) ;
#25068=VERTEX_POINT ( 'NONE', #1941 ) ;
#25069=CARTESIAN_POINT ( 'NONE',  ( 40.38414441725701209, 8.538832720399536669, 18.02099439841263973 ) ) ;
#25074=CARTESIAN_POINT ( 'NONE',  ( -156.9252506979472912, 70.73559306219775067, 10.23206411029071461 ) ) ;
#25075=CARTESIAN_POINT ( 'NONE',  ( -118.8392474096542486, 43.20060570451231285, -71.85748745244474378 ) ) ;
#25076=CARTESIAN_POINT ( 'NONE',  ( 212.1734186221015932, 119.0499290057855291, 37.39989276221264447 ) ) ;
#25077=CARTESIAN_POINT ( 'NONE',  ( -76.31381168750405664, 21.43908608416557726, -62.32252567794670028 ) ) ;
#25079=DIRECTION ( 'NONE',  ( -0.000000000000000000, 1.000000000000000000, -0.000000000000000000 ) ) ;
#25082=CARTESIAN_POINT ( 'NONE',  ( 12.46490660984525611, 7.423426948220648747, -9.446422529437963789 ) ) ;
#25084=CARTESIAN_POINT ( 'NONE',  ( 197.3707490726349647, 96.80690576410101755, -15.34896122626384596 ) ) ;
#25088=CARTESIAN_POINT ( 'NONE',  ( -142.9843132609582597, 60.12226089556228459, 68.77572048107622038 ) ) ;
#25090=CARTESIAN_POINT ( 'NONE',  ( 204.6977192012829789, 108.0580384837234931, -90.01503221354883522 ) ) ;
#25093=CARTESIAN_POINT ( 'NONE',  ( 12.68603346975294954, 7.427591953486043508, -36.18624911206273254 ) ) ;
#25095=VERTEX_POINT ( 'NONE', #60313 ) ;
#25096=ADVANCED_FACE ( 'NONE', ( #23729 ), #33941, .F. ) ;
#25098=EDGE_CURVE ( 'NONE', #19832, #60092, #18601, .T. ) ;
#25102=EDGE_CURVE ( 'NONE', #18664, #17986, #61700, .T. ) ;
#25110=CARTESIAN_POINT ( 'NONE',  ( 15.78827728214693416, 6.500811158483284835, 56.85925826316891829 ) ) ;
#25111=CARTESIAN_POINT ( 'NONE',  ( 210.5008983495072243, 116.4753531594350733, 14.62071003477614539 ) ) ;
#25112=CARTESIAN_POINT ( 'NONE',  ( -180.5230320745700965, 95.76406004447552789, -43.46080055680893395 ) ) ;
#25113=CARTESIAN_POINT ( 'NONE',  ( 89.22118407503262461, 20.32164250407901207, -9.435028923643752563 ) ) ;
#25114=CARTESIAN_POINT ( 'NONE',  ( -25.48750459758501918, 9.705678256319572483, 59.97090248023433645 ) ) ;
#25116=CARTESIAN_POINT ( 'NONE',  ( -53.38256734720888375, 14.24001356352780689, 57.34620933837434364 ) ) ;
#25117=B_SPLINE_CURVE_WITH_KNOTS ( 'NONE', 3,
 ( #9907, #53132, #53479, #10234, #63716, #69329, #31024, #9559, #31361, #52463, #15528, #26425, #368, #21152, #20442, #5310, #47867, #10576, #36981, #4285, #25748, #21476, #26769, #47178, #4961, #47510, #63371, #42597, #52792, #64049, #15860, #15179, #32397, #42922, #63018, #37307, #68636, #36642, #31697, #4616, #58418, #26080, #41908, #22, #20795, #53822 ),
 .UNSPECIFIED., .F., .F.,
 ( 4, 2, 2, 2, 2, 2, 2, 2, 2, 2, 2, 2, 2, 2, 2, 2, 2, 2, 2, 2, 2, 2, 4 ),
 ( 1.387778780781445676E-17, 0.003736383952885407537, 0.005604575929328104583, 0.007472767905770801196, 0.008406863893992139528, 0.009340959882213476992, 0.01120915185865615366, 0.01214324784687749979, 0.01307734383509884593, 0.01401143982332018860, 0.01494553581154153474, 0.01587963179976283751, 0.01681372778798414028, 0.01774782377620543958, 0.01868191976442676316, 0.01961601575264808675, 0.02055011174086940687, 0.02148420772909072698, 0.02241830371731204710, 0.02428649569375476713, 0.02615468767019748370, 0.02802287964664020026, 0.02989107162308291682 ),
 .UNSPECIFIED. ) ;
#25121=EDGE_CURVE ( 'NONE', #24590, #3542, #2874, .T. ) ;
#25123=CARTESIAN_POINT ( 'NONE',  ( 155.7265855639938650, 57.57443315515123317, 56.44615811012038620 ) ) ;
#25124=CARTESIAN_POINT ( 'NONE',  ( -108.9145525555662743, 37.42858360505778847, -72.86609022197936270 ) ) ;
#25125=CARTESIAN_POINT ( 'NONE',  ( -50.52927270563905182, 13.51486287463704450, -48.71881382000154304 ) ) ;
#25127=CARTESIAN_POINT ( 'NONE',  ( -0.7313957694713866253, 7.539606919072873836, 93.82462488541915491 ) ) ;
#25128=ORIENTED_EDGE ( 'NONE', *, *, #63975, .F. ) ;
#25129=CARTESIAN_POINT ( 'NONE',  ( -190.5273690078732329, 108.8856264335149859, -91.58113276652414925 ) ) ;
#25135=CARTESIAN_POINT ( 'NONE',  ( -180.6011569556095822, 95.85968111394265634, -69.68656036792953046 ) ) ;
#25137=ORIENTED_EDGE ( 'NONE', *, *, #14642, .T. ) ;
#25140=CARTESIAN_POINT ( 'NONE',  ( -5.871577929436022636, 6.771181646175755908, 18.02891427094515464 ) ) ;
#25142=CARTESIAN_POINT ( 'NONE',  ( 57.41085175769453741, 12.46982565415947697, -48.21039516881924669 ) ) ;
#25144=CARTESIAN_POINT ( 'NONE',  ( 152.1847562093922193, 53.65517908050956208, 85.26709633804618704 ) ) ;
#25145=VECTOR ( 'NONE', #53081, 1000.000000000000000 ) ;
#25146=CARTESIAN_POINT ( 'NONE',  ( 137.4117721579687839, 43.61242559081431835, 16.78681578490248327 ) ) ;
#25152=CARTESIAN_POINT ( 'NONE',  ( 8.540853903193189822, 6.376814430361481989, 66.30478470236579369 ) ) ;
#25153=CARTESIAN_POINT ( 'NONE',  ( 202.7540649946182896, 105.3989460363904698, 29.45258215039039484 ) ) ;
#25154=CARTESIAN_POINT ( 'NONE',  ( -71.19449361276183197, 20.67900126374447467, 90.88156997529951298 ) ) ;
#25155=CARTESIAN_POINT ( 'NONE',  ( -118.4669749820149605, 41.79437899234314813, 90.71051623639903028 ) ) ;
#25157=CARTESIAN_POINT ( 'NONE',  ( 64.69738688745242428, 14.10375742873389093, 44.62596110400481564 ) ) ;
#25159=AXIS2_PLACEMENT_3D ( 'NONE', #44364, #65847, #11656 ) ;
#25161=CARTESIAN_POINT ( 'NONE',  ( -144.2029146819478456, 59.80706661873674079, 70.38930589792778392 ) ) ;
#25162=CARTESIAN_POINT ( 'NONE',  ( 217.9999999999999716, 128.6235316737731296, -95.00000000000133582 ) ) ;
#25164=CARTESIAN_POINT ( 'NONE',  ( 15.78827728214693771, 7.507518794609575608, -62.36349468914946925 ) ) ;
#25165=CARTESIAN_POINT ( 'NONE',  ( -122.7930600691577894, 44.48546375740912140, 71.80916449259312628 ) ) ;
#25167=CARTESIAN_POINT ( 'NONE',  ( 21.89475364395364565, 7.780723588097695043, -92.33322761029084802 ) ) ;
#25168=B_SPLINE_CURVE_WITH_KNOTS ( 'NONE', 3,
 ( #50968, #67847, #29167, #13676, #28825, #55900, #18262, #45338, #24598, #8053, #66470, #46030, #35131, #35483, #40750, #24932, #50275, #50616, #29859, #51664, #56587, #61175, #41108, #34462, #8408, #39720, #30213, #46366, #13002, #67497, #29504, #24250, #40068, #7719, #19293, #61523, #19644, #2099, #62207, #56945, #2434, #3471, #23891, #45693 ),
 .UNSPECIFIED., .F., .F.,
 ( 4, 2, 2, 2, 2, 2, 2, 2, 2, 2, 2, 2, 2, 2, 2, 2, 2, 2, 2, 2, 2, 4 ),
 ( 6.938893903907228378E-18, 0.001476829494128773521, 0.002215244241193168630, 0.002953658988257563522, 0.004430488482386362413, 0.005907317976515161738, 0.007384147470643961063, 0.008122562217708370266, 0.008860976964772776868, 0.01033780645890160395, 0.01181463595303043276, 0.01255305070009485324, 0.01329146544715927719, 0.01476829494128812509, 0.01550670968835255251, 0.01624512443541697992, 0.01772195392954586599, 0.01919878342367475205, 0.01993719817073918640, 0.02067561291780362076, 0.02215244241193247213, 0.02362927190606132002 ),
 .UNSPECIFIED. ) ;
#25169=CARTESIAN_POINT ( 'NONE',  ( -47.55256438668344288, 13.83151366677316219, 37.57512454685291914 ) ) ;
#25178=CARTESIAN_POINT ( 'NONE',  ( -145.4282275380300575, 62.09266785189831239, 85.60967048720104344 ) ) ;
#25185=ADVANCED_FACE ( 'NONE', ( #57126 ), #31089, .F. ) ;
#25186=CARTESIAN_POINT ( 'NONE',  ( 174.6519463786725339, 72.34076406854485697, -93.55046425245691921 ) ) ;
#25189=CARTESIAN_POINT ( 'NONE',  ( -58.76099769480629220, 16.75353773354893150, 44.34096742449668938 ) ) ;
#25193=CARTESIAN_POINT ( 'NONE',  ( 33.03621582719333816, 7.666716336587122704, 60.28506365736417649 ) ) ;
#25194=CARTESIAN_POINT ( 'NONE',  ( 46.09004436292335782, 9.373833359422084399, 87.69295583249557069 ) ) ;
#25196=CARTESIAN_POINT ( 'NONE',  ( -4.504169684898453596, 6.697401007565306763, -36.18904655353872357 ) ) ;
#25197=CARTESIAN_POINT ( 'NONE',  ( 186.2651679807462131, 84.00458780104315792, 58.20990309437074472 ) ) ;
#25198=CARTESIAN_POINT ( 'NONE',  ( -124.1033713525885673, 45.32626312604503482, 18.56215417726921757 ) ) ;
#25201=CARTESIAN_POINT ( 'NONE',  ( 17.72992212664810552, 6.570588738776101501, 57.11079023146151457 ) ) ;
#25202=CARTESIAN_POINT ( 'NONE',  ( 22.51798020284707036, 7.817376421459706570, -19.49430492783765700 ) ) ;
#25203=CARTESIAN_POINT ( 'NONE',  ( 201.9777685760379882, 102.6876480786893069, 56.55075970390274875 ) ) ;
#25206=ADVANCED_FACE ( 'NONE', ( #8938 ), #25471, .F. ) ;
#25207=ORIENTED_EDGE ( 'NONE', *, *, #69377, .F. ) ;
#25210=CARTESIAN_POINT ( 'NONE',  ( 132.9557829392754513, 42.05591979570419170, -50.98300341427673743 ) ) ;
#25211=CARTESIAN_POINT ( 'NONE',  ( -126.8005235842505840, 47.09307471149450208, -34.95511893173629403 ) ) ;
#25212=CARTESIAN_POINT ( 'NONE',  ( -105.4642082819536313, 35.56541171990214423, -35.70785606305261695 ) ) ;
#25216=CARTESIAN_POINT ( 'NONE',  ( -149.5074843970971017, 64.17983161892347255, -7.968279941028269420 ) ) ;
#25219=CARTESIAN_POINT ( 'NONE',  ( 164.5010389544228246, 64.64604269109669588, 87.96214707110127051 ) ) ;
#25221=CARTESIAN_POINT ( 'NONE',  ( 126.3554864210862121, 38.22801630372152459, -70.13989239923940033 ) ) ;
#25222=CARTESIAN_POINT ( 'NONE',  ( 133.3996297101684547, 41.14871796345732946, 44.51034083899536142 ) ) ;
#25223=CARTESIAN_POINT ( 'NONE',  ( -149.5074843970971017, 65.50121172469319220, 45.72082123989907387 ) ) ;
#25231=CARTESIAN_POINT ( 'NONE',  ( -166.7136514167008841, 81.71618216218794828, 7.570113361991930745 ) ) ;
#25232=AXIS2_PLACEMENT_3D ( 'NONE', #51953, #25586, #47024 ) ;
#25233=CARTESIAN_POINT ( 'NONE',  ( 204.6977192012829789, -170.0000000000000000, -70.67048162308527992 ) ) ;
#25234=CARTESIAN_POINT ( 'NONE',  ( -132.0738857626834033, 51.93126104279147626, 60.70775882567303228 ) ) ;
#25236=CARTESIAN_POINT ( 'NONE',  ( -102.9275459269102129, 34.24179444430608044, 84.23033673724052051 ) ) ;
#25240=EDGE_CURVE ( 'NONE', #12998, #50390, #5127, .T. ) ;
#25241=DIRECTION ( 'NONE',  ( -0.000000000000000000, 1.000000000000000000, -0.000000000000000000 ) ) ;
#25243=CARTESIAN_POINT ( 'NONE',  ( -131.6253556217205016, 51.61436399519948282, -74.12161565071266978 ) ) ;
#25244=CARTESIAN_POINT ( 'NONE',  ( 117.7417271423229863, 33.63613196344607559, 37.64637180083228429 ) ) ;
#25247=CARTESIAN_POINT ( 'NONE',  ( 70.46579300139241298, 15.56614468937218732, -69.06676961812144100 ) ) ;
#25249=ORIENTED_EDGE ( 'NONE', *, *, #46747, .T. ) ;
#25252=DIRECTION ( 'NONE',  ( 0.000000000000000000, 0.000000000000000000, 1.000000000000000000 ) ) ;
#25254=CARTESIAN_POINT ( 'NONE',  ( -49.97682018836099616, 14.41498301761731327, -90.86710540830219429 ) ) ;
#25256=CARTESIAN_POINT ( 'NONE',  ( 69.49112875363883290, 15.30845942322121722, -47.01275429639923686 ) ) ;
#25259=CARTESIAN_POINT ( 'NONE',  ( 210.9506883977751954, 115.3310071214937125, 59.40277579576930833 ) ) ;
#25260=EDGE_LOOP ( 'NONE', ( #66624, #46215, #27917, #36035 ) ) ;
#25262=ADVANCED_FACE ( 'NONE', ( #90 ), #5380, .F. ) ;
#25265=DIRECTION ( 'NONE',  ( -0.000000000000000000, 1.000000000000000000, -0.000000000000000000 ) ) ;
#25267=CARTESIAN_POINT ( 'NONE',  ( -84.48447130825533691, 24.62360807013167729, -91.56658158870699538 ) ) ;
#25268=CARTESIAN_POINT ( 'NONE',  ( -190.4966031023458868, 108.8421921967458559, -64.77830472940530626 ) ) ;
#25271=CARTESIAN_POINT ( 'NONE',  ( 38.42020198992003799, 8.283430712587433575, 3.117809402762283355 ) ) ;
#25274=CARTESIAN_POINT ( 'NONE',  ( -78.66644367742111399, 23.39876645725286863, 72.26275173013684139 ) ) ;
#25275=ORIENTED_EDGE ( 'NONE', *, *, #55841, .T. ) ;
#25276=CARTESIAN_POINT ( 'NONE',  ( -120.8704515857978521, 44.46077770807175256, -90.51607353834583591 ) ) ;
#25279=CARTESIAN_POINT ( 'NONE',  ( 8.337549025192448227, 7.382630697225775585, -70.85121512598109916 ) ) ;
#25280=CARTESIAN_POINT ( 'NONE',  ( -23.99924996210629047, 8.487987924059027023, 11.85155207052061321 ) ) ;
#25282=CARTESIAN_POINT ( 'NONE',  ( -14.19447842053094533, 7.389800932646228837, -65.79454045135867091 ) ) ;
#25283=CARTESIAN_POINT ( 'NONE',  ( -99.97541017369788108, 31.62502926470686049, -8.517426260003034599 ) ) ;
#25284=CARTESIAN_POINT ( 'NONE',  ( 152.8672128926848188, 55.41186463791520822, -49.55020588636439527 ) ) ;
#25286=B_SPLINE_CURVE_WITH_KNOTS ( 'NONE', 3,
 ( #1992, #61062, #6558, #23448, #28002, #49446, #45228, #44886, #23782, #39611, #12889, #45575, #29067, #50512, #24133, #66706, #66367, #1279, #18158, #44170, #67057, #29401, #22736, #34351, #12187, #55791, #2332, #7616, #18502, #13235, #39956, #33651, #61412, #34696, #50163, #65657, #66020, #56131 ),
 .UNSPECIFIED., .F., .F.,
 ( 4, 2, 2, 2, 2, 2, 2, 2, 2, 2, 2, 2, 2, 2, 2, 2, 2, 2, 4 ),
 ( 0.000000000000000000, 0.001559859933532175419, 0.003119719867064350838, 0.004679579800596527124, 0.006239439734128701676, 0.007799299667660877095, 0.008579229634426983886, 0.009359159601193090677, 0.01091901953472530599, 0.01169894950149142840, 0.01247887946825755080, 0.01403873940178979561, 0.01559859933532203868, 0.01715845926885430431, 0.01871831920238656646, 0.02027817913591883209, 0.02183803906945109771, 0.02339789900298335987, 0.02495775893651562202 ),
 .UNSPECIFIED. ) ;
#25290=CARTESIAN_POINT ( 'NONE',  ( -155.2836587093738956, 70.59655508952970138, 60.27484905456947928 ) ) ;
#25291=CARTESIAN_POINT ( 'NONE',  ( 173.6024011093110175, 72.73634049052007811, -17.48363501179885660 ) ) ;
#25294=CARTESIAN_POINT ( 'NONE',  ( -118.5043919384112030, 41.81711884544881030, 39.43039629447052619 ) ) ;
#25298=CARTESIAN_POINT ( 'NONE',  ( -180.6209674222603212, 97.47999311542517376, -69.22316660788568754 ) ) ;
#25300=CARTESIAN_POINT ( 'NONE',  ( 86.62931800182293784, 19.42108912189596381, 56.55663816294300261 ) ) ;
#25301=CARTESIAN_POINT ( 'NONE',  ( 116.0773578185793298, 31.67580513411751042, 32.37210107868605036 ) ) ;
#25302=VECTOR ( 'NONE', #13545, 1000.000000000000000 ) ;
#25305=CARTESIAN_POINT ( 'NONE',  ( -173.1211646369891071, 87.12891641440859303, -34.71195716474998960 ) ) ;
#25307=CARTESIAN_POINT ( 'NONE',  ( 197.6316695787930939, 97.13022718399024313, 39.23981542666417255 ) ) ;
#25308=CARTESIAN_POINT ( 'NONE',  ( 117.6865880453676283, 32.48051379280607875, -71.32223984317171528 ) ) ;
#25310=CARTESIAN_POINT ( 'NONE',  ( 139.7883986595927581, 46.32091287009613723, 5.569321396343120512 ) ) ;
#25314=CARTESIAN_POINT ( 'NONE',  ( 180.6713229637342408, 79.61878926895393249, 56.15314469597510794 ) ) ;
#25316=CARTESIAN_POINT ( 'NONE',  ( 67.93317348534928612, 14.90531593353391848, 69.84145773790685041 ) ) ;
#25320=CARTESIAN_POINT ( 'NONE',  ( -175.9852529046322616, 90.37283472601130541, 45.26617804551248270 ) ) ;
#25326=CARTESIAN_POINT ( 'NONE',  ( 55.65927616287137170, 12.11203904137339471, 89.50322596452608082 ) ) ;
#25328=CARTESIAN_POINT ( 'NONE',  ( 15.78827728214693416, 7.507518794609575608, 45.01470767270524931 ) ) ;
#25332=CARTESIAN_POINT ( 'NONE',  ( 151.1873096904021168, 52.92629247302095763, 67.85776711895714186 ) ) ;
#25335=CARTESIAN_POINT ( 'NONE',  ( -95.88693721180807472, 30.76307528361165566, 68.79313100246496049 ) ) ;
#25339=CARTESIAN_POINT ( 'NONE',  ( 157.2533363798599737, 58.75760182111577024, -24.27963370867399107 ) ) ;
#25340=CARTESIAN_POINT ( 'NONE',  ( 207.2640160519426615, 111.6867652229576322, -24.03161405320629029 ) ) ;
#25342=CARTESIAN_POINT ( 'NONE',  ( 109.3047140914111708, 29.55674059952506738, 44.56730977590374465 ) ) ;
#25344=LINE ( 'NONE', #68251, #44913 ) ;
#25345=CARTESIAN_POINT ( 'NONE',  ( 188.2962140587030149, 87.71627202537838741, 7.885122216152835151 ) ) ;
#25347=CARTESIAN_POINT ( 'NONE',  ( 211.8476521439974078, 116.6941316755177525, -41.53835296956879830 ) ) ;
#25349=CARTESIAN_POINT ( 'NONE',  ( 173.6710158776850506, 71.42507420636735560, 8.787227813904088691 ) ) ;
#25351=ORIENTED_EDGE ( 'NONE', *, *, #449, .F. ) ;
#25355=CARTESIAN_POINT ( 'NONE',  ( -73.63128929564827274, 21.53548093502884697, 70.32671424837877794 ) ) ;
#25360=CARTESIAN_POINT ( 'NONE',  ( -14.46762367737944288, 7.414939723119872816, 87.80640566984232009 ) ) ;
#25361=CARTESIAN_POINT ( 'NONE',  ( -108.5248383251030475, 37.21456094989611785, -19.83122018436582934 ) ) ;
#25363=CARTESIAN_POINT ( 'NONE',  ( -73.63346300764936814, 20.46798018699517385, 59.19690935554574196 ) ) ;
#25364=CARTESIAN_POINT ( 'NONE',  ( 198.7554884879576491, 98.53603447819021710, -92.93361033491551382 ) ) ;
#25367=CARTESIAN_POINT ( 'NONE',  ( -156.6819053601226130, 70.51177710383656461, 40.47953577721239071 ) ) ;
#25369=CARTESIAN_POINT ( 'NONE',  ( 176.6258282025054598, 74.21441092921635629, -22.91608747162088733 ) ) ;
#25378=CARTESIAN_POINT ( 'NONE',  ( 212.1931396682533375, 117.2245435827729239, 10.17688792897256356 ) ) ;
#25379=CARTESIAN_POINT ( 'NONE',  ( 13.83281508467570831, 7.452090093180183672, 71.61672662805924006 ) ) ;
#25381=FACE_BOUND ( 'NONE', #45624, .T. ) ;
#25385=ORIENTED_EDGE ( 'NONE', *, *, #66005, .F. ) ;
#25387=CARTESIAN_POINT ( 'NONE',  ( 181.0840389613909736, -170.0000000000000000, -36.22505766587961062 ) ) ;
#25388=CARTESIAN_POINT ( 'NONE',  ( -127.0966118282843809, 48.50115527717463948, 84.40066604616777113 ) ) ;
#25390=CARTESIAN_POINT ( 'NONE',  ( -166.5686015187718567, 80.11916873959170005, -11.70817783129956879 ) ) ;
#25391=CARTESIAN_POINT ( 'NONE',  ( -176.3856149167965555, 92.38076834121982017, 18.24363522339888988 ) ) ;
#25392=CARTESIAN_POINT ( 'NONE',  ( 22.93685557200797831, 6.834779360682496474, 93.49618427415832400 ) ) ;
#25398=CARTESIAN_POINT ( 'NONE',  ( -97.47339919287391297, 30.40512551257289076, 70.64169830722899235 ) ) ;
#25399=ORIENTED_EDGE ( 'NONE', *, *, #67294, .F. ) ;
#25400=CARTESIAN_POINT ( 'NONE',  ( -80.54757501605357106, 23.04700348514570152, 18.33782076323183219 ) ) ;
#25401=VERTEX_POINT ( 'NONE', #20864 ) ;
#25403=CARTESIAN_POINT ( 'NONE',  ( -56.02289203441038978, 15.98631679403371741, -8.418896321847350706 ) ) ;
#25406=CARTESIAN_POINT ( 'NONE',  ( 8.336031647119272137, 6.376437040857336314, -42.04032280401278854 ) ) ;
#25407=CARTESIAN_POINT ( 'NONE',  ( -109.2504972001306101, 37.61384092494594000, -93.42565027757478902 ) ) ;
#25408=CARTESIAN_POINT ( 'NONE',  ( 130.3019683985926349, 39.31883119822049366, 57.23370010971977706 ) ) ;
#25410=CARTESIAN_POINT ( 'NONE',  ( -37.53974046071399329, 10.67241809297004806, 86.99493448681049301 ) ) ;
#25411=ADVANCED_FACE ( 'NONE', ( #15594 ), #10642, .F. ) ;
#25412=CARTESIAN_POINT ( 'NONE',  ( 174.6307688320643479, 73.70327352126999187, -74.40040851124921062 ) ) ;
#25413=CARTESIAN_POINT ( 'NONE',  ( -125.8938041572051389, 46.49392987655492249, 30.61994787315706290 ) ) ;
#25414=CARTESIAN_POINT ( 'NONE',  ( 110.2429982417149432, 28.88204397445229077, -35.92243756565368784 ) ) ;
#25415=CARTESIAN_POINT ( 'NONE',  ( 81.05403189674298403, 18.64820877954959499, -48.36183566878465712 ) ) ;
#25419=CARTESIAN_POINT ( 'NONE',  ( -78.66644367742111399, 23.39876645725286153, -61.96000122218157458 ) ) ;
#25420=CARTESIAN_POINT ( 'NONE',  ( 178.1888264190355073, 77.13727704498029425, 16.89608322330665047 ) ) ;
#25423=CARTESIAN_POINT ( 'NONE',  ( 126.4324872316703363, 37.11876756822024959, 11.26176343780550404 ) ) ;
#25424=CARTESIAN_POINT ( 'NONE',  ( 32.35876450276292360, 7.597628455623533839, -94.19814380599602543 ) ) ;
#25427=DIRECTION ( 'NONE',  ( -0.000000000000000000, 1.000000000000000000, -0.000000000000000000 ) ) ;
#25433=CARTESIAN_POINT ( 'NONE',  ( -62.48837791900216132, 17.85349220731796649, 92.54043131072742767 ) ) ;
#25434=VERTEX_POINT ( 'NONE', #49658 ) ;
#25436=CARTESIAN_POINT ( 'NONE',  ( 199.7255144154428308, 99.76581417577200739, -22.61533049155591613 ) ) ;
#25441=CARTESIAN_POINT ( 'NONE',  ( 8.000000000000007105, 249.8719672152120381, -95.00000000000133582 ) ) ;
#25444=CARTESIAN_POINT ( 'NONE',  ( 36.31593203568479566, 8.028139509847015631, -49.95989190410476510 ) ) ;
#25446=CARTESIAN_POINT ( 'NONE',  ( 8.767814708128309320, 7.383611927972544287, -45.66910925475413308 ) ) ;
#25448=DIRECTION ( 'NONE',  ( 0.000000000000000000, 0.000000000000000000, 1.000000000000000000 ) ) ;
#25449=CARTESIAN_POINT ( 'NONE',  ( 132.7179291807800894, 40.74118679001688292, -50.93987571790520974 ) ) ;
#25452=CARTESIAN_POINT ( 'NONE',  ( 173.6387410343579347, 72.77029877349359310, 91.48744382001903830 ) ) ;
#25454=CARTESIAN_POINT ( 'NONE',  ( -78.66644367742109978, 22.32174330031321574, 72.26275173013684139 ) ) ;
#25455=CARTESIAN_POINT ( 'NONE',  ( -24.70911172866234651, 8.583078995053019966, -73.00837023266150538 ) ) ;
#25457=CARTESIAN_POINT ( 'NONE',  ( 9.288975942802416341, 6.379608420846962780, 14.42107178552651270 ) ) ;
#25458=CARTESIAN_POINT ( 'NONE',  ( 44.34362023773822159, 10.12115849931653599, -75.62784561966921615 ) ) ;
#25459=CYLINDRICAL_SURFACE ( 'NONE', #23371, 7.500000000000013323 ) ;
#25460=CARTESIAN_POINT ( 'NONE',  ( 178.1903523079567435, 75.72906488635190669, -77.50250463138750945 ) ) ;
#25463=CARTESIAN_POINT ( 'NONE',  ( 86.62931800182293784, 19.42108912189600645, -8.977013608448025650 ) ) ;
#25464=DIRECTION ( 'NONE',  ( -0.8118923937861950435, -0.5838071093367415143, 0.000000000000000000 ) ) ;
#25466=ADVANCED_FACE ( 'NONE', ( #33516 ), #23307, .F. ) ;
#25468=VERTEX_POINT ( 'NONE', #44393 ) ;
#25471=CYLINDRICAL_SURFACE ( 'NONE', #19750, 7.500000000000013323 ) ;
#25476=CARTESIAN_POINT ( 'NONE',  ( -189.6704649493768216, 107.6868404312579486, -93.25980815284229664 ) ) ;
#25477=CARTESIAN_POINT ( 'NONE',  ( -58.76005811686688673, 15.70653557534867595, 71.19953605005537156 ) ) ;
#25480=ORIENTED_EDGE ( 'NONE', *, *, #1028, .T. ) ;
#25481=CARTESIAN_POINT ( 'NONE',  ( 180.2572128312848179, 77.77323980479702925, -51.19118848864500393 ) ) ;
#25482=CARTESIAN_POINT ( 'NONE',  ( -179.2177980985565000, 94.18084789436636584, -73.43254121296298820 ) ) ;
#25483=DIRECTION ( 'NONE',  ( 0.000000000000000000, 0.000000000000000000, 1.000000000000000000 ) ) ;
#25486=CYLINDRICAL_SURFACE ( 'NONE', #27770, 7.500000000000013323 ) ;
#25488=CARTESIAN_POINT ( 'NONE',  ( 55.76255201544533691, 12.13275766515752707, -45.19241930457960166 ) ) ;
#25489=CARTESIAN_POINT ( 'NONE',  ( -82.93126516400698733, 25.07709093823494229, 31.74405965836805876 ) ) ;
#25491=CARTESIAN_POINT ( 'NONE',  ( -26.50207385662994852, 9.849226639603649858, -21.64023079453380305 ) ) ;
#25493=CARTESIAN_POINT ( 'NONE',  ( 94.11746922806584337, 22.11341285603782580, 37.70410127150352508 ) ) ;
#25495=ADVANCED_FACE ( 'NONE', ( #7479 ), #66919, .F. ) ;
#25499=CARTESIAN_POINT ( 'NONE',  ( 9.288975942802411012, 6.379608420846962780, 68.11017296645387376 ) ) ;
#25500=CARTESIAN_POINT ( 'NONE',  ( -26.88234027341226451, 9.904106450608205492, 31.73948476484182635 ) ) ;
#25502=CARTESIAN_POINT ( 'NONE',  ( -71.23338454616570914, 20.69243496265646698, 90.55446336941628260 ) ) ;
#25507=EDGE_LOOP ( 'NONE', ( #64848, #58184 ) ) ;
#25508=CARTESIAN_POINT ( 'NONE',  ( 117.6853163455685234, 33.60747889659832310, -69.20596546345770150 ) ) ;
#25513=CARTESIAN_POINT ( 'NONE',  ( -83.13046924527390047, 25.15778674529014936, -21.80259833107481526 ) ) ;
#25519=EDGE_CURVE ( 'NONE', #18819, #51047, #28028, .T. ) ;
#25520=CARTESIAN_POINT ( 'NONE',  ( -102.2801239173131052, 33.91021738430207222, 18.67452391595144334 ) ) ;
#25521=CARTESIAN_POINT ( 'NONE',  ( -78.66644367742109978, 23.39876645725290061, -35.11545063171788428 ) ) ;
#25522=CARTESIAN_POINT ( 'NONE',  ( 103.4225970396116452, 25.85249226022213520, 87.66116462355037697 ) ) ;
#25525=CARTESIAN_POINT ( 'NONE',  ( -190.6985136298601731, 109.1272424661242582, -95.00000000000133582 ) ) ;
#25530=ORIENTED_EDGE ( 'NONE', *, *, #31760, .T. ) ;
#25532=CARTESIAN_POINT ( 'NONE',  ( -150.3831389294225005, 66.25266777263972529, -22.92020021732201229 ) ) ;
#25535=AXIS2_PLACEMENT_3D ( 'NONE', #56860, #18876, #18529 ) ;
#25537=CARTESIAN_POINT ( 'NONE',  ( -156.0300823189601829, 69.91528270335481920, -19.20893955606299386 ) ) ;
#25539=CARTESIAN_POINT ( 'NONE',  ( 32.56927464314651388, 7.618924692399912324, 61.15594928078879633 ) ) ;
#25540=CARTESIAN_POINT ( 'NONE',  ( 15.78827728214693416, 6.500811158483284835, -23.67439350822212774 ) ) ;
#25541=ORIENTED_EDGE ( 'NONE', *, *, #15732, .F. ) ;
#25543=CARTESIAN_POINT ( 'NONE',  ( 23.24047374271772881, 7.861801299833793166, 11.64928986029708646 ) ) ;
#25544=CARTESIAN_POINT ( 'NONE',  ( 188.4389256074243804, 86.37278721358588029, 65.15060996993756248 ) ) ;
#25545=CARTESIAN_POINT ( 'NONE',  ( -125.0023254877051784, 45.90912477771773581, 3.814780357039786018 ) ) ;
#25546=CARTESIAN_POINT ( 'NONE',  ( 67.56108154898466012, 13.77276756375642819, -64.07949261852301959 ) ) ;
#25555=CARTESIAN_POINT ( 'NONE',  ( 127.2107679985236501, 38.70844091144996213, -40.00839590869377105 ) ) ;
#25556=DIRECTION ( 'NONE',  ( -0.000000000000000000, 1.000000000000000000, -0.000000000000000000 ) ) ;
#25558=CARTESIAN_POINT ( 'NONE',  ( 186.2575601542430661, 85.47765906955507376, -38.28966198675566091 ) ) ;
#25564=CARTESIAN_POINT ( 'NONE',  ( 117.7447573007802930, 32.50990724960316669, 64.44597210225181527 ) ) ;
#25565=ORIENTED_EDGE ( 'NONE', *, *, #32697, .F. ) ;
#25566=CARTESIAN_POINT ( 'NONE',  ( 126.4219470349616472, 38.26519385429185149, -69.34525928969384267 ) ) ;
#25567=CARTESIAN_POINT ( 'NONE',  ( 131.6189313563687620, 40.08924984825279125, 44.18369947482882054 ) ) ;
#25569=CARTESIAN_POINT ( 'NONE',  ( -94.77925136849378873, 29.13093715379786985, 38.25092316674201953 ) ) ;
#25570=ADVANCED_FACE ( 'NONE', ( #51070 ), #29961, .F. ) ;
#25573=VERTEX_POINT ( 'NONE', #3918 ) ;
#25575=ADVANCED_FACE ( 'NONE', ( #14806 ), #25038, .F. ) ;
#25579=CARTESIAN_POINT ( 'NONE',  ( -121.5921196778231348, 43.72569502503143468, -21.73089978396855315 ) ) ;
#25586=DIRECTION ( 'NONE',  ( -0.000000000000000000, 1.000000000000000000, -0.000000000000000000 ) ) ;
#25588=DIRECTION ( 'NONE',  ( -0.000000000000000000, 1.000000000000000000, -0.000000000000000000 ) ) ;
#25590=VERTEX_POINT ( 'NONE', #46128 ) ;
#25592=CARTESIAN_POINT ( 'NONE',  ( -56.97107423601133291, 15.20373812575556016, -23.13835194742880219 ) ) ;
#25594=CARTESIAN_POINT ( 'NONE',  ( -126.7944042662569331, 48.29830493043731821, -76.71781960598816852 ) ) ;
#25595=LINE ( 'NONE', #64239, #54992 ) ;
#25597=CARTESIAN_POINT ( 'NONE',  ( 66.73431804020511038, 14.60294556126670074, -76.58299347307310256 ) ) ;
#25601=CARTESIAN_POINT ( 'NONE',  ( 186.6118452967671999, 84.37814701615438651, -65.47550467027663501 ) ) ;
#25604=CARTESIAN_POINT ( 'NONE',  ( 15.78827728214693416, -170.0000000000000000, 30.01470767270522089 ) ) ;
#25605=CARTESIAN_POINT ( 'NONE',  ( -76.10382222627279702, 22.43453174720079346, 44.97093298109892601 ) ) ;
#25606=DIRECTION ( 'NONE',  ( 0.000000000000000000, 0.000000000000000000, 1.000000000000000000 ) ) ;
#25607=CARTESIAN_POINT ( 'NONE',  ( 68.62997155117720638, 15.08415013720829023, -38.22382599589664665 ) ) ;
#25608=CARTESIAN_POINT ( 'NONE',  ( -124.9915686518654638, 47.10215472274616388, 45.61994787315713040 ) ) ;
#25609=CARTESIAN_POINT ( 'NONE',  ( -167.1534554062404254, 80.72263015867913793, -64.50659429279633628 ) ) ;
#25613=CARTESIAN_POINT ( 'NONE',  ( -38.92726670956012924, 10.94099576009806540, 10.38315399778749182 ) ) ;
#25617=CARTESIAN_POINT ( 'NONE',  ( 36.99999522780156269, 9.122638774496634184, 3.460098081212315879 ) ) ;
#25619=B_SPLINE_CURVE_WITH_KNOTS ( 'NONE', 3,
 ( #60132, #34470, #11946, #66830, #65419, #34112, #44293, #44664, #13012, #23559, #18275, #17927, #39041, #39381, #55550, #2443, #7381, #42676, #26162, #21562, #52875, #31781, #42340, #57831, #52544, #47594, #63455, #69052, #43005, #41991, #37743, #26850, #43358, #10319, #64481, #58497, #53564, #37392, #64132, #15609, #4367, #4700, #47944 ),
 .UNSPECIFIED., .F., .F.,
 ( 4, 2, 2, 2, 2, 2, 2, 2, 1, 2, 2, 2, 2, 2, 2, 2, 2, 2, 2, 2, 2, 4 ),
 ( 0.000000000000000000, 0.001466540241398133155, 0.002199810362097199840, 0.002933080482796266309, 0.004399620724194398813, 0.005866160965592531751, 0.007332701206990664689, 0.008065971327689734627, 0.008799241448388802830, 0.009532511569087872769, 0.01026578168978694271, 0.01173232193118507391, 0.01319886217258320858, 0.01466540241398133979, 0.01539867253468040625, 0.01613194265537947272, 0.01759848289677760913, 0.01906502313817574554, 0.01979829325887481201, 0.02053156337957387848, 0.02199810362097201488, 0.02346464386237014782 ),
 .UNSPECIFIED. ) ;
#25622=LINE ( 'NONE', #37186, #56225 ) ;
#25628=CARTESIAN_POINT ( 'NONE',  ( 9.045716588192249219, 7.384596431530731309, -66.54232190796312807 ) ) ;
#25629=CARTESIAN_POINT ( 'NONE',  ( -29.04258984626622819, 9.210213971636683539, 3.760888133432336300 ) ) ;
#25631=CARTESIAN_POINT ( 'NONE',  ( -61.37337919387653784, 16.46775785994717722, -92.36217547766979408 ) ) ;
#25632=CARTESIAN_POINT ( 'NONE',  ( -94.89192151156323973, 29.18342430963126333, -16.98616732492110515 ) ) ;
#25634=CARTESIAN_POINT ( 'NONE',  ( 150.7770046255792806, 53.87214803240242134, -40.23014915691795323 ) ) ;
#25636=ORIENTED_EDGE ( 'NONE', *, *, #34581, .F. ) ;
#25638=CARTESIAN_POINT ( 'NONE',  ( -156.8773151811563196, 72.06122063279305223, 66.48491347657433437 ) ) ;
#25640=CARTESIAN_POINT ( 'NONE',  ( -102.2801239173131052, 33.91021738430207222, -8.170026674512225640 ) ) ;
#25642=CARTESIAN_POINT ( 'NONE',  ( -126.3453033442920912, 47.99870040347946087, -49.91370389823397602 ) ) ;
#25644=CARTESIAN_POINT ( 'NONE',  ( -178.5848962563134137, 94.99295350784007042, -63.89442975738296582 ) ) ;
#25646=CARTESIAN_POINT ( 'NONE',  ( 89.22118407503262461, 20.32164250407901562, 71.09862284774732188 ) ) ;
#25647=CARTESIAN_POINT ( 'NONE',  ( 115.0454575488273434, 31.16784721673997183, 31.34535846184481755 ) ) ;
#25650=CARTESIAN_POINT ( 'NONE',  ( 140.5781926063689298, 45.63383190293698988, 33.67300037928345802 ) ) ;
#25652=CARTESIAN_POINT ( 'NONE',  ( 201.9777685760379882, 102.6876480786892500, 29.70620911343904780 ) ) ;
#25653=CARTESIAN_POINT ( 'NONE',  ( 113.8748103246145433, 30.59837980920001854, -63.68721912812959118 ) ) ;
#25655=CARTESIAN_POINT ( 'NONE',  ( 186.3581035978320131, 84.10482028537325050, -92.06749394508619844 ) ) ;
#25657=ORIENTED_EDGE ( 'NONE', *, *, #15706, .T. ) ;
#25658=CARTESIAN_POINT ( 'NONE',  ( 179.0091171455097765, 77.94933395983134972, 56.43303025292213704 ) ) ;
#25661=CARTESIAN_POINT ( 'NONE',  ( -109.7816385129979295, 36.75776661907239173, -43.01526495903692648 ) ) ;
#25662=CARTESIAN_POINT ( 'NONE',  ( 127.2283196959457001, 37.56363777789739800, 87.17274213372091651 ) ) ;
#25663=CARTESIAN_POINT ( 'NONE',  ( -62.45176220516619026, 16.79101814080731359, 39.06955276880188421 ) ) ;
#25667=EDGE_CURVE ( 'NONE', #68633, #66387, #51758, .T. ) ;
#25669=CARTESIAN_POINT ( 'NONE',  ( 116.0963032583227772, 32.80867113471310148, -48.13800676814181401 ) ) ;
#25670=EDGE_LOOP ( 'NONE', ( #57020, #24001, #35380, #19167 ) ) ;
#25675=ORIENTED_EDGE ( 'NONE', *, *, #31957, .F. ) ;
#25676=CARTESIAN_POINT ( 'NONE',  ( 140.5781926063689582, 45.63383190293701119, 60.51755096974717674 ) ) ;
#25677=CARTESIAN_POINT ( 'NONE',  ( -165.6210506643949429, 79.15024150453837137, 38.62296396642691576 ) ) ;
#25678=CARTESIAN_POINT ( 'NONE',  ( 152.8430172091323413, 54.14068524174419395, 57.84683868187476463 ) ) ;
#25680=EDGE_CURVE ( 'NONE', #34130, #145, #9193, .T. ) ;
#25683=CARTESIAN_POINT ( 'NONE',  ( 41.80372346091802171, 9.750024116765237281, 17.67854651459926529 ) ) ;
#25686=CARTESIAN_POINT ( 'NONE',  ( 152.6804161981488619, 55.27286404993341051, -22.55585361910392095 ) ) ;
#25688=CARTESIAN_POINT ( 'NONE',  ( -58.41772555885023621, 15.60941139747057349, 84.79622561241443179 ) ) ;
#25690=CARTESIAN_POINT ( 'NONE',  ( -155.5978531700835674, 69.52241200678680855, -64.77328047304274605 ) ) ;
#25691=CARTESIAN_POINT ( 'NONE',  ( 55.92341725501096761, 11.13877080681674414, 88.53962230442249393 ) ) ;
#25692=CARTESIAN_POINT ( 'NONE',  ( 188.2086267457325448, 87.61890531228284829, 7.603719067856809843 ) ) ;
#25693=CARTESIAN_POINT ( 'NONE',  ( 206.3125232506203304, 108.5822159704962218, -36.49056922416787785 ) ) ;
#25697=ORIENTED_EDGE ( 'NONE', *, *, #57101, .F. ) ;
#25698=CARTESIAN_POINT ( 'NONE',  ( -76.79042791651912125, 22.68960395613480685, 72.02825304396196771 ) ) ;
#25699=CARTESIAN_POINT ( 'NONE',  ( 188.1848725084043110, 87.59259440284084519, -95.00000000000133582 ) ) ;
#25702=CARTESIAN_POINT ( 'NONE',  ( -0.3421259600789157140, 6.519162826741678352, 91.90210512622793715 ) ) ;
#25705=CARTESIAN_POINT ( 'NONE',  ( -72.21652659655761397, 19.96855882996549525, 60.90274179765688700 ) ) ;
#25706=CARTESIAN_POINT ( 'NONE',  ( -170.2747214445850261, 84.01465441107045251, 72.11803030135118320 ) ) ;
#25709=B_SPLINE_CURVE_WITH_KNOTS ( 'NONE', 3,
 ( #67184, #9805, #61865, #13693, #46042, #62218, #14039, #64295, #16103, #624 ),
 .UNSPECIFIED., .F., .F.,
 ( 4, 2, 2, 2, 4 ),
 ( 0.000000000000000000, 0.002514917400237022104, 0.005029834800474044208, 0.007544752200711065879, 0.01005966960094808842 ),
 .UNSPECIFIED. ) ;
#25710=CARTESIAN_POINT ( 'NONE',  ( -149.9449619562961686, 64.55090813009799433, 30.72082123989904900 ) ) ;
#25711=CARTESIAN_POINT ( 'NONE',  ( 57.08336938683660833, 11.37442068895386349, -38.60525425700638635 ) ) ;
#25712=CARTESIAN_POINT ( 'NONE',  ( 127.7121523762017858, 37.83617439506281244, 94.99999999999866418 ) ) ;
#25713=CARTESIAN_POINT ( 'NONE',  ( 181.0840389613909736, -170.0000000000000000, 9.964043515047732669 ) ) ;
#25716=CARTESIAN_POINT ( 'NONE',  ( -132.6092625803566989, 52.31125232006264980, 41.46967621612935773 ) ) ;
#25718=CARTESIAN_POINT ( 'NONE',  ( 206.2980740120524388, 108.5619562183279925, 2.524772047937632102 ) ) ;
#25719=CARTESIAN_POINT ( 'NONE',  ( 10.82760985890677219, 7.398654328676804504, 70.00562821550327897 ) ) ;
#25720=CARTESIAN_POINT ( 'NONE',  ( 210.9506883977752523, 115.3310071214937267, 32.55822520530563224 ) ) ;
#25721=EDGE_CURVE ( 'NONE', #60122, #11337, #2882, .T. ) ;
#25728=CARTESIAN_POINT ( 'NONE',  ( -128.2034271809940549, 49.24731531185076250, 84.65107715705232749 ) ) ;
#25729=CARTESIAN_POINT ( 'NONE',  ( 33.75794032130628608, 8.754084575552436576, -65.00099313904955523 ) ) ;
#25731=CARTESIAN_POINT ( 'NONE',  ( 10.95123459301218816, 6.393971377372064779, 85.46269591332465154 ) ) ;
#25732=CARTESIAN_POINT ( 'NONE',  ( 18.36632403430998295, 7.603901913571097460, 84.15309218088728471 ) ) ;
#25734=EDGE_LOOP ( 'NONE', ( #14924, #64012, #58633, #54333 ) ) ;
#25737=CARTESIAN_POINT ( 'NONE',  ( -101.3492134984965389, 32.31003911421603192, 72.32043172286272181 ) ) ;
#25739=ADVANCED_FACE ( 'NONE', ( #32380 ), #21465, .F. ) ;
#25740=CARTESIAN_POINT ( 'NONE',  ( -81.67992981004165642, 23.49232121719083111, 4.201518040229789364 ) ) ;
#25745=ORIENTED_EDGE ( 'NONE', *, *, #11405, .F. ) ;
#25746=CARTESIAN_POINT ( 'NONE',  ( -122.8202784017355782, 45.69728649588468272, 18.12070328134850783 ) ) ;
#25748=CARTESIAN_POINT ( 'NONE',  ( -180.6209440844958181, 95.88392769199012378, 65.48622505976561570 ) ) ;
#25749=CARTESIAN_POINT ( 'NONE',  ( 133.6288034103009750, 41.28708886999548611, 56.35489142945903041 ) ) ;
#25755=FACE_OUTER_BOUND ( 'NONE', #49209, .T. ) ;
#25757=CARTESIAN_POINT ( 'NONE',  ( -29.75049355503753290, 9.320234381800291956, 30.40492039785981504 ) ) ;
#25764=CARTESIAN_POINT ( 'NONE',  ( -81.00768240531206743, 24.30850321514432011, -76.58921506343186536 ) ) ;
#25765=CARTESIAN_POINT ( 'NONE',  ( 175.8874477961783782, 74.89984466412600739, 15.39286893903958742 ) ) ;
#25768=CARTESIAN_POINT ( 'NONE',  ( 129.6961120139403647, 38.96846414226716604, 3.921094800805867919 ) ) ;
#25769=CARTESIAN_POINT ( 'NONE',  ( -149.5074843970971017, 64.17983161892347255, 18.87627064943540134 ) ) ;
#25771=CARTESIAN_POINT ( 'NONE',  ( 211.4997502125519304, 118.0043045815490075, 33.53397494038922844 ) ) ;
#25773=CARTESIAN_POINT ( 'NONE',  ( -106.6781182590523400, 35.07133425426479079, 44.11266599922410592 ) ) ;
#25774=VERTEX_POINT ( 'NONE', #7 ) ;
#25775=CARTESIAN_POINT ( 'NONE',  ( -61.07136008913403202, 17.42761989316184668, 87.01993574156381328 ) ) ;
#25777=CARTESIAN_POINT ( 'NONE',  ( -78.66644367742111399, -170.0000000000000000, 3.573650549209445693 ) ) ;
#25781=CARTESIAN_POINT ( 'NONE',  ( 23.28845814680233062, 7.864847136539614425, -70.35012750131396331 ) ) ;
#25782=CARTESIAN_POINT ( 'NONE',  ( 8.000000000000007105, 249.8719672152120381, 94.99999999999866418 ) ) ;
#25783=CARTESIAN_POINT ( 'NONE',  ( -146.1201263095600495, 62.66021356509619977, 71.76068813120549805 ) ) ;
#25786=CARTESIAN_POINT ( 'NONE',  ( 140.2058232509808136, 46.59155168125935376, -39.49978839522578511 ) ) ;
#25787=CARTESIAN_POINT ( 'NONE',  ( 33.75639351246966413, 7.742023566824293823, -48.08197975767080834 ) ) ;
#25788=CARTESIAN_POINT ( 'NONE',  ( 8.288696687633805738, 7.382586467017841159, -43.51982814552570034 ) ) ;
#25793=CARTESIAN_POINT ( 'NONE',  ( 173.6288500197769338, 72.76107365126398463, 89.65482327789845840 ) ) ;
#25795=CARTESIAN_POINT ( 'NONE',  ( 127.5827380604433188, 38.91881311236849683, -93.08189994083937790 ) ) ;
#25799=CARTESIAN_POINT ( 'NONE',  ( 181.0840389613909451, 80.03940679743416808, -9.380507075415923879 ) ) ;
#25802=CARTESIAN_POINT ( 'NONE',  ( 94.07616572255075482, 22.09777530676769430, -17.50139387669658220 ) ) ;
#25803=DIRECTION ( 'NONE',  ( -0.000000000000000000, 1.000000000000000000, -0.000000000000000000 ) ) ;
#25810=CARTESIAN_POINT ( 'NONE',  ( 157.4703587214989398, 58.92748579479259519, 71.25401806271709404 ) ) ;
#25813=CARTESIAN_POINT ( 'NONE',  ( 39.40195752203892710, 9.424259417798131366, 3.069283715499574239 ) ) ;
#25818=FACE_OUTER_BOUND ( 'NONE', #64013, .T. ) ;
#25820=B_SPLINE_CURVE_WITH_KNOTS ( 'NONE', 3,
 ( #3948, #62344, #3261, #61648, #24375, #19423, #56031, #45818, #8884, #8188, #39847, #34595, #35618, #30335, #51787, #3598, #25066, #46496 ),
 .UNSPECIFIED., .F., .F.,
 ( 4, 2, 2, 2, 2, 2, 2, 2, 4 ),
 ( 0.01419378663595921401, 0.01762610661014687996, 0.01934226659724071207, 0.02105842658433454417, 0.02277458657142837628, 0.02449074655852220839, 0.02620690654561604049, 0.02706498653916294267, 0.02792306653270984484 ),
 .UNSPECIFIED. ) ;
#25821=ORIENTED_EDGE ( 'NONE', *, *, #39306, .T. ) ;
#25822=CARTESIAN_POINT ( 'NONE',  ( 32.01010588308077587, 8.573952726883749875, 92.53496508106553620 ) ) ;
#25823=CARTESIAN_POINT ( 'NONE',  ( -1.298947065946362001, -170.0000000000000000, 94.99999999999866418 ) ) ;
#25825=ORIENTED_EDGE ( 'NONE', *, *, #47700, .T. ) ;
#25827=EDGE_CURVE ( 'NONE', #42723, #25068, #10325, .T. ) ;
#25830=CARTESIAN_POINT ( 'NONE',  ( 37.00112095025829717, 8.109340230899350743, -9.165684967028395747 ) ) ;
#25831=EDGE_CURVE ( 'NONE', #27030, #19968, #2742, .T. ) ;
#25832=CARTESIAN_POINT ( 'NONE',  ( 174.6242782760050147, 73.69713439533578025, -39.90515018124950331 ) ) ;
#25834=CARTESIAN_POINT ( 'NONE',  ( -151.6648563624119390, 67.36546864992754990, -76.35397280829764100 ) ) ;
#25836=EDGE_LOOP ( 'NONE', ( #39874, #31621, #61516, #35941 ) ) ;
#25838=CARTESIAN_POINT ( 'NONE',  ( 10.13405324523498763, 6.385324379632245417, 59.40699386941561499 ) ) ;
#25839=CARTESIAN_POINT ( 'NONE',  ( 15.78827728214693416, 6.500811158483284835, 30.01470767270522089 ) ) ;
#25840=CARTESIAN_POINT ( 'NONE',  ( 197.8588046850313447, 99.02485934465606476, 39.80106156302998954 ) ) ;
#25841=CARTESIAN_POINT ( 'NONE',  ( -73.15154738012903124, 21.36451140970928364, 86.51439797908847140 ) ) ;
#25847=ORIENTED_EDGE ( 'NONE', *, *, #61538, .T. ) ;
#25850=CARTESIAN_POINT ( 'NONE',  ( 203.1511228994172598, 104.2426341584999250, -78.05527855006161531 ) ) ;
#25853=CARTESIAN_POINT ( 'NONE',  ( -118.7011677090247019, 41.93687969120208692, 62.82317554766216006 ) ) ;
#25854=CARTESIAN_POINT ( 'NONE',  ( -81.24432217070641116, 24.40203426192926273, -8.723820200429852179 ) ) ;
#25855=CARTESIAN_POINT ( 'NONE',  ( 19.53470118933706345, 6.649487981843460460, -22.67626940826310999 ) ) ;
#25856=CARTESIAN_POINT ( 'NONE',  ( -156.9252506979472912, 70.73559306219776488, -43.45703707063664467 ) ) ;
#25860=CARTESIAN_POINT ( 'NONE',  ( -80.54915509118112027, 24.12810583352864313, -49.87922971066491584 ) ) ;
#25861=CARTESIAN_POINT ( 'NONE',  ( 162.8142581494936110, 61.92799983924231810, 69.03799929907479793 ) ) ;
#25863=CARTESIAN_POINT ( 'NONE',  ( -151.6797345123119101, 67.37848486615951060, 18.56841981061283420 ) ) ;
#25867=ORIENTED_EDGE ( 'NONE', *, *, #20731, .T. ) ;
#25869=EDGE_LOOP ( 'NONE', ( #45941, #41775, #9574, #47154 ) ) ;
#25873=CARTESIAN_POINT ( 'NONE',  ( -35.17718245314462422, 11.25729435722176852, -63.15510929693514441 ) ) ;
#25874=CARTESIAN_POINT ( 'NONE',  ( -156.1462053606562392, 70.02140399657014314, -11.96835739834466850 ) ) ;
#25877=CARTESIAN_POINT ( 'NONE',  ( -31.43908319763709969, 10.61114334766715572, 3.371903815725488585 ) ) ;
#25878=CARTESIAN_POINT ( 'NONE',  ( 8.528421445032398296, 6.376778749352035369, -18.11991088350285395 ) ) ;
#25879=CARTESIAN_POINT ( 'NONE',  ( 22.51798020284707391, 7.817376421459706570, 7.350245662626018195 ) ) ;
#25881=CARTESIAN_POINT ( 'NONE',  ( -118.5043919384110893, 41.81711884544878188, 12.58584570400684832 ) ) ;
#25883=CARTESIAN_POINT ( 'NONE',  ( 126.8237978310704221, 37.33705012421151537, -14.06003659058230326 ) ) ;
#25884=DIRECTION ( 'NONE',  ( 0.000000000000000000, 0.000000000000000000, 1.000000000000000000 ) ) ;
#25885=EDGE_CURVE ( 'NONE', #21982, #8644, #60671, .T. ) ;
#25886=CARTESIAN_POINT ( 'NONE',  ( 8.337549025192451779, 7.382630697225775585, 9.682436645409964626 ) ) ;
#25889=FACE_OUTER_BOUND ( 'NONE', #68337, .T. ) ;
#25891=CARTESIAN_POINT ( 'NONE',  ( 173.8575673535406168, 71.59843387604338716, 34.78079572034797451 ) ) ;
#25892=CARTESIAN_POINT ( 'NONE',  ( 63.01563776193091826, -170.0000000000000000, 10.46841034875760279 ) ) ;
#25893=CARTESIAN_POINT ( 'NONE',  ( -109.7811201291769692, 37.90784085457602970, -42.28424908827382467 ) ) ;
#25894=CARTESIAN_POINT ( 'NONE',  ( 184.0001683447903815, 83.06228184427187955, -50.64836551222349925 ) ) ;
#25897=CARTESIAN_POINT ( 'NONE',  ( -27.70005010046228122, 9.007417901453010245, -9.466521581063075175 ) ) ;
#25898=EDGE_CURVE ( 'NONE', #18637, #34501, #51466, .T. ) ;
#25899=CARTESIAN_POINT ( 'NONE',  ( 202.7506655727289342, 105.3943386412348957, 17.11760266916378725 ) ) ;
#25905=CARTESIAN_POINT ( 'NONE',  ( 128.3856248084844651, 38.21741401878865219, 31.85676776503090224 ) ) ;
#25906=EDGE_CURVE ( 'NONE', #41593, #36484, #54799, .T. ) ;
#25914=EDGE_LOOP ( 'NONE', ( #54426, #46786 ) ) ;
#25916=CARTESIAN_POINT ( 'NONE',  ( -173.1211646369891355, 88.63826465341151106, 3.977144016177345254 ) ) ;
#25919=CARTESIAN_POINT ( 'NONE',  ( -149.0732005398558044, 63.81212100765654327, -34.82227269216089383 ) ) ;
#25921=DIRECTION ( 'NONE',  ( -0.000000000000000000, 1.000000000000000000, -0.000000000000000000 ) ) ;
#25924=FACE_OUTER_BOUND ( 'NONE', #63101, .T. ) ;
#25926=CARTESIAN_POINT ( 'NONE',  ( -126.3495878770406478, 48.00153794568856824, -61.75825448869760947 ) ) ;
#25928=CARTESIAN_POINT ( 'NONE',  ( -130.2071229607962266, 50.62285182196874445, 17.42881725291558936 ) ) ;
#25929=CARTESIAN_POINT ( 'NONE',  ( -150.9154386825424865, 65.38313372076783025, -88.63248908416815652 ) ) ;
#25932=CARTESIAN_POINT ( 'NONE',  ( 188.5843222076478867, 86.53342480589840591, -70.27300197745584853 ) ) ;
#25933=CARTESIAN_POINT ( 'NONE',  ( -165.6398193834832853, 79.16932278174807891, -42.82268507880024089 ) ) ;
#25934=LINE ( 'NONE', #62172, #49710 ) ;
#25935=CARTESIAN_POINT ( 'NONE',  ( 104.7227067006896561, 27.50728936118535728, -75.36740411498894332 ) ) ;
#25937=CARTESIAN_POINT ( 'NONE',  ( -76.78104518372332166, 22.68568622761702258, 30.64349253551715080 ) ) ;
#25938=CARTESIAN_POINT ( 'NONE',  ( -73.63128929564827274, 21.53548093502884697, -63.89603870393958829 ) ) ;
#25939=CARTESIAN_POINT ( 'NONE',  ( -145.9095871962850310, 61.18682730038538864, 44.80555181577465618 ) ) ;
#25940=CARTESIAN_POINT ( 'NONE',  ( -118.7011544766493643, 43.11604763363182968, 40.26125301860250261 ) ) ;
#25941=CARTESIAN_POINT ( 'NONE',  ( -167.6386155194958292, 81.22597462185140671, -63.91328706315006514 ) ) ;
#25944=CARTESIAN_POINT ( 'NONE',  ( -107.7893514267588273, 35.66840175773126731, -20.78274561057057568 ) ) ;
#25945=B_SPLINE_CURVE_WITH_KNOTS ( 'NONE', 3,
 ( #14269, #56477, #68091, #8301, #19185, #35730, #24491, #45929, #40639, #46613, #35378, #8651, #30105, #51560, #8996, #30443, #51891, #3704, #25178, #19892, #41350, #43050, #20921, #59230, #64520, #63490, #26548, #53941, #53605, #15304, #5433, #26886, #68749, #9684, #11049, #16673, #38127, #5082, #48311, #53252, #32510, #144, #15645, #64169, #16330, #58536, #5764, #63835, #15983, #26200, #37096, #48659, #10355, #37785, #31149, #42374, #31821, #47980 ),
 .UNSPECIFIED., .F., .F.,
 ( 4, 2, 2, 2, 2, 2, 2, 2, 2, 2, 2, 2, 2, 2, 2, 2, 2, 2, 2, 2, 2, 2, 2, 2, 2, 2, 2, 2, 4 ),
 ( 0.000000000000000000, 0.002115217322790804468, 0.003172825984186181981, 0.004230434645581559495, 0.005288043306976936142, 0.006345651968372312789, 0.007403260629767689435, 0.008460869291163065214, 0.01057608661395382198, 0.01163369527534918041, 0.01269130393674454231, 0.01480652125953524009, 0.01692173858232593614, 0.01797934724372131712, 0.01903695590511669811, 0.02115217322790744967, 0.02220978188930281677, 0.02326739055069818735, 0.02538260787348892850, 0.02644021653488426091, 0.02749782519627959679, 0.02802662952697726820, 0.02855543385767493961, 0.02961304251907029977, 0.03014184684976798159, 0.03067065118046566341, 0.03172825984186106868, 0.03278586850325648089, 0.03384347716465187922 ),
 .UNSPECIFIED. ) ;
#25947=AXIS2_PLACEMENT_3D ( 'NONE', #17145, #48799, #44229 ) ;
#25948=CARTESIAN_POINT ( 'NONE',  ( -33.36721086971962080, 9.915747831546610769, 18.12394761578280367 ) ) ;
#25951=CARTESIAN_POINT ( 'NONE',  ( -190.3061188229049208, 108.5745819235682035, -65.07512604326164762 ) ) ;
#25955=CARTESIAN_POINT ( 'NONE',  ( -95.63694837622350065, 30.64472169584719197, -65.86884539641842196 ) ) ;
#25956=CARTESIAN_POINT ( 'NONE',  ( -37.39246151129642470, 11.66872370876246201, -11.38479204114821286 ) ) ;
#25961=CARTESIAN_POINT ( 'NONE',  ( 61.09977118998600787, 13.26754120022606642, 56.90226584646475061 ) ) ;
#25962=CARTESIAN_POINT ( 'NONE',  ( 8.763528846667103522, 7.383598436776581231, -67.22465256489064700 ) ) ;
#25965=CARTESIAN_POINT ( 'NONE',  ( -10.23867141318106455, 7.059827648235817321, -76.88073892781783059 ) ) ;
#25967=CARTESIAN_POINT ( 'NONE',  ( -95.04120270830169659, 29.25306318840326725, -13.64142617559394388 ) ) ;
#25968=CARTESIAN_POINT ( 'NONE',  ( 150.0516754638056227, 53.34587188591233797, -44.75957873094871076 ) ) ;
#25969=EDGE_CURVE ( 'NONE', #65764, #52913, #26292, .T. ) ;
#25970=EDGE_LOOP ( 'NONE', ( #55663, #24678, #30062, #5035 ) ) ;
#25974=CARTESIAN_POINT ( 'NONE',  ( 174.9099402067542997, 73.96774984027638311, -12.61427854525189929 ) ) ;
#25979=CARTESIAN_POINT ( 'NONE',  ( -1.083610669212420996, 6.545642299653492202, -12.75074224467104322 ) ) ;
#25980=CARTESIAN_POINT ( 'NONE',  ( 200.8383807319521566, 102.8517715783673623, -23.42650824558267075 ) ) ;
#25981=CARTESIAN_POINT ( 'NONE',  ( -156.3413281584584809, 70.19975255048969132, 94.99999999999866418 ) ) ;
#25984=CARTESIAN_POINT ( 'NONE',  ( 134.3172730033263349, 41.70277427218489663, 44.51034083899535432 ) ) ;
#25985=EDGE_CURVE ( 'NONE', #60940, #58006, #29655, .T. ) ;
#25986=ORIENTED_EDGE ( 'NONE', *, *, #46747, .F. ) ;
#25988=DIRECTION ( 'NONE',  ( 0.000000000000000000, -1.000000000000000000, 0.000000000000000000 ) ) ;
#25989=EDGE_CURVE ( 'NONE', #41887, #51139, #8948, .T. ) ;
#25990=CARTESIAN_POINT ( 'NONE',  ( 187.2296622856351860, 86.53808614709454616, 32.50155238689070814 ) ) ;
#25991=CARTESIAN_POINT ( 'NONE',  ( 164.1352994389932576, 64.33767534192701021, 6.615417748415636012 ) ) ;
#25995=ORIENTED_EDGE ( 'NONE', *, *, #52728, .F. ) ;
#26001=CARTESIAN_POINT ( 'NONE',  ( -57.42615654242915468, 15.33060010148603070, 44.93600813576141206 ) ) ;
#26002=CARTESIAN_POINT ( 'NONE',  ( 197.6319840686292082, 98.73992647122672395, -95.00000000000133582 ) ) ;
#26004=CARTESIAN_POINT ( 'NONE',  ( -180.2252811616041583, 95.40045830523430936, 40.74347283216714288 ) ) ;
#26007=CARTESIAN_POINT ( 'NONE',  ( 116.0822834687217124, 32.80169113915573575, -38.68990360584331967 ) ) ;
#26011=CARTESIAN_POINT ( 'NONE',  ( 136.1310312718401008, 42.81430973242785143, 71.01667174595678489 ) ) ;
#26012=CARTESIAN_POINT ( 'NONE',  ( -125.8938041572051389, -170.0000000000000000, -69.25825448869763079 ) ) ;
#26013=CARTESIAN_POINT ( 'NONE',  ( 133.8566784816069344, -170.0000000000000000, 63.85489142945905172 ) ) ;
#26016=CARTESIAN_POINT ( 'NONE',  ( 46.84154678921881043, 10.51341196666389344, 9.587434892585696034 ) ) ;
#26018=CARTESIAN_POINT ( 'NONE',  ( 153.2523375521184619, 55.69936538551848315, -22.98567760057999365 ) ) ;
#26019=CARTESIAN_POINT ( 'NONE',  ( 212.1978255065451151, 119.0880569674902745, -16.63249047809884473 ) ) ;
#26021=CARTESIAN_POINT ( 'NONE',  ( -156.6692143066620986, 70.50016761530888232, -71.40156983480068220 ) ) ;
#26022=CARTESIAN_POINT ( 'NONE',  ( -109.7844028549000370, 36.75929263860175666, 91.49416231544373090 ) ) ;
#26023=CARTESIAN_POINT ( 'NONE',  ( 183.7875981612220073, 82.83906702837188618, 16.96311135807992798 ) ) ;
#26024=CARTESIAN_POINT ( 'NONE',  ( 212.1535111375854399, 117.1635556319084657, -42.99501597635795491 ) ) ;
#26027=FACE_OUTER_BOUND ( 'NONE', #64676, .T. ) ;
#26029=CARTESIAN_POINT ( 'NONE',  ( -74.79539698934962644, 21.95498232236881719, 58.33441674758699236 ) ) ;
#26031=CARTESIAN_POINT ( 'NONE',  ( -95.50384525802328994, 29.46973564057716288, -39.28996472385307470 ) ) ;
#26032=CARTESIAN_POINT ( 'NONE',  ( 59.29615173875417611, 11.84060224810187911, -76.58255111298183238 ) ) ;
#26035=CARTESIAN_POINT ( 'NONE',  ( 16.77104078056616032, 7.540619757007628543, 44.96607726379911441 ) ) ;
#26037=DIRECTION ( 'NONE',  ( -0.000000000000000000, 1.000000000000000000, -0.000000000000000000 ) ) ;
#26041=CARTESIAN_POINT ( 'NONE',  ( -171.4814970982680791, 85.32124710276292490, 72.49661911005092918 ) ) ;
#26044=CARTESIAN_POINT ( 'NONE',  ( -30.94745021534356155, 10.53010394565407282, -62.16174795566551126 ) ) ;
#26051=CARTESIAN_POINT ( 'NONE',  ( -142.0062637385110236, 58.06920992247432167, 11.92674320627384255 ) ) ;
#26055=CARTESIAN_POINT ( 'NONE',  ( -133.3944793432480367, 52.87251459353622352, 38.37487159473982246 ) ) ;
#26057=CARTESIAN_POINT ( 'NONE',  ( 209.6877167158270652, 113.4449353909247264, 15.46721332339767585 ) ) ;
#26058=CARTESIAN_POINT ( 'NONE',  ( 184.5140223535449309, 83.60465277292396991, -90.70322354721781721 ) ) ;
#26060=CARTESIAN_POINT ( 'NONE',  ( -5.183193881612060849, 7.740932022135019963, 71.48359962217394070 ) ) ;
#26065=CARTESIAN_POINT ( 'NONE',  ( -119.1064753703575718, 43.36500113374746945, 94.99999999999866418 ) ) ;
#26066=CARTESIAN_POINT ( 'NONE',  ( 36.08914434112045200, 9.014684630517857400, -63.23120754001776334 ) ) ;
#26068=CARTESIAN_POINT ( 'NONE',  ( 70.38121440378668581, 14.50253793787158507, 38.79010627313403603 ) ) ;
#26069=CARTESIAN_POINT ( 'NONE',  ( 16.12102920665804362, 7.518218183539778998, 83.70402026746120328 ) ) ;
#26074=B_SPLINE_CURVE_WITH_KNOTS ( 'NONE', 3,
 ( #34437, #28084, #38648, #40041, #45667, #67145, #55516, #7693, #12615, #61500, #60089, #66099, #13317, #8028, #6636, #33729, #34774, #55878, #65741, #49527, #11910, #44621, #66794, #33387, #1713, #17893, #39348, #29481, #2756, #7344, #24219, #60451, #39007, #12267, #55162, #28438, #1362, #6985, #49890, #66449, #50248, #28800, #60791, #2070, #44964 ),
 .UNSPECIFIED., .F., .F.,
 ( 4, 2, 2, 2, 2, 2, 2, 2, 2, 2, 2, 1, 2, 2, 2, 2, 2, 2, 2, 2, 2, 2, 4 ),
 ( 0.000000000000000000, 0.001512548138464676417, 0.002268822207697016903, 0.003025096276929357172, 0.004537644415394002581, 0.005293918484626342416, 0.006050192553858681384, 0.007562740692323361054, 0.009075288830788039857, 0.01058783696925271953, 0.01134411103848505589, 0.01210038510771739399, 0.01285665917694972689, 0.01361293324618205978, 0.01512548138464670650, 0.01588175545387902204, 0.01663802952311134106, 0.01815057766157596175, 0.01966312580004058938, 0.02041939986927290493, 0.02117567393850521701, 0.02268822207696980994, 0.02420077021543439941 ),
 .UNSPECIFIED. ) ;
#26075=CARTESIAN_POINT ( 'NONE',  ( -78.66644367742109978, 22.32174330031319442, 3.573650549209446137 ) ) ;
#26079=CARTESIAN_POINT ( 'NONE',  ( -118.4709174626548531, 42.97515378817185194, 12.38156042881829677 ) ) ;
#26080=CARTESIAN_POINT ( 'NONE',  ( -175.1920326508032986, 89.46239303019289935, 57.94521480769297739 ) ) ;
#26081=CARTESIAN_POINT ( 'NONE',  ( 133.3996297101684831, 41.14871796345732946, 71.35489142945908725 ) ) ;
#26084=CARTESIAN_POINT ( 'NONE',  ( -38.93122880031071276, 10.94177517338562389, 90.93378199072627410 ) ) ;
#26087=CARTESIAN_POINT ( 'NONE',  ( 105.8022841538864185, 26.88074187880708621, -49.48557371029213670 ) ) ;
#26088=CARTESIAN_POINT ( 'NONE',  ( -25.50312845906834980, 8.692070753302669317, 33.12567030776318688 ) ) ;
#26093=CARTESIAN_POINT ( 'NONE',  ( -81.01931326044683601, 24.31309346877660715, -62.33462428330359728 ) ) ;
#26094=CARTESIAN_POINT ( 'NONE',  ( 173.5844030397475706, 72.71952271766126330, 9.659088270331640302 ) ) ;
#26097=CARTESIAN_POINT ( 'NONE',  ( -83.51110947562231956, 25.31252704029285283, 5.343194909942403648 ) ) ;
#26098=CARTESIAN_POINT ( 'NONE',  ( 132.0582325211145189, 40.34869848118184166, 17.46102436708167360 ) ) ;
#26099=CARTESIAN_POINT ( 'NONE',  ( -152.2964402771109178, 66.58174574061955298, 18.34200323450853531 ) ) ;
#26100=CARTESIAN_POINT ( 'NONE',  ( 197.3671887352768408, 98.40825776222057186, 88.79584330558347460 ) ) ;
#26101=CARTESIAN_POINT ( 'NONE',  ( 69.73342236697679652, 14.33173522011652601, 7.097129799427905006 ) ) ;
#26103=LINE ( 'NONE', #58442, #63477 ) ;
#26107=CARTESIAN_POINT ( 'NONE',  ( -60.23623261180705413, 17.18081742568415038, 86.05829893146599829 ) ) ;
#26108=ORIENTED_EDGE ( 'NONE', *, *, #27692, .T. ) ;
#26110=EDGE_LOOP ( 'NONE', ( #32584, #25697 ) ) ;
#26111=CARTESIAN_POINT ( 'NONE',  ( 22.15926701483429895, 7.796117250416235933, -65.89848683517405448 ) ) ;
#26112=CARTESIAN_POINT ( 'NONE',  ( -168.1811549361197251, 83.25427431521137578, 32.67343048873900102 ) ) ;
#26114=CARTESIAN_POINT ( 'NONE',  ( 134.3135005523732559, 42.87884033955815966, -51.01290741596099565 ) ) ;
#26120=ADVANCED_FACE ( 'NONE', ( #52199 ), #24782, .F. ) ;
#26121=VERTEX_POINT ( 'NONE', #26157 ) ;
#26123=CARTESIAN_POINT ( 'NONE',  ( 174.8710133519038550, 73.93068202503360453, 94.71388927649152834 ) ) ;
#26125=CARTESIAN_POINT ( 'NONE',  ( 130.2230634515710790, 40.43733067189506869, -90.64009857926562574 ) ) ;
#26127=VECTOR ( 'NONE', #10915, 1000.000000000000000 ) ;
#26131=CARTESIAN_POINT ( 'NONE',  ( 181.9411407973024950, 80.91291802046383452, -9.380507075415929208 ) ) ;
#26132=CARTESIAN_POINT ( 'NONE',  ( 174.6176230994777825, 72.30829341023250834, -66.73030761740862715 ) ) ;
#26135=CARTESIAN_POINT ( 'NONE',  ( 93.71772995179816235, 21.96265635001559602, -14.01375245968642957 ) ) ;
#26136=DIRECTION ( 'NONE',  ( 0.000000000000000000, 0.000000000000000000, 1.000000000000000000 ) ) ;
#26138=CARTESIAN_POINT ( 'NONE',  ( 163.2911130186311084, 63.63047778106599139, 68.49022856848731067 ) ) ;
#26142=ORIENTED_EDGE ( 'NONE', *, *, #1113, .T. ) ;
#26143=CARTESIAN_POINT ( 'NONE',  ( -124.9927180788553613, 45.90286323198617424, -34.95429498894391429 ) ) ;
#26145=LINE ( 'NONE', #47577, #21747 ) ;
#26147=CARTESIAN_POINT ( 'NONE',  ( 149.9552318077303994, 52.03645901322386891, 10.08806978535764109 ) ) ;
#26150=CARTESIAN_POINT ( 'NONE',  ( -13.12090985667452969, 8.303654651054307223, 85.96412694177334402 ) ) ;
#26156=CARTESIAN_POINT ( 'NONE',  ( 46.58804170569938918, 10.47239957174000047, 88.93053816599565664 ) ) ;
#26157=CARTESIAN_POINT ( 'NONE',  ( -173.1211646369891355, 88.63826465341151106, -88.40105834567734178 ) ) ;
#26158=DIRECTION ( 'NONE',  ( -0.8118923937861950435, -0.5838071093367415143, 0.000000000000000000 ) ) ;
#26162=CARTESIAN_POINT ( 'NONE',  ( -0.5783162822156601157, 7.534184941292926929, 12.71782406034808588 ) ) ;
#26163=CARTESIAN_POINT ( 'NONE',  ( 158.3636111008086402, 59.62671916656141491, 44.40946747225338243 ) ) ;
#26164=CARTESIAN_POINT ( 'NONE',  ( -154.6085044440278580, 69.98390342970668598, -74.66063903122440593 ) ) ;
#26170=CARTESIAN_POINT ( 'NONE',  ( 12.46490660984525078, 7.423426948220647859, 44.24267865148938483 ) ) ;
#26172=CARTESIAN_POINT ( 'NONE',  ( -86.09946351606596693, 26.38487962042298207, 90.55497946160751610 ) ) ;
#26173=DIRECTION ( 'NONE',  ( 0.000000000000000000, 0.000000000000000000, 1.000000000000000000 ) ) ;
#26177=EDGE_LOOP ( 'NONE', ( #50058, #37190 ) ) ;
#26179=CARTESIAN_POINT ( 'NONE',  ( 116.8917656767876565, 33.20682060519245482, -66.78745051061426352 ) ) ;
#26180=FACE_OUTER_BOUND ( 'NONE', #63459, .T. ) ;
#26182=CARTESIAN_POINT ( 'NONE',  ( 198.7084915431529737, 98.47675983942191635, -75.19271672455441546 ) ) ;
#26183=CARTESIAN_POINT ( 'NONE',  ( -33.36965723649377935, 10.93726715887724232, 57.30962576113447682 ) ) ;
#26185=CARTESIAN_POINT ( 'NONE',  ( -10.92576759990585167, 8.121994053275074066, -9.239980494406424327 ) ) ;
#26186=CARTESIAN_POINT ( 'NONE',  ( 150.2809931605061990, 52.27058242113233888, -72.62185156043770462 ) ) ;
#26190=CARTESIAN_POINT ( 'NONE',  ( -149.5074843970971301, 64.17983161892345834, -49.81283053149198992 ) ) ;
#26193=CARTESIAN_POINT ( 'NONE',  ( 70.11969827741707206, 15.47408882293423638, -13.92140172406558030 ) ) ;
#26195=CIRCLE ( 'NONE', #46421, 243.4957430088094839 ) ;
#26196=CARTESIAN_POINT ( 'NONE',  ( 103.6419690634046589, 25.94571131443040102, 94.42721007842214931 ) ) ;
#26197=CARTESIAN_POINT ( 'NONE',  ( -153.1031717208032319, 68.63449618039567213, 4.790432509985504517 ) ) ;
#26199=CARTESIAN_POINT ( 'NONE',  ( 19.53470118933705990, 6.649487981843464013, 31.01283177266423152 ) ) ;
#26200=CARTESIAN_POINT ( 'NONE',  ( -157.0038757045938667, 72.17867991799593597, 91.61780177421432825 ) ) ;
#26201=EDGE_LOOP ( 'NONE', ( #16513, #59322 ) ) ;
#26206=CARTESIAN_POINT ( 'NONE',  ( 38.90907126433564400, 9.359889524363177671, -35.61981746542775795 ) ) ;
#26207=CARTESIAN_POINT ( 'NONE',  ( 110.2429982417149432, 28.88204397445230853, -89.61153874658103291 ) ) ;
#26210=CARTESIAN_POINT ( 'NONE',  ( 203.1423857108908066, 105.9238244286949850, 56.20468668297329629 ) ) ;
#26212=CARTESIAN_POINT ( 'NONE',  ( 32.67604581760325999, 7.629767527669977234, 67.58595727477110415 ) ) ;
#26213=CARTESIAN_POINT ( 'NONE',  ( 9.057575839850580124, 6.378493414438676012, -12.85657236994559582 ) ) ;
#26215=CARTESIAN_POINT ( 'NONE',  ( 19.75315861330098244, 7.667327050329334703, 4.299178115857797522 ) ) ;
#26216=CARTESIAN_POINT ( 'NONE',  ( 188.2076037774874351, 86.11782719225436722, 61.28972546789033515 ) ) ;
#26218=CARTESIAN_POINT ( 'NONE',  ( -85.75222301046099460, 25.14826148333819233, -40.10669955425598943 ) ) ;
#26219=CARTESIAN_POINT ( 'NONE',  ( 23.03864809957654103, 6.841061756139153793, 66.29383730662293317 ) ) ;
#26221=CARTESIAN_POINT ( 'NONE',  ( 110.2429982417149574, 29.99119854320843714, 17.76666361527367499 ) ) ;
#26223=ORIENTED_EDGE ( 'NONE', *, *, #43178, .F. ) ;
#26225=CARTESIAN_POINT ( 'NONE',  ( 187.5272808203428099, 85.37192123373904451, 6.087187552396759571 ) ) ;
#26228=CARTESIAN_POINT ( 'NONE',  ( -31.93169728792081941, 10.69234447276976674, -35.31719736520182806 ) ) ;
#26230=CARTESIAN_POINT ( 'NONE',  ( -105.8879245385188312, 35.79035667534148502, -35.92177053218349414 ) ) ;
#26238=CARTESIAN_POINT ( 'NONE',  ( -25.98312968277007684, 8.759224980175270403, -21.12456965610049053 ) ) ;
#26240=CARTESIAN_POINT ( 'NONE',  ( 174.0302671031634247, 71.75925975512330979, 87.94198868075041275 ) ) ;
#26241=ORIENTED_EDGE ( 'NONE', *, *, #42162, .T. ) ;
#26243=B_SPLINE_CURVE_WITH_KNOTS ( 'NONE', 3,
 ( #48291, #53922, #38106, #49692, #55326, #54630, #65196, #16649, #27906, #16991, #48992, #59550, #11719, #12084, #38460, #832, #6457, #37762, #16309, #11367, #59207, #44429, #32834, #6091, #33192, #17345, #49342, #11027, #32491, #5745, #479, #7150, #1522, #33551, #27200, #1175, #54265, #21927, #22630, #27550, #44069, #48635, #64849, #122, #60614 ),
 .UNSPECIFIED., .F., .F.,
 ( 4, 2, 2, 2, 2, 2, 2, 2, 1, 2, 2, 2, 2, 2, 2, 2, 2, 2, 2, 2, 2, 2, 4 ),
 ( 0.000000000000000000, 0.001467747071934226953, 0.002201620607901337394, 0.002935494143868447835, 0.004403241215802664379, 0.005870988287736880057, 0.007338735359671097469, 0.008072608895638206175, 0.008806482431605313146, 0.009540355967572421853, 0.01027422950353953056, 0.01174197657547374797, 0.01247585011144085147, 0.01320972364740795497, 0.01467747071934215851, 0.01541134425530925681, 0.01614521779127635684, 0.01761296486321056037, 0.01908071193514476738, 0.01981458547111187435, 0.02054845900707898479, 0.02201620607901318832, 0.02348395315094739533 ),
 .UNSPECIFIED. ) ;
#26244=CARTESIAN_POINT ( 'NONE',  ( 150.5165549438847563, 53.68267614960137024, 93.43292638355033830 ) ) ;
#26248=CARTESIAN_POINT ( 'NONE',  ( -95.54114085644955878, 30.59949910443587839, 94.99999999999866418 ) ) ;
#26250=CARTESIAN_POINT ( 'NONE',  ( -99.31850058233800382, 31.30166762705811223, 44.91357497810577115 ) ) ;
#26253=ORIENTED_EDGE ( 'NONE', *, *, #63510, .F. ) ;
#26256=ORIENTED_EDGE ( 'NONE', *, *, #3499, .F. ) ;
#26259=CARTESIAN_POINT ( 'NONE',  ( -178.2381786520593323, 93.01028335822120141, -9.878879645691533540 ) ) ;
#26261=CARTESIAN_POINT ( 'NONE',  ( -149.5074843970971017, 64.17983161892347255, -34.81283053149196149 ) ) ;
#26262=VERTEX_POINT ( 'NONE', #65173 ) ;
#26263=CARTESIAN_POINT ( 'NONE',  ( -109.7868734384453973, 37.91103670584237051, 91.81079717178241140 ) ) ;
#26264=VERTEX_POINT ( 'NONE', #11005 ) ;
#26265=CARTESIAN_POINT ( 'NONE',  ( -55.54058841405667835, 14.81234591756537533, -8.371773407996172978 ) ) ;
#26266=CARTESIAN_POINT ( 'NONE',  ( -132.4896623150434607, 52.22616402022729432, -65.67901329176390846 ) ) ;
#26268=VECTOR ( 'NONE', #1870, 1000.000000000000000 ) ;
#26270=CARTESIAN_POINT ( 'NONE',  ( -94.77925136849377452, 29.13093715379787696, 11.40637257627832213 ) ) ;
#26273=ORIENTED_EDGE ( 'NONE', *, *, #19805, .F. ) ;
#26275=CARTESIAN_POINT ( 'NONE',  ( 183.1865184929770862, 80.75677158533825661, -77.77206949057716656 ) ) ;
#26279=CARTESIAN_POINT ( 'NONE',  ( -86.05211524933166345, -170.0000000000000000, -95.00000000000133582 ) ) ;
#26281=CARTESIAN_POINT ( 'NONE',  ( 85.67138972405899722, 19.09593469918315023, 29.75815417200340818 ) ) ;
#26282=CARTESIAN_POINT ( 'NONE',  ( 211.7634543339367781, 116.5654349622355141, -95.00000000000133582 ) ) ;
#26284=CARTESIAN_POINT ( 'NONE',  ( 42.03719354205839664, 9.783015072457470040, -36.09375209584154476 ) ) ;
#26285=CARTESIAN_POINT ( 'NONE',  ( 212.1700216741373879, 117.1889356120871071, 62.82458332484058872 ) ) ;
#26289=DIRECTION ( 'NONE',  ( 0.000000000000000000, 0.000000000000000000, 1.000000000000000000 ) ) ;
#26291=CARTESIAN_POINT ( 'NONE',  ( -15.08468253268400439, 7.472949889606721463, -44.86592640746919614 ) ) ;
#26292=B_SPLINE_CURVE_WITH_KNOTS ( 'NONE', 3,
 ( #6860, #41820, #63622, #31272, #52699, #4526, #15432, #47420, #58324, #10142, #53043, #40262, #67355, #24095, #67015, #8609, #45187, #19146, #33952, #13868, #35334, #23742, #66665, #7910, #24445, #1952, #40601, #45534, #7576, #34303, #34990, #17771, #55385, #50123, #18808, #1583, #34658, #39228, #7214, #29030, #50471, #39913, #2292, #55748, #13194, #62053, #45886, #61709, #13535, #18465 ),
 .UNSPECIFIED., .F., .F.,
 ( 4, 2, 2, 2, 2, 2, 2, 2, 2, 2, 2, 2, 2, 2, 2, 2, 2, 2, 2, 2, 2, 2, 2, 2, 4 ),
 ( 0.02688458561150008225, 0.02770990876165290925, 0.02853523191180573973, 0.03018587821211140762, 0.03183652451241707898, 0.03266184766256991640, 0.03348717081272276075, 0.03513781711302837313, 0.03678846341333399245, 0.03761378656348677435, 0.03843910971363955625, 0.03926443286379233816, 0.04008975601394512006, 0.04174040231425066305, 0.04256572546440344496, 0.04339104861455622686, 0.04421637176470900876, 0.04504169491486179067, 0.04586701806501457257, 0.04669234121516735447, 0.04834298751547297379, 0.04916831066562575570, 0.04999363381577853066, 0.05164428011608408753, 0.05329492641638965134 ),
 .UNSPECIFIED. ) ;
#26294=FACE_OUTER_BOUND ( 'NONE', #58559, .T. ) ;
#26295=EDGE_CURVE ( 'NONE', #37698, #18334, #32814, .T. ) ;
#26296=CARTESIAN_POINT ( 'NONE',  ( 92.20490818459941806, 22.47175429302963678, 69.09674679565556232 ) ) ;
#26297=CARTESIAN_POINT ( 'NONE',  ( 157.0336341255055856, 57.31169401067818825, -24.27963370867398751 ) ) ;
#26301=CARTESIAN_POINT ( 'NONE',  ( 35.65775178405255019, 7.951994368745591402, -76.46754290437888812 ) ) ;
#26304=CARTESIAN_POINT ( 'NONE',  ( -33.85171821065140563, 11.02091558840054653, -8.854690906676584206 ) ) ;
#26310=CARTESIAN_POINT ( 'NONE',  ( -189.2739965869453442, 107.1373753350176514, 10.69858136700815621 ) ) ;
#26312=CARTESIAN_POINT ( 'NONE',  ( -0.3249717932738299675, 6.518578686837485314, 38.10374936827246728 ) ) ;
#26314=CARTESIAN_POINT ( 'NONE',  ( 154.0281735872262061, 56.28213428456461287, -36.95677541368942087 ) ) ;
#26318=CARTESIAN_POINT ( 'NONE',  ( 175.0634607207818760, 74.11351956991630630, -12.40074815326527791 ) ) ;
#26323=CARTESIAN_POINT ( 'NONE',  ( -4.081377963939787357, 6.676029627840612157, -22.57677576480380921 ) ) ;
#26325=CARTESIAN_POINT ( 'NONE',  ( 197.6341357773624168, 98.74251867088339907, -14.44262121195315096 ) ) ;
#26326=CARTESIAN_POINT ( 'NONE',  ( -142.0521142816473059, 58.10507551552675665, 91.07448709527056963 ) ) ;
#26331=CYLINDRICAL_SURFACE ( 'NONE', #28330, 7.500000000000013323 ) ;
#26332=CARTESIAN_POINT ( 'NONE',  ( 160.9097745014958036, 61.67033591969549633, 16.73367501025392912 ) ) ;
#26333=DIRECTION ( 'NONE',  ( 0.000000000000000000, -1.000000000000000000, 0.000000000000000000 ) ) ;
#26337=CARTESIAN_POINT ( 'NONE',  ( 173.7263186949343776, 72.85225335320951956, 62.17071978413066091 ) ) ;
#26339=VERTEX_POINT ( 'NONE', #65527 ) ;
#26340=CARTESIAN_POINT ( 'NONE',  ( -109.7793173546316723, 36.75648380851384900, -42.23093992832588839 ) ) ;
#26341=CARTESIAN_POINT ( 'NONE',  ( 65.62848231372478836, 13.29388722724788430, -77.09954622703783400 ) ) ;
#26342=AXIS2_PLACEMENT_3D ( 'NONE', #7582, #8260, #40267 ) ;
#26343=CARTESIAN_POINT ( 'NONE',  ( -55.05276343752909440, 14.68156374112637863, 45.31732777293115788 ) ) ;
#26345=EDGE_LOOP ( 'NONE', ( #52381, #61044 ) ) ;
#26346=CARTESIAN_POINT ( 'NONE',  ( -173.9656771507954716, 88.06879734510549440, 45.82169460664104577 ) ) ;
#26348=CARTESIAN_POINT ( 'NONE',  ( 117.0069443446175512, 33.26475960880694061, -40.17220626710923170 ) ) ;
#26353=CARTESIAN_POINT ( 'NONE',  ( 140.2332932573541484, 45.41010019581509027, 67.83493447615286698 ) ) ;
#26355=CARTESIAN_POINT ( 'NONE',  ( -168.7150276173047700, 82.35404041280327192, 44.40934749284262750 ) ) ;
#26356=CARTESIAN_POINT ( 'NONE',  ( 131.6115093721024891, 41.25402743071398959, 56.69510300717567475 ) ) ;
#26358=ORIENTED_EDGE ( 'NONE', *, *, #43892, .T. ) ;
#26359=CARTESIAN_POINT ( 'NONE',  ( 45.89232972083999584, 10.36128169546909561, 6.802839851248819514 ) ) ;
#26362=CARTESIAN_POINT ( 'NONE',  ( -102.2801239173131052, 33.91021738430208643, -88.70367844590326456 ) ) ;
#26363=CARTESIAN_POINT ( 'NONE',  ( -62.43534356913686878, 16.78604954659376247, 92.86776280466541778 ) ) ;
#26365=CYLINDRICAL_SURFACE ( 'NONE', #10837, 7.500000000000013323 ) ;
#26366=CARTESIAN_POINT ( 'NONE',  ( -109.0191069781766657, 36.33811634972921922, 94.99999999999866418 ) ) ;
#26367=CARTESIAN_POINT ( 'NONE',  ( 185.5457097283155008, 84.70846743303870596, 16.01068182946670149 ) ) ;
#26374=CARTESIAN_POINT ( 'NONE',  ( -76.32456871438915869, 22.51591205926310479, 57.62160030318823090 ) ) ;
#26375=ADVANCED_FACE ( 'NONE', ( #66584 ), #18724, .F. ) ;
#26376=CARTESIAN_POINT ( 'NONE',  ( -95.61819996182572368, 29.52346081122276900, -39.06019279122138244 ) ) ;
#26377=B_SPLINE_CURVE_WITH_KNOTS ( 'NONE', 3,
 ( #53657, #10406, #30848, #47345, #37144, #52294, #20282, #4114, #37486, #25579, #57920, #68803, #9737, #20618, #10073, #47686, #31199, #52631, #53304, #4453, #16033, #15695, #15356, #36814, #48032, #31532, #58256, #64220, #26596, #4791, #69150, #20974, #58588, #31876, #69493, #58936, #54343, #54701, #49768, #33962, #32906, #65628, #60686, #12504, #5481, #55052 ),
 .UNSPECIFIED., .F., .F.,
 ( 4, 2, 2, 2, 2, 2, 2, 2, 2, 2, 2, 2, 2, 2, 2, 2, 2, 2, 2, 2, 2, 2, 4 ),
 ( 0.02584318557310392658, 0.02743529570732763587, 0.02823135077443949398, 0.02902740584155135556, 0.03061951597577504403, 0.03221162610999873943, 0.03380373624422242790, 0.03459979131133428948, 0.03539584637844615800, 0.03619190144555801958, 0.03698795651266988116, 0.03858006664689359738, 0.03937612171400545896, 0.04017217678111731360, 0.04096823184822917518, 0.04176428691534103677, 0.04335639704956475993, 0.04494850718378848309, 0.04654061731801220625, 0.04813272745223592941, 0.04892878251934780487, 0.04972483758645968033, 0.05131694772068347982 ),
 .UNSPECIFIED. ) ;
#26378=CARTESIAN_POINT ( 'NONE',  ( 59.08638499266955080, 11.79550614876701786, -76.45822759883306219 ) ) ;
#26381=CARTESIAN_POINT ( 'NONE',  ( 17.73567516211396722, 7.577454475141605528, 30.25539365111569978 ) ) ;
#26382=CARTESIAN_POINT ( 'NONE',  ( 160.9097745014957752, 61.67033591969547501, -63.79997676113709559 ) ) ;
#26383=VECTOR ( 'NONE', #39548, 1000.000000000000000 ) ;
#26385=CARTESIAN_POINT ( 'NONE',  ( -73.10694748374054086, 20.28107308417881427, 59.70508575492568326 ) ) ;
#26386=CARTESIAN_POINT ( 'NONE',  ( -172.3018509397888636, 86.22053936367350957, 72.63294570045411547 ) ) ;
#26391=CARTESIAN_POINT ( 'NONE',  ( -31.43908319763711390, 10.61114334766715928, 18.37190381572551701 ) ) ;
#26401=LINE ( 'NONE', #43241, #3175 ) ;
#26404=DIRECTION ( 'NONE',  ( 0.000000000000000000, 0.000000000000000000, 1.000000000000000000 ) ) ;
#26406=CARTESIAN_POINT ( 'NONE',  ( -78.66644367742111399, -170.0000000000000000, -8.270900041254199309 ) ) ;
#26408=EDGE_LOOP ( 'NONE', ( #53608, #14949, #45531, #52922 ) ) ;
#26409=CARTESIAN_POINT ( 'NONE',  ( 157.4703587214989113, 57.65129005721575339, -24.27963370867398396 ) ) ;
#26411=CARTESIAN_POINT ( 'NONE',  ( -166.2028193222418793, 79.74385139484274987, -18.27775044557155582 ) ) ;
#26422=AXIS2_PLACEMENT_3D ( 'NONE', #30265, #66183, #45744 ) ;
#26424=CARTESIAN_POINT ( 'NONE',  ( 9.416603677636258496, 6.380307115728825806, -46.98271897290301524 ) ) ;
#26425=CARTESIAN_POINT ( 'NONE',  ( -179.2262621278718200, 94.19039042964669761, 69.55156446434544648 ) ) ;
#26427=CARTESIAN_POINT ( 'NONE',  ( 127.6144785300460711, 37.78099129859916872, 59.68968456894913288 ) ) ;
#26431=VECTOR ( 'NONE', #14575, 1000.000000000000000 ) ;
#26438=CARTESIAN_POINT ( 'NONE',  ( 103.0026233023292832, 25.67408295205787994, -45.44575129055834850 ) ) ;
#26439=CARTESIAN_POINT ( 'NONE',  ( -24.70354720400823823, 8.582324684301861240, 41.05222872378217147 ) ) ;
#26446=CARTESIAN_POINT ( 'NONE',  ( -125.8938041572051105, 47.69968343338781835, -34.91370389823391918 ) ) ;
#26448=CARTESIAN_POINT ( 'NONE',  ( 133.6288034103010318, 41.28708886999551453, 2.665790248531665352 ) ) ;
#26449=CARTESIAN_POINT ( 'NONE',  ( -154.7998111145352311, 68.80117179139330119, 6.040483385297001462 ) ) ;
#26450=CARTESIAN_POINT ( 'NONE',  ( -118.6302575928420140, 43.07263081214307476, -67.37114707264666436 ) ) ;
#26451=CARTESIAN_POINT ( 'NONE',  ( -125.8938041572051389, -170.0000000000000000, 64.96449846362078517 ) ) ;
#26452=CARTESIAN_POINT ( 'NONE',  ( -78.66644367742111399, 23.39876645725286863, 72.26275173013684139 ) ) ;
#26453=CARTESIAN_POINT ( 'NONE',  ( 44.33335936148068868, 10.11981604950586622, -91.15432397735798986 ) ) ;
#26455=CARTESIAN_POINT ( 'NONE',  ( 8.000000000000007105, 249.8719672152120381, -95.00000000000133582 ) ) ;
#26459=EDGE_CURVE ( 'NONE', #35148, #30648, #6080, .T. ) ;
#26460=CARTESIAN_POINT ( 'NONE',  ( 22.51849650178394668, 7.817407610814550267, -66.54469324731199720 ) ) ;
#26462=DIRECTION ( 'NONE',  ( -0.000000000000000000, 1.000000000000000000, -0.000000000000000000 ) ) ;
#26463=CARTESIAN_POINT ( 'NONE',  ( 69.73342236697681074, 14.33173522011652423, -19.74742079103577552 ) ) ;
#26465=CARTESIAN_POINT ( 'NONE',  ( -50.14523569787234436, 14.45648954445650780, -75.25403677891537768 ) ) ;
#26466=DIRECTION ( 'NONE',  ( -0.000000000000000000, 1.000000000000000000, -0.000000000000000000 ) ) ;
#26468=ORIENTED_EDGE ( 'NONE', *, *, #8595, .T. ) ;
#26470=CARTESIAN_POINT ( 'NONE',  ( 66.30567821786758032, 13.45988234822861251, -36.47644505420841909 ) ) ;
#26472=CARTESIAN_POINT ( 'NONE',  ( 181.5278511219383688, 80.49241794770389902, 83.00548516787387143 ) ) ;
#26473=CARTESIAN_POINT ( 'NONE',  ( -169.8972248494843029, 85.08697738648014308, -8.580859100646367921 ) ) ;
#26475=CARTESIAN_POINT ( 'NONE',  ( 65.02425260195224155, 14.18239149161751733, -89.67225535254971192 ) ) ;
#26479=CARTESIAN_POINT ( 'NONE',  ( -15.31363169557738679, 7.494880774892001440, 63.97268137111493047 ) ) ;
#26480=CARTESIAN_POINT ( 'NONE',  ( 204.6977192012829505, 108.0580384837234931, 2.363170148305746565 ) ) ;
#26482=CARTESIAN_POINT ( 'NONE',  ( -85.97236666747350853, 26.33140062794030811, -94.54850636960576082 ) ) ;
#26483=CARTESIAN_POINT ( 'NONE',  ( 42.71504753277075395, 8.863481902720387495, -9.542259995937373063 ) ) ;
#26487=EDGE_LOOP ( 'NONE', ( #18280, #549, #49916, #22838 ) ) ;
#26492=CARTESIAN_POINT ( 'NONE',  ( 150.0889146124742979, 52.13243511955544562, 8.708654298008204009 ) ) ;
#26493=CARTESIAN_POINT ( 'NONE',  ( -13.95225484952729822, 8.378029245909427658, 86.96665100290213957 ) ) ;
#26494=EDGE_CURVE ( 'NONE', #33732, #4217, #46834, .T. ) ;
#26499=VERTEX_POINT ( 'NONE', #8870 ) ;
#26500=CARTESIAN_POINT ( 'NONE',  ( 37.78224319576848700, 9.218056077237706702, 83.77244032528042794 ) ) ;
#26502=DIRECTION ( 'NONE',  ( 0.000000000000000000, 0.000000000000000000, 1.000000000000000000 ) ) ;
#26504=CARTESIAN_POINT ( 'NONE',  ( -60.97011009284707939, 16.34812508431679134, -64.92641111431414913 ) ) ;
#26505=CARTESIAN_POINT ( 'NONE',  ( -7.825402957745085430, 6.891034867348157178, 18.27103044898354511 ) ) ;
#26506=CARTESIAN_POINT ( 'NONE',  ( 35.65775178405256440, 7.951994368745586961, -22.77844172345153595 ) ) ;
#26507=CARTESIAN_POINT ( 'NONE',  ( 175.5429257635130966, 74.57009623370761631, -38.64485354243735316 ) ) ;
#26509=CARTESIAN_POINT ( 'NONE',  ( 86.62931800182293784, 19.42108912189597092, 29.71208757247930521 ) ) ;
#26514=DIRECTION ( 'NONE',  ( 0.000000000000000000, 0.000000000000000000, 1.000000000000000000 ) ) ;
#26516=CARTESIAN_POINT ( 'NONE',  ( 203.9228889538744625, 106.9879579748727991, 29.23739942787593193 ) ) ;
#26517=CARTESIAN_POINT ( 'NONE',  ( 79.43147385343415579, 17.08938890961555046, 88.76640830538551086 ) ) ;
#26520=VERTEX_POINT ( 'NONE', #14815 ) ;
#26521=EDGE_LOOP ( 'NONE', ( #54947, #46379 ) ) ;
#26526=CARTESIAN_POINT ( 'NONE',  ( -188.8754233303960746, 108.3048424661242137, 94.99999999999866418 ) ) ;
#26531=CARTESIAN_POINT ( 'NONE',  ( -34.06637338149494809, 11.05895377318623218, 57.53204137510643790 ) ) ;
#26533=CARTESIAN_POINT ( 'NONE',  ( 156.5977259323288990, 56.97512126940428345, -77.93088349121646274 ) ) ;
#26536=CARTESIAN_POINT ( 'NONE',  ( -156.9910258076866114, 70.79617246506499839, -42.88647977470814965 ) ) ;
#26540=CARTESIAN_POINT ( 'NONE',  ( 69.36287815987334682, 15.27486453472191563, -20.37900260559285215 ) ) ;
#26541=CARTESIAN_POINT ( 'NONE',  ( -80.56139928459658961, 24.13290941644246601, -35.35486284265729040 ) ) ;
#26542=CARTESIAN_POINT ( 'NONE',  ( 157.4703587214989113, 57.65129005721576050, 71.25401806271709404 ) ) ;
#26543=CARTESIAN_POINT ( 'NONE',  ( -154.7826623253030505, 70.14150242829518334, 6.039344387218765320 ) ) ;
#26546=CARTESIAN_POINT ( 'NONE',  ( 188.0141161196705752, 85.90515114331880397, -40.84309500477795751 ) ) ;
#26548=CARTESIAN_POINT ( 'NONE',  ( -150.1466931226166537, 66.04887306281342774, 84.43241108380165372 ) ) ;
#26550=ORIENTED_EDGE ( 'NONE', *, *, #58407, .F. ) ;
#26552=CARTESIAN_POINT ( 'NONE',  ( -155.7457403566965581, 71.01814553754121562, -19.66200801844618695 ) ) ;
#26553=CARTESIAN_POINT ( 'NONE',  ( 32.09610685027467980, 8.582590950734839907, -44.83291474007333477 ) ) ;
#26554=CARTESIAN_POINT ( 'NONE',  ( -35.99019277275120032, 10.38248800679342132, 70.54226521342960154 ) ) ;
#26555=CARTESIAN_POINT ( 'NONE',  ( -152.5067928559255108, 66.76529500553620267, -22.35681670066612270 ) ) ;
#26557=CARTESIAN_POINT ( 'NONE',  ( 36.09137906183517686, 8.001963043161767430, 57.52411210887189696 ) ) ;
#26559=CARTESIAN_POINT ( 'NONE',  ( -7.330587818645180498, 7.867004275019547244, -35.41807073194381417 ) ) ;
#26562=CARTESIAN_POINT ( 'NONE',  ( -81.00507684688697907, 23.22613445438386037, -35.48540021743968254 ) ) ;
#26565=CARTESIAN_POINT ( 'NONE',  ( 13.37708032728285978, 7.441924986912761497, 3.564073605040367632 ) ) ;
#26570=CARTESIAN_POINT ( 'NONE',  ( 178.1999009735082495, 75.73911533785330619, 43.73541319493209301 ) ) ;
#26571=CARTESIAN_POINT ( 'NONE',  ( -132.2352756077771687, 50.81350938245627447, -46.42641520675586264 ) ) ;
#26572=CARTESIAN_POINT ( 'NONE',  ( -105.4487797565983982, 35.55724615608639283, -49.32840306322937352 ) ) ;
#26577=ORIENTED_EDGE ( 'NONE', *, *, #9927, .T. ) ;
#26578=CARTESIAN_POINT ( 'NONE',  ( -24.33435124463267485, 8.532637995283108623, -13.55733912248031992 ) ) ;
#26579=CARTESIAN_POINT ( 'NONE',  ( 197.3119541548906852, 98.33923235143193153, 8.549100434825948724 ) ) ;
#26586=DIRECTION ( 'NONE',  ( 0.000000000000000000, 0.000000000000000000, 1.000000000000000000 ) ) ;
#26590=CARTESIAN_POINT ( 'NONE',  ( 93.33480479917542993, 21.81892021443993812, -39.92446842644995542 ) ) ;
#26592=EDGE_CURVE ( 'NONE', #16384, #21098, #56703, .T. ) ;
#26596=CARTESIAN_POINT ( 'NONE',  ( -118.6849742182705540, 41.92701402439732306, -13.48273187576209153 ) ) ;
#26598=CARTESIAN_POINT ( 'NONE',  ( -180.6009936245623635, 95.85948119829089364, -14.73603367312734846 ) ) ;
#26603=CARTESIAN_POINT ( 'NONE',  ( 60.63380853769238144, 13.16344960520422092, 3.352510954306818558 ) ) ;
#26606=CARTESIAN_POINT ( 'NONE',  ( 55.53366667017859015, 12.08690898290841709, 91.85515229178750474 ) ) ;
#26607=CARTESIAN_POINT ( 'NONE',  ( -61.75956139478098095, 16.58288496614413177, -19.23791488395762528 ) ) ;
#26608=CARTESIAN_POINT ( 'NONE',  ( 79.19132716134491545, 17.01584750883626995, -17.47194662292698553 ) ) ;
#26610=CARTESIAN_POINT ( 'NONE',  ( -130.1938957973835613, 50.61368074696265751, -75.42079035589019043 ) ) ;
#26613=CARTESIAN_POINT ( 'NONE',  ( -97.49219489034499020, 30.41416107059309937, -75.15255229431038231 ) ) ;
#26614=ORIENTED_EDGE ( 'NONE', *, *, #45495, .F. ) ;
#26619=CARTESIAN_POINT ( 'NONE',  ( -78.66644367742111399, 22.32174330031318377, 57.26275173013680586 ) ) ;
#26620=CARTESIAN_POINT ( 'NONE',  ( -165.6393662153604964, 79.16886183052817216, -41.60625904825717214 ) ) ;
#26625=CARTESIAN_POINT ( 'NONE',  ( 108.3942953861066627, 29.14039925067521608, -77.55066643792520154 ) ) ;
#26626=CARTESIAN_POINT ( 'NONE',  ( -73.10086105983762650, 21.34631349770503306, 42.96954990387450835 ) ) ;
#26627=CARTESIAN_POINT ( 'NONE',  ( 83.38067517854670996, 18.33799117207140128, 30.44781216307082872 ) ) ;
#26629=CARTESIAN_POINT ( 'NONE',  ( 68.63585058221465829, 15.08566240483130727, -48.21148126164135306 ) ) ;
#26630=CARTESIAN_POINT ( 'NONE',  ( 40.38495044702529668, 9.554194848483446023, -50.57113278200800721 ) ) ;
#26635=CARTESIAN_POINT ( 'NONE',  ( -13.78293860383719327, 7.352367295275509029, -38.33539452421117488 ) ) ;
#26638=CARTESIAN_POINT ( 'NONE',  ( 91.50468583833759340, 22.21368636549395958, 58.33610043527986733 ) ) ;
#26639=CARTESIAN_POINT ( 'NONE',  ( 150.8925291903903485, 52.71218673668931842, -20.42211489697474036 ) ) ;
#26640=CARTESIAN_POINT ( 'NONE',  ( 34.82939798935585429, 8.870855050008907838, 16.53448816255987097 ) ) ;
#26643=CARTESIAN_POINT ( 'NONE',  ( 111.7895558633182702, 30.71656550562548205, -89.76251668449653209 ) ) ;
#26646=ORIENTED_EDGE ( 'NONE', *, *, #7947, .T. ) ;
#26647=CARTESIAN_POINT ( 'NONE',  ( 59.73312635112158375, 12.96464920523511744, 57.39663913394880268 ) ) ;
#26648=DIRECTION ( 'NONE',  ( 0.000000000000000000, 0.000000000000000000, 1.000000000000000000 ) ) ;
#26650=CARTESIAN_POINT ( 'NONE',  ( -3.244108878396733342, 6.635632329121485817, 43.57411160445457199 ) ) ;
#26651=CARTESIAN_POINT ( 'NONE',  ( -94.79534239005248253, 29.13842790650041792, -16.21322624192772111 ) ) ;
#26652=CARTESIAN_POINT ( 'NONE',  ( 93.99303524761531037, 23.14219721139955865, 89.43772427296207184 ) ) ;
#26655=CYLINDRICAL_SURFACE ( 'NONE', #1481, 7.500000000000020428 ) ;
#26656=CARTESIAN_POINT ( 'NONE',  ( -132.2199390322348620, 50.80243550247268303, 15.33512913661918020 ) ) ;
#26657=CARTESIAN_POINT ( 'NONE',  ( -109.6752351740181837, 37.84903014964775281, 66.14036768415373047 ) ) ;
#26659=CARTESIAN_POINT ( 'NONE',  ( -131.2955621888335429, 51.38237199780171238, -47.63902616610417340 ) ) ;
#26662=CARTESIAN_POINT ( 'NONE',  ( 93.92910382125421620, 22.04227458821882024, 65.79627513581792186 ) ) ;
#26665=CARTESIAN_POINT ( 'NONE',  ( -149.3419259515906674, 64.03919805169483936, 84.40698907434087062 ) ) ;
#26671=CARTESIAN_POINT ( 'NONE',  ( 81.05403189674299824, 18.64820877954959499, 5.327265512142696835 ) ) ;
#26673=CARTESIAN_POINT ( 'NONE',  ( 158.3516718297675538, 59.61984652322052369, 2.603653821445219840 ) ) ;
#26677=AXIS2_PLACEMENT_3D ( 'NONE', #6700, #11269, #59457 ) ;
#26679=CARTESIAN_POINT ( 'NONE',  ( 174.4912080999799002, 73.57140295268875718, 67.23920894112048074 ) ) ;
#26682=CARTESIAN_POINT ( 'NONE',  ( -106.6940984894958149, 35.07986071359380986, -48.59687766299582279 ) ) ;
#26683=CARTESIAN_POINT ( 'NONE',  ( 64.93495251696903381, 13.12601614965099195, -77.31956637496439555 ) ) ;
#26685=CARTESIAN_POINT ( 'NONE',  ( 133.8566784816069060, 42.60093787723654657, -62.86786152285933582 ) ) ;
#26687=CARTESIAN_POINT ( 'NONE',  ( 151.7783534118502189, 54.60545177578661935, 14.95502099461759293 ) ) ;
#26688=ORIENTED_EDGE ( 'NONE', *, *, #56614, .T. ) ;
#26690=DIRECTION ( 'NONE',  ( -0.000000000000000000, 1.000000000000000000, -0.000000000000000000 ) ) ;
#26691=CARTESIAN_POINT ( 'NONE',  ( 117.6853163455684665, 33.60747889659833021, -42.36141487299401120 ) ) ;
#26695=CARTESIAN_POINT ( 'NONE',  ( -170.2747214445849693, 84.01465441107040988, 45.27347971088749290 ) ) ;
#26696=CARTESIAN_POINT ( 'NONE',  ( -37.07086358537074489, 10.58360809068250141, -64.68456555099868410 ) ) ;
#26698=CARTESIAN_POINT ( 'NONE',  ( 43.14669449386823175, 9.942681284149131216, 17.08585798182755511 ) ) ;
#26699=EDGE_LOOP ( 'NONE', ( #9310, #57928, #46994, #22955 ) ) ;
#26703=CARTESIAN_POINT ( 'NONE',  ( -49.04224900313972313, 13.15187391237128800, 87.00896093370914741 ) ) ;
#26705=CARTESIAN_POINT ( 'NONE',  ( -154.2585856850056132, 68.31650218414625897, -74.96551107100964373 ) ) ;
#26707=CARTESIAN_POINT ( 'NONE',  ( 70.21064619801208551, 14.45739791461312507, 88.85860685527731562 ) ) ;
#26709=DIRECTION ( 'NONE',  ( 0.000000000000000000, 0.000000000000000000, 1.000000000000000000 ) ) ;
#26710=CARTESIAN_POINT ( 'NONE',  ( -131.6133495896317243, 50.37677745548730712, 69.82229305692996491 ) ) ;
#26716=CARTESIAN_POINT ( 'NONE',  ( -74.18622060908364801, 21.73430079572372975, 58.72855139418935977 ) ) ;
#26717=CARTESIAN_POINT ( 'NONE',  ( 183.3913492984167419, 80.96922346472075560, 29.66909328504869237 ) ) ;
#26718=CARTESIAN_POINT ( 'NONE',  ( 42.48820792780865219, 9.847387255477759282, -23.11522967762586234 ) ) ;
#26720=CARTESIAN_POINT ( 'NONE',  ( -73.10694748374055507, 20.28107308417883559, 6.015984573998315099 ) ) ;
#26721=CARTESIAN_POINT ( 'NONE',  ( -119.5563837756079835, 43.64229894412653721, 69.00696829185407921 ) ) ;
#26722=CARTESIAN_POINT ( 'NONE',  ( 8.000000000000007105, 249.8719672152120381, -95.00000000000133582 ) ) ;
#26730=CARTESIAN_POINT ( 'NONE',  ( -25.07901552294942960, 9.649193085547778992, -65.67922684374194375 ) ) ;
#26731=CARTESIAN_POINT ( 'NONE',  ( 56.19211641164836379, 11.19288081156168424, -46.34333600376012896 ) ) ;
#26733=CARTESIAN_POINT ( 'NONE',  ( 157.4703587214989398, -170.0000000000000000, -51.12418429913766005 ) ) ;
#26735=DIRECTION ( 'NONE',  ( -0.000000000000000000, 1.000000000000000000, -0.000000000000000000 ) ) ;
#26736=EDGE_LOOP ( 'NONE', ( #26550, #10533, #28170, #67433 ) ) ;
#26737=ORIENTED_EDGE ( 'NONE', *, *, #43705, .F. ) ;
#26738=CARTESIAN_POINT ( 'NONE',  ( 22.25657943806483274, -170.0000000000000000, 94.99999999999866418 ) ) ;
#26740=CARTESIAN_POINT ( 'NONE',  ( 207.8675797643809062, 110.7908513421271550, 16.67352291382450957 ) ) ;
#26741=CARTESIAN_POINT ( 'NONE',  ( -142.1332311300252798, 59.44822332309653490, 36.82517692171189339 ) ) ;
#26742=CARTESIAN_POINT ( 'NONE',  ( 57.08336938683662964, 11.37442068895389014, 68.77294810484833931 ) ) ;
#26748=DIRECTION ( 'NONE',  ( -0.000000000000000000, 1.000000000000000000, -0.000000000000000000 ) ) ;
#26752=CARTESIAN_POINT ( 'NONE',  ( 86.62931800182293784, -170.0000000000000000, 37.21208757247931942 ) ) ;
#26753=CARTESIAN_POINT ( 'NONE',  ( -167.6386155194958576, 81.22597462185134987, -10.22418588222271474 ) ) ;
#26756=CARTESIAN_POINT ( 'NONE',  ( 10.95373880336383543, 7.400264897461164004, 85.46052647922621759 ) ) ;
#26759=CARTESIAN_POINT ( 'NONE',  ( -98.67723517640902742, 30.98797878696539598, 71.44587722449948330 ) ) ;
#26760=EDGE_LOOP ( 'NONE', ( #62287, #42499, #51598, #14867 ) ) ;
#26768=CARTESIAN_POINT ( 'NONE',  ( -119.2949674747224975, 43.48097822533564738, 14.87828489523786857 ) ) ;
#26769=CARTESIAN_POINT ( 'NONE',  ( -180.6011569556094969, 95.85968111394261371, 64.53619258438885709 ) ) ;
#26771=CARTESIAN_POINT ( 'NONE',  ( 126.5710838895481345, 37.19597237024179748, 62.05496881366955364 ) ) ;
#26773=B_SPLINE_CURVE_WITH_KNOTS ( 'NONE', 3,
 ( #18526, #18873, #40321, #67083, #61766, #60733, #12553, #39631, #60393, #29087, #3048, #13592, #29424, #24156, #2354, #45247, #39976, #35052, #56494, #65679, #34013, #51230 ),
 .UNSPECIFIED., .F., .F.,
 ( 4, 2, 2, 2, 2, 2, 2, 2, 2, 2, 4 ),
 ( 9.309503074677274191E-17, 0.001318139496345222808, 0.001977209244517771219, 0.002636278992690319848, 0.003954418489035408865, 0.005272557985380498316, 0.005931627733553053450, 0.006590697481725609451, 0.007908836978070743137, 0.009226976474415879426, 0.01054511597076101224 ),
 .UNSPECIFIED. ) ;
#26775=CARTESIAN_POINT ( 'NONE',  ( 149.9838583332408177, 52.05699766415859386, 36.38096985813713502 ) ) ;
#26779=CARTESIAN_POINT ( 'NONE',  ( 86.62931800182293784, -170.0000000000000000, -97.01066537983908233 ) ) ;
#26780=CARTESIAN_POINT ( 'NONE',  ( -25.35398647985413589, 8.671412257862211703, 33.32529752127744871 ) ) ;
#26781=CARTESIAN_POINT ( 'NONE',  ( -142.8556048422594813, 60.01994222009838609, -65.68255109197973240 ) ) ;
#26783=DIRECTION ( 'NONE',  ( 1.000000000000000000, 0.000000000000000000, 0.000000000000000000 ) ) ;
#26787=CARTESIAN_POINT ( 'NONE',  ( -120.6420427933462207, 44.31795133507804962, -47.77366304952625597 ) ) ;
#26788=CARTESIAN_POINT ( 'NONE',  ( -85.12122836439577611, 25.97531040437156946, 14.92485516287107217 ) ) ;
#26792=CARTESIAN_POINT ( 'NONE',  ( -78.24476289916013627, 22.16113887290258333, -88.80455181264525777 ) ) ;
#26793=DIRECTION ( 'NONE',  ( -0.000000000000000000, 1.000000000000000000, -0.000000000000000000 ) ) ;
#26794=CARTESIAN_POINT ( 'NONE',  ( 160.4963793545269368, 60.04225845346905288, 3.187966924173012195 ) ) ;
#26795=CARTESIAN_POINT ( 'NONE',  ( 45.79927714077020795, 10.34658019240735705, -92.88875141923965373 ) ) ;
#26800=ORIENTED_EDGE ( 'NONE', *, *, #64624, .T. ) ;
#26801=CARTESIAN_POINT ( 'NONE',  ( 18.43272992546528855, 7.606837839440253823, -62.84086927382109877 ) ) ;
#26802=CARTESIAN_POINT ( 'NONE',  ( 111.5555719986353864, 30.60523913099746451, 83.38823749445282374 ) ) ;
#26805=CARTESIAN_POINT ( 'NONE',  ( -190.6985136298601731, 109.1272424661242582, 94.99999999999866418 ) ) ;
#26806=CARTESIAN_POINT ( 'NONE',  ( 210.1064829626521941, 115.8779605595242970, -92.30285115593483170 ) ) ;
#26807=CARTESIAN_POINT ( 'NONE',  ( 8.000000000000007105, 249.8719672152120381, -95.00000000000133582 ) ) ;
#26810=ORIENTED_EDGE ( 'NONE', *, *, #34660, .F. ) ;
#26812=CARTESIAN_POINT ( 'NONE',  ( 174.3147410850615131, 73.40482959803648555, 93.74842768471017962 ) ) ;
#26817=ORIENTED_EDGE ( 'NONE', *, *, #42848, .F. ) ;
#26820=CARTESIAN_POINT ( 'NONE',  ( 90.91356992076215704, 21.99794663086828805, 16.52815484461689266 ) ) ;
#26821=CARTESIAN_POINT ( 'NONE',  ( -10.23402954931276376, 7.059791383763807104, 71.56709959516479103 ) ) ;
#26822=CARTESIAN_POINT ( 'NONE',  ( 212.1734186221016500, 119.0499290057855291, 10.55534217174901812 ) ) ;
#26824=CARTESIAN_POINT ( 'NONE',  ( 46.84183314611287585, 9.494161546644496852, -15.29600076990992541 ) ) ;
#26825=CARTESIAN_POINT ( 'NONE',  ( 208.5889601154908917, 111.8333159387241693, -23.40665082623701920 ) ) ;
#26826=FACE_BOUND ( 'NONE', #14343, .T. ) ;
#26827=CARTESIAN_POINT ( 'NONE',  ( 159.2325040199867487, 60.31699144791976153, 71.09951541772399253 ) ) ;
#26828=EDGE_CURVE ( 'NONE', #33435, #19003, #52196, .T. ) ;
#26832=CARTESIAN_POINT ( 'NONE',  ( 88.28889510440060917, 21.05995314109331318, -36.00360628347565495 ) ) ;
#26833=ADVANCED_FACE ( 'NONE', ( #60530 ), #55240, .F. ) ;
#26834=DIRECTION ( 'NONE',  ( -0.000000000000000000, 1.000000000000000000, -0.000000000000000000 ) ) ;
#26836=CARTESIAN_POINT ( 'NONE',  ( 151.6351261592328683, 53.25263237790402826, 14.78337374240360447 ) ) ;
#26838=B_SPLINE_CURVE_WITH_KNOTS ( 'NONE', 3,
 ( #69514, #21335, #58276, #26625, #43129, #53686, #31901, #64251, #54014, #42448, #20646, #25935, #5506, #5844, #42107, #63906, #68497, #20301, #37168, #58616, #15031, #16059, #53332, #4478, #48386, #36489, #58965, #47368, #64601, #26959, #47715, #10779, #68823, #21680, #16409, #63565, #37866, #15376, #59314, #36837 ),
 .UNSPECIFIED., .F., .F.,
 ( 4, 2, 2, 2, 2, 2, 2, 2, 2, 2, 2, 2, 2, 2, 2, 2, 2, 2, 2, 4 ),
 ( 0.02472759712254454789, 0.02626001169882803687, 0.02779242627511152933, 0.02932484085139501831, 0.03009104813953675586, 0.03085725542767849341, 0.03238967000396194423, 0.03315587729210369566, 0.03392208458024545403, 0.03545449915652894302, 0.03698691373281243200, 0.03851932830909592098, 0.04005174288537940996, 0.04158415746166289895, 0.04311657203794638793, 0.04464898661422987691, 0.04541519390237162834, 0.04618140119051337977, 0.04771381576679688957, 0.04924623034308040631 ),
 .UNSPECIFIED. ) ;
#26844=CARTESIAN_POINT ( 'NONE',  ( 40.72999892410475553, 9.601203897218297811, 83.71404436111639313 ) ) ;
#26846=CARTESIAN_POINT ( 'NONE',  ( 103.1567541746301373, 25.73937982110322409, 34.60279117723898423 ) ) ;
#26847=ADVANCED_FACE ( 'NONE', ( #32751 ), #56290, .F. ) ;
#26849=CARTESIAN_POINT ( 'NONE',  ( -56.02358673658414290, 14.94347049174936437, -77.01342999705896375 ) ) ;
#26850=CARTESIAN_POINT ( 'NONE',  ( -2.172839205444464294, 7.595638683704372340, 5.816862989022147268 ) ) ;
#26853=CARTESIAN_POINT ( 'NONE',  ( 164.9036507189915710, 63.66930857265032273, 91.66500914631893693 ) ) ;
#26854=CARTESIAN_POINT ( 'NONE',  ( 93.32502112557682494, 21.81526022999038972, 33.79663101393975921 ) ) ;
#26856=CARTESIAN_POINT ( 'NONE',  ( 105.4134760436918157, 27.80903124201757493, -10.81885116605370989 ) ) ;
#26859=CARTESIAN_POINT ( 'NONE',  ( -1.298947065946361112, 7.560777410219321482, 94.99999999999866418 ) ) ;
#26861=CARTESIAN_POINT ( 'NONE',  ( -83.52199252699273302, 25.31691946248441383, 85.88269580995972774 ) ) ;
#26864=ORIENTED_EDGE ( 'NONE', *, *, #56195, .F. ) ;
#26867=CARTESIAN_POINT ( 'NONE',  ( 110.2429982417149574, 29.99119854320844425, -62.76698815611734972 ) ) ;
#26869=CARTESIAN_POINT ( 'NONE',  ( -190.6985136298602015, 109.1272424661243434, -37.65993730791821292 ) ) ;
#26871=CARTESIAN_POINT ( 'NONE',  ( -34.74023699876257609, 11.17830703027882855, 57.80909291234753056 ) ) ;
#26873=CARTESIAN_POINT ( 'NONE',  ( 150.2794558856211040, 52.26944788078752424, -68.26897188648571557 ) ) ;
#26879=CARTESIAN_POINT ( 'NONE',  ( 69.83617901654359628, 15.39919709983077389, -19.50531207266840639 ) ) ;
#26880=CARTESIAN_POINT ( 'NONE',  ( -84.21836162213173793, 25.60181819557221417, -47.68121567810126038 ) ) ;
#26882=CARTESIAN_POINT ( 'NONE',  ( -156.8728827992624986, 72.05711009495561825, 9.933813873631594404 ) ) ;
#26885=CARTESIAN_POINT ( 'NONE',  ( 23.24028701062093916, 6.853614888934261629, 38.49265168136174253 ) ) ;
#26886=CARTESIAN_POINT ( 'NONE',  ( -152.9826564381572211, 68.52733426032347097, 85.25801961117713290 ) ) ;
#26890=CARTESIAN_POINT ( 'NONE',  ( -13.78293860383719505, 7.352367295275509029, 15.35370665671618973 ) ) ;
#26891=CARTESIAN_POINT ( 'NONE',  ( 86.62931800182292363, 20.48449268398425716, -89.51066537983906812 ) ) ;
#26892=CARTESIAN_POINT ( 'NONE',  ( -38.55214349681827457, 10.86754840574841552, 62.13239515233281196 ) ) ;
#26894=DIRECTION ( 'NONE',  ( -0.000000000000000000, 1.000000000000000000, -0.000000000000000000 ) ) ;
#26895=ORIENTED_EDGE ( 'NONE', *, *, #38675, .F. ) ;
#26897=CARTESIAN_POINT ( 'NONE',  ( -55.05276343752910151, 14.68156374112636620, 3.472777182467474244 ) ) ;
#26899=CARTESIAN_POINT ( 'NONE',  ( 19.54326199789021601, 7.657220834818549093, 4.173189189204250304 ) ) ;
#26900=CARTESIAN_POINT ( 'NONE',  ( 110.2429982417149432, 28.88204397445229432, 17.76666361527367499 ) ) ;
#26902=CARTESIAN_POINT ( 'NONE',  ( -86.17927978631389863, 25.32700573188344251, -42.60343115903025790 ) ) ;
#26903=CARTESIAN_POINT ( 'NONE',  ( 181.0840389613909736, 78.60582251573003987, 44.30859410551141764 ) ) ;
#26905=CARTESIAN_POINT ( 'NONE',  ( 13.14401442664831166, 6.430459733718342896, -62.84079615501572391 ) ) ;
#26912=CARTESIAN_POINT ( 'NONE',  ( -132.9409505933031994, 51.31241517713431222, -45.03336911783197394 ) ) ;
#26913=CARTESIAN_POINT ( 'NONE',  ( 46.13320811200730276, 9.380653113584049407, -73.30836824486340220 ) ) ;
#26915=CARTESIAN_POINT ( 'NONE',  ( 182.7686108735401262, 81.77235358504611895, -51.04580610545474428 ) ) ;
#26918=CARTESIAN_POINT ( 'NONE',  ( -31.43908319763710679, 9.591432048623756756, -8.472646774738153752 ) ) ;
#26919=CARTESIAN_POINT ( 'NONE',  ( 173.7154822107653445, 71.46636395518601148, 89.08536180762163781 ) ) ;
#26922=CARTESIAN_POINT ( 'NONE',  ( 115.7746371641014775, 31.52600568297704697, 69.04386463718626032 ) ) ;
#26925=CARTESIAN_POINT ( 'NONE',  ( 127.4669243510812890, 38.85312661085428232, -66.40869171650194858 ) ) ;
#26927=CARTESIAN_POINT ( 'NONE',  ( 139.7883986595928434, 46.32091287009617986, 59.25842257727051532 ) ) ;
#26930=CARTESIAN_POINT ( 'NONE',  ( -102.2801239173131194, 32.78103895658057354, 45.51907450641513009 ) ) ;
#26931=DIRECTION ( 'NONE',  ( -0.000000000000000000, 1.000000000000000000, -0.000000000000000000 ) ) ;
#26938=CARTESIAN_POINT ( 'NONE',  ( 181.0840389613909736, 80.03940679743416808, -78.06960825634331513 ) ) ;
#26939=CARTESIAN_POINT ( 'NONE',  ( -165.6397095829521788, 80.60756690931940227, -69.66568759875811168 ) ) ;
#26940=CARTESIAN_POINT ( 'NONE',  ( -142.0685766576042113, 58.11789490499572963, -41.20363413018768028 ) ) ;
#26945=CARTESIAN_POINT ( 'NONE',  ( -129.6001310305489085, 48.98284622040321068, 44.64431382829574346 ) ) ;
#26946=CARTESIAN_POINT ( 'NONE',  ( -71.97767679134960872, 19.88555875055813971, 94.99999999999866418 ) ) ;
#26947=CARTESIAN_POINT ( 'NONE',  ( 84.97343609940688225, 18.86260005312943733, -9.158222328408974988 ) ) ;
#26950=CARTESIAN_POINT ( 'NONE',  ( -94.79166046756728292, 29.13671350128075588, 11.66547666712828857 ) ) ;
#26951=CARTESIAN_POINT ( 'NONE',  ( -98.67723517640901321, 30.98797878696538888, -62.77687572781893977 ) ) ;
#26954=CARTESIAN_POINT ( 'NONE',  ( 188.4937788906149194, 86.43336847120859545, -69.37079316943395213 ) ) ;
#26955=CARTESIAN_POINT ( 'NONE',  ( 10.13405324523498585, 6.385324379632243641, 32.56244327895191049 ) ) ;
#26959=CARTESIAN_POINT ( 'NONE',  ( 105.4134760436918441, 27.80903124201756427, -64.50795234698105673 ) ) ;
#26961=CARTESIAN_POINT ( 'NONE',  ( 82.74007713545064746, 18.13042311233563808, 30.79472337014629346 ) ) ;
#26963=CARTESIAN_POINT ( 'NONE',  ( -120.4666325602656087, 44.20829586446610904, 32.93748705592776815 ) ) ;
#26964=CARTESIAN_POINT ( 'NONE',  ( 206.3125232506203304, 108.5822159704962360, 70.88763313768686203 ) ) ;
#26965=EDGE_LOOP ( 'NONE', ( #21661, #49937 ) ) ;
#26969=CARTESIAN_POINT ( 'NONE',  ( -31.92580063159127590, 9.671320706097196407, 3.371903815725487252 ) ) ;
#26970=CARTESIAN_POINT ( 'NONE',  ( -83.97920458302543523, 24.41672699001660263, 86.30411619380763000 ) ) ;
#26971=CARTESIAN_POINT ( 'NONE',  ( 94.06699947028486974, 23.17027898120150198, 63.05914927619607369 ) ) ;
#26972=CARTESIAN_POINT ( 'NONE',  ( 149.9872551245001375, 52.05943539582082025, -16.20506168770759459 ) ) ;
#26973=CARTESIAN_POINT ( 'NONE',  ( 32.37980458033285913, 8.611076697115695566, 13.21509809174489547 ) ) ;
#26974=CARTESIAN_POINT ( 'NONE',  ( -95.21085197937823352, 30.44372064875429373, -66.80218551204211508 ) ) ;
#26977=FACE_OUTER_BOUND ( 'NONE', #36129, .T. ) ;
#26978=DIRECTION ( 'NONE',  ( -0.000000000000000000, 1.000000000000000000, -0.000000000000000000 ) ) ;
#26981=CARTESIAN_POINT ( 'NONE',  ( 14.80291736570134731, 7.477373894757626260, -62.41206896596168718 ) ) ;
#26987=EDGE_CURVE ( 'NONE', #8573, #8018, #48796, .T. ) ;
#26988=CARTESIAN_POINT ( 'NONE',  ( 94.13654418975937688, 23.19669502308961029, 90.80720038674762407 ) ) ;
#26992=CARTESIAN_POINT ( 'NONE',  ( -190.3074740493607635, 108.5764897054613698, -19.14891730205166809 ) ) ;
#26993=CARTESIAN_POINT ( 'NONE',  ( -102.2801239173131052, 33.91021738430207932, -76.85912785543962400 ) ) ;
#26994=CARTESIAN_POINT ( 'NONE',  ( -105.4642082819535887, 35.56541171990215844, 71.67034629880215846 ) ) ;
#26996=CARTESIAN_POINT ( 'NONE',  ( -180.6099868604459573, 95.87049015238672212, 92.56375689375346383 ) ) ;
#26998=CARTESIAN_POINT ( 'NONE',  ( 157.4703587214989398, -170.0000000000000000, -43.62418429913764584 ) ) ;
#26999=CARTESIAN_POINT ( 'NONE',  ( -3.252497086158844031, 6.636017118948017490, -22.03862939399687093 ) ) ;
#27001=CARTESIAN_POINT ( 'NONE',  ( -156.5309640077389304, 70.37330322764253765, 89.25824053272464198 ) ) ;
#27002=CARTESIAN_POINT ( 'NONE',  ( 139.6359093656973585, 45.02518919224740301, 41.79700139785594359 ) ) ;
#27003=EDGE_CURVE ( 'NONE', #9227, #57612, #16049, .T. ) ;
#27006=CARTESIAN_POINT ( 'NONE',  ( 83.37782009939532202, 19.39546426214658226, 17.13040966651107055 ) ) ;
#27007=CARTESIAN_POINT ( 'NONE',  ( 163.5944442552010116, 63.88381951184479846, 14.40178751837228077 ) ) ;
#27008=LINE ( 'NONE', #21386, #30819 ) ;
#27015=CARTESIAN_POINT ( 'NONE',  ( -72.78737098446268305, 20.16853011470089641, -20.45466042152229846 ) ) ;
#27016=CARTESIAN_POINT ( 'NONE',  ( 157.4703587214989113, 58.92748579479260229, 44.40946747225338953 ) ) ;
#27018=ORIENTED_EDGE ( 'NONE', *, *, #12915, .F. ) ;
#27019=CARTESIAN_POINT ( 'NONE',  ( 157.9160637431159557, 57.99786926216935967, 44.40946747225338953 ) ) ;
#27023=VERTEX_POINT ( 'NONE', #49521 ) ;
#27027=CARTESIAN_POINT ( 'NONE',  ( 134.7697261969508418, 41.97802808873665015, 56.39672482949090693 ) ) ;
#27028=CARTESIAN_POINT ( 'NONE',  ( -178.2328124332056234, 94.56955476227572888, 32.81359777475018547 ) ) ;
#27029=CARTESIAN_POINT ( 'NONE',  ( -33.37566357177429666, 9.916833145467595756, -76.92377550660138752 ) ) ;
#27030=VERTEX_POINT ( 'NONE', #64680 ) ;
#27032=ORIENTED_EDGE ( 'NONE', *, *, #44122, .F. ) ;
#27034=CARTESIAN_POINT ( 'NONE',  ( -47.78549779818827403, 12.85263308667515680, 89.62398069324977712 ) ) ;
#27036=CARTESIAN_POINT ( 'NONE',  ( -107.7020481907979530, 35.62148549414491328, 86.51664613115644897 ) ) ;
#27040=EDGE_LOOP ( 'NONE', ( #15559, #28469 ) ) ;
#27045=CARTESIAN_POINT ( 'NONE',  ( 212.0739503583954217, 117.0412199804969617, -72.06906948032111870 ) ) ;
#27049=CARTESIAN_POINT ( 'NONE',  ( -35.47329415418259657, 10.28840791552277700, -90.18009615600030315 ) ) ;
#27050=DIRECTION ( 'NONE',  ( 0.000000000000000000, 0.000000000000000000, 1.000000000000000000 ) ) ;
#27051=CARTESIAN_POINT ( 'NONE',  ( -190.6985136298601731, 109.1272424661242582, -73.40678087856149148 ) ) ;
#27060=CARTESIAN_POINT ( 'NONE',  ( -24.71645982722742474, 9.599558729461499240, -66.32750219526168678 ) ) ;
#27061=CARTESIAN_POINT ( 'NONE',  ( 56.66775172211444556, 11.28938863449060115, -39.21877147530136654 ) ) ;
#27064=CARTESIAN_POINT ( 'NONE',  ( -142.5211356634642073, 58.47296527616906303, 8.634676124789878671 ) ) ;
#27065=EDGE_CURVE ( 'NONE', #63745, #34735, #37941, .T. ) ;
#27070=ORIENTED_EDGE ( 'NONE', *, *, #34346, .T. ) ;
#27072=CARTESIAN_POINT ( 'NONE',  ( -142.9756886485677683, 60.11539876121631920, 34.52562815318861311 ) ) ;
#27076=CARTESIAN_POINT ( 'NONE',  ( -31.01172313875360587, 10.54069851409512282, -89.00629854612918734 ) ) ;
#27082=ORIENTED_EDGE ( 'NONE', *, *, #43644, .F. ) ;
#27083=FACE_OUTER_BOUND ( 'NONE', #63229, .T. ) ;
#27084=CYLINDRICAL_SURFACE ( 'NONE', #44032, 7.500000000000013323 ) ;
#27086=CARTESIAN_POINT ( 'NONE',  ( 134.3159642998340075, 41.70198410084976359, -77.86786152285935714 ) ) ;
#27087=CARTESIAN_POINT ( 'NONE',  ( 64.69649025047539226, 13.06878919510320891, 29.99968890139355082 ) ) ;
#27089=EDGE_CURVE ( 'NONE', #64204, #59065, #5950, .T. ) ;
#27090=CARTESIAN_POINT ( 'NONE',  ( 18.97570931738674815, 7.630744579664928473, 84.40680895099953318 ) ) ;
#27092=ORIENTED_EDGE ( 'NONE', *, *, #67370, .F. ) ;
#27094=DIRECTION ( 'NONE',  ( 0.000000000000000000, 0.000000000000000000, 1.000000000000000000 ) ) ;
#27099=CARTESIAN_POINT ( 'NONE',  ( 12.03317402819681803, 6.409531826169462931, -49.51584580361413401 ) ) ;
#27101=CARTESIAN_POINT ( 'NONE',  ( -125.8938041572051105, 47.69968343338781125, -88.60280507916129977 ) ) ;
#27103=CARTESIAN_POINT ( 'NONE',  ( 103.0463737467386665, -170.0000000000000000, -95.00000000000133582 ) ) ;
#27106=CARTESIAN_POINT ( 'NONE',  ( 69.36287815987333261, 15.27486453472191208, 33.31009857533451424 ) ) ;
#27108=DIRECTION ( 'NONE',  ( -0.000000000000000000, 1.000000000000000000, -0.000000000000000000 ) ) ;
#27110=CARTESIAN_POINT ( 'NONE',  ( -26.50364027666004318, 8.832969329054181529, 32.04808994178188897 ) ) ;
#27112=B_SPLINE_CURVE_WITH_KNOTS ( 'NONE', 3,
 ( #65301, #32594, #64255, #42453, #16063, #49095, #26284, #21339, #37517, #32934, #22035, #38560, #21683, #38214, #53689, #48746, #54019, #5847, #10782, #64604, #32256, #22382, #15724, #43133, #69519, #584, #16412, #31906, #27303, #59652, #17091, #11467, #54376, #60006, #53336, #6202, #27654, #11827, #4815, #69180, #5167, #26630, #48064, #39612 ),
 .UNSPECIFIED., .F., .F.,
 ( 4, 2, 2, 2, 2, 2, 2, 2, 2, 2, 2, 2, 2, 2, 2, 2, 2, 2, 2, 2, 2, 4 ),
 ( 0.000000000000000000, 0.001472974678681631235, 0.002209462018022446961, 0.002945949357363262470, 0.004418924036044874840, 0.005891898714726486776, 0.007364873393408098712, 0.008101360732748905114, 0.008837848072089711515, 0.01031082275077132258, 0.01178379742945293539, 0.01252028476879375046, 0.01325677210813456554, 0.01472974678681621824, 0.01546623412615704372, 0.01620272146549786921, 0.01767569614417952364, 0.01914867082286117461, 0.01988515816220199489, 0.02062164550154281517, 0.02209462018022445920, 0.02356759485890609976 ),
 .UNSPECIFIED. ) ;
#27115=FACE_BOUND ( 'NONE', #39361, .T. ) ;
#27116=CARTESIAN_POINT ( 'NONE',  ( -0.3747453031323932926, 6.520267647591907689, -70.75102776234530211 ) ) ;
#27117=CARTESIAN_POINT ( 'NONE',  ( -180.6215424137751882, 97.48070480470862265, 65.47218828009727076 ) ) ;
#27123=CARTESIAN_POINT ( 'NONE',  ( -76.57217434633363951, 21.53469935507370181, -89.09026432457217481 ) ) ;
#27125=CARTESIAN_POINT ( 'NONE',  ( 66.73594759725088466, 13.56641407806656296, 16.98519729053115412 ) ) ;
#27128=CARTESIAN_POINT ( 'NONE',  ( 90.30732934992394689, 21.77797012484618833, -9.923057525364814779 ) ) ;
#27131=CARTESIAN_POINT ( 'NONE',  ( -33.38294402636583413, 10.93918551420889251, 18.13226767664806971 ) ) ;
#27135=CARTESIAN_POINT ( 'NONE',  ( 82.94816950786174914, 19.25538918181906922, -63.62716752535860110 ) ) ;
#27136=CARTESIAN_POINT ( 'NONE',  ( 102.9205852613134482, 26.73239185155387432, 92.46039132013983419 ) ) ;
#27137=CARTESIAN_POINT ( 'NONE',  ( -148.0058283997321666, 64.22864592525512251, 57.71403787313865053 ) ) ;
#27138=CARTESIAN_POINT ( 'NONE',  ( 68.93219921887765622, 14.12322281954860870, -20.99186324365028611 ) ) ;
#27140=CARTESIAN_POINT ( 'NONE',  ( -23.95089599695169014, 9.496585844566149959, -43.30571257647613947 ) ) ;
#27141=CARTESIAN_POINT ( 'NONE',  ( -47.60266343315663562, 13.84328785304053433, -68.56165223857558999 ) ) ;
#27142=CARTESIAN_POINT ( 'NONE',  ( 204.6977192012829789, -170.0000000000000000, -9.481380442157897548 ) ) ;
#27143=CARTESIAN_POINT ( 'NONE',  ( -121.5928001448269384, 44.91559452735374691, -9.407046580589417673 ) ) ;
#27147=CARTESIAN_POINT ( 'NONE',  ( 36.77024545412684375, 9.095083943590502429, 57.23105213408622660 ) ) ;
#27148=CARTESIAN_POINT ( 'NONE',  ( -170.2951623264596890, 85.51757001115473145, 72.12628606607438542 ) ) ;
#27152=CARTESIAN_POINT ( 'NONE',  ( 68.19664458616936997, 14.97277333049207826, -91.47147629385359835 ) ) ;
#27154=CARTESIAN_POINT ( 'NONE',  ( 93.87111289824404992, 23.09598275302506920, 12.38314846173391004 ) ) ;
#27155=CARTESIAN_POINT ( 'NONE',  ( 188.5842358232186200, 88.03712271786933741, -17.17993020127526549 ) ) ;
#27156=CARTESIAN_POINT ( 'NONE',  ( 211.7357196141372242, 118.3691710715567069, 12.47229085737326848 ) ) ;
#27159=CARTESIAN_POINT ( 'NONE',  ( 207.4696221732442325, 110.2206209205162111, -23.96229707863594882 ) ) ;
#27161=CARTESIAN_POINT ( 'NONE',  ( 161.7031777507227162, 62.31724004902786618, 69.96241716275324052 ) ) ;
#27165=CARTESIAN_POINT ( 'NONE',  ( -53.13788504024110182, 15.21566150156364472, 57.39441362419945847 ) ) ;
#27168=CARTESIAN_POINT ( 'NONE',  ( -2.077198674172494819, 7.591450106608311543, 86.44301495747437514 ) ) ;
#27170=ORIENTED_EDGE ( 'NONE', *, *, #34058, .T. ) ;
#27172=CARTESIAN_POINT ( 'NONE',  ( 60.40277045393654021, 12.08176563382370006, 17.50278692932749180 ) ) ;
#27173=CARTESIAN_POINT ( 'NONE',  ( -7.825402957745087207, 6.891034867348160731, -62.26262132240749736 ) ) ;
#27174=ORIENTED_EDGE ( 'NONE', *, *, #3418, .F. ) ;
#27178=CARTESIAN_POINT ( 'NONE',  ( 44.27343555294838495, 10.11032640759955825, 85.36175225958380963 ) ) ;
#27181=VERTEX_POINT ( 'NONE', #6979 ) ;
#27183=CARTESIAN_POINT ( 'NONE',  ( -58.76005811686687963, 15.70653557534867595, -63.02321690226305151 ) ) ;
#27185=CARTESIAN_POINT ( 'NONE',  ( 31.96227686234410470, 7.558148489540043258, -17.25635040805548215 ) ) ;
#27186=CARTESIAN_POINT ( 'NONE',  ( 173.6700117628887483, 72.79957362875117610, -42.55458116747357167 ) ) ;
#27187=CARTESIAN_POINT ( 'NONE',  ( -149.5074843970971017, 65.50121172469319220, -76.65738112195568021 ) ) ;
#27188=CARTESIAN_POINT ( 'NONE',  ( 89.22118407503259618, 20.32164250407898010, 44.25407225728361738 ) ) ;
#27190=CARTESIAN_POINT ( 'NONE',  ( -47.60266343315662141, 13.84328785304053255, -41.71710164811194943 ) ) ;
#27194=CARTESIAN_POINT ( 'NONE',  ( 39.40195752203892710, 8.409560354027398432, -23.77526687496409608 ) ) ;
#27200=CARTESIAN_POINT ( 'NONE',  ( -12.77647591501652435, 7.263973827022343066, -21.72877552418942315 ) ) ;
#27201=CARTESIAN_POINT ( 'NONE',  ( -174.5218377053110430, 90.22516661118194747, 84.63846801733375003 ) ) ;
#27202=FACE_OUTER_BOUND ( 'NONE', #58884, .T. ) ;
#27205=CARTESIAN_POINT ( 'NONE',  ( -62.14837099232444473, 17.75045801599139850, -40.27407517813967530 ) ) ;
#27207=CARTESIAN_POINT ( 'NONE',  ( -15.13211202216340645, 8.488266782358815377, -17.78287500119007447 ) ) ;
#27208=CARTESIAN_POINT ( 'NONE',  ( 154.0293889979056985, 55.02370422818217577, -77.14919040647539816 ) ) ;
#27214=ORIENTED_EDGE ( 'NONE', *, *, #15115, .F. ) ;
#27218=CARTESIAN_POINT ( 'NONE',  ( -25.74393077470917746, 9.741270655232812103, 86.48243346646731311 ) ) ;
#27219=CARTESIAN_POINT ( 'NONE',  ( -154.0833774771448930, 69.51012195447350450, 17.33764892392960277 ) ) ;
#27222=CARTESIAN_POINT ( 'NONE',  ( 22.80839748737788497, 6.826915557457463812, 34.86363334158694727 ) ) ;
#27223=CARTESIAN_POINT ( 'NONE',  ( -189.2776534485022069, 108.4862893474047638, -95.00000000000133582 ) ) ;
#27226=VERTEX_POINT ( 'NONE', #43041 ) ;
#27229=CARTESIAN_POINT ( 'NONE',  ( 32.15613847490628530, 8.588587416860166357, -45.07158521509305160 ) ) ;
#27236=CARTESIAN_POINT ( 'NONE',  ( 188.5651904823862139, 88.01586411309102687, 64.26411188446218148 ) ) ;
#27237=CARTESIAN_POINT ( 'NONE',  ( -155.2912910578197057, 69.24479901948500071, 69.84663848284604626 ) ) ;
#27238=CARTESIAN_POINT ( 'NONE',  ( -5.888165822225390755, 7.780336669456525023, -35.66840708012240668 ) ) ;
#27241=CARTESIAN_POINT ( 'NONE',  ( -85.10774223992955001, 24.88053943842882632, -46.46551204592482520 ) ) ;
#27244=DIRECTION ( 'NONE',  ( 0.000000000000000000, 0.000000000000000000, 1.000000000000000000 ) ) ;
#27249=CARTESIAN_POINT ( 'NONE',  ( -128.9925397612932727, 48.56800623462827815, -49.24758187794226671 ) ) ;
#27251=CARTESIAN_POINT ( 'NONE',  ( 55.76255201544532980, 12.13275766515752174, -72.03696989504328485 ) ) ;
#27254=LINE ( 'NONE', #32542, #46000 ) ;
#27255=CARTESIAN_POINT ( 'NONE',  ( 174.3253633919052277, 72.03478936859502824, 93.75446226051346343 ) ) ;
#27258=CARTESIAN_POINT ( 'NONE',  ( 181.0840389613909736, 80.03940679743416808, 29.30859410551139277 ) ) ;
#27262=CARTESIAN_POINT ( 'NONE',  ( 103.8956072042905276, 27.14952820414103840, -93.09487571133699646 ) ) ;
#27264=CARTESIAN_POINT ( 'NONE',  ( -74.17694007417655655, 20.66176641130876845, -36.58787508697967183 ) ) ;
#27265=CARTESIAN_POINT ( 'NONE',  ( 80.95159210695670993, 17.56111694104498611, -92.09322649547419815 ) ) ;
#27266=CARTESIAN_POINT ( 'NONE',  ( 94.02921784728462740, 22.08005910033066499, -42.07469127671826215 ) ) ;
#27267=CIRCLE ( 'NONE', #2589, 243.4957430088094839 ) ;
#27269=B_SPLINE_CURVE_WITH_KNOTS ( 'NONE', 3,
 ( #68875, #20700, #15433, #36890, #58668, #47771, #42503, #22084, #54779, #43525, #28399, #6947, #11511, #1322, #44928, #23135, #12233, #22777, #44220, #49142, #65003, #17496, #32984, #39314, #33697, #28763, #6246, #23489, #39656, #18203, #1673, #17136, #633, #33348, #38254, #55125 ),
 .UNSPECIFIED., .F., .F.,
 ( 4, 2, 2, 2, 2, 2, 2, 2, 2, 2, 2, 2, 2, 2, 2, 2, 2, 4 ),
 ( 1.551583845779545699E-17, 0.001548367318450204286, 0.003096734636900392960, 0.004645101955350582068, 0.006193469273800770308, 0.007741836592250959416, 0.008516020251476042260, 0.009290203910701125972, 0.01083857122915127431, 0.01238693854760142092, 0.01393530586605156926, 0.01548367318450171587, 0.01703204050295186248, 0.01858040782140200908, 0.02012877513985215569, 0.02167714245830229883, 0.02322550977675244543, 0.02477387709520258857 ),
 .UNSPECIFIED. ) ;
#27275=CARTESIAN_POINT ( 'NONE',  ( -144.9417090887490929, 61.69631066549399634, -48.26759783987280628 ) ) ;
#27279=CARTESIAN_POINT ( 'NONE',  ( -149.5074843970971301, -170.0000000000000000, -69.15738112195565179 ) ) ;
#27283=FACE_OUTER_BOUND ( 'NONE', #35849, .T. ) ;
#27285=B_SPLINE_CURVE_WITH_KNOTS ( 'NONE', 3,
 ( #20601, #32543, #21298, #15680, #27255, #179, #5801, #14984, #68786, #42063, #63522, #37128, #36798, #53291, #58239, #10056, #26919, #48345, #31515, #4772, #26240, #47672, #48016, #69478, #58920, #10737, #55381, #7571, #17401, #33603, #64910, #65971, #27606, #65249, #33948, #55033, #44489, #38512, #22685, #50118, #1232, #38877, #6855, #21985, #60321, #43432, #16704, #60668, #12141, #39223, #28306, #49746, #61018, #17767, #12485, #39567, #7209, #1577, #38161, #23043, #59602, #18111, #28665, #1947, #23403, #44839, #66323, #49404, #29026, #59959 ),
 .UNSPECIFIED., .F., .F.,
 ( 4, 2, 2, 2, 2, 2, 2, 2, 2, 2, 2, 2, 2, 2, 2, 2, 2, 2, 2, 2, 2, 2, 2, 2, 2, 2, 2, 2, 2, 2, 2, 2, 2, 2, 4 ),
 ( 0.000000000000000000, 0.001217324661923814902, 0.001825986992885731026, 0.002434649323847647151, 0.003651973985771530141, 0.004260636316733491802, 0.004869298647695453897, 0.006086623309619333851, 0.006695285640581253445, 0.007303947971543172171, 0.007912610302505092633, 0.008521272633467011359, 0.009738597295390867895, 0.01095592195731472270, 0.01217324661923857923, 0.01339057128116243577, 0.01460789594308629057, 0.01704254526693400537, 0.01825986992885789487, 0.01947719459078178089, 0.02191184391462955988, 0.02312916857655346325, 0.02434649323847737010, 0.02678114256232515256, 0.02799846722424905593, 0.02921579188617295930, 0.03043311654809685574, 0.03165044121002075911, 0.03225910354098271426, 0.03286776587194466942, 0.03408509053386857973, 0.03530241519579249004, 0.03651973985771640036, 0.03773706451964031067, 0.03895438918156422098 ),
 .UNSPECIFIED. ) ;
#27287=CARTESIAN_POINT ( 'NONE',  ( 136.9798231265810387, 43.34196232604177368, -23.51336826870209507 ) ) ;
#27292=CARTESIAN_POINT ( 'NONE',  ( -99.11448999425219597, 31.20120877265622283, -76.17449768191258386 ) ) ;
#27295=EDGE_CURVE ( 'NONE', #7511, #37504, #28655, .T. ) ;
#27296=CARTESIAN_POINT ( 'NONE',  ( 43.96465529479667822, 9.046527005589350523, 31.44099358552342949 ) ) ;
#27301=CARTESIAN_POINT ( 'NONE',  ( -78.18897186942403721, 23.21604822208489338, -61.96000122218158168 ) ) ;
#27302=CARTESIAN_POINT ( 'NONE',  ( 63.99027454648599189, 13.93445177372598565, -50.67285947261250811 ) ) ;
#27303=CARTESIAN_POINT ( 'NONE',  ( 46.12611922993085045, 10.39838587005582404, -46.45098542691543031 ) ) ;
#27305=EDGE_LOOP ( 'NONE', ( #34975, #64561, #7006, #35825 ) ) ;
#27307=EDGE_LOOP ( 'NONE', ( #67039, #11870 ) ) ;
#27308=CARTESIAN_POINT ( 'NONE',  ( -12.39701069459754379, 7.231688578592715189, -48.88370839588166916 ) ) ;
#27311=CARTESIAN_POINT ( 'NONE',  ( 92.53033045403535084, 22.59263332688195902, 59.40129347602972842 ) ) ;
#27313=CARTESIAN_POINT ( 'NONE',  ( 152.8558173410470147, 54.14978343559393892, -10.84730958789643829 ) ) ;
#27317=CARTESIAN_POINT ( 'NONE',  ( 211.5170725404452412, 116.1892283197351645, 87.25311100178144841 ) ) ;
#27324=CARTESIAN_POINT ( 'NONE',  ( 39.89582146299187571, 9.488756994579086168, -62.46436805589146957 ) ) ;
#27325=CARTESIAN_POINT ( 'NONE',  ( -5.871577929436018195, 6.771181646175757685, 44.87346486140882718 ) ) ;
#27328=CARTESIAN_POINT ( 'NONE',  ( 93.72616975926867156, 23.04113753715060398, 88.45117781230963772 ) ) ;
#27330=VERTEX_POINT ( 'NONE', #60972 ) ;
#27331=B_SPLINE_CURVE_WITH_KNOTS ( 'NONE', 3,
 ( #3911, #8499, #63690, #8851, #25027, #52764, #9884, #68282, #14114, #57721, #20421, #67942, #36612, #35923, #35577, #25720, #41885, #57036, #29951, #24684, #62994, #46118, #51750, #19388, #19736, #30994, #9533, #15154, #4591, #67589, #30302, #41197, #62658, #14466, #57374, #52441, #9186, #68945, #30643, #20086, #42228, #6318, #10204, #69301, #47838, #701, #33063, #2996, #31672, #48170 ),
 .UNSPECIFIED., .F., .F.,
 ( 4, 2, 2, 2, 2, 2, 2, 2, 2, 2, 2, 2, 2, 2, 2, 2, 2, 2, 2, 2, 2, 2, 2, 2, 4 ),
 ( 0.03126542424884323074, 0.03330676804260265106, 0.03534811183636207832, 0.03738945563012149864, 0.03943079942388091896, 0.04045147132076062912, 0.04147214321764033929, 0.04249281511452004945, 0.04351348701139975961, 0.04555483080515919381, 0.04657550270203893172, 0.04759617459891865576, 0.04810651054735851084, 0.04861684649579836592, 0.04963751839267807608, 0.05065819028955779318, 0.05167886218643750335, 0.05269953408331721351, 0.05372020598019692367, 0.05474087787707663383, 0.05576154977395634399, 0.05780289356771584064, 0.05984423736147533035, 0.06188558115523482006, 0.06392692494899430977 ),
 .UNSPECIFIED. ) ;
#27334=CARTESIAN_POINT ( 'NONE',  ( -190.0468231512975592, 108.2116162189844601, -18.66563101447177431 ) ) ;
#27335=CARTESIAN_POINT ( 'NONE',  ( -133.3958821919892728, 51.63629593114587379, 10.76119976374093312 ) ) ;
#27336=CARTESIAN_POINT ( 'NONE',  ( -166.0012244511291328, 80.97916541034756222, -44.58685355227834890 ) ) ;
#27338=CARTESIAN_POINT ( 'NONE',  ( -132.9126122820979390, 52.52752252041130276, -45.07027942257388986 ) ) ;
#27342=CARTESIAN_POINT ( 'NONE',  ( 199.3764470687682433, 100.9548044849098858, -11.69055677975092067 ) ) ;
#27343=CARTESIAN_POINT ( 'NONE',  ( -150.6746572836342182, 65.17487362867251477, 84.48152048434670291 ) ) ;
#27346=DIRECTION ( 'NONE',  ( 0.000000000000000000, 0.000000000000000000, 1.000000000000000000 ) ) ;
#27348=CARTESIAN_POINT ( 'NONE',  ( -149.7268278745401346, 65.68859631971236013, 30.72082123989904900 ) ) ;
#27349=ORIENTED_EDGE ( 'NONE', *, *, #18491, .T. ) ;
#27354=CARTESIAN_POINT ( 'NONE',  ( -123.0615383220166024, 44.65678520910835658, -89.14556082492318012 ) ) ;
#27360=CARTESIAN_POINT ( 'NONE',  ( 164.0158927577712689, 62.92463143894071465, 33.20978262532335634 ) ) ;
#27362=FACE_OUTER_BOUND ( 'NONE', #65436, .T. ) ;
#27369=CARTESIAN_POINT ( 'NONE',  ( -38.26732153931116187, 10.81230693396213560, -19.08489745522991043 ) ) ;
#27370=CARTESIAN_POINT ( 'NONE',  ( -180.3114074031036296, 97.09758726817787533, 36.16720739342910917 ) ) ;
#27372=CARTESIAN_POINT ( 'NONE',  ( -36.37663950036512261, 10.45389057208229033, -63.99519408383326180 ) ) ;
#27378=CARTESIAN_POINT ( 'NONE',  ( -103.2061297292848963, 34.38496953192505146, 3.717327809790629267 ) ) ;
#27381=CARTESIAN_POINT ( 'NONE',  ( -109.3054070592207125, 36.49501222209682538, 94.41388992448162298 ) ) ;
#27384=CARTESIAN_POINT ( 'NONE',  ( 86.14852828165534504, 19.25704475759651757, 71.55663816294307367 ) ) ;
#27385=ORIENTED_EDGE ( 'NONE', *, *, #22243, .F. ) ;
#27389=CARTESIAN_POINT ( 'NONE',  ( 208.9781236209186943, 112.4006213943320063, -64.49528624921919118 ) ) ;
#27391=B_SPLINE_CURVE_WITH_KNOTS ( 'NONE', 3,
 ( #17874, #53748, #17156, #2738, #24553, #35441, #61482, #2054, #19249, #55496, #66776, #50232, #62159, #23506, #45989, #35089, #44948, #28782 ),
 .UNSPECIFIED., .F., .F.,
 ( 4, 2, 2, 2, 2, 2, 2, 2, 4 ),
 ( 0.000000000000000000, 0.001462886883184502792, 0.002194330324776737600, 0.002925773766368972625, 0.004388660649553535915, 0.005851547532738099640, 0.008777321299107172445, 0.01024020818229175525, 0.01170309506547633979 ),
 .UNSPECIFIED. ) ;
#27393=CARTESIAN_POINT ( 'NONE',  ( -76.77329340382465261, 21.60914066444074422, 18.34659420984980471 ) ) ;
#27395=CARTESIAN_POINT ( 'NONE',  ( -54.57280099357649306, 14.55288945003959178, 3.472777182467475576 ) ) ;
#27396=CARTESIAN_POINT ( 'NONE',  ( 198.3476137557912864, 98.02317921105191090, 94.40621084052870060 ) ) ;
#27399=EDGE_CURVE ( 'NONE', #47203, #25401, #65210, .T. ) ;
#27400=CARTESIAN_POINT ( 'NONE',  ( -7.825402957745087207, -170.0000000000000000, -69.76262132240751157 ) ) ;
#27406=CARTESIAN_POINT ( 'NONE',  ( -85.45399718454962112, 25.02415453493131636, 41.11853589859573788 ) ) ;
#27417=CARTESIAN_POINT ( 'NONE',  ( 205.5105258529713126, 107.4632495673648549, 17.33006175898614032 ) ) ;
#27418=CARTESIAN_POINT ( 'NONE',  ( 181.4357232180614403, 80.39782411996594647, -89.91415884680694148 ) ) ;
#27420=CARTESIAN_POINT ( 'NONE',  ( 55.56474667084419394, 11.06706367715628581, 65.15011283490898109 ) ) ;
#27421=CARTESIAN_POINT ( 'NONE',  ( 140.0012045870120687, 46.45892655944614091, 94.99999999999866418 ) ) ;
#27423=CARTESIAN_POINT ( 'NONE',  ( -27.58705350908502396, 10.00788090876177172, -90.06758292199550908 ) ) ;
#27433=CARTESIAN_POINT ( 'NONE',  ( 63.98971758354224448, 12.90030016320048212, 44.76545530976716236 ) ) ;
#27435=EDGE_CURVE ( 'NONE', #40675, #31531, #58055, .T. ) ;
#27436=CARTESIAN_POINT ( 'NONE',  ( 85.67452303415198855, 19.09699411916382772, 17.82172837155005141 ) ) ;
#27438=CARTESIAN_POINT ( 'NONE',  ( -77.02372450489322375, 21.70271995013165522, 30.59644576040608399 ) ) ;
#27441=VERTEX_POINT ( 'NONE', #30701 ) ;
#27442=CARTESIAN_POINT ( 'NONE',  ( -122.8011284400168108, 45.68452922414294193, 4.427239656831918779 ) ) ;
#27447=ADVANCED_FACE ( 'NONE', ( #35287 ), #14519, .F. ) ;
#27449=CARTESIAN_POINT ( 'NONE',  ( 150.2076397309211302, 52.21780102759852582, 35.01788660041049894 ) ) ;
#27451=LINE ( 'NONE', #23248, #68975 ) ;
#27460=FACE_BOUND ( 'NONE', #29118, .T. ) ;
#27461=CARTESIAN_POINT ( 'NONE',  ( -0.7215816834507551292, 6.532459459468099361, -72.18059463655460206 ) ) ;
#27463=CARTESIAN_POINT ( 'NONE',  ( -180.6209674222602359, 97.47999311542517376, 64.99958634443271421 ) ) ;
#27464=CARTESIAN_POINT ( 'NONE',  ( 116.1047574213934439, 31.68944982538900135, -92.41450183877563518 ) ) ;
#27465=CARTESIAN_POINT ( 'NONE',  ( -121.2119672714299696, 44.67540322905996675, -36.53450468182285960 ) ) ;
#27466=CARTESIAN_POINT ( 'NONE',  ( -80.56139928459660382, 24.13290941644248022, 18.33423833827008309 ) ) ;
#27471=CARTESIAN_POINT ( 'NONE',  ( 70.26722489419893236, 14.47234958177331343, 8.490884802020540079 ) ) ;
#27472=CARTESIAN_POINT ( 'NONE',  ( 164.7250737226290767, 63.51898362052166647, 11.98738555690816732 ) ) ;
#27473=CARTESIAN_POINT ( 'NONE',  ( 94.06416612695409185, 23.16920323269612325, -15.45855970408906011 ) ) ;
#27475=CARTESIAN_POINT ( 'NONE',  ( -37.05762690088739220, 11.60527003175540628, 5.897699859483924278 ) ) ;
#27479=B_SPLINE_CURVE_WITH_KNOTS ( 'NONE', 3,
 ( #41680, #31472, #5427, #53247, #25860, #10349, #47629, #42367, #48304, #139, #20916, #31814, #30787, #26880, #68743, #47288, #57517, #52907, #10691, #42023, #20559, #68420, #14940, #5074, #9325, #69083, #4057, #63139, #63483, #15298, #36406, #32166, #58530, #63828, #57859, #58201, #53596, #21596, #43042, #10021, #14600, #26541, #64164, #9679, #47974, #25521 ),
 .UNSPECIFIED., .F., .F.,
 ( 4, 2, 2, 2, 2, 2, 2, 2, 2, 2, 2, 2, 2, 2, 2, 2, 2, 2, 2, 2, 2, 2, 4 ),
 ( 0.02420077021543442022, 0.02572112563160194529, 0.02648130333968569047, 0.02724148104776943566, 0.02876183646393689480, 0.02952201417202062611, 0.03028219188010435395, 0.03180254729627184085, 0.03332290271243932428, 0.03408308042052305559, 0.03484325812860679383, 0.03636361354477425645, 0.03712379125285799469, 0.03788396896094173294, 0.03864414666902546425, 0.03940432437710920249, 0.04092467979327665817, 0.04244503520944410691, 0.04396539062561156258, 0.04548574604177901826, 0.04624592374986272181, 0.04700610145794643924, 0.04852645687411389491 ),
 .UNSPECIFIED. ) ;
#27480=CARTESIAN_POINT ( 'NONE',  ( 86.62931800182293784, 20.48449268398422163, -62.66611478937537782 ) ) ;
#27481=CARTESIAN_POINT ( 'NONE',  ( 104.7547004776452582, 27.52138740370904912, 85.67756394359689409 ) ) ;
#27482=DIRECTION ( 'NONE',  ( -0.000000000000000000, 1.000000000000000000, -0.000000000000000000 ) ) ;
#27486=CARTESIAN_POINT ( 'NONE',  ( -30.46358361599564191, 10.45190018822943756, -35.36507249517946860 ) ) ;
#27487=CARTESIAN_POINT ( 'NONE',  ( -47.94960849910474820, 13.92522873833625674, -67.10330844354571411 ) ) ;
#27490=CARTESIAN_POINT ( 'NONE',  ( -122.3759299995709426, 45.41285412136513600, -22.20987056239383506 ) ) ;
#27494=CARTESIAN_POINT ( 'NONE',  ( 177.0024338932394130, 74.57605685449964028, 69.96155076402908435 ) ) ;
#27495=CARTESIAN_POINT ( 'NONE',  ( -165.7149569557575717, 80.68479365246975021, 66.38705370719434029 ) ) ;
#27496=CARTESIAN_POINT ( 'NONE',  ( -165.7713056973201446, 80.74264649718243447, -13.84472355417442024 ) ) ;
#27501=CARTESIAN_POINT ( 'NONE',  ( -12.39413342787890748, 7.231444436041486235, 70.42808861608598647 ) ) ;
#27502=CARTESIAN_POINT ( 'NONE',  ( 212.1488570093002011, 119.0116247937291405, 8.991641410805247148 ) ) ;
#27505=CARTESIAN_POINT ( 'NONE',  ( 46.89006465517228150, 9.501960077668739402, -15.78642848764656392 ) ) ;
#27506=CARTESIAN_POINT ( 'NONE',  ( 209.6525588430077676, 113.3929734759396837, -22.61648424082018494 ) ) ;
#27507=CARTESIAN_POINT ( 'NONE',  ( 157.4703587214989398, -170.0000000000000000, -70.46873488960132192 ) ) ;
#27508=CARTESIAN_POINT ( 'NONE',  ( 163.5944155533005926, 63.88379440759430139, 59.41703486054432659 ) ) ;
#27511=CARTESIAN_POINT ( 'NONE',  ( -31.43908319763710679, -170.0000000000000000, -42.81719736520184938 ) ) ;
#27513=CARTESIAN_POINT ( 'NONE',  ( -47.80251179448168131, 13.89045662648309865, 66.64588604812638550 ) ) ;
#27515=CARTESIAN_POINT ( 'NONE',  ( 156.5909039492009924, 56.96742803863246252, 17.56491688178971344 ) ) ;
#27516=CARTESIAN_POINT ( 'NONE',  ( -7.174370261180697206, 7.857450515965657800, 83.82589638950733502 ) ) ;
#27520=CARTESIAN_POINT ( 'NONE',  ( 56.66438910147189034, 11.28870326331393592, 6.471904661552231985 ) ) ;
#27524=EDGE_CURVE ( 'NONE', #46420, #68404, #40218, .T. ) ;
#27526=CARTESIAN_POINT ( 'NONE',  ( -78.66644367742109978, 22.32174330031320508, -61.96000122218157458 ) ) ;
#27527=DIRECTION ( 'NONE',  ( -0.000000000000000000, 1.000000000000000000, -0.000000000000000000 ) ) ;
#27528=CARTESIAN_POINT ( 'NONE',  ( 108.3819860115547300, 28.02992728837240577, 29.83061142536935506 ) ) ;
#27530=CARTESIAN_POINT ( 'NONE',  ( 63.50537371531940778, 13.81987663608982331, 71.65751152968502424 ) ) ;
#27533=CARTESIAN_POINT ( 'NONE',  ( 164.6561571795775478, 64.77723933022096503, 39.12902952882128460 ) ) ;
#27534=CARTESIAN_POINT ( 'NONE',  ( -156.8728827992623849, 72.05711009495558983, -70.59983789775942853 ) ) ;
#27535=FACE_OUTER_BOUND ( 'NONE', #48237, .T. ) ;
#27538=B_SPLINE_CURVE_WITH_KNOTS ( 'NONE', 3,
 ( #19822, #52170, #24756, #14538, #3988, #57110, #67669, #40572, #19465, #46539, #68357, #2603, #46893, #19116, #25457, #40923, #30029, #35997, #62026, #68015, #20160, #56406, #18778, #62382, #41274, #57448, #62734, #30372, #24414, #41615, #36341, #3296, #45857, #40236, #61682, #8582, #24062, #51822, #63070, #57793, #29676, #9613, #31076 ),
 .UNSPECIFIED., .F., .F.,
 ( 4, 2, 2, 2, 2, 2, 2, 2, 1, 2, 2, 2, 2, 2, 2, 2, 2, 2, 2, 2, 2, 4 ),
 ( 0.000000000000000000, 0.001465684626643342118, 0.002198526939965013936, 0.002931369253286685971, 0.004397053879930031342, 0.005862738506573376279, 0.007328423133216720349, 0.008061265446538396287, 0.008794107759860071358, 0.009526950073181746428, 0.01025979238650341976, 0.01172547701314676297, 0.01319116163979010443, 0.01465684626643344590, 0.01538968857975511750, 0.01612253089307678910, 0.01758821551972013578, 0.01905390014636348245, 0.01978674245968515405, 0.02051958477300682565, 0.02198526939965016538, 0.02345095402629350512 ),
 .UNSPECIFIED. ) ;
#27539=CARTESIAN_POINT ( 'NONE',  ( -48.34500911884040875, 14.01939034823941199, -39.35210440960034362 ) ) ;
#27541=ADVANCED_FACE ( 'NONE', ( #45839 ), #29659, .F. ) ;
#27542=CARTESIAN_POINT ( 'NONE',  ( -28.35957743809535003, 10.12373109553627870, 30.87345809538040697 ) ) ;
#27544=EDGE_CURVE ( 'NONE', #68729, #44045, #32078, .T. ) ;
#27549=VERTEX_POINT ( 'NONE', #53 ) ;
#27550=CARTESIAN_POINT ( 'NONE',  ( -10.91976120871578004, 7.112268444252501709, -22.90984318353010352 ) ) ;
#27551=CARTESIAN_POINT ( 'NONE',  ( -173.5307404820223951, 89.09910556100925305, 84.51787358894112856 ) ) ;
#27554=CARTESIAN_POINT ( 'NONE',  ( -59.57462349605616225, 16.98779896904798292, -48.71995552614745151 ) ) ;
#27556=CARTESIAN_POINT ( 'NONE',  ( -71.97767679134960872, 20.95111989827391596, 94.99999999999866418 ) ) ;
#27557=CARTESIAN_POINT ( 'NONE',  ( 22.89234820949993932, 6.832052815347870123, -18.59162056771186400 ) ) ;
#27558=ORIENTED_EDGE ( 'NONE', *, *, #1603, .F. ) ;
#27566=CARTESIAN_POINT ( 'NONE',  ( 116.8407179855993263, 32.05539589248573407, 94.43210676044013496 ) ) ;
#27567=DIRECTION ( 'NONE',  ( -0.000000000000000000, 1.000000000000000000, -0.000000000000000000 ) ) ;
#27569=CARTESIAN_POINT ( 'NONE',  ( -109.6660553119434951, 36.69391917620600196, 12.50300354649735723 ) ) ;
#27570=CARTESIAN_POINT ( 'NONE',  ( 23.23895241123075195, 6.853530908437178049, 36.52650928985956114 ) ) ;
#27576=VERTEX_POINT ( 'NONE', #69362 ) ;
#27579=CARTESIAN_POINT ( 'NONE',  ( -152.5101325120252795, 68.10842280990927122, -8.581351422625143499 ) ) ;
#27580=CARTESIAN_POINT ( 'NONE',  ( 33.46033188299905703, 8.722678254080108218, -47.70326261524692768 ) ) ;
#27582=CARTESIAN_POINT ( 'NONE',  ( -37.92511097250854135, 10.74631978746599970, 68.33491338229495682 ) ) ;
#27583=CARTESIAN_POINT ( 'NONE',  ( 157.4703587214989398, -170.0000000000000000, 36.90946747225337532 ) ) ;
#27584=EDGE_LOOP ( 'NONE', ( #16935, #49691, #68807, #54606 ) ) ;
#27589=CARTESIAN_POINT ( 'NONE',  ( 102.7425154123292259, 25.56407025871218863, 10.02495677748274616 ) ) ;
#27591=CARTESIAN_POINT ( 'NONE',  ( 8.000000000000007105, 249.8719672152120381, 94.99999999999866418 ) ) ;
#27592=CARTESIAN_POINT ( 'NONE',  ( 19.74724861314306423, 6.659670522263896331, 57.98450509540965214 ) ) ;
#27594=CARTESIAN_POINT ( 'NONE',  ( 8.336031647119270360, 6.376437040857335425, -68.88487339447647173 ) ) ;
#27598=CARTESIAN_POINT ( 'NONE',  ( -131.6133495896317243, 50.37677745548732133, -64.40045989538849369 ) ) ;
#27599=CARTESIAN_POINT ( 'NONE',  ( -131.7724154034330581, 50.48821165954358037, -37.74950181090596857 ) ) ;
#27600=CARTESIAN_POINT ( 'NONE',  ( 42.49453823366106064, 8.831814337191470798, -63.12732282323006672 ) ) ;
#27605=EDGE_CURVE ( 'NONE', #51770, #36565, #1744, .T. ) ;
#27606=CARTESIAN_POINT ( 'NONE',  ( 177.5697161277706755, 75.12518909700808933, 83.86496702357472088 ) ) ;
#27610=ADVANCED_FACE ( 'NONE', ( #36323 ), #20477, .F. ) ;
#27611=DIRECTION ( 'NONE',  ( -0.000000000000000000, 0.000000000000000000, -1.000000000000000000 ) ) ;
#27614=CARTESIAN_POINT ( 'NONE',  ( 113.8724110608469147, 31.71510301790680941, 57.37498895187409431 ) ) ;
#27616=CARTESIAN_POINT ( 'NONE',  ( 141.3400002717723112, 47.33399859146518907, 64.42256861941518764 ) ) ;
#27618=CARTESIAN_POINT ( 'NONE',  ( -101.8145602049405767, 32.54453702486149780, 45.51907450641512298 ) ) ;
#27620=VECTOR ( 'NONE', #14485, 1000.000000000000000 ) ;
#27621=CARTESIAN_POINT ( 'NONE',  ( 17.45749844226121539, 6.558648963513285857, -89.34746460272506852 ) ) ;
#27622=CARTESIAN_POINT ( 'NONE',  ( -47.94960849910472689, 13.92522873833625141, -13.41420726261837437 ) ) ;
#27629=EDGE_CURVE ( 'NONE', #54090, #68705, #55261, .T. ) ;
#27630=CARTESIAN_POINT ( 'NONE',  ( -146.1140637052938587, 62.65471088530801325, -49.01697918332925497 ) ) ;
#27635=CARTESIAN_POINT ( 'NONE',  ( 59.72647370436684611, 12.96353798836696214, 17.21311330783555604 ) ) ;
#27637=CARTESIAN_POINT ( 'NONE',  ( -148.6426981422629012, 63.44891673852537650, 57.60271724892876222 ) ) ;
#27640=CARTESIAN_POINT ( 'NONE',  ( 87.59078297315394934, 20.81577753000344444, 29.75859342957748410 ) ) ;
#27641=CARTESIAN_POINT ( 'NONE',  ( 79.82127737190243977, 17.20935440217364487, -19.63345140900991481 ) ) ;
#27642=DIRECTION ( 'NONE',  ( 0.000000000000000000, 0.000000000000000000, 1.000000000000000000 ) ) ;
#27643=CARTESIAN_POINT ( 'NONE',  ( -96.02415295709704424, 29.71480036090584775, 7.030227792584213375 ) ) ;
#27647=CARTESIAN_POINT ( 'NONE',  ( 46.13856685535755986, 9.381502944822525336, 40.74731373655765054 ) ) ;
#27654=CARTESIAN_POINT ( 'NONE',  ( 43.14565945994676355, 9.942782559600567893, -49.62327275826700657 ) ) ;
#27655=CARTESIAN_POINT ( 'NONE',  ( 211.5175447467296124, 116.1901475271414199, 66.68740704858620916 ) ) ;
#27657=CARTESIAN_POINT ( 'NONE',  ( -26.88234027341226096, 9.904106450608200163, 4.894934174378152925 ) ) ;
#27662=CARTESIAN_POINT ( 'NONE',  ( 89.88147981065577596, 21.62466191578947416, 70.83207453719057867 ) ) ;
#27663=CARTESIAN_POINT ( 'NONE',  ( 150.5550643769628323, 52.46819381604269239, -19.69512367869445058 ) ) ;
#27667=CARTESIAN_POINT ( 'NONE',  ( 111.0244322366040564, 30.35584396427519849, -89.64231344153266434 ) ) ;
#27669=DIRECTION ( 'NONE',  ( -0.000000000000000000, 1.000000000000000000, -0.000000000000000000 ) ) ;
#27672=CARTESIAN_POINT ( 'NONE',  ( 197.9812431552294072, 97.56504682326740863, 87.03682254010664110 ) ) ;
#27674=CARTESIAN_POINT ( 'NONE',  ( -30.94753041835916108, 9.510749728915506296, 18.37190381572551701 ) ) ;
#27676=CARTESIAN_POINT ( 'NONE',  ( -62.33640798863619636, 16.75617156245991168, -94.56231254894214544 ) ) ;
#27677=CARTESIAN_POINT ( 'NONE',  ( -108.5289085648060734, 36.07014995015116199, -65.20415147196632688 ) ) ;
#27678=CARTESIAN_POINT ( 'NONE',  ( 93.96365369154807468, 23.13106400759562575, 92.50572082305301080 ) ) ;
#27679=CIRCLE ( 'NONE', #67032, 243.4957430088094839 ) ;
#27683=CARTESIAN_POINT ( 'NONE',  ( -128.1219934350341703, 47.97781708504715681, 18.45142153448720279 ) ) ;
#27687=CARTESIAN_POINT ( 'NONE',  ( -179.7029633946883393, 94.76610802182018745, 88.39967368985821849 ) ) ;
#27688=ORIENTED_EDGE ( 'NONE', *, *, #35155, .F. ) ;
#27689=CARTESIAN_POINT ( 'NONE',  ( -125.0023254877051500, 45.90912477771773581, -49.87432082388755816 ) ) ;
#27690=DIRECTION ( 'NONE',  ( 0.000000000000000000, 0.000000000000000000, 1.000000000000000000 ) ) ;
#27692=EDGE_CURVE ( 'NONE', #34735, #31501, #68029, .T. ) ;
#27693=CARTESIAN_POINT ( 'NONE',  ( -5.879983509979052059, 7.779504553499493547, -77.02244074307444066 ) ) ;
#27698=CARTESIAN_POINT ( 'NONE',  ( 86.62931800182293784, 20.48449268398422518, 2.867536982015617575 ) ) ;
#27702=CARTESIAN_POINT ( 'NONE',  ( 112.5612011511789916, 31.08353758940340583, 3.118228259027523652 ) ) ;
#27707=VECTOR ( 'NONE', #12263, 1000.000000000000000 ) ;
#27708=CARTESIAN_POINT ( 'NONE',  ( -124.2579583355759212, 45.42576894968487267, -88.77160920751813933 ) ) ;
#27710=CARTESIAN_POINT ( 'NONE',  ( -37.62144393131467268, 11.71252597733099421, -92.23831152112933296 ) ) ;
#27711=CARTESIAN_POINT ( 'NONE',  ( 149.9714610887121751, 53.28792066194168342, 9.757508091027073505 ) ) ;
#27715=CARTESIAN_POINT ( 'NONE',  ( -78.66644367742109978, 23.39876645725290061, -35.11545063171788428 ) ) ;
#27717=EDGE_LOOP ( 'NONE', ( #22835, #177, #59982, #27070 ) ) ;
#27722=CARTESIAN_POINT ( 'NONE',  ( -35.99019277275120032, 10.38248800679341777, -9.991386557961455139 ) ) ;
#27724=CARTESIAN_POINT ( 'NONE',  ( 128.4157044224114372, 39.39296260757095780, 58.67006427216110609 ) ) ;
#27725=CARTESIAN_POINT ( 'NONE',  ( 15.78827728214693771, 7.507518794609574719, 71.85925826316895382 ) ) ;
#27727=B_SPLINE_CURVE_WITH_KNOTS ( 'NONE', 3,
 ( #55736, #44114, #38505, #33940, #1224, #64899, #7563, #49738, #7199, #12132, #39214, #50111, #16697, #27598, #60312, #33595, #65962, #12477, #6844, #28659, #880, #28299, #59950, #44482, #55375, #33245, #1940, #23397, #18103, #66315, #38152, #11412, #32883, #54317, #40588, #30047, #67343, #19834, #19134, #34978, #45872, #35319, #41291, #8242, #46206, #2281 ),
 .UNSPECIFIED., .F., .F.,
 ( 4, 2, 2, 2, 2, 2, 2, 2, 2, 2, 2, 2, 2, 2, 2, 2, 2, 2, 2, 2, 2, 2, 4 ),
 ( 6.938893903907228378E-18, 0.001615199098318979148, 0.003230398196637951358, 0.004037997745797443534, 0.004845597294956941782, 0.006460796393275941747, 0.007268395942435461679, 0.008075995491594980744, 0.009691194589913980709, 0.01049879413907351539, 0.01130639368823305180, 0.01211399323739258647, 0.01292159278655212115, 0.01453679188487114887, 0.01615199098319018006, 0.01695959053234967484, 0.01776719008150916962, 0.01938238917982816265, 0.02099758827814715567, 0.02180518782730661922, 0.02261278737646608278, 0.02422798647478500988, 0.02584318557310393699 ),
 .UNSPECIFIED. ) ;
#27732=CARTESIAN_POINT ( 'NONE',  ( -38.89042640463650002, 10.93374343663409753, -41.82923595654042259 ) ) ;
#27733=CARTESIAN_POINT ( 'NONE',  ( -106.2787154433887764, 34.85886827088950213, 85.35571367539338894 ) ) ;
#27736=CARTESIAN_POINT ( 'NONE',  ( -48.35591483259475609, 14.02198755119445117, 88.11419938166893928 ) ) ;
#27737=CARTESIAN_POINT ( 'NONE',  ( 79.22946426532583075, 17.02750615740070472, 62.80933842788154209 ) ) ;
#27742=CARTESIAN_POINT ( 'NONE',  ( 188.4359598230020651, 86.36951380984523041, 35.29673132375548050 ) ) ;
#27745=CARTESIAN_POINT ( 'NONE',  ( -75.64857587248467041, 21.19501514561448019, 17.94384578064662250 ) ) ;
#27746=CARTESIAN_POINT ( 'NONE',  ( -34.34971582436550364, 10.08696685283320704, -89.58086001246577723 ) ) ;
#27747=CARTESIAN_POINT ( 'NONE',  ( 20.36233635256088448, 7.697399815318437533, 31.55093273888049410 ) ) ;
#27756=FACE_OUTER_BOUND ( 'NONE', #61842, .T. ) ;
#27759=CARTESIAN_POINT ( 'NONE',  ( -78.66644367742109978, 22.32174330031319442, 30.41820113967310490 ) ) ;
#27760=CARTESIAN_POINT ( 'NONE',  ( 155.2992895652387517, 57.24699634758577815, -77.66147854539327966 ) ) ;
#27761=CARTESIAN_POINT ( 'NONE',  ( 45.35146934743634262, 10.27620685439442205, 42.00691914349181388 ) ) ;
#27764=B_SPLINE_CURVE_WITH_KNOTS ( 'NONE', 3,
 ( #14776, #58369, #42545, #20394, #15812, #5258, #10183, #47463, #48148, #57351, #46789, #31644, #64000, #15129, #58037, #68261, #30622, #20064, #20747, #29998, #64340, #63668, #9858, #41517, #31316, #53082, #52417, #21429, #4912, #36241, #9162, #52742, #57698, #9508, #4568, #26378, #26032, #68922, #42207, #30971, #47816, #4234, #69276, #58707 ),
 .UNSPECIFIED., .F., .F.,
 ( 4, 2, 2, 2, 2, 2, 2, 2, 2, 2, 2, 2, 2, 2, 2, 2, 2, 2, 2, 2, 2, 4 ),
 ( 0.000000000000000000, 0.001482469635030009411, 0.002223704452545014875, 0.002964939270060020123, 0.004447408905090030617, 0.005929878540120041112, 0.007412348175150052475, 0.008153582992665062493, 0.008894817810180075113, 0.01037728744521010382, 0.01185975708024013600, 0.01260099189775512954, 0.01334222671527012308, 0.01482469635030015179, 0.01556593116781516094, 0.01630716598533017009, 0.01778963562036014676, 0.01927210525539012342, 0.02001334007290511002, 0.02075457489042010009, 0.02223704452545009758, 0.02371951416048009159 ),
 .UNSPECIFIED. ) ;
#27765=CARTESIAN_POINT ( 'NONE',  ( -149.5074843970971017, 64.17983161892347255, 18.87627064943540134 ) ) ;
#27767=ORIENTED_EDGE ( 'NONE', *, *, #19229, .F. ) ;
#27770=AXIS2_PLACEMENT_3D ( 'NONE', #15607, #62763, #63452 ) ;
#27774=CARTESIAN_POINT ( 'NONE',  ( 57.07734607129820148, 11.37318329671159844, 59.55008699787213544 ) ) ;
#27775=CARTESIAN_POINT ( 'NONE',  ( 140.5011603602752359, 46.78412964631613136, 87.20346307703584898 ) ) ;
#27777=B_SPLINE_CURVE_WITH_KNOTS ( 'NONE', 3,
 ( #29064, #44167, #38921, #55075, #2329, #56835, #13912, #14602, #67055, #13569, #29744, #46607, #50852, #14266, #18848, #35027, #8648, #30101, #56474, #46960, #45924, #8297 ),
 .UNSPECIFIED., .F., .F.,
 ( 4, 2, 2, 2, 2, 2, 2, 2, 2, 2, 4 ),
 ( 8.002322828458971877E-17, 0.001318139496345188981, 0.001977209244517727418, 0.002636278992690265204, 0.003954418489035351619, 0.005272557985380436733, 0.005931627733553000541, 0.006590697481725565215, 0.007908836978070717116, 0.009226976474415867283, 0.01054511597076101918 ),
 .UNSPECIFIED. ) ;
#27781=CIRCLE ( 'NONE', #17654, 243.4957430088094839 ) ;
#27788=CARTESIAN_POINT ( 'NONE',  ( -172.3018509397888067, 86.22053936367346694, -7.900706070936963421 ) ) ;
#27789=CARTESIAN_POINT ( 'NONE',  ( 134.3182571105338923, 42.88121222759019702, 17.66579024853170665 ) ) ;
#27793=CARTESIAN_POINT ( 'NONE',  ( 85.67138972405899722, 19.09593469918313957, 2.913603581539713883 ) ) ;
#27795=CARTESIAN_POINT ( 'NONE',  ( -71.37402418445425667, 19.67651958824262337, 36.14765569274855039 ) ) ;
#27796=ORIENTED_EDGE ( 'NONE', *, *, #58489, .T. ) ;
#27799=ORIENTED_EDGE ( 'NONE', *, *, #54559, .T. ) ;
#27802=CARTESIAN_POINT ( 'NONE',  ( 91.49345572560149265, 21.13836538408682841, 4.653589174503819592 ) ) ;
#27805=VECTOR ( 'NONE', #14229, 1000.000000000000000 ) ;
#27811=CARTESIAN_POINT ( 'NONE',  ( -132.8123438040339863, 51.22132183644643533, -12.66178842039164643 ) ) ;
#27815=CARTESIAN_POINT ( 'NONE',  ( 138.2136629441929188, 45.30947856186676148, -76.49082427909780790 ) ) ;
#27819=FACE_BOUND ( 'NONE', #59372, .T. ) ;
#27821=CARTESIAN_POINT ( 'NONE',  ( -1.857619870843140397, 6.575690665396234813, -65.19364777147656298 ) ) ;
#27822=CARTESIAN_POINT ( 'NONE',  ( -180.4651598106648294, 97.28730001475651079, 66.71784663132508797 ) ) ;
#27823=CARTESIAN_POINT ( 'NONE',  ( -146.5309471467636797, 62.99917515507674892, -8.580487756379419295 ) ) ;
#27828=CARTESIAN_POINT ( 'NONE',  ( -119.9771613955297198, 43.90337778233483590, -73.87421532651727318 ) ) ;
#27829=CARTESIAN_POINT ( 'NONE',  ( -13.29455179262033226, 8.319166883236665200, 32.47767114274684985 ) ) ;
#27830=CARTESIAN_POINT ( 'NONE',  ( 157.4703587214989113, 57.65129005721576050, 17.56491688178971700 ) ) ;
#27831=CARTESIAN_POINT ( 'NONE',  ( 44.17331380303619426, 10.09560889695571895, -91.01863521069090268 ) ) ;
#27837=CARTESIAN_POINT ( 'NONE',  ( 84.05289558242220949, 19.61733656419351135, -77.21376866862176769 ) ) ;
#27838=CARTESIAN_POINT ( 'NONE',  ( 115.0394167068075149, 32.28558853680154783, 85.02507986354113712 ) ) ;
#27842=CARTESIAN_POINT ( 'NONE',  ( -54.08488990389050599, 15.46443908526321920, -77.01379507922334255 ) ) ;
#27844=CARTESIAN_POINT ( 'NONE',  ( -72.84536430560291365, 21.25605944016604809, -91.57030382287797465 ) ) ;
#27845=CARTESIAN_POINT ( 'NONE',  ( -119.6801029354224966, 43.71909921132878196, -19.77672661693413403 ) ) ;
#27848=CARTESIAN_POINT ( 'NONE',  ( 39.40195752203891999, 9.424259417798145577, 71.75838489642698903 ) ) ;
#27850=EDGE_CURVE ( 'NONE', #11578, #27916, #3354, .T. ) ;
#27852=CARTESIAN_POINT ( 'NONE',  ( -95.54114085644955878, -170.0000000000000000, 94.99999999999866418 ) ) ;
#27853=ORIENTED_EDGE ( 'NONE', *, *, #29123, .F. ) ;
#27854=CARTESIAN_POINT ( 'NONE',  ( 107.9342863085848450, 28.93180871323605885, -50.57385741719785699 ) ) ;
#27855=CARTESIAN_POINT ( 'NONE',  ( -11.14880195267006435, 7.129907723790824825, 71.20152023141297093 ) ) ;
#27856=CARTESIAN_POINT ( 'NONE',  ( -78.66644367742111399, 22.32174330031316956, -8.270900041254197532 ) ) ;
#27858=CARTESIAN_POINT ( 'NONE',  ( 40.38414441725701209, 8.538832720399536669, -8.823556192051034586 ) ) ;
#27860=FACE_BOUND ( 'NONE', #42008, .T. ) ;
#27862=CARTESIAN_POINT ( 'NONE',  ( -60.13226458141420494, 16.10241298991027392, -37.19286980334710790 ) ) ;
#27864=VECTOR ( 'NONE', #18091, 1000.000000000000000 ) ;
#27865=EDGE_CURVE ( 'NONE', #47842, #45708, #27764, .T. ) ;
#27866=VERTEX_POINT ( 'NONE', #25699 ) ;
#27869=CARTESIAN_POINT ( 'NONE',  ( 93.32228019177711076, 22.88890999585039765, -46.71524922504401900 ) ) ;
#27871=CARTESIAN_POINT ( 'NONE',  ( -180.5200658187032161, 97.35517482626558206, 10.21020346323557604 ) ) ;
#27873=CARTESIAN_POINT ( 'NONE',  ( 212.1488570093001442, 119.0116247937291689, 62.68074259173258866 ) ) ;
#27878=CARTESIAN_POINT ( 'NONE',  ( -62.49130718206700408, 16.80297926264070085, 63.67143424412796548 ) ) ;
#27880=CIRCLE ( 'NONE', #42496, 243.4957430088094839 ) ;
#27881=ORIENTED_EDGE ( 'NONE', *, *, #18646, .F. ) ;
#27884=CARTESIAN_POINT ( 'NONE',  ( 103.5839822277949764, 25.92130892112108143, 40.57116130282916799 ) ) ;
#27888=DIRECTION ( 'NONE',  ( -0.000000000000000000, 1.000000000000000000, -0.000000000000000000 ) ) ;
#27893=CARTESIAN_POINT ( 'NONE',  ( 105.8229724512851391, 27.98935528750254065, 4.202583732138563732 ) ) ;
#27895=CARTESIAN_POINT ( 'NONE',  ( 92.21267147730743829, 21.40196534721315302, 42.24347036755128926 ) ) ;
#27896=CARTESIAN_POINT ( 'NONE',  ( 103.5589117581614573, 27.00490790413960696, -13.13767299798190713 ) ) ;
#27897=CARTESIAN_POINT ( 'NONE',  ( -47.94960849910471978, 13.92522873833624963, 13.43034332784529994 ) ) ;
#27898=CARTESIAN_POINT ( 'NONE',  ( -8.679044977515172121, 7.955195573549007193, -89.10717191287118055 ) ) ;
#27899=CARTESIAN_POINT ( 'NONE',  ( -156.8684223695132971, 72.05296926946580527, -94.46708670589811163 ) ) ;
#27900=CARTESIAN_POINT ( 'NONE',  ( 63.01563776193091826, 12.67277567978495512, -89.40979201309708913 ) ) ;
#27901=CARTESIAN_POINT ( 'NONE',  ( 92.99453320039974358, 21.69191284572291778, 86.92040988721714712 ) ) ;
#27906=CARTESIAN_POINT ( 'NONE',  ( -11.57931195747592668, 7.164335452024273465, -9.562147327756052917 ) ) ;
#27907=CARTESIAN_POINT ( 'NONE',  ( -51.13073217147958616, 13.66490163179656925, 44.21480333522377748 ) ) ;
#27910=CARTESIAN_POINT ( 'NONE',  ( -37.93983213483218719, 11.77368372188051282, 68.33345614380237976 ) ) ;
#27912=CARTESIAN_POINT ( 'NONE',  ( -76.32962633615588288, 21.44528079176261670, -76.59068498040936390 ) ) ;
#27913=CARTESIAN_POINT ( 'NONE',  ( 22.53041628628729853, 6.810083298012986397, -12.85235912044543127 ) ) ;
#27914=ORIENTED_EDGE ( 'NONE', *, *, #27850, .T. ) ;
#27916=VERTEX_POINT ( 'NONE', #6994 ) ;
#27917=ORIENTED_EDGE ( 'NONE', *, *, #20307, .F. ) ;
#27920=CARTESIAN_POINT ( 'NONE',  ( -27.20808966803983608, 9.951893639754503695, 85.20453094359582735 ) ) ;
#27921=CARTESIAN_POINT ( 'NONE',  ( -97.49219489034500441, 30.41416107059310647, -48.30800170384669912 ) ) ;
#27927=ORIENTED_EDGE ( 'NONE', *, *, #42638, .T. ) ;
#27931=CARTESIAN_POINT ( 'NONE',  ( -153.6994314938755792, 69.16570456337670691, -9.232507601247755602 ) ) ;
#27932=CARTESIAN_POINT ( 'NONE',  ( 37.46254810722765427, 8.164772623042710009, -77.22570432960662856 ) ) ;
#27933=CARTESIAN_POINT ( 'NONE',  ( 62.52742438962777527, 12.55954017561948000, -8.876140241706055534 ) ) ;
#27934=CARTESIAN_POINT ( 'NONE',  ( -33.37566357177431087, 9.916833145467595756, 57.29897744571702844 ) ) ;
#27937=CARTESIAN_POINT ( 'NONE',  ( 188.2086267457324880, 87.61890531228281986, 61.29282024878416735 ) ) ;
#27940=CARTESIAN_POINT ( 'NONE',  ( -0.3740447803642804048, 7.527031846085010081, -43.90199697603654272 ) ) ;
#27941=CARTESIAN_POINT ( 'NONE',  ( -165.7699288023689235, 79.30174988963858596, 9.961564374601575622 ) ) ;
#27943=FACE_BOUND ( 'NONE', #66060, .T. ) ;
#27945=CARTESIAN_POINT ( 'NONE',  ( 204.6977192012829505, 108.0580384837234931, 56.05227132923312183 ) ) ;
#27946=CARTESIAN_POINT ( 'NONE',  ( 9.416603677636260272, 6.380307115728824030, -73.82726956336668422 ) ) ;
#27950=EDGE_LOOP ( 'NONE', ( #42788, #58196 ) ) ;
#27952=CARTESIAN_POINT ( 'NONE',  ( 177.2011275744679324, 74.76848439756737719, 30.38803117832052791 ) ) ;
#27953=PLANE ( 'NONE',  #46660 ) ;
#27954=CARTESIAN_POINT ( 'NONE',  ( 40.38414441725700499, 8.538832720399511800, -62.51265737297843827 ) ) ;
#27956=ORIENTED_EDGE ( 'NONE', *, *, #32858, .T. ) ;
#27961=EDGE_LOOP ( 'NONE', ( #60820, #46356, #10608, #40178 ) ) ;
#27962=CARTESIAN_POINT ( 'NONE',  ( 173.7227242028391174, 71.47307702680404873, -45.18960647539945796 ) ) ;
#27964=ORIENTED_EDGE ( 'NONE', *, *, #44143, .T. ) ;
#27966=CARTESIAN_POINT ( 'NONE',  ( 63.01563776193090405, 12.67277567978497643, -8.876140241706053757 ) ) ;
#27968=CARTESIAN_POINT ( 'NONE',  ( -7.825402957745085430, 6.891034867348157178, -8.573520141480125645 ) ) ;
#27969=CARTESIAN_POINT ( 'NONE',  ( -78.18913509716432486, 22.13995206110505976, -35.11545063171788428 ) ) ;
#27972=CARTESIAN_POINT ( 'NONE',  ( -30.46358361599563480, 10.45190018822943578, -8.520521904715787187 ) ) ;
#27973=CARTESIAN_POINT ( 'NONE',  ( -48.34500911884040875, 14.01939034823941377, -12.50755381913665687 ) ) ;
#27975=ORIENTED_EDGE ( 'NONE', *, *, #36448, .T. ) ;
#27976=CARTESIAN_POINT ( 'NONE',  ( 114.4640969196985907, 30.88424258798504596, -49.62645197922152107 ) ) ;
#27978=CARTESIAN_POINT ( 'NONE',  ( 43.96465529479667111, 9.046527005589345194, -49.09265818586762720 ) ) ;
#27979=CARTESIAN_POINT ( 'NONE',  ( -167.0073208999198471, 82.02183861952782706, -73.40875188435131804 ) ) ;
#27981=ORIENTED_EDGE ( 'NONE', *, *, #43344, .T. ) ;
#27982=CARTESIAN_POINT ( 'NONE',  ( 57.57684776206770749, 12.50442334002048561, 5.298377812166513934 ) ) ;
#27984=DIRECTION ( 'NONE',  ( 0.000000000000000000, 0.000000000000000000, 1.000000000000000000 ) ) ;
#27988=CARTESIAN_POINT ( 'NONE',  ( 83.38067517854670996, 18.33799117207142260, -23.24128901785653412 ) ) ;
#27989=CARTESIAN_POINT ( 'NONE',  ( 42.48820792780866640, 9.847387255477761059, 3.729320912837806201 ) ) ;
#27990=CYLINDRICAL_SURFACE ( 'NONE', #10635, 7.500000000000020428 ) ;
#27992=CARTESIAN_POINT ( 'NONE',  ( -156.3850008295872556, 70.23964984807268763, -92.99996502729436543 ) ) ;
#27995=CARTESIAN_POINT ( 'NONE',  ( 41.80536115778105710, 8.734184316430670947, 30.30514126477402570 ) ) ;
#27998=AXIS2_PLACEMENT_3D ( 'NONE', #29468, #28070, #40371 ) ;
#28000=CARTESIAN_POINT ( 'NONE',  ( 208.9585401441655961, 114.1617785893844257, -37.63730762774075345 ) ) ;
#28001=CARTESIAN_POINT ( 'NONE',  ( -71.23176719684943237, 20.69188312694500098, -68.44020852477699179 ) ) ;
#28002=CARTESIAN_POINT ( 'NONE',  ( -104.5730787903383145, 33.96058035148152499, 72.02022507236867455 ) ) ;
#28003=CARTESIAN_POINT ( 'NONE',  ( -24.93568128341084034, 8.613819379861698877, -39.04933227581432220 ) ) ;
#28011=PLANE ( 'NONE',  #15081 ) ;
#28013=CARTESIAN_POINT ( 'NONE',  ( 132.0249343950657135, 41.49728247212332377, 44.34218584777070049 ) ) ;
#28019=CARTESIAN_POINT ( 'NONE',  ( 209.7190351965047057, 113.4909703304756903, 84.81773753047731645 ) ) ;
#28022=CARTESIAN_POINT ( 'NONE',  ( 57.39233401791017997, 12.46575990788836030, 69.14437610160888426 ) ) ;
#28023=CARTESIAN_POINT ( 'NONE',  ( 10.13563904803031512, 7.391572367417534650, -64.90997110317320562 ) ) ;
#28028=B_SPLINE_CURVE_WITH_KNOTS ( 'NONE', 3,
 ( #17673, #12394, #50022, #60922, #13438, #28570, #23646, #28929, #1856, #34206, #7815, #50380, #66230, #39819, #13098, #45438, #45086, #23992, #27871, #40166, #61623, #49310, #1142, #6762, #17313, #38784, #60231, #12044, #28211, #47159, #52104, #35587, #62310, #63004, #45791, #61954, #8510, #25391, #29604, #62667, #67268, #51423, #19054, #46824 ),
 .UNSPECIFIED., .F., .F.,
 ( 4, 2, 2, 2, 2, 2, 2, 2, 2, 2, 2, 2, 2, 2, 2, 2, 2, 2, 2, 2, 2, 4 ),
 ( 0.02908143158676660539, 0.03095422299093868179, 0.03282701439511075819, 0.03469980579928283460, 0.03657259720345491100, 0.03844538860762698740, 0.04031818001179907074, 0.04125457571388507771, 0.04219097141597108469, 0.04312736711805709861, 0.04359556496910010209, 0.04406376282014311252, 0.04500015852222912643, 0.04593655422431514035, 0.04687294992640115426, 0.04780934562848716818, 0.04968213703265923764, 0.05155492843683130710, 0.05342771984100337657, 0.05530051124517543909, 0.05717330264934750855, 0.05904609405351957108 ),
 .UNSPECIFIED. ) ;
#28039=CARTESIAN_POINT ( 'NONE',  ( -132.0738857626834601, 51.93126104279146205, -46.67044353618173602 ) ) ;
#28041=CARTESIAN_POINT ( 'NONE',  ( -118.9468627709229480, 42.08677365399180559, -39.57500987869580911 ) ) ;
#28043=CARTESIAN_POINT ( 'NONE',  ( -142.6264002846224059, 58.55577336362198082, -18.46366008300287120 ) ) ;
#28044=CARTESIAN_POINT ( 'NONE',  ( -142.5336480376679162, 58.48275793139958267, 94.69040015390055487 ) ) ;
#28046=ORIENTED_EDGE ( 'NONE', *, *, #42848, .T. ) ;
#28048=CARTESIAN_POINT ( 'NONE',  ( 198.7029050523552485, 98.46895521196212542, -39.29008233195586541 ) ) ;
#28052=CARTESIAN_POINT ( 'NONE',  ( -56.02358673658417132, 14.94347049174937503, 3.520221774332097375 ) ) ;
#28053=ORIENTED_EDGE ( 'NONE', *, *, #44367, .T. ) ;
#28057=ORIENTED_EDGE ( 'NONE', *, *, #27605, .F. ) ;
#28058=CARTESIAN_POINT ( 'NONE',  ( -72.76696720809547969, 20.16136115364207981, -11.11340259104759554 ) ) ;
#28060=CARTESIAN_POINT ( 'NONE',  ( -15.13211202216340467, 8.488266782358831364, -71.47197618211744441 ) ) ;
#28063=CARTESIAN_POINT ( 'NONE',  ( 181.0840389613909451, 80.03940679743416808, -36.22505766587961062 ) ) ;
#28068=CARTESIAN_POINT ( 'NONE',  ( -38.84150381976579780, 10.92416363971238980, -17.20362598305740320 ) ) ;
#28069=CARTESIAN_POINT ( 'NONE',  ( 151.7977579753110433, 53.37137838551321778, -92.38936414380266626 ) ) ;
#28070=DIRECTION ( 'NONE',  ( -0.000000000000000000, 1.000000000000000000, -0.000000000000000000 ) ) ;
#28071=CARTESIAN_POINT ( 'NONE',  ( 18.43272992546528499, 7.606837839440253823, 71.38188367849733140 ) ) ;
#28077=CARTESIAN_POINT ( 'NONE',  ( -105.4487797565983840, 35.55724615608637862, 4.360698117697985765 ) ) ;
#28080=CARTESIAN_POINT ( 'NONE',  ( -38.93922791710217268, 10.94334660650242341, -43.05910848483384967 ) ) ;
#28082=DIRECTION ( 'NONE',  ( -0.000000000000000000, 1.000000000000000000, -0.000000000000000000 ) ) ;
#28084=CARTESIAN_POINT ( 'NONE',  ( -78.18897186942403721, 23.21604822208489338, -8.270900041254201085 ) ) ;
#28086=CARTESIAN_POINT ( 'NONE',  ( 80.30232379693109124, 17.35837133860834314, 60.02175339020114819 ) ) ;
#28087=ORIENTED_EDGE ( 'NONE', *, *, #36274, .F. ) ;
#28091=CARTESIAN_POINT ( 'NONE',  ( 181.9295719569814196, 79.46350097013163349, 29.34415077797327953 ) ) ;
#28093=CARTESIAN_POINT ( 'NONE',  ( -73.63346300764936814, 20.46798018699518806, 5.507808174618403996 ) ) ;
#28094=CARTESIAN_POINT ( 'NONE',  ( -118.6302575928420424, 43.07263081214306055, 66.85160587967178003 ) ) ;
#28095=ADVANCED_FACE ( 'NONE', ( #51310 ), #40733, .F. ) ;
#28098=CARTESIAN_POINT ( 'NONE',  ( 154.6667526376337207, 55.50347409140649546, -36.66424293194626216 ) ) ;
#28107=CARTESIAN_POINT ( 'NONE',  ( -79.14678386417816114, 22.50468917936073154, 45.41820113967313688 ) ) ;
#28108=CARTESIAN_POINT ( 'NONE',  ( -30.46002654261638298, 10.45132580906815356, -77.11350681613473057 ) ) ;
#28109=CARTESIAN_POINT ( 'NONE',  ( 44.34689728705970424, 10.12166135033765357, 43.07394473429382487 ) ) ;
#28110=CARTESIAN_POINT ( 'NONE',  ( -28.81317668042940383, 9.175023678939295380, 57.53151503497319652 ) ) ;
#28111=ADVANCED_FACE ( 'NONE', ( #55523 ), #61835, .F. ) ;
#28118=CARTESIAN_POINT ( 'NONE',  ( 36.30999198706538067, 9.040534725358945423, -9.437934728592482614 ) ) ;
#28121=CARTESIAN_POINT ( 'NONE',  ( -0.5783162822156577842, 7.534184941292926041, 66.40692524127545937 ) ) ;
#28122=CARTESIAN_POINT ( 'NONE',  ( -24.26658464276621885, 9.538695081344586768, -94.14796338366534201 ) ) ;
#28125=CARTESIAN_POINT ( 'NONE',  ( 15.78827728214693416, 6.500811158483329244, 45.01470767270524931 ) ) ;
#28128=CARTESIAN_POINT ( 'NONE',  ( 164.8942204024297951, 63.66138186734712434, -15.67721590130059717 ) ) ;
#28131=CARTESIAN_POINT ( 'NONE',  ( 138.1901928158493718, 45.29454828899443442, 16.30506375331225755 ) ) ;
#28135=CARTESIAN_POINT ( 'NONE',  ( 81.74909803672913711, 17.81295302817861881, 4.650954357442839360 ) ) ;
#28140=ORIENTED_EDGE ( 'NONE', *, *, #30818, .F. ) ;
#28143=CARTESIAN_POINT ( 'NONE',  ( 94.06703982324147262, 22.09435144471462920, 11.36492375468983340 ) ) ;
#28147=CARTESIAN_POINT ( 'NONE',  ( 58.97837225874348377, 12.80135346511094774, 84.67264224153834107 ) ) ;
#28148=CARTESIAN_POINT ( 'NONE',  ( 34.45158752686798209, 8.829194381142002612, 43.06926157878825023 ) ) ;
#28149=CARTESIAN_POINT ( 'NONE',  ( -178.2328124332056234, 94.56955476227571467, -47.72005399664082859 ) ) ;
#28150=CARTESIAN_POINT ( 'NONE',  ( -180.3582430093886728, 97.15509181467152189, -93.85725392925826327 ) ) ;
#28155=CARTESIAN_POINT ( 'NONE',  ( -147.3669217311067712, 63.69361261596463919, -76.34879821478752149 ) ) ;
#28157=DIRECTION ( 'NONE',  ( -0.000000000000000000, 1.000000000000000000, -0.000000000000000000 ) ) ;
#28165=CARTESIAN_POINT ( 'NONE',  ( -121.5680658099884397, 44.89994870382100345, -75.40337873448993378 ) ) ;
#28167=CARTESIAN_POINT ( 'NONE',  ( -12.40598104375063038, 8.242193636955557068, 43.57465072453484822 ) ) ;
#28168=CARTESIAN_POINT ( 'NONE',  ( 157.9160637431159557, 57.99786926216935967, 17.56491688178972055 ) ) ;
#28169=CARTESIAN_POINT ( 'NONE',  ( 46.19578020946207175, 10.40950134816946537, -93.62501912019730810 ) ) ;
#28170=ORIENTED_EDGE ( 'NONE', *, *, #17306, .T. ) ;
#28171=CARTESIAN_POINT ( 'NONE',  ( -32.40928421737413601, 10.77259363352673205, 3.418817049811458730 ) ) ;
#28175=CARTESIAN_POINT ( 'NONE',  ( 84.97658021689289853, 19.92447159015899771, -77.48566349683447640 ) ) ;
#28176=CARTESIAN_POINT ( 'NONE',  ( 109.9676357272098244, 29.86308433357949355, 83.29856572268397485 ) ) ;
#28177=CARTESIAN_POINT ( 'NONE',  ( -173.1211646369891071, 87.12891641440859303, 3.977144016177345254 ) ) ;
#28179=CARTESIAN_POINT ( 'NONE',  ( -14.86660400085235345, 7.452266534569882417, 88.70135958064247461 ) ) ;
#28184=DIRECTION ( 'NONE',  ( -0.000000000000000000, 1.000000000000000000, -0.000000000000000000 ) ) ;
#28186=ORIENTED_EDGE ( 'NONE', *, *, #27544, .T. ) ;
#28187=EDGE_LOOP ( 'NONE', ( #29440, #61531 ) ) ;
#28188=CARTESIAN_POINT ( 'NONE',  ( 31.96192885395476324, 8.569232728322420556, 65.23638710323480439 ) ) ;
#28189=CARTESIAN_POINT ( 'NONE',  ( 175.5406524085944966, 73.17873692326774915, 58.57573781641595190 ) ) ;
#28192=CARTESIAN_POINT ( 'NONE',  ( -165.7690020878297901, 80.74028011998679233, 63.65475612973403940 ) ) ;
#28193=CARTESIAN_POINT ( 'NONE',  ( -165.6397095829521504, 80.60756690931940227, -15.97658641783072930 ) ) ;
#28198=B_SPLINE_CURVE_WITH_KNOTS ( 'NONE', 3,
 ( #42550, #68927, #53434, #63671, #64699, #26382, #20751, #16508, #37966, #54113, #59064, #59409, #11221, #58376, #65048, #10186, #16157, #42879, #16846, #31649, #5263, #683, #47820, #38305, #31322, #52747, #4572, #69281, #15819, #22481, #23190, #49901, #1374, #33743, #12631, #2087, #44272, #49193, #7360, #54471, #18249, #55178, #39360, #43918 ),
 .UNSPECIFIED., .F., .F.,
 ( 4, 2, 2, 2, 2, 2, 2, 2, 2, 2, 2, 2, 2, 2, 2, 2, 2, 2, 2, 2, 2, 4 ),
 ( 0.000000000000000000, 0.003360573201437605691, 0.004200716501796969600, 0.005040859802156333509, 0.006721146402875015358, 0.007561289703234363654, 0.008401433003593711951, 0.009241576303953058513, 0.01008171960431240508, 0.01176200620503115198, 0.01260214950539053497, 0.01344229280574991969, 0.01428243610610930268, 0.01512257940646868741, 0.01680286600718746901, 0.01764300930754684679, 0.01848315260790622805, 0.02016343920862500791, 0.02184372580934379124, 0.02352401241006257110, 0.02520429901078135443, 0.02688458561150013429 ),
 .UNSPECIFIED. ) ;
#28199=CARTESIAN_POINT ( 'NONE',  ( 93.32228019177713918, 22.88890999585040831, 6.973851955883334064 ) ) ;
#28202=CARTESIAN_POINT ( 'NONE',  ( -83.74134668872638088, 25.40628965235943681, -90.76525586021888614 ) ) ;
#28204=CARTESIAN_POINT ( 'NONE',  ( 8.000000000000007105, 249.8719672152120381, 94.99999999999866418 ) ) ;
#28205=FACE_BOUND ( 'NONE', #46801, .T. ) ;
#28207=ORIENTED_EDGE ( 'NONE', *, *, #4846, .F. ) ;
#28210=CARTESIAN_POINT ( 'NONE',  ( -48.58279704072702287, 14.07632445131079812, 68.46338809851388874 ) ) ;
#28211=CARTESIAN_POINT ( 'NONE',  ( -180.2243452982808947, 96.99029284948629481, 13.90186183527965547 ) ) ;
#28212=CARTESIAN_POINT ( 'NONE',  ( 208.5884523568771556, 113.6152425727544824, 69.97810575574392544 ) ) ;
#28215=CARTESIAN_POINT ( 'NONE',  ( 56.30171512200999473, 11.21502580416398764, 13.82023505722669476 ) ) ;
#28216=CARTESIAN_POINT ( 'NONE',  ( -61.52143283897135717, 16.51181063611434752, 60.85814816128657156 ) ) ;
#28218=ORIENTED_EDGE ( 'NONE', *, *, #40051, .F. ) ;
#28219=CARTESIAN_POINT ( 'NONE',  ( 133.8566784816069344, -170.0000000000000000, 2.665790248531674678 ) ) ;
#28220=CARTESIAN_POINT ( 'NONE',  ( -61.10880364359507411, 17.43879918625640002, -20.30299724292251184 ) ) ;
#28221=CARTESIAN_POINT ( 'NONE',  ( 87.58754341703161117, 20.81465688423120142, -62.71234923768123792 ) ) ;
#28225=CARTESIAN_POINT ( 'NONE',  ( 36.09137906183517686, 8.001963043161762101, -23.00953966251914906 ) ) ;
#28226=CARTESIAN_POINT ( 'NONE',  ( 164.8914542114683570, 64.97670918603525081, 35.78822635281908759 ) ) ;
#28228=CARTESIAN_POINT ( 'NONE',  ( 68.94948716683070700, 15.16699441119058100, 5.855287509081221309 ) ) ;
#28229=CARTESIAN_POINT ( 'NONE',  ( -190.6985136298601731, 109.1272424661242582, 94.99999999999866418 ) ) ;
#28237=CARTESIAN_POINT ( 'NONE',  ( -50.14440374537738876, 14.45628984983895293, 16.66475555544458587 ) ) ;
#28247=CARTESIAN_POINT ( 'NONE',  ( -166.5879373373658154, 81.58564870376412159, 88.31158596434660524 ) ) ;
#28248=CARTESIAN_POINT ( 'NONE',  ( -51.77439426130689526, 13.82695438436703839, -9.121836570883877116 ) ) ;
#28251=CARTESIAN_POINT ( 'NONE',  ( -62.15063206372443716, 17.75106610013996189, -45.18927541931358149 ) ) ;
#28253=DIRECTION ( 'NONE',  ( 0.000000000000000000, 0.000000000000000000, 1.000000000000000000 ) ) ;
#28254=CARTESIAN_POINT ( 'NONE',  ( -71.22878586122430988, 19.62649588091169406, -68.46191443494774376 ) ) ;
#28255=CARTESIAN_POINT ( 'NONE',  ( 19.11168290073779730, 6.629794975642855803, -9.446444181573534493 ) ) ;
#28260=CARTESIAN_POINT ( 'NONE',  ( 66.73431804020508196, 14.60294556126670429, -22.89389229214575394 ) ) ;
#28261=CARTESIAN_POINT ( 'NONE',  ( -60.43316470166142551, 17.23897012780379612, -91.17587151978018767 ) ) ;
#28262=CARTESIAN_POINT ( 'NONE',  ( -24.07246351276930696, 9.512772164140772091, 89.95986364399971080 ) ) ;
#28264=CARTESIAN_POINT ( 'NONE',  ( 113.8724110608469431, 31.71510301790681652, -23.15866281951693750 ) ) ;
#28267=CARTESIAN_POINT ( 'NONE',  ( 138.1901928158493433, 45.29454828899443442, -10.53948683715141854 ) ) ;
#28274=CARTESIAN_POINT ( 'NONE',  ( 57.07734607129817306, 11.37318329671159134, -20.98356477351893901 ) ) ;
#28285=CARTESIAN_POINT ( 'NONE',  ( 185.1660960081724170, 84.30194217633010112, 57.35720483677989989 ) ) ;
#28286=CARTESIAN_POINT ( 'NONE',  ( 176.6214367443247966, 74.20967084876663478, -64.52294413732886369 ) ) ;
#28289=CARTESIAN_POINT ( 'NONE',  ( -1.327237339234996982, 7.561837009978233048, -39.16517982428524647 ) ) ;
#28291=CARTESIAN_POINT ( 'NONE',  ( -166.7049310409072120, 80.25944422923579680, 15.36979968814921627 ) ) ;
#28293=FACE_BOUND ( 'NONE', #64077, .T. ) ;
#28299=CARTESIAN_POINT ( 'NONE',  ( -133.2698123908828336, 51.54642138335022139, -67.87415851310558423 ) ) ;
#28301=CARTESIAN_POINT ( 'NONE',  ( 46.64694836521739063, 9.462741877720628025, -71.91924328827956003 ) ) ;
#28304=ORIENTED_EDGE ( 'NONE', *, *, #10065, .T. ) ;
#28305=CARTESIAN_POINT ( 'NONE',  ( -127.5425607999732307, 47.58841438093516274, -88.77439082497835443 ) ) ;
#28306=CARTESIAN_POINT ( 'NONE',  ( 187.1633130089971644, 84.97574503406409008, 86.09156961515144246 ) ) ;
#28307=VERTEX_POINT ( 'NONE', #15393 ) ;
#28308=ORIENTED_EDGE ( 'NONE', *, *, #5489, .T. ) ;
#28309=CARTESIAN_POINT ( 'NONE',  ( 173.6710158776850506, 71.42507420636738402, -44.90187336702329191 ) ) ;
#28310=CARTESIAN_POINT ( 'NONE',  ( 162.8034185388970627, 63.22443559329410334, 4.769821300519481611 ) ) ;
#28314=CARTESIAN_POINT ( 'NONE',  ( 141.0792860804900499, 47.16255757051797559, 61.76377827337359605 ) ) ;
#28315=CARTESIAN_POINT ( 'NONE',  ( -71.97434903038468690, 19.88430675376531909, -46.03817687804183123 ) ) ;
#28316=CARTESIAN_POINT ( 'NONE',  ( -109.0191069781766657, 37.48620563201052391, 94.99999999999866418 ) ) ;
#28318=CARTESIAN_POINT ( 'NONE',  ( -49.13048465129991627, 14.20828170588045758, -11.24350225477614629 ) ) ;
#28321=CARTESIAN_POINT ( 'NONE',  ( 115.7561705820729259, 31.51689401996058493, -48.53024572195440101 ) ) ;
#28322=ADVANCED_FACE ( 'NONE', ( #47383 ), #15734, .F. ) ;
#28323=B_SPLINE_CURVE_WITH_KNOTS ( 'NONE', 3,
 ( #1513, #27899, #50404, #33881, #54620, #12423, #55673, #1167, #7506, #59890, #28959, #6448, #2221, #49334, #43709, #22621, #60257, #45114, #66597, #55319, #65542, #65187, #17338, #38453 ),
 .UNSPECIFIED., .F., .F.,
 ( 4, 2, 2, 2, 2, 2, 2, 2, 2, 2, 2, 4 ),
 ( 0.000000000000000000, 0.001596609432691784665, 0.002394914149037695103, 0.003193218865383606192, 0.003991523581729517281, 0.004789828298075427503, 0.006386437730767201108, 0.007184742447113077503, 0.007983047163458954765, 0.009579656596150731840, 0.01117626602884251238, 0.01277287546153429119 ),
 .UNSPECIFIED. ) ;
#28324=CARTESIAN_POINT ( 'NONE',  ( -72.35078170365746075, 21.08176362823952843, 7.021010477035512842 ) ) ;
#28325=CARTESIAN_POINT ( 'NONE',  ( -144.7530445311634253, 61.54314312182906832, -48.11838420148568218 ) ) ;
#28327=CARTESIAN_POINT ( 'NONE',  ( -122.3638092602184457, 44.21314101515333306, 85.18516341637682387 ) ) ;
#28329=CARTESIAN_POINT ( 'NONE',  ( 59.29474530993689285, 12.86968658439548285, 16.98489541084898491 ) ) ;
#28330=AXIS2_PLACEMENT_3D ( 'NONE', #58322, #15767, #16460 ) ;
#28333=CARTESIAN_POINT ( 'NONE',  ( -149.0782809666403352, 63.81577337591401289, 57.56537183036275707 ) ) ;
#28337=CARTESIAN_POINT ( 'NONE',  ( 183.9986899696430669, 81.60141257362812439, -23.80433703628514763 ) ) ;
#28339=EDGE_CURVE ( 'NONE', #4867, #33777, #13033, .T. ) ;
#28340=CARTESIAN_POINT ( 'NONE',  ( 138.6020257460769187, 44.36414356192206299, -10.85064934410134008 ) ) ;
#28342=CARTESIAN_POINT ( 'NONE',  ( 91.11342358617751813, 21.00000175105272149, -76.18291065189346511 ) ) ;
#28346=ORIENTED_EDGE ( 'NONE', *, *, #25680, .F. ) ;
#28347=EDGE_CURVE ( 'NONE', #61401, #59876, #13448, .T. ) ;
#28348=CARTESIAN_POINT ( 'NONE',  ( 41.33692564073607656, 8.668977654195481719, 30.16360919430110599 ) ) ;
#28352=DIRECTION ( 'NONE',  ( -0.000000000000000000, 1.000000000000000000, -0.000000000000000000 ) ) ;
#28353=CARTESIAN_POINT ( 'NONE',  ( 212.1976655298228707, 119.0878071902807847, -44.00379268766470631 ) ) ;
#28354=CARTESIAN_POINT ( 'NONE',  ( 204.6977192012829789, -170.0000000000000000, -36.32593103262158252 ) ) ;
#28356=FACE_OUTER_BOUND ( 'NONE', #57031, .T. ) ;
#28359=CARTESIAN_POINT ( 'NONE',  ( -25.80443741485377984, 9.749985135376002532, 15.84590824961209066 ) ) ;
#28360=VERTEX_POINT ( 'NONE', #10794 ) ;
#28362=CARTESIAN_POINT ( 'NONE',  ( -86.11780422997766493, 25.30122877727817254, 92.52076852176431032 ) ) ;
#28364=CARTESIAN_POINT ( 'NONE',  ( 127.4992165631961569, 38.87141012667724027, 32.99998151848554073 ) ) ;
#28368=EDGE_CURVE ( 'NONE', #29554, #347, #2933, .T. ) ;
#28371=CARTESIAN_POINT ( 'NONE',  ( 212.1962697089473693, 117.2293607936260429, 90.12784865809409496 ) ) ;
#28373=CARTESIAN_POINT ( 'NONE',  ( 55.51637278631174155, 12.08345311280959500, 63.64786402826049994 ) ) ;
#28375=CARTESIAN_POINT ( 'NONE',  ( -12.40598104375063215, 8.242193636955555291, 16.73010013407117214 ) ) ;
#28379=CARTESIAN_POINT ( 'NONE',  ( -95.39402268064687007, 29.41819732823228861, -93.22295461411728468 ) ) ;
#28384=CARTESIAN_POINT ( 'NONE',  ( -37.05762690088739930, 11.60527003175541161, -47.79140132144340214 ) ) ;
#28385=CARTESIAN_POINT ( 'NONE',  ( -167.6566265204789943, 82.70140535081090150, -37.06906935447201334 ) ) ;
#28386=CARTESIAN_POINT ( 'NONE',  ( -179.0096683247334681, 93.93079036873261600, 87.35646014482341570 ) ) ;
#28390=CARTESIAN_POINT ( 'NONE',  ( 39.40195752203892710, 9.424259417798134919, 29.91383430596324899 ) ) ;
#28391=CARTESIAN_POINT ( 'NONE',  ( -148.6426981422629012, 63.44891673852540492, -22.93093452246228026 ) ) ;
#28393=CARTESIAN_POINT ( 'NONE',  ( -4.506365319453816909, 7.705038994660851515, -76.49273962913744640 ) ) ;
#28397=CARTESIAN_POINT ( 'NONE',  ( 159.2802156694726534, 60.35763705070695551, -90.02572906011900500 ) ) ;
#28398=CARTESIAN_POINT ( 'NONE',  ( 201.6034029841262338, 102.1956603101140644, -36.98047612985361354 ) ) ;
#28399=CARTESIAN_POINT ( 'NONE',  ( -96.45303203827903360, 31.03218867996498531, 42.76688867157084672 ) ) ;
#28401=CARTESIAN_POINT ( 'NONE',  ( 15.78827728214693416, 6.500811158483284835, -50.51894409868581448 ) ) ;
#28402=CARTESIAN_POINT ( 'NONE',  ( 114.6659427952414489, 32.10199811723106222, 16.34235119158301330 ) ) ;
#28404=CARTESIAN_POINT ( 'NONE',  ( 175.5429257635131250, 74.57009623370761631, 68.73334881941738672 ) ) ;
#28407=CARTESIAN_POINT ( 'NONE',  ( -72.20490592113145567, 19.96451062593609649, -11.93102570283482855 ) ) ;
#28412=CARTESIAN_POINT ( 'NONE',  ( 164.9697211531230039, 63.72502658717167634, 36.61266077936287644 ) ) ;
#28413=DIRECTION ( 'NONE',  ( 0.000000000000000000, 0.000000000000000000, 1.000000000000000000 ) ) ;
#28416=CARTESIAN_POINT ( 'NONE',  ( -146.3632089724601144, 62.86016173369542059, -89.17980501507723545 ) ) ;
#28418=CARTESIAN_POINT ( 'NONE',  ( -38.26497993382595553, 10.81185389040525635, -12.85537468134073080 ) ) ;
#28419=CARTESIAN_POINT ( 'NONE',  ( -180.2243452982808947, 96.99029284948633745, 40.74641242574331557 ) ) ;
#28420=CARTESIAN_POINT ( 'NONE',  ( 130.3035708464390439, 40.48418876551455270, 70.47724502307815442 ) ) ;
#28421=EDGE_CURVE ( 'NONE', #46743, #51410, #59663, .T. ) ;
#28431=CARTESIAN_POINT ( 'NONE',  ( -31.43908319763709969, 10.61114334766716105, 30.21645440618916112 ) ) ;
#28434=DIRECTION ( 'NONE',  ( 0.000000000000000000, 0.000000000000000000, 1.000000000000000000 ) ) ;
#28437=CARTESIAN_POINT ( 'NONE',  ( -133.2698123908828336, 51.54642138335022139, 66.34859443921281752 ) ) ;
#28438=CARTESIAN_POINT ( 'NONE',  ( -74.18622060908361959, 21.73430079572373330, -21.80510037720168270 ) ) ;
#28439=ORIENTED_EDGE ( 'NONE', *, *, #36220, .F. ) ;
#28441=CARTESIAN_POINT ( 'NONE',  ( 81.74909803672915132, 17.81295302817863302, 58.34005553837022262 ) ) ;
#28442=EDGE_LOOP ( 'NONE', ( #54313, #53668 ) ) ;
#28443=CARTESIAN_POINT ( 'NONE',  ( -96.05874693101999640, 30.84461336787882502, -92.00895264577386001 ) ) ;
#28445=CARTESIAN_POINT ( 'NONE',  ( 63.01563776193091826, -170.0000000000000000, -96.90979201309711755 ) ) ;
#28449=CARTESIAN_POINT ( 'NONE',  ( 204.6977192012829789, 108.0580384837235073, -63.17048162308526571 ) ) ;
#28451=CARTESIAN_POINT ( 'NONE',  ( -54.08504625707234226, 14.42374043447187404, 18.42598598950144861 ) ) ;
#28457=B_SPLINE_CURVE_WITH_KNOTS ( 'NONE', 3,
 ( #21705, #27324, #954, #602, #22058, #64978, #66636, #54397, #16774, #18434, #2605, #43154, #5531, #43847, #13165, #38233, #18780, #34633, #64625, #10809, #32278, #53708, #16438, #37894, #6219, #59674, #14539, #52513, #47227, #57795, #68685, #67331, #19823, #25458, #3297, #20161, #36342, #41275, #51823, #9614, #40239, #62383, #19119, #51140 ),
 .UNSPECIFIED., .F., .F.,
 ( 4, 2, 2, 2, 2, 2, 2, 2, 2, 2, 2, 2, 2, 2, 2, 2, 2, 2, 2, 2, 2, 4 ),
 ( 6.938893903907228378E-18, 0.001472974678681662894, 0.002209462018022494666, 0.002945949357363326655, 0.004418924036045004944, 0.005891898714726683667, 0.007364873393408363257, 0.008101360732749184404, 0.008837848072090008153, 0.01031082275077161575, 0.01178379742945322335, 0.01252028476879400720, 0.01325677210813478932, 0.01472974678681635181, 0.01546623412615715995, 0.01620272146549796982, 0.01767569614417961385, 0.01914867082286125788, 0.01988515816220207469, 0.02062164550154288803, 0.02209462018022450430, 0.02356759485890611364 ),
 .UNSPECIFIED. ) ;
#28458=DIRECTION ( 'NONE',  ( -0.000000000000000000, 1.000000000000000000, -0.000000000000000000 ) ) ;
#28465=CARTESIAN_POINT ( 'NONE',  ( -86.09999398724993114, 25.29376521564873670, 38.94662278282052625 ) ) ;
#28466=CARTESIAN_POINT ( 'NONE',  ( 150.0980941434704619, 53.37942190380066165, -71.87366452615613355 ) ) ;
#28467=CARTESIAN_POINT ( 'NONE',  ( 59.95259601283825646, 11.98300577492408259, -50.07103179405425664 ) ) ;
#28468=CARTESIAN_POINT ( 'NONE',  ( 137.3958226571046737, 43.60243650158412265, -50.15227799746330106 ) ) ;
#28469=ORIENTED_EDGE ( 'NONE', *, *, #7309, .F. ) ;
#28473=CARTESIAN_POINT ( 'NONE',  ( 35.65622260226241025, 8.964590916200318560, -9.772986381556050262 ) ) ;
#28476=CARTESIAN_POINT ( 'NONE',  ( 136.9486907385599750, 44.50999891875532910, 83.85916308499764682 ) ) ;
#28477=CARTESIAN_POINT ( 'NONE',  ( -24.09190246691234805, 9.515371887976103338, -95.00000000000133582 ) ) ;
#28483=DIRECTION ( 'NONE',  ( -0.000000000000000000, 1.000000000000000000, -0.000000000000000000 ) ) ;
#28487=B_SPLINE_CURVE_WITH_KNOTS ( 'NONE', 3,
 ( #8784, #14401, #24958, #67517, #35851, #57305, #52368, #31270, #62928, #18976, #68211, #14728, #61870, #40427, #20021, #20349, #52023, #9463, #41818, #9810, #9115, #25308, #30573, #13698, #3837, #46739, #36194, #19316, #30924, #35150, #40771, #14044, #35503, #25653, #63272, #56964, #15080, #36543, #54064, #11172 ),
 .UNSPECIFIED., .F., .F.,
 ( 4, 2, 2, 2, 2, 2, 2, 2, 2, 2, 2, 2, 2, 2, 2, 2, 2, 2, 2, 4 ),
 ( 0.02454308262169000235, 0.02608670964102868459, 0.02685852315069804305, 0.02763033666036740499, 0.02917396367970614274, 0.02994577718937551161, 0.03071759069904488049, 0.03226121771838367375, 0.03303303122805310160, 0.03380484473772252946, 0.03534847175706141986, 0.03689209877640031721, 0.03843572579573920067, 0.03997935281507809802, 0.04152297983441698148, 0.04306660685375587189, 0.04461023387309476229, 0.04615386089243365270, 0.04769748791177254310, 0.04924111493111143351 ),
 .UNSPECIFIED. ) ;
#28488=CARTESIAN_POINT ( 'NONE',  ( -133.2386331335365242, 52.76072997738348391, -94.50456680151590660 ) ) ;
#28489=CARTESIAN_POINT ( 'NONE',  ( -190.6985136298601731, 109.1272424661242582, 94.99999999999866418 ) ) ;
#28494=EDGE_CURVE ( 'NONE', #51562, #27030, #32141, .T. ) ;
#28495=ORIENTED_EDGE ( 'NONE', *, *, #44221, .T. ) ;
#28496=AXIS2_PLACEMENT_3D ( 'NONE', #52854, #58154, #52184 ) ;
#28497=CARTESIAN_POINT ( 'NONE',  ( 15.78827728214693416, 6.500811158483329244, 45.01470767270524931 ) ) ;
#28499=EDGE_CURVE ( 'NONE', #5653, #44052, #50128, .T. ) ;
#28502=AXIS2_PLACEMENT_3D ( 'NONE', #42883, #10532, #52750 ) ;
#28504=CARTESIAN_POINT ( 'NONE',  ( -148.6426981422628728, 63.44891673852540492, -76.62003570338966085 ) ) ;
#28505=CARTESIAN_POINT ( 'NONE',  ( 89.22118407503263882, 20.32164250407901207, 17.40952166681993063 ) ) ;
#28510=CARTESIAN_POINT ( 'NONE',  ( 38.42095780754793566, 9.297684251045559733, 44.86571034329109153 ) ) ;
#28511=CARTESIAN_POINT ( 'NONE',  ( -179.5109681715918555, 96.11572638569522553, -46.17695725115778771 ) ) ;
#28513=CARTESIAN_POINT ( 'NONE',  ( -149.1099326198686583, 63.84262089027424736, -88.50193171241930656 ) ) ;
#28515=CARTESIAN_POINT ( 'NONE',  ( 127.4953815656694758, 37.71366486045442912, -66.36346676285383239 ) ) ;
#28517=CARTESIAN_POINT ( 'NONE',  ( 138.5943620234098717, 45.55242290395135285, -76.20239256362549440 ) ) ;
#28520=VERTEX_POINT ( 'NONE', #2343 ) ;
#28521=CARTESIAN_POINT ( 'NONE',  ( -149.5074843970971017, 65.50121172469319220, -49.81283053149199702 ) ) ;
#28522=CARTESIAN_POINT ( 'NONE',  ( -4.081377963939778475, 6.676029627840592617, -76.26587694573117915 ) ) ;
#28523=CARTESIAN_POINT ( 'NONE',  ( -38.93847286785604211, 11.96870349976818204, 37.20973207589809562 ) ) ;
#28526=LINE ( 'NONE', #44343, #58001 ) ;
#28527=CARTESIAN_POINT ( 'NONE',  ( -11.10395507987084329, 7.126520090179309541, -89.84858484025937742 ) ) ;
#28530=CARTESIAN_POINT ( 'NONE',  ( -11.57950265606958418, 8.174070387114797498, 44.11303985588816090 ) ) ;
#28531=CARTESIAN_POINT ( 'NONE',  ( 117.7411475730015269, 32.50808475802731579, 9.724032258917603144 ) ) ;
#28533=ORIENTED_EDGE ( 'NONE', *, *, #29174, .T. ) ;
#28535=CARTESIAN_POINT ( 'NONE',  ( -95.60805465865863084, 30.63099276904602775, -45.97777768882416893 ) ) ;
#28539=CARTESIAN_POINT ( 'NONE',  ( 39.89571693415784637, 8.473773298340393723, 71.75838489642697482 ) ) ;
#28544=CARTESIAN_POINT ( 'NONE',  ( 62.20483532083785860, 13.51802415804941937, -89.44279409927861479 ) ) ;
#28545=CARTESIAN_POINT ( 'NONE',  ( -124.7710763417278201, 46.96042092553521030, -22.98812073115930232 ) ) ;
#28551=CARTESIAN_POINT ( 'NONE',  ( 174.1251613516844259, 71.84747073139214990, 66.50424727365492572 ) ) ;
#28553=CARTESIAN_POINT ( 'NONE',  ( -166.0031475600389115, 80.98114714564771077, 67.54672357681444339 ) ) ;
#28555=CARTESIAN_POINT ( 'NONE',  ( -166.2065256787326177, 81.19093426984588291, -12.44839775261722181 ) ) ;
#28558=EDGE_LOOP ( 'NONE', ( #52748, #23368 ) ) ;
#28559=CARTESIAN_POINT ( 'NONE',  ( 109.3154830994003532, 29.56170298203815605, -50.87960775427016813 ) ) ;
#28560=CARTESIAN_POINT ( 'NONE',  ( 157.4703587214989113, 57.65129005721576050, -62.96873488960130771 ) ) ;
#28561=CARTESIAN_POINT ( 'NONE',  ( 15.29912143387263690, 7.491799981865499447, 56.85925826316893250 ) ) ;
#28563=DIRECTION ( 'NONE',  ( -0.000000000000000000, 1.000000000000000000, -0.000000000000000000 ) ) ;
#28564=FACE_BOUND ( 'NONE', #68626, .T. ) ;
#28565=CARTESIAN_POINT ( 'NONE',  ( -62.30100056228381789, 16.74548393487071252, -40.72482722506486397 ) ) ;
#28568=CARTESIAN_POINT ( 'NONE',  ( 87.10672734544985474, 20.64813880796636170, -50.82156419891173016 ) ) ;
#28570=CARTESIAN_POINT ( 'NONE',  ( -175.9864315813574080, 91.91454246454364352, 4.533208682208026197 ) ) ;
#28571=CARTESIAN_POINT ( 'NONE',  ( 205.5130322755755401, 109.1888880665735542, 71.05227132923313604 ) ) ;
#28572=CARTESIAN_POINT ( 'NONE',  ( 84.05098130332766004, 18.55728792516086401, -63.11908039286798555 ) ) ;
#28574=ORIENTED_EDGE ( 'NONE', *, *, #34734, .T. ) ;
#28575=CARTESIAN_POINT ( 'NONE',  ( 59.95259601283823514, 11.98300577492410390, 3.618069386873109305 ) ) ;
#28576=CARTESIAN_POINT ( 'NONE',  ( -58.76006735892197241, 15.70681061434692261, 58.13766844807554435 ) ) ;
#28583=CARTESIAN_POINT ( 'NONE',  ( -62.14837099232443762, 17.75045801599140205, -13.42952458767598856 ) ) ;
#28584=EDGE_CURVE ( 'NONE', #45708, #33533, #62107, .T. ) ;
#28585=CARTESIAN_POINT ( 'NONE',  ( 157.4703587214989398, -170.0000000000000000, 29.40946747225336466 ) ) ;
#28590=CARTESIAN_POINT ( 'NONE',  ( 43.14669449386823885, 9.942681284149136545, 70.77495916275495347 ) ) ;
#28591=CARTESIAN_POINT ( 'NONE',  ( 164.4760519199596160, 64.62478832434435105, 39.63968248660635396 ) ) ;
#28592=CARTESIAN_POINT ( 'NONE',  ( -155.7455325080991599, 71.01834415181984639, -64.98546709743690997 ) ) ;
#28593=CARTESIAN_POINT ( 'NONE',  ( 66.73431804020508196, 14.60294556126668475, 3.950658298317914596 ) ) ;
#28594=VECTOR ( 'NONE', #35053, 1000.000000000000000 ) ;
#28595=CARTESIAN_POINT ( 'NONE',  ( 86.62931800182292363, 19.42108912189597092, 44.71208757247933363 ) ) ;
#28600=CYLINDRICAL_SURFACE ( 'NONE', #5067, 7.500000000000013323 ) ;
#28602=CARTESIAN_POINT ( 'NONE',  ( -133.3923804760465543, 52.87100816290224969, -16.13643682761781761 ) ) ;
#28606=DIRECTION ( 'NONE',  ( -0.000000000000000000, 1.000000000000000000, -0.000000000000000000 ) ) ;
#28612=CARTESIAN_POINT ( 'NONE',  ( 175.5498284945444709, 74.57669191966279243, 4.876327785689846372 ) ) ;
#28614=CARTESIAN_POINT ( 'NONE',  ( 107.9301116202191793, 27.82606182274595241, -23.72815433879570790 ) ) ;
#28615=CARTESIAN_POINT ( 'NONE',  ( 141.0229350107040887, 45.92325889728665800, -95.00000000000133582 ) ) ;
#28616=CARTESIAN_POINT ( 'NONE',  ( -58.32502757340553501, 16.62877055630752920, -49.48199589557358280 ) ) ;
#28619=CARTESIAN_POINT ( 'NONE',  ( -14.19447842053094178, 7.389800932646232390, 41.58366191049604055 ) ) ;
#28625=CARTESIAN_POINT ( 'NONE',  ( -171.4943428135323131, 86.82484920477510570, 45.69172056196202192 ) ) ;
#28626=CARTESIAN_POINT ( 'NONE',  ( 117.6924004117966689, 33.61107268965020012, -17.59174222879768834 ) ) ;
#28627=CARTESIAN_POINT ( 'NONE',  ( -105.4556185321791304, 34.42302275449793569, 17.98560306758872329 ) ) ;
#28629=CARTESIAN_POINT ( 'NONE',  ( 136.9822423813093337, 44.53121110416873307, -23.50049531503082889 ) ) ;
#28630=ORIENTED_EDGE ( 'NONE', *, *, #39488, .T. ) ;
#28632=ORIENTED_EDGE ( 'NONE', *, *, #29785, .T. ) ;
#28635=CYLINDRICAL_SURFACE ( 'NONE', #3838, 7.500000000000013323 ) ;
#28640=CARTESIAN_POINT ( 'NONE',  ( -102.2801239173131052, 32.78103895658057354, -23.17002667451225406 ) ) ;
#28643=AXIS2_PLACEMENT_3D ( 'NONE', #49468, #37893, #26648 ) ;
#28645=CARTESIAN_POINT ( 'NONE',  ( 197.5344630110112121, 98.61758706718741507, -72.91483488310812788 ) ) ;
#28646=EDGE_CURVE ( 'NONE', #38367, #69371, #66379, .T. ) ;
#28652=FACE_BOUND ( 'NONE', #30350, .T. ) ;
#28655=B_SPLINE_CURVE_WITH_KNOTS ( 'NONE', 3,
 ( #43393, #64163, #32165, #57857, #36405, #15975, #64514, #69439, #53595, #16322, #42022, #5072, #63481, #36752, #5426, #52906, #4728, #26193, #58529, #47628, #69081, #20915, #42366, #15638, #37089, #31813, #53246, #26879, #42705, #137, #26540, #11041, #48303, #59221, #32503, #18073, #28260, #2247, #844, #12096, #50427, #54283, #66281, #12797 ),
 .UNSPECIFIED., .F., .F.,
 ( 4, 2, 2, 2, 2, 2, 2, 2, 2, 2, 2, 2, 2, 2, 2, 2, 2, 2, 2, 2, 2, 4 ),
 ( 0.000000000000000000, 0.001487235713946821964, 0.002230853570920213538, 0.002974471427893605763, 0.004461707141840350749, 0.005948942855787096168, 0.007436178569733841587, 0.008179796426707214296, 0.008923414283680587006, 0.01041064999762734804, 0.01189788571157410907, 0.01264150356854749566, 0.01338512142552088224, 0.01487235713946764674, 0.01561597499644103507, 0.01635959285341442512, 0.01784682856736120524, 0.01933406428130798535, 0.02007768213828137541, 0.02082129999525476199, 0.02230853570920153170, 0.02379577142314830140 ),
 .UNSPECIFIED. ) ;
#28659=CARTESIAN_POINT ( 'NONE',  ( -133.0808647576834005, 51.41195281028755915, -67.09815806457598342 ) ) ;
#28661=CARTESIAN_POINT ( 'NONE',  ( -125.8938041572051105, 46.49392987655495091, 72.46449846362081360 ) ) ;
#28664=DIRECTION ( 'NONE',  ( 0.000000000000000000, 0.000000000000000000, 1.000000000000000000 ) ) ;
#28665=CARTESIAN_POINT ( 'NONE',  ( 188.5164425382173192, 86.45836816134917058, 91.57835675204685799 ) ) ;
#28669=CARTESIAN_POINT ( 'NONE',  ( 173.5837434292113812, 71.34409607026158540, -44.01311006594448827 ) ) ;
#28670=CARTESIAN_POINT ( 'NONE',  ( -178.0633751203917825, 92.80295726428047942, -63.41043722487919609 ) ) ;
#28674=CARTESIAN_POINT ( 'NONE',  ( -180.3158531669106424, 95.51092859788509770, 9.337317216626621175 ) ) ;
#28675=CARTESIAN_POINT ( 'NONE',  ( -76.10397364431021572, 21.36211154336728768, -49.66815503544774657 ) ) ;
#28677=CARTESIAN_POINT ( 'NONE',  ( 79.66256042745894206, 17.16036700714778718, -94.20191509326981816 ) ) ;
#28679=CARTESIAN_POINT ( 'NONE',  ( -50.53243683205842984, 14.55237037207940887, -9.867349686703617451 ) ) ;
#28681=ORIENTED_EDGE ( 'NONE', *, *, #66338, .T. ) ;
#28682=CARTESIAN_POINT ( 'NONE',  ( -149.5074843970971017, 65.50121172469319220, 72.56537183036277838 ) ) ;
#28684=CARTESIAN_POINT ( 'NONE',  ( -71.15374617000810531, 20.66492714610677339, 11.08381322999615293 ) ) ;
#28687=CARTESIAN_POINT ( 'NONE',  ( -166.7136514167008841, 81.71618216218797670, -72.96353840939907798 ) ) ;
#28689=CARTESIAN_POINT ( 'NONE',  ( -133.2683599795575446, 51.54537714913664814, 90.40267370649584677 ) ) ;
#28691=CARTESIAN_POINT ( 'NONE',  ( 83.38067517854670996, 18.33799117207140483, -50.08583960832021376 ) ) ;
#28697=CARTESIAN_POINT ( 'NONE',  ( -129.6165111262477865, 48.99406349865703447, 31.60480352819717353 ) ) ;
#28701=CARTESIAN_POINT ( 'NONE',  ( 89.65730223173024172, 21.54473673261223610, 30.34629236393602625 ) ) ;
#28702=CARTESIAN_POINT ( 'NONE',  ( -121.5921196778231490, 43.72569502503144179, 58.80275198742250353 ) ) ;
#28704=CARTESIAN_POINT ( 'NONE',  ( -180.5200658187031877, 97.35517482626552521, -16.63434712722808229 ) ) ;
#28706=CARTESIAN_POINT ( 'NONE',  ( -53.14657859411973817, 15.21831473227210552, 45.07509434600507348 ) ) ;
#28707=EDGE_LOOP ( 'NONE', ( #61129, #56088 ) ) ;
#28711=CARTESIAN_POINT ( 'NONE',  ( 198.7029050523552201, 98.46895521196213963, -12.44553174149221064 ) ) ;
#28714=CARTESIAN_POINT ( 'NONE',  ( 212.0803491126037272, 118.9047894217573571, -42.46139465240390365 ) ) ;
#28717=DIRECTION ( 'NONE',  ( -0.000000000000000000, 1.000000000000000000, -0.000000000000000000 ) ) ;
#28722=CARTESIAN_POINT ( 'NONE',  ( -74.87059534020256990, 20.91186903862810098, 85.13133443590446348 ) ) ;
#28724=CARTESIAN_POINT ( 'NONE',  ( 129.1310456962234809, 39.80382822048402147, 31.16611068083063074 ) ) ;
#28727=CARTESIAN_POINT ( 'NONE',  ( -95.60805465865863084, 30.63099276904604906, -19.13322709836046442 ) ) ;
#28728=CARTESIAN_POINT ( 'NONE',  ( 60.61895554631703931, 13.15982272268127851, 44.43620800597218334 ) ) ;
#28731=ORIENTED_EDGE ( 'NONE', *, *, #63763, .T. ) ;
#28732=CARTESIAN_POINT ( 'NONE',  ( 55.57634120535664124, 12.09544293553730476, 65.14168292286281314 ) ) ;
#28734=CARTESIAN_POINT ( 'NONE',  ( -14.93280618462406473, 8.469244267267914239, 13.17839159822831441 ) ) ;
#28737=CARTESIAN_POINT ( 'NONE',  ( 132.2818448028687612, 41.65267246304674842, -24.01511195972667778 ) ) ;
#28738=EDGE_CURVE ( 'NONE', #47361, #14330, #31018, .T. ) ;
#28740=EDGE_LOOP ( 'NONE', ( #62684, #63912, #33441, #13187 ) ) ;
#28743=CARTESIAN_POINT ( 'NONE',  ( -34.52542994698664813, 11.14027065218092005, -35.97735163564012595 ) ) ;
#28744=CARTESIAN_POINT ( 'NONE',  ( -165.9121868482146454, 80.88751546905565704, -44.30229986177329238 ) ) ;
#28746=CYLINDRICAL_SURFACE ( 'NONE', #10799, 7.500000000000013323 ) ;
#28750=AXIS2_PLACEMENT_3D ( 'NONE', #31766, #53197, #5025 ) ;
#28754=CARTESIAN_POINT ( 'NONE',  ( -142.9728934044262019, 58.82891228489263113, -19.18790406048661268 ) ) ;
#28758=DIRECTION ( 'NONE',  ( -0.000000000000000000, 1.000000000000000000, -0.000000000000000000 ) ) ;
#28760=ORIENTED_EDGE ( 'NONE', *, *, #28646, .F. ) ;
#28762=CARTESIAN_POINT ( 'NONE',  ( 85.67165909753201447, 20.15791549876374944, 17.82174123723708448 ) ) ;
#28763=CARTESIAN_POINT ( 'NONE',  ( -96.43817545481741149, 31.02509717589736127, 33.28916959688606880 ) ) ;
#28765=CARTESIAN_POINT ( 'NONE',  ( -7.825402957745085430, 7.899365992529253866, -89.10717191287116634 ) ) ;
#28768=CARTESIAN_POINT ( 'NONE',  ( 55.90910788310613810, 11.13585330978400911, 39.76043137525509508 ) ) ;
#28771=CARTESIAN_POINT ( 'NONE',  ( -78.66644367742111399, 22.32174330031316956, -8.270900041254197532 ) ) ;
#28774=CARTESIAN_POINT ( 'NONE',  ( -9.524904342798460988, 8.016391612076533946, -77.07167657488317047 ) ) ;
#28777=CARTESIAN_POINT ( 'NONE',  ( -26.49928411671542960, 9.848831533840668229, 43.38111134601233942 ) ) ;
#28778=EDGE_CURVE ( 'NONE', #52011, #7422, #56170, .T. ) ;
#28782=CARTESIAN_POINT ( 'NONE',  ( 181.0840389613909736, 80.03940679743415387, -89.91415884680696990 ) ) ;
#28783=CARTESIAN_POINT ( 'NONE',  ( -33.84080342750782933, 9.997552308299118451, -23.09450778006452509 ) ) ;
#28784=CARTESIAN_POINT ( 'NONE',  ( 155.6786224008560851, 56.27084630678375277, -90.02132744223033001 ) ) ;
#28785=CARTESIAN_POINT ( 'NONE',  ( -125.8938041572051389, 47.69968343338778283, 3.775397282693376155 ) ) ;
#28786=CARTESIAN_POINT ( 'NONE',  ( 157.4703587214989113, 57.65129005721575339, 56.25401806271706562 ) ) ;
#28787=ORIENTED_EDGE ( 'NONE', *, *, #48676, .F. ) ;
#28788=ORIENTED_EDGE ( 'NONE', *, *, #8680, .T. ) ;
#28795=CARTESIAN_POINT ( 'NONE',  ( -38.93878980550034186, 10.94326053663842302, -42.32003742428015869 ) ) ;
#28796=CARTESIAN_POINT ( 'NONE',  ( -95.00979396555173651, 29.23841379431415888, 89.83681514907920018 ) ) ;
#28799=CARTESIAN_POINT ( 'NONE',  ( -133.3149301983942223, 51.57857650535018479, 66.08309739370045577 ) ) ;
#28800=CARTESIAN_POINT ( 'NONE',  ( -76.78104518372332166, 22.68568622761704034, -23.04560864541017295 ) ) ;
#28803=CARTESIAN_POINT ( 'NONE',  ( 81.03898448521317732, 17.58847173596442559, 59.03229392868342984 ) ) ;
#28805=CARTESIAN_POINT ( 'NONE',  ( 32.67604596315971577, 7.629767358313821468, 34.08620588322428091 ) ) ;
#28808=CARTESIAN_POINT ( 'NONE',  ( 188.0141161196704900, 85.90515114331880397, 39.69055676661305654 ) ) ;
#28811=CARTESIAN_POINT ( 'NONE',  ( -124.9970785861867739, 47.10847819093960709, 57.51488436916137914 ) ) ;
#28812=CARTESIAN_POINT ( 'NONE',  ( -9.524904342798462764, 8.016391612076533946, -50.22712598441950149 ) ) ;
#28820=CARTESIAN_POINT ( 'NONE',  ( -94.87734348028330089, 29.17663635873013561, -95.00000000000133582 ) ) ;
#28821=DIRECTION ( 'NONE',  ( -0.000000000000000000, 1.000000000000000000, -0.000000000000000000 ) ) ;
#28824=CARTESIAN_POINT ( 'NONE',  ( -11.14880195267006435, 7.129907723790826601, -63.02123272090544503 ) ) ;
#28825=CARTESIAN_POINT ( 'NONE',  ( -33.36721086971961370, 9.915747831546605440, 44.96849820624647265 ) ) ;
#28826=CARTESIAN_POINT ( 'NONE',  ( 141.3707934840545022, 46.15056991286791543, -43.55297844023782261 ) ) ;
#28831=CARTESIAN_POINT ( 'NONE',  ( 32.66364305947234925, 8.639871491745255483, -12.94525474216406735 ) ) ;
#28833=LINE ( 'NONE', #7728, #20633 ) ;
#28834=CARTESIAN_POINT ( 'NONE',  ( -4.731197926646205865, 7.716745361328041675, 57.62373423735959221 ) ) ;
#28837=CARTESIAN_POINT ( 'NONE',  ( 197.8055825329258823, 98.95774805991030121, -94.51229222371586047 ) ) ;
#28838=SURFACE_STYLE_FILL_AREA ( #7384 ) ;
#28843=CARTESIAN_POINT ( 'NONE',  ( 162.1014732644455307, 61.34312237409764634, -10.86097702891884076 ) ) ;
#28847=CARTESIAN_POINT ( 'NONE',  ( 140.9169160367233360, 45.85398962664667977, -67.78391568571109360 ) ) ;
#28852=CARTESIAN_POINT ( 'NONE',  ( -118.9668643994983483, 43.27909474462862960, 67.85177516854167834 ) ) ;
#28853=CARTESIAN_POINT ( 'NONE',  ( 164.8444104055694481, 64.93678790243654930, -18.17606153825600757 ) ) ;
#28854=CARTESIAN_POINT ( 'NONE',  ( 8.528421445032394743, 6.376778749352037146, 35.56919029742448402 ) ) ;
#28857=CARTESIAN_POINT ( 'NONE',  ( 65.39792658623288446, 14.27332852928127949, 71.27325231829686913 ) ) ;
#28860=CARTESIAN_POINT ( 'NONE',  ( 163.5944442552009548, 63.88381951184481267, -39.28731366255506430 ) ) ;
#28861=CARTESIAN_POINT ( 'NONE',  ( 88.53517449242357884, 20.08005703101045469, 17.62531166502685309 ) ) ;
#28863=CARTESIAN_POINT ( 'NONE',  ( 163.7464701930789772, 62.69993100427429056, -47.76119388460286075 ) ) ;
#28866=CARTESIAN_POINT ( 'NONE',  ( -95.04371414958063724, 30.36527049547256851, 9.135576169247952905 ) ) ;
#28868=CARTESIAN_POINT ( 'NONE',  ( 33.77444274891860942, 8.756048688386680823, 32.44976720788645252 ) ) ;
#28869=CARTESIAN_POINT ( 'NONE',  ( -180.6021503146988607, 97.45669259943413465, -41.59167162592825662 ) ) ;
#28870=CARTESIAN_POINT ( 'NONE',  ( -132.6161619568759988, 51.08240647571221871, -18.90511423407786040 ) ) ;
#28871=CARTESIAN_POINT ( 'NONE',  ( -146.7427626416307476, 61.86902255109500004, -89.01813897100886663 ) ) ;
#28872=CARTESIAN_POINT ( 'NONE',  ( 126.8237978310704221, 37.33705012421152247, -67.74913777150965188 ) ) ;
#28875=CARTESIAN_POINT ( 'NONE',  ( 134.3135005523731706, 42.87884033955813123, -77.85745800642466463 ) ) ;
#28876=CARTESIAN_POINT ( 'NONE',  ( -10.69547592951790982, 8.103864096836389308, 57.51816172537316163 ) ) ;
#28878=CARTESIAN_POINT ( 'NONE',  ( -156.1477286774994582, 71.38742644140637594, -38.81583713021509396 ) ) ;
#28880=CARTESIAN_POINT ( 'NONE',  ( -36.37229078872272936, 11.47648211215765990, 32.04620998045675151 ) ) ;
#28882=CARTESIAN_POINT ( 'NONE',  ( -3.255961059272217906, 7.643453059677443484, 43.58302407791597943 ) ) ;
#28885=CARTESIAN_POINT ( 'NONE',  ( 207.8484262634767674, 110.7633525054914401, -50.64494125179354711 ) ) ;
#28886=CARTESIAN_POINT ( 'NONE',  ( -15.07235766390729026, 8.482541916553470784, 35.66812363169304945 ) ) ;
#28887=CARTESIAN_POINT ( 'NONE',  ( 164.9697211531229470, 63.72502658717164792, 9.768110188899187918 ) ) ;
#28889=VERTEX_POINT ( 'NONE', #29938 ) ;
#28891=CARTESIAN_POINT ( 'NONE',  ( -96.43817545481742570, 31.02509717589737193, -47.24448217450499499 ) ) ;
#28894=CARTESIAN_POINT ( 'NONE',  ( 45.76553115525425142, 10.34124506813254740, -20.25205682851913025 ) ) ;
#28895=VECTOR ( 'NONE', #31930, 1000.000000000000000 ) ;
#28904=CARTESIAN_POINT ( 'NONE',  ( -118.4470345550925998, 42.96051736048244862, -16.61147982237926968 ) ) ;
#28908=CYLINDRICAL_SURFACE ( 'NONE', #54518, 7.500000000000013323 ) ;
#28911=CARTESIAN_POINT ( 'NONE',  ( 107.9213359589208636, 28.92595015506873679, 71.10305713611002432 ) ) ;
#28913=DIRECTION ( 'NONE',  ( 0.000000000000000000, 0.000000000000000000, 1.000000000000000000 ) ) ;
#28915=ORIENTED_EDGE ( 'NONE', *, *, #19860, .F. ) ;
#28918=CARTESIAN_POINT ( 'NONE',  ( -82.53770812813171176, 23.83403279300013722, -22.19906966960727246 ) ) ;
#28921=FACE_BOUND ( 'NONE', #44189, .T. ) ;
#28922=ADVANCED_FACE ( 'NONE', ( #57363 ), #67931, .F. ) ;
#28928=CARTESIAN_POINT ( 'NONE',  ( 32.15284246740100116, 8.588257691344875155, -68.02502300723051576 ) ) ;
#28929=CARTESIAN_POINT ( 'NONE',  ( -177.1381400275771796, 93.26609858452820845, 5.128634852069275496 ) ) ;
#28930=CARTESIAN_POINT ( 'NONE',  ( 152.2940756559019064, 53.73566983921583073, 4.632148972456340275 ) ) ;
#28932=VECTOR ( 'NONE', #14803, 1000.000000000000000 ) ;
#28935=CARTESIAN_POINT ( 'NONE',  ( 197.3119541548905715, 98.33923235143190311, -45.14000074610142832 ) ) ;
#28942=CARTESIAN_POINT ( 'NONE',  ( 91.12448333640237763, 22.07449368110502164, -76.18914264227882427 ) ) ;
#28944=CIRCLE ( 'NONE', #40137, 243.4957430088094839 ) ;
#28945=VERTEX_POINT ( 'NONE', #9175 ) ;
#28947=CARTESIAN_POINT ( 'NONE',  ( 163.7379901688713346, 64.00402364591249693, 41.03665140154781454 ) ) ;
#28948=VECTOR ( 'NONE', #35257, 1000.000000000000000 ) ;
#28949=CARTESIAN_POINT ( 'NONE',  ( -156.3734885497382265, 71.59531449004289527, -72.18732252565617102 ) ) ;
#28950=CARTESIAN_POINT ( 'NONE',  ( 70.51522979775971578, 15.57935281015687146, 10.97061778370436436 ) ) ;
#28957=CARTESIAN_POINT ( 'NONE',  ( -53.38065169970960966, 15.27943072477081721, 18.28795179123243742 ) ) ;
#28958=CARTESIAN_POINT ( 'NONE',  ( -11.85813018568104305, 8.195977661838494299, -90.22625169180082594 ) ) ;
#28959=CARTESIAN_POINT ( 'NONE',  ( -155.2449610530290158, 70.56131896221211264, -91.16623920745314535 ) ) ;
#28961=CARTESIAN_POINT ( 'NONE',  ( 79.79041068698137451, 17.19981260293680236, 87.80323115344171470 ) ) ;
#28966=CARTESIAN_POINT ( 'NONE',  ( 40.37438610703016906, 8.537526699166109623, 3.116409814543585455 ) ) ;
#28967=CARTESIAN_POINT ( 'NONE',  ( -179.6930825076241831, 96.33844031696564514, 88.38185184032300867 ) ) ;
#28969=CARTESIAN_POINT ( 'NONE',  ( 103.4696172145935122, 25.87254488218943749, -13.34745220050455750 ) ) ;
#28970=CARTESIAN_POINT ( 'NONE',  ( 200.8298320869469933, 101.1869877914233484, 3.423144167023327356 ) ) ;
#28971=CARTESIAN_POINT ( 'NONE',  ( 208.2960261509592215, 113.1866506096883143, 83.81060036596683460 ) ) ;
#28973=CARTESIAN_POINT ( 'NONE',  ( -71.97434903038468690, 19.88430675376532974, -72.88272746850553574 ) ) ;
#28974=CARTESIAN_POINT ( 'NONE',  ( -11.57931195747592312, 7.164335452024272577, 44.12695385317129393 ) ) ;
#28976=CARTESIAN_POINT ( 'NONE',  ( 13.83281508467571363, 7.452090093180184560, -8.916925143331820180 ) ) ;
#28978=ORIENTED_EDGE ( 'NONE', *, *, #55726, .T. ) ;
#28979=CARTESIAN_POINT ( 'NONE',  ( -145.9181947914994737, 62.49417193455356312, 17.96563906742083461 ) ) ;
#28980=B_SPLINE_CURVE_WITH_KNOTS ( 'NONE', 3,
 ( #53478, #31360, #20, #68967, #25746, #5309, #37305, #47175, #41563, #52462, #47866, #4284, #63715, #68635, #26768, #4614, #69328, #20441, #48194, #15527, #26079, #47509, #10919, #36641, #36980, #58416, #21475, #16202, #10232, #31695, #21151, #42596, #64048, #15859, #64390, #37654, #32396, #53820, #27442, #11974, #60508, #43966, #22178, #48881, #7041, #12673 ),
 .UNSPECIFIED., .F., .F.,
 ( 4, 2, 2, 2, 2, 2, 2, 2, 2, 2, 2, 2, 2, 2, 2, 2, 2, 2, 2, 2, 2, 2, 4 ),
 ( 6.938893903907228378E-18, 0.003192770216278345216, 0.003990962770347930219, 0.004789155324417515222, 0.006385540432556695636, 0.007183732986626276303, 0.007981925540695855234, 0.009578310648835018301, 0.01037650320290461024, 0.01117469575697420045, 0.01197288831104379239, 0.01277108086511338433, 0.01436746597325256822, 0.01596385108139174863, 0.01676204363546133017, 0.01756023618953090823, 0.01835842874360048629, 0.01915662129767006783, 0.02075300640580923089, 0.02234939151394839396, 0.02394577662208755703, 0.02474396917615713856, 0.02554216173022672356 ),
 .UNSPECIFIED. ) ;
#28982=CARTESIAN_POINT ( 'NONE',  ( -166.2065256787326746, 81.19093426984592554, 41.24070342831011260 ) ) ;
#28983=CARTESIAN_POINT ( 'NONE',  ( 117.4806398654733641, 33.50379325299402922, -18.61210399727144704 ) ) ;
#28986=CARTESIAN_POINT ( 'NONE',  ( -108.9452487746634404, 36.29752968355631992, 7.697822667569220734 ) ) ;
#28987=CARTESIAN_POINT ( 'NONE',  ( 39.40195752203892710, -170.0000000000000000, 10.56928371549958889 ) ) ;
#28988=CARTESIAN_POINT ( 'NONE',  ( 141.0517870458593279, 47.14452711594498169, -14.54592510178403586 ) ) ;
#28998=CARTESIAN_POINT ( 'NONE',  ( -156.3413281584584809, 70.19975255048969132, 94.99999999999866418 ) ) ;
#29001=ADVANCED_FACE ( 'NONE', ( #20760 ), #64352, .T. ) ;
#29002=CARTESIAN_POINT ( 'NONE',  ( 198.2581645178919132, 99.52881771501675701, 67.40755752364371745 ) ) ;
#29004=AXIS2_PLACEMENT_3D ( 'NONE', #48371, #58948, #8448 ) ;
#29005=LINE ( 'NONE', #43500, #49087 ) ;
#29006=CARTESIAN_POINT ( 'NONE',  ( -58.32502757340554922, 16.62877055630752920, -76.32654648603724468 ) ) ;
#29007=CARTESIAN_POINT ( 'NONE',  ( 177.0024338932394130, 74.57605685449962607, -64.26120218828934583 ) ) ;
#29010=CARTESIAN_POINT ( 'NONE',  ( -172.3057147739576749, 86.22480007276992353, 4.010060984321524913 ) ) ;
#29012=FACE_BOUND ( 'NONE', #34054, .T. ) ;
#29013=CARTESIAN_POINT ( 'NONE',  ( -189.6935402730020428, 107.7189398452714926, 94.71296932948054348 ) ) ;
#29014=VECTOR ( 'NONE', #26462, 1000.000000000000000 ) ;
#29016=CARTESIAN_POINT ( 'NONE',  ( -2.866724795119716340, 6.618578306599220973, 70.10825721528765087 ) ) ;
#29020=CARTESIAN_POINT ( 'NONE',  ( 149.9683128897949871, 53.28564708287390772, 64.28427443997613011 ) ) ;
#29026=CARTESIAN_POINT ( 'NONE',  ( 187.2889560709053853, 85.11232376512226949, 94.72469196122591484 ) ) ;
#29030=CARTESIAN_POINT ( 'NONE',  ( 152.8373718734504507, 55.38925997611396923, 42.82746393499770932 ) ) ;
#29034=B_SPLINE_CURVE_WITH_KNOTS ( 'NONE', 3,
 ( #41321, #63809, #26516, #63117, #25153, #41659, #36736, #36040, #46581, #62776, #58180, #31793, #21238, #53227, #68062, #4712, #52554, #14916, #9655, #20535, #5053, #52212, #31118, #15958, #10328, #47956, #31452, #14580, #4377, #69422, #15617, #25840, #36387, #20894, #19865, #68724, #57839, #47272, #57496, #42685, #42350, #9999, #9302, #42004, #64144, #63464, #68398, #15274, #20203, #52886 ),
 .UNSPECIFIED., .F., .F.,
 ( 4, 2, 2, 2, 2, 2, 2, 2, 2, 2, 2, 2, 2, 2, 2, 2, 2, 2, 2, 2, 2, 2, 2, 2, 4 ),
 ( 0.03296461860586802350, 0.03492857779726595696, 0.03689253698866389042, 0.03885649618006182388, 0.04082045537145975733, 0.04278441456285769079, 0.04376639415855662629, 0.04474837375425555486, 0.04573035334995449036, 0.04671233294565341893, 0.04720332274350288321, 0.04769431254135235443, 0.04867629213705128299, 0.04965827173275021156, 0.05064025132844914706, 0.05162223092414808256, 0.05260421051984701113, 0.05358619011554593969, 0.05456816971124487520, 0.05555014930694381070, 0.05653212890264273927, 0.05849608809404058252, 0.06046004728543843271, 0.06242400647683628290, 0.06438796566823412615 ),
 .UNSPECIFIED. ) ;
#29038=CARTESIAN_POINT ( 'NONE',  ( -26.49928411671542960, 9.848831533840670005, -10.30798983491501808 ) ) ;
#29039=CARTESIAN_POINT ( 'NONE',  ( -54.08816720029309977, 15.46531105893041769, -8.418552427708386077 ) ) ;
#29042=CARTESIAN_POINT ( 'NONE',  ( 117.4696399285658543, 32.37118663718647582, -45.49517373264203002 ) ) ;
#29044=CARTESIAN_POINT ( 'NONE',  ( 45.36109889487609337, 9.259412558041161034, -38.53950509509405720 ) ) ;
#29046=LINE ( 'NONE', #18134, #18558 ) ;
#29047=LINE ( 'NONE', #17791, #33221 ) ;
#29052=CARTESIAN_POINT ( 'NONE',  ( -142.3178993725749137, 58.31327888234797996, 67.27388540028242403 ) ) ;
#29053=CARTESIAN_POINT ( 'NONE',  ( 81.05403189674299824, 18.64820877954959499, 32.17181610260639246 ) ) ;
#29057=CARTESIAN_POINT ( 'NONE',  ( 43.96421756700842565, 10.06386361114660311, 4.596548279175047824 ) ) ;
#29058=CARTESIAN_POINT ( 'NONE',  ( -179.5109681715917986, 96.11572638569518290, -19.33240666069409031 ) ) ;
#29060=VERTEX_POINT ( 'NONE', #48160 ) ;
#29062=CARTESIAN_POINT ( 'NONE',  ( 109.7774723066848850, 28.66666416591279898, 56.45576479620101651 ) ) ;
#29063=CARTESIAN_POINT ( 'NONE',  ( 159.6593397521789370, 59.37286298965125297, 56.56669563789166233 ) ) ;
#29064=CARTESIAN_POINT ( 'NONE',  ( -190.6985136298601731, 109.1272424661242582, 60.81597207375692449 ) ) ;
#29067=CARTESIAN_POINT ( 'NONE',  ( -108.6634958860518338, 36.14357436892402831, 68.80899113430457703 ) ) ;
#29068=CARTESIAN_POINT ( 'NONE',  ( -26.88245755577923646, 8.887394979218518287, -48.79474396477220210 ) ) ;
#29075=CARTESIAN_POINT ( 'NONE',  ( -76.27009788956611658, 21.42253842560091570, 84.47334644398770820 ) ) ;
#29076=CARTESIAN_POINT ( 'NONE',  ( 15.78827728214693416, -170.0000000000000000, 45.01470767270524931 ) ) ;
#29077=CARTESIAN_POINT ( 'NONE',  ( 132.0563630623056781, 41.51825634609595994, 29.72595898648637203 ) ) ;
#29082=CARTESIAN_POINT ( 'NONE',  ( 56.29445224195348629, 12.24017809212661945, 33.94850966223434341 ) ) ;
#29083=CARTESIAN_POINT ( 'NONE',  ( 32.71243998906020778, 7.633449976421425198, 87.69550224701529828 ) ) ;
#29084=VERTEX_POINT ( 'NONE', #37268 ) ;
#29085=CARTESIAN_POINT ( 'NONE',  ( -3.252497086158845363, 6.636017118947991733, -48.88317998446056833 ) ) ;
#29087=CARTESIAN_POINT ( 'NONE',  ( -189.2739965869454295, 107.1373753350176230, -42.99051981391919242 ) ) ;
#29088=CARTESIAN_POINT ( 'NONE',  ( -142.9730935922300148, 58.82921737386683247, 15.06684688205722544 ) ) ;
#29090=CARTESIAN_POINT ( 'NONE',  ( -104.1342612728951167, 33.73231160250194449, -76.64130442548571409 ) ) ;
#29091=CARTESIAN_POINT ( 'NONE',  ( 130.7260570116704059, 40.73146260246710426, -9.847617054034046191 ) ) ;
#29097=CARTESIAN_POINT ( 'NONE',  ( -36.89224332184166855, 11.57404295377975778, -47.97205884790524522 ) ) ;
#29099=CARTESIAN_POINT ( 'NONE',  ( -165.7184136928310920, 79.24930266387268318, 93.27236818605236124 ) ) ;
#29100=EDGE_LOOP ( 'NONE', ( #36549, #35891 ) ) ;
#29101=CARTESIAN_POINT ( 'NONE',  ( -118.3927673406137302, 41.74929850983304647, -42.17578386237221366 ) ) ;
#29104=CARTESIAN_POINT ( 'NONE',  ( 154.3232427916091751, 56.50492108618855980, 83.78354423499102666 ) ) ;
#29106=DIRECTION ( 'NONE',  ( -0.000000000000000000, 1.000000000000000000, -0.000000000000000000 ) ) ;
#29109=CARTESIAN_POINT ( 'NONE',  ( 19.74724861314307134, 6.659670522263898107, -49.39369726644508063 ) ) ;
#29111=ORIENTED_EDGE ( 'NONE', *, *, #35186, .F. ) ;
#29112=CARTESIAN_POINT ( 'NONE',  ( 59.72897338775216980, 11.93428797217974591, 30.56701851669645009 ) ) ;
#29113=ORIENTED_EDGE ( 'NONE', *, *, #60991, .T. ) ;
#29115=CARTESIAN_POINT ( 'NONE',  ( 174.9099402067542428, 73.96774984027642574, 41.07482263567545999 ) ) ;
#29116=CARTESIAN_POINT ( 'NONE',  ( 15.78827728214693416, 6.500811158483284835, -77.36349468914950478 ) ) ;
#29117=DIRECTION ( 'NONE',  ( -0.000000000000000000, 1.000000000000000000, -0.000000000000000000 ) ) ;
#29118=EDGE_LOOP ( 'NONE', ( #64620, #31725 ) ) ;
#29120=CARTESIAN_POINT ( 'NONE',  ( -25.49247221749738301, 9.706368398275719400, 42.31336193027286185 ) ) ;
#29121=CARTESIAN_POINT ( 'NONE',  ( -71.27103490383372275, 20.70545763375144688, -41.34176840752093796 ) ) ;
#29123=EDGE_CURVE ( 'NONE', #14016, #61067, #37721, .T. ) ;
#29124=CARTESIAN_POINT ( 'NONE',  ( 212.1669304543882220, 119.0398299474538959, -71.37118650051857571 ) ) ;
#29126=DIRECTION ( 'NONE',  ( -0.8160245890732938934, -0.5780171883497599028, 0.000000000000000000 ) ) ;
#29127=CARTESIAN_POINT ( 'NONE',  ( 115.0485321076020284, 32.28990710985444679, 42.89032573288258732 ) ) ;
#29128=CARTESIAN_POINT ( 'NONE',  ( -128.3448054685827913, 49.34430406923178225, 4.183529080979890402 ) ) ;
#29133=EDGE_LOOP ( 'NONE', ( #11988, #4288 ) ) ;
#29136=CARTESIAN_POINT ( 'NONE',  ( -38.84150381976580491, 10.92416363971239157, -44.04817657352107574 ) ) ;
#29137=LINE ( 'NONE', #50588, #10156 ) ;
#29145=ORIENTED_EDGE ( 'NONE', *, *, #7319, .F. ) ;
#29146=CARTESIAN_POINT ( 'NONE',  ( 33.75639351246965703, 7.742023566824295600, 32.45167201372024124 ) ) ;
#29151=CARTESIAN_POINT ( 'NONE',  ( -121.5680658099884255, 44.89994870382102476, 58.81937421782851771 ) ) ;
#29152=CARTESIAN_POINT ( 'NONE',  ( -48.33725449172840172, 12.98311179783360103, 7.596865058600053899 ) ) ;
#29157=CARTESIAN_POINT ( 'NONE',  ( -106.2973690786608501, 34.86887399500433560, -89.86655251325186100 ) ) ;
#29158=CARTESIAN_POINT ( 'NONE',  ( -156.6819053601226130, 70.51177710383655040, -13.20956540371496324 ) ) ;
#29161=CARTESIAN_POINT ( 'NONE',  ( -56.96436614829621448, 16.24647150911282623, 57.40554593459077637 ) ) ;
#29164=B_SPLINE_CURVE_WITH_KNOTS ( 'NONE', 3,
 ( #16592, #59836, #12018, #16932, #769, #6391, #37696, #16245, #38048, #59148, #22221, #33131, #7086, #27844, #48574, #33489, #54564, #17282, #43659, #32434, #53862, #49634 ),
 .UNSPECIFIED., .F., .F.,
 ( 4, 2, 2, 2, 2, 2, 2, 2, 2, 2, 4 ),
 ( 0.01086728410803540143, 0.01221890224361778243, 0.01357052037920016344, 0.01492213851478254444, 0.01559794758257374188, 0.01627375665036493932, 0.01762537478594729951, 0.01830118385373846399, 0.01897699292152962847, 0.02032861105711193661, 0.02168022919269424129 ),
 .UNSPECIFIED. ) ;
#29166=CARTESIAN_POINT ( 'NONE',  ( 150.9013375937531123, 53.96275732797609237, -66.84018692432205455 ) ) ;
#29167=CARTESIAN_POINT ( 'NONE',  ( -32.41627406084104734, 9.753381371531508748, 45.16836582512236475 ) ) ;
#29168=CARTESIAN_POINT ( 'NONE',  ( 133.8566784816069060, 41.42467568809810530, -51.02331093239568816 ) ) ;
#29169=EDGE_CURVE ( 'NONE', #44045, #4538, #9204, .T. ) ;
#29174=EDGE_CURVE ( 'NONE', #25573, #16185, #25168, .T. ) ;
#29175=CARTESIAN_POINT ( 'NONE',  ( -125.8938041572051389, 46.49392987655492249, 30.61994787315706290 ) ) ;
#29177=CARTESIAN_POINT ( 'NONE',  ( 36.08914434112043779, 9.014684630517859176, -9.542106359090377410 ) ) ;
#29180=CARTESIAN_POINT ( 'NONE',  ( 127.2459819677542754, 38.72844404003734553, 87.15258772988752867 ) ) ;
#29183=PRESENTATION_STYLE_ASSIGNMENT (( #38688 ) ) ;
#29185=AXIS2_PLACEMENT_3D ( 'NONE', #15955, #69420, #58857 ) ;
#29186=ORIENTED_EDGE ( 'NONE', *, *, #23199, .T. ) ;
#29189=CARTESIAN_POINT ( 'NONE',  ( 69.50572373348801136, 14.27208627753791603, 67.94843943493852123 ) ) ;
#29190=CARTESIAN_POINT ( 'NONE',  ( 133.8566784816069628, 41.42467568809806977, -62.86786152285933582 ) ) ;
#29194=CARTESIAN_POINT ( 'NONE',  ( 163.5944155533006210, 63.88379440759436534, -21.11661691084674075 ) ) ;
#29195=CARTESIAN_POINT ( 'NONE',  ( 8.848532525911927848, 6.377649276597440853, 40.39023764036181063 ) ) ;
#29196=EDGE_LOOP ( 'NONE', ( #60422, #32561 ) ) ;
#29197=CARTESIAN_POINT ( 'NONE',  ( 69.48877314113910586, 15.30784187978995092, 67.95358286125032521 ) ) ;
#29200=CARTESIAN_POINT ( 'NONE',  ( -145.3109762780891003, 60.69959559383372749, -62.92412485375768938 ) ) ;
#29204=CARTESIAN_POINT ( 'NONE',  ( 164.4615316623335275, 63.29763980349835606, -46.35316271778197006 ) ) ;
#29205=ORIENTED_EDGE ( 'NONE', *, *, #41286, .T. ) ;
#29207=LINE ( 'NONE', #13716, #49192 ) ;
#29208=EDGE_CURVE ( 'NONE', #3067, #41030, #66294, .T. ) ;
#29209=CARTESIAN_POINT ( 'NONE',  ( 33.44035656425388225, 8.720466003183672044, 41.99093887284341520 ) ) ;
#29210=CARTESIAN_POINT ( 'NONE',  ( 79.37778929114109872, 18.12554302172299714, -14.49807325564501603 ) ) ;
#29211=CARTESIAN_POINT ( 'NONE',  ( -133.3765738414514601, 51.62252165471731047, -14.99249644436331685 ) ) ;
#29213=CARTESIAN_POINT ( 'NONE',  ( 132.0440382699655117, 40.34028297386452522, -77.65984809815648759 ) ) ;
#29214=ORIENTED_EDGE ( 'NONE', *, *, #41374, .T. ) ;
#29216=CARTESIAN_POINT ( 'NONE',  ( -13.29455179262032871, 8.319166883236675858, 59.32222173321054726 ) ) ;
#29217=ORIENTED_EDGE ( 'NONE', *, *, #15426, .T. ) ;
#29219=CARTESIAN_POINT ( 'NONE',  ( -151.6648563624119390, 67.36546864992760675, -49.50942221783397201 ) ) ;
#29221=CARTESIAN_POINT ( 'NONE',  ( -38.92718193365330848, 11.96647478777219753, 38.20581357431434810 ) ) ;
#29222=CARTESIAN_POINT ( 'NONE',  ( -0.7211439451572428938, 7.539282923622931065, 40.03214358363065628 ) ) ;
#29226=CARTESIAN_POINT ( 'NONE',  ( -1.862553927312057267, 7.582910205528083480, -20.64884027158456803 ) ) ;
#29228=CARTESIAN_POINT ( 'NONE',  ( -14.33576511807125620, 8.413127487936188587, 41.37126689364819043 ) ) ;
#29229=CARTESIAN_POINT ( 'NONE',  ( -60.65612136648953623, 16.25551606627059087, 15.98195799223179492 ) ) ;
#29233=ORIENTED_EDGE ( 'NONE', *, *, #22243, .T. ) ;
#29234=CARTESIAN_POINT ( 'NONE',  ( 103.5588133492865239, 25.91050225236393345, -73.70627781999075978 ) ) ;
#29237=CARTESIAN_POINT ( 'NONE',  ( 46.65037935242576594, 9.463293687292228640, 66.20036211219351685 ) ) ;
#29238=CARTESIAN_POINT ( 'NONE',  ( 8.000000000000007105, 249.8719672152120381, 94.99999999999866418 ) ) ;
#29239=CYLINDRICAL_SURFACE ( 'NONE', #59179, 7.500000000000027534 ) ;
#29242=CARTESIAN_POINT ( 'NONE',  ( 39.40195752203892710, 8.409560354027384221, 44.91383430596327742 ) ) ;
#29249=CARTESIAN_POINT ( 'NONE',  ( 109.7782172510783170, 29.77507867835874933, 56.45576479620099519 ) ) ;
#29252=CARTESIAN_POINT ( 'NONE',  ( 60.61895554631703220, 13.15982272268128206, -9.252893174955183042 ) ) ;
#29256=CARTESIAN_POINT ( 'NONE',  ( 103.5849290181278803, 27.01613348792541913, -46.88419179696489891 ) ) ;
#29258=CARTESIAN_POINT ( 'NONE',  ( -81.01337222286375095, 23.22902179892321683, -22.91030771783860587 ) ) ;
#29260=CARTESIAN_POINT ( 'NONE',  ( 212.1931396682533375, 117.2245435827729239, -16.66766266149112496 ) ) ;
#29261=FACE_BOUND ( 'NONE', #21411, .T. ) ;
#29265=CARTESIAN_POINT ( 'NONE',  ( 89.65730223173021329, 21.54473673261222899, -50.18735940745502688 ) ) ;
#29266=CARTESIAN_POINT ( 'NONE',  ( 31.95163392065795449, 8.568192436298444292, -70.95598465355915607 ) ) ;
#29268=CARTESIAN_POINT ( 'NONE',  ( 212.1978255065450867, 119.0880569674902603, 63.90116129329218353 ) ) ;
#29270=DIRECTION ( 'NONE',  ( -0.000000000000000000, 1.000000000000000000, -0.000000000000000000 ) ) ;
#29273=CARTESIAN_POINT ( 'NONE',  ( 199.2049631873262001, 100.7347227143599753, -38.71285982394856262 ) ) ;
#29274=VERTEX_POINT ( 'NONE', #21031 ) ;
#29278=CARTESIAN_POINT ( 'NONE',  ( -58.32502757340554211, 16.62877055630752210, -22.63744530510987119 ) ) ;
#29281=ORIENTED_EDGE ( 'NONE', *, *, #49778, .F. ) ;
#29282=CARTESIAN_POINT ( 'NONE',  ( 41.34269507549200995, 9.685203600174697058, 56.99739923425319432 ) ) ;
#29283=CARTESIAN_POINT ( 'NONE',  ( -104.3632071119006923, 34.98619430863521984, -88.98640296607699440 ) ) ;
#29284=CARTESIAN_POINT ( 'NONE',  ( 103.0124792097646491, 26.77148435100179569, 8.208214002704151468 ) ) ;
#29288=CARTESIAN_POINT ( 'NONE',  ( -53.14657859411974528, 15.21831473227210552, 18.23054375554142581 ) ) ;
#29289=CARTESIAN_POINT ( 'NONE',  ( -127.6881387055492354, 48.89937523111243678, -22.85493024525475647 ) ) ;
#29291=FACE_OUTER_BOUND ( 'NONE', #53078, .T. ) ;
#29294=ORIENTED_EDGE ( 'NONE', *, *, #12997, .T. ) ;
#29295=AXIS2_PLACEMENT_3D ( 'NONE', #7871, #29321, #51477 ) ;
#29297=CARTESIAN_POINT ( 'NONE',  ( 41.09671232177014844, 8.635892912882344064, 3.259150826632041476 ) ) ;
#29299=CARTESIAN_POINT ( 'NONE',  ( -179.9997297618090784, 96.71425526203211120, 94.99999999999866418 ) ) ;
#29300=CARTESIAN_POINT ( 'NONE',  ( -48.33725449172838751, 12.98311179783359037, -19.24768553186362041 ) ) ;
#29301=CARTESIAN_POINT ( 'NONE',  ( 102.8518012651273921, 25.61025413220826863, -15.27953052830500091 ) ) ;
#29302=CARTESIAN_POINT ( 'NONE',  ( 200.4559562755962077, 100.7034888016685557, 3.660617377573986087 ) ) ;
#29304=CARTESIAN_POINT ( 'NONE',  ( 212.1648021685800245, 119.0365075864307300, 89.65931539195061362 ) ) ;
#29306=LINE ( 'NONE', #55333, #55712 ) ;
#29307=CARTESIAN_POINT ( 'NONE',  ( -85.35172689181706573, 26.07142112926219113, 61.32667841685976384 ) ) ;
#29308=CARTESIAN_POINT ( 'NONE',  ( -15.31363169557738502, 7.494880774891997888, 37.12813078065121175 ) ) ;
#29310=CARTESIAN_POINT ( 'NONE',  ( 11.81843724556921416, 7.412394300769733491, -9.806428785726447828 ) ) ;
#29311=ORIENTED_EDGE ( 'NONE', *, *, #56681, .F. ) ;
#29317=CARTESIAN_POINT ( 'NONE',  ( -173.1211646369891355, 88.63826465341152527, 45.82169460664104577 ) ) ;
#29319=CARTESIAN_POINT ( 'NONE',  ( -99.97541017369790950, 31.62502926470688180, -35.36197685046671779 ) ) ;
#29321=DIRECTION ( 'NONE',  ( -0.000000000000000000, 1.000000000000000000, -0.000000000000000000 ) ) ;
#29323=CARTESIAN_POINT ( 'NONE',  ( 129.1381264900934696, 38.64720302602604107, -37.67339026062629870 ) ) ;
#29325=ORIENTED_EDGE ( 'NONE', *, *, #27692, .F. ) ;
#29326=CARTESIAN_POINT ( 'NONE',  ( 188.0287290159266433, 87.41935856271966543, 87.65909336768878291 ) ) ;
#29329=CARTESIAN_POINT ( 'NONE',  ( 63.01563776193091826, 12.67277567978500308, -23.87614024170608218 ) ) ;
#29330=CARTESIAN_POINT ( 'NONE',  ( -51.78153763344963778, 13.82841714689604196, 31.05108900895189805 ) ) ;
#29331=CARTESIAN_POINT ( 'NONE',  ( 197.8588046850313731, 99.02485934465610740, 66.64561215349371537 ) ) ;
#29333=FACE_OUTER_BOUND ( 'NONE', #23693, .T. ) ;
#29334=CARTESIAN_POINT ( 'NONE',  ( -56.97556689808916985, 16.24958672959845885, -62.30750940606130683 ) ) ;
#29335=CARTESIAN_POINT ( 'NONE',  ( 197.1975259970231491, 98.19639476549652102, -70.34394312000644334 ) ) ;
#29338=CARTESIAN_POINT ( 'NONE',  ( 106.6192711434718206, 27.24117154335861812, 3.695783610869706415 ) ) ;
#29339=CARTESIAN_POINT ( 'NONE',  ( -165.6210506643948577, 79.15024150453834295, 11.77841337596324500 ) ) ;
#29342=CARTESIAN_POINT ( 'NONE',  ( -189.7238975269522712, 107.7611624801371022, 89.42997806037180908 ) ) ;
#29343=CARTESIAN_POINT ( 'NONE',  ( -7.330690860789852437, 6.858814156830895570, 71.96013162991093282 ) ) ;
#29351=VECTOR ( 'NONE', #59177, 1000.000000000000000 ) ;
#29352=ORIENTED_EDGE ( 'NONE', *, *, #51156, .T. ) ;
#29355=VERTEX_POINT ( 'NONE', #54399 ) ;
#29358=ORIENTED_EDGE ( 'NONE', *, *, #52712, .T. ) ;
#29360=CARTESIAN_POINT ( 'NONE',  ( -178.2381786520593323, 93.01028335822120141, -63.56798082661889282 ) ) ;
#29362=VERTEX_POINT ( 'NONE', #48416 ) ;
#29364=CARTESIAN_POINT ( 'NONE',  ( -179.8996803435688889, 95.00451760716450167, 14.69856830855032470 ) ) ;
#29365=CARTESIAN_POINT ( 'NONE',  ( -1.857619870843147725, 6.575690665396233037, 15.34000399991449015 ) ) ;
#29369=CARTESIAN_POINT ( 'NONE',  ( -24.32471770265758337, 9.546495606312143778, -18.39735782029327993 ) ) ;
#29370=CARTESIAN_POINT ( 'NONE',  ( 138.5721691894143817, 44.34516164557651052, 4.313163325010641813 ) ) ;
#29376=CARTESIAN_POINT ( 'NONE',  ( -73.09214866197366689, 21.34321757515763096, 6.031536298108171046 ) ) ;
#29381=CARTESIAN_POINT ( 'NONE',  ( 84.27368848767930842, 18.63026910897604083, -50.45834538360720956 ) ) ;
#29386=CARTESIAN_POINT ( 'NONE',  ( 186.6118452967672283, 84.37814701615442914, -11.78640348934926152 ) ) ;
#29389=CARTESIAN_POINT ( 'NONE',  ( 20.77767936488358558, 7.719073965783881164, -91.09253317339127420 ) ) ;
#29390=CARTESIAN_POINT ( 'NONE',  ( -50.14440374537738876, 14.45628984983895116, 43.50930614590824774 ) ) ;
#29391=EDGE_LOOP ( 'NONE', ( #34411, #37876 ) ) ;
#29396=CARTESIAN_POINT ( 'NONE',  ( 107.9362503323352627, 27.82881837607798303, 71.10819457095023211 ) ) ;
#29399=AXIS2_PLACEMENT_3D ( 'NONE', #13202, #22352, #11787 ) ;
#29401=CARTESIAN_POINT ( 'NONE',  ( -109.7816385129979153, 36.75776661907242726, 64.36293740281786313 ) ) ;
#29403=B_SPLINE_CURVE_WITH_KNOTS ( 'NONE', 3,
 ( #15224, #37352, #53868, #31742, #25795, #21197, #10279, #21872, #52510, #48243, #26125, #43319, #63767, #16597, #5691, #38053 ),
 .UNSPECIFIED., .F., .F.,
 ( 4, 2, 2, 2, 2, 2, 2, 4 ),
 ( 0.000000000000000000, 0.001302991001000006156, 0.002605982002000012312, 0.003908973003000018251, 0.005211964004000024624, 0.006514955005000030996, 0.007817946006000036502, 0.01042392800800004925 ),
 .UNSPECIFIED. ) ;
#29404=CARTESIAN_POINT ( 'NONE',  ( 162.1014732644455307, 61.34312237409764634, -64.55007820984620537 ) ) ;
#29405=ORIENTED_EDGE ( 'NONE', *, *, #53154, .T. ) ;
#29407=ORIENTED_EDGE ( 'NONE', *, *, #43268, .F. ) ;
#29408=EDGE_LOOP ( 'NONE', ( #39029, #29405, #13495, #9102 ) ) ;
#29411=CARTESIAN_POINT ( 'NONE',  ( -71.39537134557981801, 19.68387687359727778, 93.47482192707475690 ) ) ;
#29413=CARTESIAN_POINT ( 'NONE',  ( 67.56108154898468854, 13.77276756375645128, -37.23494202805936482 ) ) ;
#29414=DIRECTION ( 'NONE',  ( -0.8118923937861950435, -0.5838071093367415143, 0.000000000000000000 ) ) ;
#29415=CARTESIAN_POINT ( 'NONE',  ( -62.55184817504200367, 17.87278652436697968, 37.30171783089942039 ) ) ;
#29418=B_SPLINE_CURVE_WITH_KNOTS ( 'NONE', 3,
 ( #33841, #28561, #66222, #39459, #65501, #55992, #34198, #12732, #29590, #55631, #7807, #60216, #12033, #30993, #46460, #57372, #61946, #52090, #46814, #29950, #19735, #8498, #13765, #14465, #3910, #41196, #30301, #45782, #40495, #14113, #51415, #57035, #52440, #3225, #25719, #14799, #31336, #67941, #9532, #62657, #41540, #25379, #3555, #35223, #9185 ),
 .UNSPECIFIED., .F., .F.,
 ( 4, 2, 2, 1, 2, 2, 2, 2, 2, 2, 2, 2, 2, 2, 2, 2, 2, 2, 2, 2, 2, 2, 4 ),
 ( 0.02346057189573571775, 0.02492590417315498907, 0.02565857031186461953, 0.02639123645057425346, 0.02712390258928388739, 0.02785656872799351785, 0.02932190100541277183, 0.03005456714412239189, 0.03078723328283201194, 0.03225256556025124510, 0.03298523169896087903, 0.03371789783767051296, 0.03518323011508977388, 0.03664856239250902786, 0.03738122853121866179, 0.03811389466992828878, 0.03957922694734754970, 0.04104455922476681062, 0.04250989150218607154, 0.04324255764089569160, 0.04397522377960530471, 0.04544055605702456563, 0.04690588833444381961 ),
 .UNSPECIFIED. ) ;
#29419=CARTESIAN_POINT ( 'NONE',  ( 60.40531521312255592, 13.11276739283241710, 30.27770789689484943 ) ) ;
#29420=CARTESIAN_POINT ( 'NONE',  ( 33.60094621367903756, 7.725337012799395886, 86.30269869955574791 ) ) ;
#29422=CARTESIAN_POINT ( 'NONE',  ( -2.866724795119727887, 6.618578306599220085, -37.26994514656705348 ) ) ;
#29424=CARTESIAN_POINT ( 'NONE',  ( -189.2442476610617916, 107.0963225822736433, -41.67591933138472626 ) ) ;
#29427=CARTESIAN_POINT ( 'NONE',  ( -109.0297561673456244, 36.34391931706013423, -66.07908170626511435 ) ) ;
#29428=CARTESIAN_POINT ( 'NONE',  ( 126.3554864210861837, 38.22801630372153170, -16.45079121831199487 ) ) ;
#29430=CARTESIAN_POINT ( 'NONE',  ( 130.7260570116704343, 40.73146260246712558, -36.69216764449773649 ) ) ;
#29434=CARTESIAN_POINT ( 'NONE',  ( -169.3169969001603761, 82.99181976410343964, 85.54137684301231559 ) ) ;
#29436=CARTESIAN_POINT ( 'NONE',  ( 127.4992165631961569, 38.87141012667727580, 6.155430928021909942 ) ) ;
#29437=CARTESIAN_POINT ( 'NONE',  ( -143.8566410313463564, 59.53044870492036011, -10.51068613821876774 ) ) ;
#29439=CARTESIAN_POINT ( 'NONE',  ( 158.1693234658825133, 59.47518947913521714, 83.10736755387232222 ) ) ;
#29440=ORIENTED_EDGE ( 'NONE', *, *, #27865, .F. ) ;
#29442=CARTESIAN_POINT ( 'NONE',  ( -156.0209085498131856, 71.27066046086515883, 34.46375622281639295 ) ) ;
#29445=CARTESIAN_POINT ( 'NONE',  ( 81.76092782665034520, 17.81692437267514606, 16.07796231263216313 ) ) ;
#29448=CARTESIAN_POINT ( 'NONE',  ( 57.08336938683660833, 11.37442068895389014, 41.92839751438462059 ) ) ;
#29453=CARTESIAN_POINT ( 'NONE',  ( 174.6242782760049863, 73.69713439533578025, 40.62850159014154627 ) ) ;
#29455=AXIS2_PLACEMENT_3D ( 'NONE', #32651, #16474, #65722 ) ;
#29457=CARTESIAN_POINT ( 'NONE',  ( -190.6985136298601731, 109.1272424661242582, 94.99999999999866418 ) ) ;
#29459=DIRECTION ( 'NONE',  ( 0.000000000000000000, 0.000000000000000000, 1.000000000000000000 ) ) ;
#29460=EDGE_CURVE ( 'NONE', #10653, #41171, #59456, .T. ) ;
#29463=CARTESIAN_POINT ( 'NONE',  ( -72.77296415263759854, 21.23032531836536307, -47.28051332976320253 ) ) ;
#29464=ORIENTED_EDGE ( 'NONE', *, *, #12, .F. ) ;
#29465=CARTESIAN_POINT ( 'NONE',  ( 210.6592759200687794, 116.7161312026394029, -66.11224254623208196 ) ) ;
#29466=CARTESIAN_POINT ( 'NONE',  ( 137.3861614007145135, 44.78548268714477132, 43.63210590249699550 ) ) ;
#29468=CARTESIAN_POINT ( 'NONE',  ( -31.43908319763710679, -170.0000000000000000, 10.87190381572550280 ) ) ;
#29469=CARTESIAN_POINT ( 'NONE',  ( 67.93317348534927191, 14.90531593353391671, -64.38129521441156555 ) ) ;
#29470=B_SPLINE_CURVE_WITH_KNOTS ( 'NONE', 3,
 ( #22545, #55599, #7428, #8109, #29560, #67552, #39090, #60531, #19010, #66873, #28880, #51024, #60870, #33801, #49969, #55241, #7771, #56642, #1803, #45041, #28523, #12345, #29221, #12695, #23258, #50332, #8463, #67226, #29914, #51374, #7065, #40462, #66184, #3191, #23603, #44704, #34855, #17976, #34161, #2148, #39421, #18315, #39771 ),
 .UNSPECIFIED., .F., .F.,
 ( 4, 2, 2, 2, 2, 2, 2, 2, 2, 2, 2, 2, 1, 2, 2, 2, 2, 2, 2, 2, 2, 4 ),
 ( 0.02358007599568756954, 0.02505677178601662877, 0.02579511968118114798, 0.02653346757634567066, 0.02801016336667472989, 0.02948685915700378912, 0.03022520705216830833, 0.03096355494733283448, 0.03244025073766187983, 0.03391694652799092519, 0.03539364231831997054, 0.03613199021348449669, 0.03687033810864901590, 0.03760868600381354204, 0.03834703389897806125, 0.03982372968930709967, 0.04130042547963613808, 0.04277712126996517650, 0.04351546916512970264, 0.04425381706029422879, 0.04573051285062328802, 0.04720720864095235419 ),
 .UNSPECIFIED. ) ;
#29478=DIRECTION ( 'NONE',  ( -0.000000000000000000, 1.000000000000000000, -0.000000000000000000 ) ) ;
#29481=CARTESIAN_POINT ( 'NONE',  ( -71.57025115638936086, 20.80908992785612099, -18.25007248965231810 ) ) ;
#29483=CARTESIAN_POINT ( 'NONE',  ( -109.3585523124447576, 37.67345343047318806, 40.55142789949354665 ) ) ;
#29484=ORIENTED_EDGE ( 'NONE', *, *, #16464, .F. ) ;
#29485=CARTESIAN_POINT ( 'NONE',  ( -95.08295392099647358, 30.38371693924408135, -94.08104204696795136 ) ) ;
#29486=CARTESIAN_POINT ( 'NONE',  ( 84.97658021689288432, 19.92447159015899061, 56.73708945548396798 ) ) ;
#29489=CARTESIAN_POINT ( 'NONE',  ( -196.7348448768811409, -170.0000000000000000, -68.95563438847170801 ) ) ;
#29491=CARTESIAN_POINT ( 'NONE',  ( -15.27733754929849397, 8.502213909106947298, -41.93932207287456748 ) ) ;
#29494=CIRCLE ( 'NONE', #8159, 243.4957430088094839 ) ;
#29495=CARTESIAN_POINT ( 'NONE',  ( -105.5524494737681920, 34.47420209251092160, -89.44164320824525305 ) ) ;
#29496=CARTESIAN_POINT ( 'NONE',  ( -155.1302201283145905, 69.09929365814129198, -10.49887033788333746 ) ) ;
#29497=VERTEX_POINT ( 'NONE', #2357 ) ;
#29500=DIRECTION ( 'NONE',  ( 0.000000000000000000, 0.000000000000000000, 1.000000000000000000 ) ) ;
#29501=EDGE_LOOP ( 'NONE', ( #11782, #24750, #27796, #24578 ) ) ;
#29503=CARTESIAN_POINT ( 'NONE',  ( 150.2941978382489197, 53.52137138947627903, -72.66572206626821639 ) ) ;
#29504=CARTESIAN_POINT ( 'NONE',  ( -37.79823708645147917, 10.72197716414928692, 33.73258574390899156 ) ) ;
#29506=CARTESIAN_POINT ( 'NONE',  ( 138.6020257460769471, 44.36414356192210562, -37.69519993456503926 ) ) ;
#29516=CARTESIAN_POINT ( 'NONE',  ( 204.6977192012829789, 108.0580384837234931, -90.01503221354883522 ) ) ;
#29518=CARTESIAN_POINT ( 'NONE',  ( -118.6157340058430236, 41.88485941274769431, -67.42784937615110152 ) ) ;
#29519=ORIENTED_EDGE ( 'NONE', *, *, #9690, .T. ) ;
#29520=LINE ( 'NONE', #2802, #7596 ) ;
#29521=CARTESIAN_POINT ( 'NONE',  ( -31.43908319763709258, 9.591432048623765638, 18.37190381572551701 ) ) ;
#29522=CARTESIAN_POINT ( 'NONE',  ( 63.01563776193090405, 12.67277567978497643, 71.65751152968501003 ) ) ;
#29523=CARTESIAN_POINT ( 'NONE',  ( 137.6104751318276840, 44.92718313329106650, 3.668482549248312186 ) ) ;
#29525=ORIENTED_EDGE ( 'NONE', *, *, #9690, .F. ) ;
#29529=ORIENTED_EDGE ( 'NONE', *, *, #18278, .F. ) ;
#29530=CARTESIAN_POINT ( 'NONE',  ( 69.72564955710444679, 15.37006465677309386, 67.51718129031921478 ) ) ;
#29531=CARTESIAN_POINT ( 'NONE',  ( 132.3763947360081374, 40.53774838062970076, 83.34026022301281955 ) ) ;
#29534=CARTESIAN_POINT ( 'NONE',  ( 164.8908506817024033, 64.97619709085125805, -42.49963807020401418 ) ) ;
#29535=ADVANCED_FACE ( 'NONE', ( #62119 ), #67087, .F. ) ;
#29538=DIRECTION ( 'NONE',  ( 0.000000000000000000, -1.000000000000000000, 0.000000000000000000 ) ) ;
#29545=CARTESIAN_POINT ( 'NONE',  ( 80.71682498289317209, 18.54204664833077487, -11.83616858174047515 ) ) ;
#29546=CARTESIAN_POINT ( 'NONE',  ( -177.9671374276251754, 94.25162618736496256, -90.16083395623414276 ) ) ;
#29548=CARTESIAN_POINT ( 'NONE',  ( -142.2675133814582011, 58.27369719190851072, -93.98005135264823195 ) ) ;
#29549=CARTESIAN_POINT ( 'NONE',  ( 130.3245512970360664, 39.33195360491889403, -63.73478426897061411 ) ) ;
#29550=EDGE_CURVE ( 'NONE', #2387, #4848, #63720, .T. ) ;
#29552=CARTESIAN_POINT ( 'NONE',  ( -98.68609963468202295, 32.11186931716883208, 71.46360670857458786 ) ) ;
#29553=CARTESIAN_POINT ( 'NONE',  ( -10.92576759990585877, 8.121994053275063408, 71.29367127698461104 ) ) ;
#29554=VERTEX_POINT ( 'NONE', #15667 ) ;
#29558=CARTESIAN_POINT ( 'NONE',  ( -149.9471644042846776, 65.87751327280741975, -49.80312880028602507 ) ) ;
#29560=CARTESIAN_POINT ( 'NONE',  ( -33.36965723649377935, 10.93726715887721745, 30.46507517067076876 ) ) ;
#29561=CARTESIAN_POINT ( 'NONE',  ( -149.5074843970971017, 64.17983161892348676, -61.65738112195564469 ) ) ;
#29562=CYLINDRICAL_SURFACE ( 'NONE', #38172, 7.500000000000013323 ) ;
#29563=CARTESIAN_POINT ( 'NONE',  ( -48.33725449172840882, 12.98311179783359748, -72.93678671279100456 ) ) ;
#29564=CARTESIAN_POINT ( 'NONE',  ( -0.3740447803642790170, 7.527031846085009192, -17.05744638557283821 ) ) ;
#29565=CARTESIAN_POINT ( 'NONE',  ( 175.5493994043409316, 73.18740965572600032, 15.03151793349688070 ) ) ;
#29566=CARTESIAN_POINT ( 'NONE',  ( -55.05276343752909440, 14.68156374112637508, 18.47277718246750311 ) ) ;
#29569=VERTEX_POINT ( 'NONE', #26221 ) ;
#29575=CARTESIAN_POINT ( 'NONE',  ( -104.5916564445180086, 35.10571011602408475, -8.519735482012867678 ) ) ;
#29577=CARTESIAN_POINT ( 'NONE',  ( -172.7154982671752066, 86.67743928531947972, 57.66624519710474317 ) ) ;
#29585=AXIS2_PLACEMENT_3D ( 'NONE', #47725, #25265, #21015 ) ;
#29586=CARTESIAN_POINT ( 'NONE',  ( 63.01563776193090405, 13.70579113808098093, -8.876140241706053757 ) ) ;
#29587=VERTEX_POINT ( 'NONE', #52600 ) ;
#29589=CARTESIAN_POINT ( 'NONE',  ( -10.91976120871578182, 7.112268444252506150, 57.62380858786094961 ) ) ;
#29590=CARTESIAN_POINT ( 'NONE',  ( 12.04188192036244942, 7.416006018508748632, 57.85736376901041211 ) ) ;
#29593=EDGE_CURVE ( 'NONE', #17986, #35602, #19235, .T. ) ;
#29596=EDGE_CURVE ( 'NONE', #35021, #32880, #15789, .T. ) ;
#29598=ORIENTED_EDGE ( 'NONE', *, *, #15260, .F. ) ;
#29602=AXIS2_PLACEMENT_3D ( 'NONE', #26455, #15205, #42284 ) ;
#29604=CARTESIAN_POINT ( 'NONE',  ( -175.9944734395086243, 91.92390745845762012, 18.41779132216174375 ) ) ;
#29605=CARTESIAN_POINT ( 'NONE',  ( 8.984386073292506936, 6.377982749901330628, 94.42819228249486230 ) ) ;
#29606=CARTESIAN_POINT ( 'NONE',  ( 79.38459371357853911, 17.07499996355401706, -68.16129631415398649 ) ) ;
#29609=EDGE_CURVE ( 'NONE', #52822, #60122, #65960, .T. ) ;
#29615=CARTESIAN_POINT ( 'NONE',  ( -82.93267503967651066, 23.99263498936122474, -63.28692396105326168 ) ) ;
#29622=CARTESIAN_POINT ( 'NONE',  ( 46.51679720856117939, 10.46086439153924452, 61.83516232796673506 ) ) ;
#29625=CARTESIAN_POINT ( 'NONE',  ( 19.74724861314306779, 6.659670522263898107, 4.295403914482277763 ) ) ;
#29628=CARTESIAN_POINT ( 'NONE',  ( 177.0110682437507705, 75.98481089748382544, -76.88340400380999995 ) ) ;
#29631=CARTESIAN_POINT ( 'NONE',  ( 110.7114632166112216, 29.09878355652112347, -24.07788697519004373 ) ) ;
#29632=CARTESIAN_POINT ( 'NONE',  ( 79.52639011421921111, 18.17129627604989395, -40.86144025082357700 ) ) ;
#29633=DIRECTION ( 'NONE',  ( -0.000000000000000000, 1.000000000000000000, -0.000000000000000000 ) ) ;
#29639=ORIENTED_EDGE ( 'NONE', *, *, #32710, .T. ) ;
#29641=CARTESIAN_POINT ( 'NONE',  ( 46.89006465517227440, 9.501960077668742954, 11.05812210281710328 ) ) ;
#29642=CARTESIAN_POINT ( 'NONE',  ( -176.6647631907062816, 92.70765962153599560, 85.38109267834556704 ) ) ;
#29643=CARTESIAN_POINT ( 'NONE',  ( -47.56463531432803649, 12.80077789972090230, -15.38160938467773775 ) ) ;
#29644=CARTESIAN_POINT ( 'NONE',  ( 103.9652201950894721, 26.08439499369983494, -12.46680327629901619 ) ) ;
#29646=CARTESIAN_POINT ( 'NONE',  ( 201.9777685760379597, 102.6876480786892927, 2.861658522975385921 ) ) ;
#29647=AXIS2_PLACEMENT_3D ( 'NONE', #56138, #18511, #39962 ) ;
#29649=CARTESIAN_POINT ( 'NONE',  ( 206.0312234087882644, 109.9233711042669484, 82.99752539405173479 ) ) ;
#29651=CARTESIAN_POINT ( 'NONE',  ( 207.4566510040494620, 111.9649643341356011, 29.73049175326031701 ) ) ;
#29652=CARTESIAN_POINT ( 'NONE',  ( -85.89078989036973155, 26.29712602777652464, 62.73225277927918597 ) ) ;
#29655=B_SPLINE_CURVE_WITH_KNOTS ( 'NONE', 3,
 ( #56094, #44494, #29707, #65976, #60673, #12490, #61368, #28670, #29360, #23407, #44843, #66328, #18117, #39571, #50813, #61022, #12849, #58491, #31435, #41985, #15258, #51517, #25135, #41305, #57479, #58167, #36021, #57140, #52867, #63449, #15604, #25482, #41643, #3321, #4362, #35688, #3661, #36719, #63099, #52539, #46922, #14901, #9983, #30397, #68384, #36367 ),
 .UNSPECIFIED., .F., .F.,
 ( 4, 2, 2, 2, 2, 2, 2, 2, 2, 2, 2, 2, 2, 2, 2, 2, 2, 2, 2, 2, 2, 2, 4 ),
 ( 1.387778780781445676E-17, 0.003736383952885294346, 0.005604575929327934580, 0.007472767905770574814, 0.008406863893991927891, 0.009340959882213282703, 0.01120915185865596284, 0.01214324784687731938, 0.01307734383509867593, 0.01401143982332003421, 0.01494553581154139076, 0.01587963179976274730, 0.01681372778798410211, 0.01774782377620546386, 0.01868191976442681868, 0.01961601575264817349, 0.02055011174086953177, 0.02148420772909088658, 0.02241830371731224139, 0.02428649569375490244, 0.02615468767019755655, 0.02802287964664021760, 0.02989107162308287519 ),
 .UNSPECIFIED. ) ;
#29658=ORIENTED_EDGE ( 'NONE', *, *, #58975, .T. ) ;
#29659=CYLINDRICAL_SURFACE ( 'NONE', #63530, 7.500000000000013323 ) ;
#29660=CARTESIAN_POINT ( 'NONE',  ( 188.5651904823862139, 88.01586411309101265, -69.95864106785619185 ) ) ;
#29662=CARTESIAN_POINT ( 'NONE',  ( -165.9154624515710168, 80.89088623112735377, 40.42332398115727443 ) ) ;
#29664=CARTESIAN_POINT ( 'NONE',  ( -24.03640295269301319, 9.507963273819770578, 9.642600505910863262 ) ) ;
#29667=CARTESIAN_POINT ( 'NONE',  ( 126.6395826915639731, 37.23416510613625974, -45.58068663486469063 ) ) ;
#29669=B_SPLINE_CURVE_WITH_KNOTS ( 'NONE', 3,
 ( #57670, #4204, #47784, #15784, #62942, #10158, #9135, #20718, #69244, #9482, #26007, #63639, #48122, #47434, #26348, #68564, #21074, #26691, #37230, #30940, #3857, #20037, #42845, #52384, #41491, #25669, #52040, #46756, #41833, #31620, #68229, #47102, #63290, #36559, #58009, #9828 ),
 .UNSPECIFIED., .F., .F.,
 ( 4, 2, 2, 2, 2, 2, 2, 2, 2, 2, 2, 2, 2, 2, 2, 2, 2, 4 ),
 ( 3.469446951953614189E-18, 0.001545474820159074359, 0.003090949640318145248, 0.004636424460477216354, 0.006181899280636287027, 0.007727374100795358566, 0.008500111510874876555, 0.009272848920954396279, 0.01081832374111341144, 0.01236379856127242487, 0.01390927338143144003, 0.01545474820159045866, 0.01700022302174947209, 0.01854569784190848725, 0.02009117266206750588, 0.02163664748222652104, 0.02318212230238553967, 0.02472759712254455136 ),
 .UNSPECIFIED. ) ;
#29671=CARTESIAN_POINT ( 'NONE',  ( 188.5076656590985635, 87.95171816312542035, 91.58452734307059018 ) ) ;
#29672=CARTESIAN_POINT ( 'NONE',  ( -14.19493007850031852, 7.389842975086046373, 6.803802910258403891 ) ) ;
#29674=CARTESIAN_POINT ( 'NONE',  ( -26.49516976694649628, 8.831756547364854271, -64.00066573786835988 ) ) ;
#29676=CARTESIAN_POINT ( 'NONE',  ( 14.80205238535216772, 6.470775952815778886, 3.219160964839414607 ) ) ;
#29678=DIRECTION ( 'NONE',  ( -0.8160245890732938934, -0.5780171883497599028, 0.000000000000000000 ) ) ;
#29680=CARTESIAN_POINT ( 'NONE',  ( 178.4027079424739100, 75.93756746109792743, -63.56196981810690971 ) ) ;
#29683=CARTESIAN_POINT ( 'NONE',  ( 107.2672065034543039, 27.52931006625852817, 3.378187332071801663 ) ) ;
#29686=CARTESIAN_POINT ( 'NONE',  ( -48.33725449172840172, 12.98311179783358860, 61.28596623952740430 ) ) ;
#29689=CARTESIAN_POINT ( 'NONE',  ( -4.955782654901478068, 6.720825733572401539, 57.51796347446001789 ) ) ;
#29707=CARTESIAN_POINT ( 'NONE',  ( -174.7869898116916261, 88.99756909636809610, -61.69509254903428541 ) ) ;
#29713=CARTESIAN_POINT ( 'NONE',  ( -180.3153482337535536, 95.51031295027648582, 13.61842630024514378 ) ) ;
#29714=CARTESIAN_POINT ( 'NONE',  ( -1.876547441458563670, 6.576559737910136150, 6.196969845067472171 ) ) ;
#29715=CARTESIAN_POINT ( 'NONE',  ( 58.08938767906773393, 12.61185010801510487, -37.54421099187102584 ) ) ;
#29717=CARTESIAN_POINT ( 'NONE',  ( 150.0047159235711831, 52.07197026280400820, 91.64991005666685453 ) ) ;
#29718=CARTESIAN_POINT ( 'NONE',  ( 136.3292018078239778, 42.93753790426544015, 3.081257596490504458 ) ) ;
#29719=ORIENTED_EDGE ( 'NONE', *, *, #43268, .T. ) ;
#29721=CARTESIAN_POINT ( 'NONE',  ( -73.63128929564830116, 21.53548093502885052, 16.63761306745141866 ) ) ;
#29722=CARTESIAN_POINT ( 'NONE',  ( 45.02738683369923223, 9.207938468499236251, -48.08623862790063441 ) ) ;
#29726=CARTESIAN_POINT ( 'NONE',  ( 79.53408731553405175, 17.12082763744058767, -40.84044364051945308 ) ) ;
#29728=ORIENTED_EDGE ( 'NONE', *, *, #46598, .T. ) ;
#29733=CARTESIAN_POINT ( 'NONE',  ( 187.2465631085773907, 85.06582225041684353, -12.57587812946169770 ) ) ;
#29734=CARTESIAN_POINT ( 'NONE',  ( 140.0614732283738704, 45.29930344725075742, -20.89927350591657529 ) ) ;
#29735=CARTESIAN_POINT ( 'NONE',  ( -86.10360257264198935, 26.38663017581291115, -14.76872716454347767 ) ) ;
#29736=CARTESIAN_POINT ( 'NONE',  ( -179.8926034784145713, 96.58272071140100934, -18.60358020078452768 ) ) ;
#29738=CARTESIAN_POINT ( 'NONE',  ( -47.56466076048270963, 13.83435953640666938, 37.32649237162055300 ) ) ;
#29740=EDGE_LOOP ( 'NONE', ( #28574, #25275, #54654, #12740 ) ) ;
#29742=CARTESIAN_POINT ( 'NONE',  ( -31.43908319763709969, 9.591432048623765638, 30.21645440618916112 ) ) ;
#29743=CARTESIAN_POINT ( 'NONE',  ( 163.2886151008987383, 62.32020850087168640, 59.01466171590617193 ) ) ;
#29744=CARTESIAN_POINT ( 'NONE',  ( -189.2352924136013712, 107.0839554967701304, 64.82041842450834679 ) ) ;
#29748=CIRCLE ( 'NONE', #17386, 243.4957430088094839 ) ;
#29749=CARTESIAN_POINT ( 'NONE',  ( 163.7607557204680404, 62.71181783708026813, -66.35314833076057539 ) ) ;
#29757=CARTESIAN_POINT ( 'NONE',  ( -85.46258339457290276, 25.02772366257408976, 61.58065315855991173 ) ) ;
#29758=CARTESIAN_POINT ( 'NONE',  ( 66.72974708835174340, 13.56459745268606376, -49.75501017375558632 ) ) ;
#29760=CARTESIAN_POINT ( 'NONE',  ( -55.05276343752909440, 15.72344139423348430, 45.31732777293115788 ) ) ;
#29761=CARTESIAN_POINT ( 'NONE',  ( -98.68609963468200874, 32.11186931716881787, -9.070045062816474157 ) ) ;
#29762=CARTESIAN_POINT ( 'NONE',  ( 57.41085175769453741, 12.46982565415947164, 32.32325660257177447 ) ) ;
#29763=CARTESIAN_POINT ( 'NONE',  ( 39.74012880617502930, 8.453553184817396371, 83.60337793500843873 ) ) ;
#29765=CARTESIAN_POINT ( 'NONE',  ( -0.5780275525703858497, 6.527356703336898214, -44.86394364185162686 ) ) ;
#29770=CARTESIAN_POINT ( 'NONE',  ( 17.48988570800758779, 7.568061572928498570, -8.865890789862755028 ) ) ;
#29772=CARTESIAN_POINT ( 'NONE',  ( 199.3743599161303166, 99.31857334527875025, 68.86014906300715666 ) ) ;
#29774=B_SPLINE_CURVE_WITH_KNOTS ( 'NONE', 3,
 ( #29317, #55342, #28625, #45139, #35290, #60974, #56391, #18766, #8211, #66283, #18415, #19102, #40556, #51473, #28982, #44445, #29662, #18075, #51122, #2935, #24399, #45841, #50429, #22999, #34615, #65934, #17729, #34257, #39186, #39525, #7170, #23361, #12800, #56050, #9941, #35643, #26112, #20479, #41944, #63408, #15211, #57435, #31394, #36674, #31056, #37015 ),
 .UNSPECIFIED., .F., .F.,
 ( 4, 2, 2, 2, 2, 2, 2, 2, 2, 2, 2, 2, 2, 2, 2, 2, 2, 2, 2, 2, 2, 2, 4 ),
 ( 1.387778780781445676E-17, 0.003635178948345801821, 0.005452768422518668688, 0.007270357896691534254, 0.008179152633777973108, 0.009087947370864411095, 0.01090553684503733217, 0.01181433158212380832, 0.01272312631921028447, 0.01363192105629676062, 0.01454071579338323504, 0.01544951053046971119, 0.01635830526755618908, 0.01726710000464266176, 0.01817589474172913791, 0.01908468947881561406, 0.01999348421590209021, 0.02090227895298856636, 0.02181107369007504251, 0.02362866316424793930, 0.02544625263842083263, 0.02726384211259372595, 0.02908143158676661927 ),
 .UNSPECIFIED. ) ;
#29775=ORIENTED_EDGE ( 'NONE', *, *, #68602, .F. ) ;
#29776=CARTESIAN_POINT ( 'NONE',  ( -125.8938041572051105, 46.49392987655492959, 57.46449846362076386 ) ) ;
#29780=CARTESIAN_POINT ( 'NONE',  ( -165.6837635325849760, 79.21404047536307758, 91.02581465340531963 ) ) ;
#29782=CARTESIAN_POINT ( 'NONE',  ( 126.4219470349615904, 38.26519385429184439, 11.18839248169725131 ) ) ;
#29785=EDGE_CURVE ( 'NONE', #43079, #61401, #31578, .T. ) ;
#29790=CARTESIAN_POINT ( 'NONE',  ( 163.0539896041220800, 63.43291176144029464, 85.57986349963141492 ) ) ;
#29791=VERTEX_POINT ( 'NONE', #37194 ) ;
#29792=CARTESIAN_POINT ( 'NONE',  ( -58.76099769480632062, 16.75353773354894571, 17.49641683403302039 ) ) ;
#29796=CARTESIAN_POINT ( 'NONE',  ( -155.2836587093739524, 70.59655508952972980, 33.43029846410576766 ) ) ;
#29804=CARTESIAN_POINT ( 'NONE',  ( 58.48209831743719178, 11.66636741727081805, 43.30750159671042354 ) ) ;
#29808=CARTESIAN_POINT ( 'NONE',  ( 177.7886308167536527, 76.74396398590874924, 43.56092108689954046 ) ) ;
#29810=CARTESIAN_POINT ( 'NONE',  ( 23.09541709302173018, 6.844586979481588784, -71.57097287790641360 ) ) ;
#29811=CARTESIAN_POINT ( 'NONE',  ( -129.4036885357274116, 50.06837984316183565, 71.59659508659780158 ) ) ;
#29813=CARTESIAN_POINT ( 'NONE',  ( -97.58423681613963652, 31.57579159344722086, 85.85188415635715842 ) ) ;
#29814=CARTESIAN_POINT ( 'NONE',  ( -71.97658551692140350, 20.95070248419150971, -46.01531844971390228 ) ) ;
#29815=ORIENTED_EDGE ( 'NONE', *, *, #29937, .F. ) ;
#29816=CARTESIAN_POINT ( 'NONE',  ( 210.0055645826033413, 115.7254585628714381, -75.99226608288455509 ) ) ;
#29818=CARTESIAN_POINT ( 'NONE',  ( 113.4418023215250457, 31.50656691678295473, 30.31107852835060612 ) ) ;
#29820=CARTESIAN_POINT ( 'NONE',  ( 39.40195752203892710, 8.409560354027400209, 56.75838489642694640 ) ) ;
#29829=CARTESIAN_POINT ( 'NONE',  ( -172.7116702014380110, 86.67317892691259829, -61.55650775521370122 ) ) ;
#29831=CARTESIAN_POINT ( 'NONE',  ( -109.7079446832838983, 37.86719386855315861, 36.94873819821719252 ) ) ;
#29832=VERTEX_POINT ( 'NONE', #68524 ) ;
#29834=CARTESIAN_POINT ( 'NONE',  ( -38.93878980550034186, 10.94326053663841947, 11.36906375664720947 ) ) ;
#29835=CARTESIAN_POINT ( 'NONE',  ( 82.34401416830216647, 19.05992892018825557, 57.89662370918314593 ) ) ;
#29838=CARTESIAN_POINT ( 'NONE',  ( -189.2442476610617632, 107.0963225822736291, -68.52046992184840235 ) ) ;
#29842=CARTESIAN_POINT ( 'NONE',  ( 33.44983424733137412, 7.709709042132403489, 15.15903636718023328 ) ) ;
#29843=CARTESIAN_POINT ( 'NONE',  ( -14.93280618462406828, 8.469244267267916015, -40.51070958269902889 ) ) ;
#29845=EDGE_CURVE ( 'NONE', #55324, #14098, #42132, .T. ) ;
#29846=VECTOR ( 'NONE', #12128, 1000.000000000000000 ) ;
#29847=VECTOR ( 'NONE', #36271, 1000.000000000000000 ) ;
#29850=ORIENTED_EDGE ( 'NONE', *, *, #1415, .F. ) ;
#29852=CARTESIAN_POINT ( 'NONE',  ( -61.76386578474848932, 17.63453064612501109, 61.27715783582140574 ) ) ;
#29853=FACE_OUTER_BOUND ( 'NONE', #6252, .T. ) ;
#29857=CARTESIAN_POINT ( 'NONE',  ( 153.2208437558771550, 55.67531116261156399, -64.27115891943437020 ) ) ;
#29858=EDGE_CURVE ( 'NONE', #44762, #33459, #53014, .T. ) ;
#29859=CARTESIAN_POINT ( 'NONE',  ( -38.69408084385329971, 10.89529537250243152, 39.68205672784471005 ) ) ;
#29860=CARTESIAN_POINT ( 'NONE',  ( 133.8566784816069628, 41.42467568809806977, -36.02331093239566684 ) ) ;
#29867=CARTESIAN_POINT ( 'NONE',  ( -123.4416615615272832, 44.90042688650404301, 45.21152833363236567 ) ) ;
#29868=CARTESIAN_POINT ( 'NONE',  ( -62.45176220516621868, 16.79101814080731714, -41.46409900258914405 ) ) ;
#29871=B_SPLINE_CURVE_WITH_KNOTS ( 'NONE', 3,
 ( #42016, #5751, #4722, #64856, #31807, #36747, #43034, #21934, #42361, #37082, #16658, #32158, #63475, #64508, #15290, #32840, #48297, #47282, #26873, #130, #58192, #64156, #58524, #21585, #15970, #58870, #16315, #26186, #69073, #37418, #69433, #5419, #10013, #31465, #10342, #52901, #21250, #486, #11034, #47622, #27208, #37771, #63821, #53240, #26533, #47968, #54275 ),
 .UNSPECIFIED., .F., .F.,
 ( 4, 2, 2, 2, 2, 2, 2, 2, 2, 2, 2, 1, 2, 2, 2, 2, 2, 2, 2, 2, 2, 2, 2, 4 ),
 ( 0.000000000000000000, 0.003297771944418878293, 0.004122214930523569569, 0.004946657916628260411, 0.006595543888837659442, 0.007419986874942373703, 0.008244429861047088831, 0.009068872847151803959, 0.009893315833256519087, 0.01154220180546601179, 0.01236664479157075641, 0.01319108777767550277, 0.01401553076378025085, 0.01483997374988499547, 0.01566441673598974182, 0.01648885972209448644, 0.01813774569430391323, 0.01896218868040866826, 0.01978663166651342328, 0.02061107465261817831, 0.02143551763872292987, 0.02308440361093241910, 0.02473328958314190834, 0.02638217555535140105 ),
 .UNSPECIFIED. ) ;
#29872=CARTESIAN_POINT ( 'NONE',  ( 89.21005684773501798, 20.31770592753386850, 57.01058117278675041 ) ) ;
#29876=B_SPLINE_CURVE_WITH_KNOTS ( 'NONE', 3,
 ( #64211, #56436, #65980, #51173, #34994, #7914, #61715, #45193, #33956, #55389, #50476, #8259, #8614, #29364, #2990, #30068, #29713, #51521, #23746, #24449, #7218, #13872, #45890, #44499, #34663, #28674, #66332, #61373, #39575, #39917, #19151, #13539, #39233, #24099, #12494, #50129, #40266, #23052, #7581, #67360, #50818, #1956, #40605, #18469, #62057, #17775 ),
 .UNSPECIFIED., .F., .F.,
 ( 4, 2, 2, 2, 2, 2, 2, 2, 2, 2, 2, 2, 2, 2, 2, 2, 2, 2, 2, 2, 2, 2, 4 ),
 ( 0.000000000000000000, 0.003736383952885362434, 0.005604575929328028255, 0.007472767905770694510, 0.008406863893992026771, 0.009340959882213357296, 0.01120915185865602355, 0.01214324784687736622, 0.01307734383509870889, 0.01401143982332004982, 0.01494553581154139249, 0.01587963179976273342, 0.01681372778798407436, 0.01774782377620541529, 0.01868191976442675623, 0.01961601575264810063, 0.02055011174086944156, 0.02148420772909078943, 0.02241830371731213037, 0.02428649569375483999, 0.02615468767019754615, 0.02802287964664025230, 0.02989107162308296539 ),
 .UNSPECIFIED. ) ;
#29879=CARTESIAN_POINT ( 'NONE',  ( 203.9181091394787018, 105.2759068139670973, 44.20772073876945285 ) ) ;
#29881=CARTESIAN_POINT ( 'NONE',  ( 66.73594759725092729, 13.56641407806657540, 70.67429847145855604 ) ) ;
#29882=CARTESIAN_POINT ( 'NONE',  ( 188.0300953578913266, 85.92260131067908446, -94.54474959917212118 ) ) ;
#29885=CARTESIAN_POINT ( 'NONE',  ( 164.8908506817023465, 64.97619709085121542, -15.65508747974032566 ) ) ;
#29888=CARTESIAN_POINT ( 'NONE',  ( 70.46579300139245561, 15.56614468937219264, 65.15598333419700339 ) ) ;
#29889=CARTESIAN_POINT ( 'NONE',  ( 126.5017642286235287, 37.15732438686229244, 89.18760059589644129 ) ) ;
#29892=CARTESIAN_POINT ( 'NONE',  ( -143.3925773749112125, 59.16144459815139811, -64.80734044691615736 ) ) ;
#29902=CARTESIAN_POINT ( 'NONE',  ( 152.9696068220085863, 55.48791888908662884, -91.30131104750859095 ) ) ;
#29907=CARTESIAN_POINT ( 'NONE',  ( 88.98064924903390249, 21.30386569031176336, 44.33800583418702246 ) ) ;
#29909=CARTESIAN_POINT ( 'NONE',  ( -94.77890319529970498, 30.24118571794802435, 64.36354809645237651 ) ) ;
#29910=CARTESIAN_POINT ( 'NONE',  ( -14.56631729561072852, 8.434645566888203660, 67.78470214004869376 ) ) ;
#29912=CARTESIAN_POINT ( 'NONE',  ( 151.1700480242206197, 54.15904440870133385, -12.70232037378493573 ) ) ;
#29914=CARTESIAN_POINT ( 'NONE',  ( -38.17232309348611352, 11.81874355808867882, 41.05688953177845235 ) ) ;
#29916=CARTESIAN_POINT ( 'NONE',  ( -154.0775378574013814, 68.15437918458555089, -63.19143630128887423 ) ) ;
#29917=CARTESIAN_POINT ( 'NONE',  ( 56.67004931728209982, 11.28989923258780159, 94.99999999999866418 ) ) ;
#29918=CARTESIAN_POINT ( 'NONE',  ( -51.99406906667275052, 13.88268392809765395, -62.70866649372558754 ) ) ;
#29919=CARTESIAN_POINT ( 'NONE',  ( -4.072522659361689890, 7.683023425615370883, -22.57170394412693071 ) ) ;
#29920=CARTESIAN_POINT ( 'NONE',  ( 174.6127059037623042, 72.30368563770915102, 6.133683309753402035 ) ) ;
#29925=CARTESIAN_POINT ( 'NONE',  ( 105.8203563788590742, 26.88901185006199057, -64.20487891140942338 ) ) ;
#29929=CARTESIAN_POINT ( 'NONE',  ( -11.84613025833866473, 7.186187877555967773, 84.96521102128788527 ) ) ;
#29930=CARTESIAN_POINT ( 'NONE',  ( -107.7677210873466009, 36.80113675102408166, -20.80525371622632846 ) ) ;
#29931=ORIENTED_EDGE ( 'NONE', *, *, #24301, .F. ) ;
#29933=CARTESIAN_POINT ( 'NONE',  ( -167.1534554062404538, 80.72263015867915215, 69.71615865952209390 ) ) ;
#29937=EDGE_CURVE ( 'NONE', #18071, #62698, #13128, .T. ) ;
#29938=CARTESIAN_POINT ( 'NONE',  ( -180.5668408223793904, 95.81768001203278118, -95.00000000000133582 ) ) ;
#29939=CARTESIAN_POINT ( 'NONE',  ( 173.6012773665503914, 71.36035397668605640, -17.46879726638741559 ) ) ;
#29941=CARTESIAN_POINT ( 'NONE',  ( 103.8325688302027459, 27.12251147381400784, 60.05448002011801378 ) ) ;
#29943=AXIS2_PLACEMENT_3D ( 'NONE', #34003, #23101, #50865 ) ;
#29944=ADVANCED_FACE ( 'NONE', ( #47394 ), #42808, .F. ) ;
#29945=CARTESIAN_POINT ( 'NONE',  ( 56.52885800925549376, 12.28784885070978916, -20.17303737264423447 ) ) ;
#29948=VERTEX_POINT ( 'NONE', #53358 ) ;
#29949=CARTESIAN_POINT ( 'NONE',  ( 208.6132326550593916, 111.8685719053116543, 16.27391699821244231 ) ) ;
#29950=CARTESIAN_POINT ( 'NONE',  ( 8.683910719548892487, 7.383368463746301735, 61.94290726329433028 ) ) ;
#29951=CARTESIAN_POINT ( 'NONE',  ( 211.7419975634644800, 116.5322580952101390, 34.05327329600243758 ) ) ;
#29952=CARTESIAN_POINT ( 'NONE',  ( 10.79880987033570783, 6.392085142689816202, -91.09258533748153752 ) ) ;
#29953=CARTESIAN_POINT ( 'NONE',  ( -77.71448999903253707, 21.96089801565739208, 18.52841490789106160 ) ) ;
#29960=CARTESIAN_POINT ( 'NONE',  ( 34.45972925205163762, 8.830088223935240066, -75.62682501707777760 ) ) ;
#29961=CYLINDRICAL_SURFACE ( 'NONE', #66923, 7.500000000000020428 ) ;
#29962=CARTESIAN_POINT ( 'NONE',  ( 12.30794027880714303, 6.414170680043896233, 84.55216331891460868 ) ) ;
#29964=B_SPLINE_CURVE_WITH_KNOTS ( 'NONE', 3,
 ( #32070, #31383, #21173, #36661, #4638, #43294, #68994, #59478, #5664, #393, #69354, #64770, #54189, #42948, #15886, #21851, #26101, #47531, #27471, #10951, #10258, #64418, #63742, #20819, #32420, #48914, #42278, #44, #58783, #37001, #53151, #31719, #64074, #6011, #58112, #27125, #4985, #752, #42618, #22207, #59129, #52816, #43645 ),
 .UNSPECIFIED., .F., .F.,
 ( 4, 2, 2, 2, 2, 2, 2, 2, 2, 2, 2, 2, 1, 2, 2, 2, 2, 2, 2, 2, 2, 4 ),
 ( 0.02371951416048007424, 0.02520633211177540287, 0.02594974108742304636, 0.02669315006307068985, 0.02817996801436598031, 0.02966678596566126730, 0.03041019494130891426, 0.03115360391695655776, 0.03264042186825184821, 0.03412723981954713520, 0.03561405777084242219, 0.03635746674649006915, 0.03710087572213771612, 0.03784428469778536308, 0.03858769367343301004, 0.04007451162472831091, 0.04156132957602361178, 0.04304814752731891958, 0.04379155650296657348, 0.04453496547861422045, 0.04602178342990952825, 0.04750860138120482912 ),
 .UNSPECIFIED. ) ;
#29965=CARTESIAN_POINT ( 'NONE',  ( 22.59201934342795681, 7.821623272182323561, 94.42844641394751193 ) ) ;
#29968=CARTESIAN_POINT ( 'NONE',  ( 203.1423857108907498, 105.9238244286949708, -51.17351567888142228 ) ) ;
#29969=VERTEX_POINT ( 'NONE', #3814 ) ;
#29972=CARTESIAN_POINT ( 'NONE',  ( -85.91089317961402116, 25.21459833389208782, -71.46727687246068683 ) ) ;
#29974=ORIENTED_EDGE ( 'NONE', *, *, #48989, .T. ) ;
#29976=CARTESIAN_POINT ( 'NONE',  ( 10.83046137699561484, 6.392429922561258415, -37.37009112564436464 ) ) ;
#29977=CARTESIAN_POINT ( 'NONE',  ( -108.8556526337305996, 37.39618721751735819, -92.58918846270292136 ) ) ;
#29978=CARTESIAN_POINT ( 'NONE',  ( 103.8055367708241050, 27.11070767929348335, 14.14709985013681148 ) ) ;
#29983=CARTESIAN_POINT ( 'NONE',  ( 176.6238742729554474, 75.60943990211363541, -76.61804891973169163 ) ) ;
#29985=B_SPLINE_CURVE_WITH_KNOTS ( 'NONE', 3,
 ( #69006, #762, #10962, #22216, #1111, #17640, #16239, #38390, #6730, #54198, #48229, #43653, #32769, #44357, #5348, #22561, #48569, #65841, #16586, #39107, #27838, #54, #12360, #37691, #54906, #6021, #21514, #26802, #404, #28176, #60546, #17275, #32429, #65132, #43304, #38749, #12011, #59831, #5673, #27481, #64780, #33817, #44004, #11649, #65482, #60193, #42957, #48922, #64428, #33484, #49628, #53856, #16926, #27136, #1457, #38043, #21861, #33126, #54556, #59487 ),
 .UNSPECIFIED., .F., .F.,
 ( 4, 2, 2, 2, 2, 2, 2, 2, 2, 2, 2, 2, 2, 2, 2, 2, 2, 2, 2, 2, 2, 2, 2, 2, 2, 2, 2, 2, 2, 4 ),
 ( 0.000000000000000000, 0.002104973360485384165, 0.003157460040728082319, 0.004209946720970781341, 0.005262433401213479495, 0.006314920081456177649, 0.007367406761698876670, 0.008419893441941574824, 0.009472380122184272111, 0.01052486680242696940, 0.01157735348266966668, 0.01262984016291236397, 0.01368232684315506473, 0.01473481352339776722, 0.01683978688388317740, 0.01789227356412587816, 0.01894476024436858239, 0.01999724692461128661, 0.02104973360485398737, 0.02315470696533938194, 0.02420719364558207923, 0.02525968032582477651, 0.02631216700606748074, 0.02736465368631018150, 0.02841714036655287878, 0.02946962704679557954, 0.03052211372703827683, 0.03157460040728097411, 0.03262708708752367487, 0.03367957376776637562 ),
 .UNSPECIFIED. ) ;
#29986=CARTESIAN_POINT ( 'NONE',  ( 112.7784411285249178, 30.07270878825233851, -23.64024644625330751 ) ) ;
#29987=CARTESIAN_POINT ( 'NONE',  ( 84.26390409839196138, 19.68678207880321196, -36.18818452320425649 ) ) ;
#29993=CARTESIAN_POINT ( 'NONE',  ( 45.90693067088658097, 9.344800815249309167, 14.33438021413847530 ) ) ;
#29998=CARTESIAN_POINT ( 'NONE',  ( 55.56474667084417263, 11.06706367715628758, -69.07264011740940646 ) ) ;
#30000=CARTESIAN_POINT ( 'NONE',  ( 126.4754729582247847, 37.14269484129876275, 11.52096225339949598 ) ) ;
#30001=CARTESIAN_POINT ( 'NONE',  ( -31.01099134985120642, 9.521461689106248016, -89.01550512782000624 ) ) ;
#30002=CARTESIAN_POINT ( 'NONE',  ( 211.9209160201162945, 118.6566773314361001, 88.36684836799790332 ) ) ;
#30003=CARTESIAN_POINT ( 'NONE',  ( 208.9583973663597192, 114.1615900753670445, 30.51926161164170992 ) ) ;
#30004=CARTESIAN_POINT ( 'NONE',  ( -83.13046924527392889, 25.15778674529014225, 58.73105344031623787 ) ) ;
#30008=CARTESIAN_POINT ( 'NONE',  ( 8.537735592981562149, 7.383000420390739116, -14.24046554414789867 ) ) ;
#30010=CARTESIAN_POINT ( 'NONE',  ( 197.8572563162090887, 97.41072138832261373, -13.89129495889377175 ) ) ;
#30012=CARTESIAN_POINT ( 'NONE',  ( -148.6471085600699951, 64.76880961642446266, 3.913156007458206798 ) ) ;
#30013=CARTESIAN_POINT ( 'NONE',  ( 187.8973304652193406, 87.27378997243175718, -73.71654343158144229 ) ) ;
#30014=CARTESIAN_POINT ( 'NONE',  ( -38.20537251366653209, 11.82499390270895390, 88.10609205668197319 ) ) ;
#30015=CARTESIAN_POINT ( 'NONE',  ( -94.78109144324895396, 29.13179392050636807, -42.79980480196593362 ) ) ;
#30016=CARTESIAN_POINT ( 'NONE',  ( -29.50439180771548209, 10.29976981300626804, 3.609381438886668736 ) ) ;
#30017=CYLINDRICAL_SURFACE ( 'NONE', #29295, 7.500000000000020428 ) ;
#30018=CYLINDRICAL_SURFACE ( 'NONE', #21368, 7.500000000000013323 ) ;
#30019=CARTESIAN_POINT ( 'NONE',  ( 129.4987365823222376, 38.85470922756776702, -49.63207471537052129 ) ) ;
#30026=CARTESIAN_POINT ( 'NONE',  ( -27.70562707895079768, 9.007984652865422603, -76.18518309368259622 ) ) ;
#30029=CARTESIAN_POINT ( 'NONE',  ( 8.848532525911927848, 6.377649276597439965, 13.54568704989812034 ) ) ;
#30030=ORIENTED_EDGE ( 'NONE', *, *, #56639, .T. ) ;
#30032=CARTESIAN_POINT ( 'NONE',  ( -59.57462349605617646, 16.98779896904799358, -75.56450611661117023 ) ) ;
#30033=CARTESIAN_POINT ( 'NONE',  ( 174.9053416555737215, 72.57849647436445650, -74.85130122728419622 ) ) ;
#30038=CARTESIAN_POINT ( 'NONE',  ( -24.95029760921699946, 9.631514785009935409, 60.79180759298469638 ) ) ;
#30040=CARTESIAN_POINT ( 'NONE',  ( -50.14771795543005339, 13.42081263859821050, 58.96722719906514953 ) ) ;
#30042=EDGE_CURVE ( 'NONE', #14210, #31197, #29005, .T. ) ;
#30043=CARTESIAN_POINT ( 'NONE',  ( -0.7174461528505765573, 6.532311451815528969, 66.86584012114198572 ) ) ;
#30047=CARTESIAN_POINT ( 'NONE',  ( -130.6002960060535827, 49.67125682092490990, -75.11777304400855826 ) ) ;
#30049=CARTESIAN_POINT ( 'NONE',  ( -47.60396279792517760, 12.80997843568595229, -43.72255466512232402 ) ) ;
#30055=AXIS2_PLACEMENT_3D ( 'NONE', #24786, #14904, #14232 ) ;
#30061=B_SPLINE_CURVE_WITH_KNOTS ( 'NONE', 3,
 ( #46752, #47097, #57666, #15098, #68224, #19675, #41136, #42170, #41486, #9824, #12764, #68559, #34224, #62937, #20362, #14741, #41829, #63286, #36553, #31282, #52709, #22094, #43188, #42840, #27711, #10842, #63633, #22440, #37225, #281, #64662, #53051, #4876, #21068, #16471, #48800, #26687, #65011, #64311, #42514, #54079, #53741, #642, #16806, #5898, #63966, #58335, #10494, #47780, #48116 ),
 .UNSPECIFIED., .F., .F.,
 ( 4, 2, 2, 2, 2, 2, 2, 2, 2, 2, 2, 2, 2, 2, 2, 2, 2, 2, 2, 2, 2, 2, 2, 2, 4 ),
 ( 0.02688458561150008919, 0.02770990876165288844, 0.02853523191180568769, 0.03018587821211130354, 0.03183652451241691245, 0.03266184766256971517, 0.03348717081272251789, 0.03513781711302807476, 0.03678846341333363162, 0.03761378656348642741, 0.03843910971363923013, 0.03926443286379202591, 0.04008975601394482863, 0.04174040231425042713, 0.04256572546440322291, 0.04339104861455601175, 0.04421637176470880753, 0.04504169491486159638, 0.04586701806501439216, 0.04669234121516718794, 0.04834298751547283501, 0.04916831066562561692, 0.04999363381577841270, 0.05164428011608405977, 0.05329492641638969297 ),
 .UNSPECIFIED. ) ;
#30062=ORIENTED_EDGE ( 'NONE', *, *, #46604, .F. ) ;
#30066=EDGE_LOOP ( 'NONE', ( #36412, #37689 ) ) ;
#30068=CARTESIAN_POINT ( 'NONE',  ( -180.2252811616041868, 95.40045830523435200, 13.89892224170345614 ) ) ;
#30072=CARTESIAN_POINT ( 'NONE',  ( -30.95341298663139540, 10.53108683215057795, -23.47264677473819816 ) ) ;
#30073=CARTESIAN_POINT ( 'NONE',  ( 135.4423125506059478, 42.39015362494586725, 2.831777643547055856 ) ) ;
#30077=CARTESIAN_POINT ( 'NONE',  ( 46.13856685535758118, 9.381502944822518231, -39.78633803483338482 ) ) ;
#30078=CARTESIAN_POINT ( 'NONE',  ( -71.63719014813169395, 20.83242381180886937, 88.97194804729541318 ) ) ;
#30079=CARTESIAN_POINT ( 'NONE',  ( -189.2776534485022069, -170.0000000000000000, -95.00000000000133582 ) ) ;
#30084=CARTESIAN_POINT ( 'NONE',  ( -142.0251973982164770, 58.08401473564117623, 64.47829236375538642 ) ) ;
#30089=DIRECTION ( 'NONE',  ( -0.000000000000000000, 1.000000000000000000, -0.000000000000000000 ) ) ;
#30091=CARTESIAN_POINT ( 'NONE',  ( -81.01931326044685022, 24.31309346877660715, -8.645523102376230895 ) ) ;
#30093=ADVANCED_FACE ( 'NONE', ( #29333 ), #61346, .F. ) ;
#30094=CARTESIAN_POINT ( 'NONE',  ( -151.2497169612549044, 65.66843968092747730, -34.96368695887081657 ) ) ;
#30098=CARTESIAN_POINT ( 'NONE',  ( -109.7643866341847172, 37.89854104106755273, 10.62320483512874070 ) ) ;
#30099=CARTESIAN_POINT ( 'NONE',  ( 109.3079614081140818, 28.45126415661779617, 71.41187614436252318 ) ) ;
#30101=CARTESIAN_POINT ( 'NONE',  ( -189.7987719395348734, 107.8653664616570609, 68.14804509738834781 ) ) ;
#30105=CARTESIAN_POINT ( 'NONE',  ( -142.9201923544618182, 60.07121543956493781, 88.30931796572481574 ) ) ;
#30107=EDGE_CURVE ( 'NONE', #23015, #48266, #50784, .T. ) ;
#30108=ORIENTED_EDGE ( 'NONE', *, *, #58570, .T. ) ;
#30109=EDGE_CURVE ( 'NONE', #2286, #32665, #28457, .T. ) ;
#30113=CYLINDRICAL_SURFACE ( 'NONE', #22912, 7.500000000000020428 ) ;
#30114=CARTESIAN_POINT ( 'NONE',  ( 174.7690563370620112, 72.45075441521997561, -93.36227965153190667 ) ) ;
#30115=CARTESIAN_POINT ( 'NONE',  ( 64.69649025047537805, 13.06878919510321602, -50.53396286999748099 ) ) ;
#30116=CARTESIAN_POINT ( 'NONE',  ( 109.8560624239070336, 28.70302459854760713, -89.61153874658104712 ) ) ;
#30117=EDGE_CURVE ( 'NONE', #56201, #48145, #28944, .T. ) ;
#30118=CARTESIAN_POINT ( 'NONE',  ( -56.01329802674221980, 15.98369420723828860, 30.36332081584329856 ) ) ;
#30119=B_SPLINE_CURVE_WITH_KNOTS ( 'NONE', 3,
 ( #55612, #7441, #21858, #43300, #64776, #9161, #46093, #13066, #29925, #66537, #18326, #40819, #62273, #35551, #45052, #2849, #46436, #56303, #19713, #14092, #34866, #51388, #67915, #41174, #50346, #13403, #67562, #45757, #23954, #29234, #8827, #14443, #45404, #24316, #57349, #35895, #67237, #19021, #39784, #66887, #40472, #55970, #18681, #8122 ),
 .UNSPECIFIED., .F., .F.,
 ( 4, 2, 2, 2, 2, 2, 2, 2, 2, 2, 2, 2, 2, 2, 2, 2, 2, 2, 2, 2, 2, 4 ),
 ( 0.000000000000000000, 0.001533942663855612787, 0.003067885327711225574, 0.004601827991566838361, 0.005368799323494643019, 0.006135770655422447678, 0.007669713319278084751, 0.008436684651205901553, 0.009203655983133720089, 0.01073759864698937451, 0.01150456997891720172, 0.01227154131084502893, 0.01303851264277285787, 0.01380548397470068335, 0.01533942663855629787, 0.01687336930241191066, 0.01840731196626752345, 0.01994125463012313623, 0.02070822596205094956, 0.02147519729397876637, 0.02300913995783438262, 0.02454308262169000235 ),
 .UNSPECIFIED. ) ;
#30120=CARTESIAN_POINT ( 'NONE',  ( -37.93983213483220140, 11.77368372188049328, -65.88929680851603621 ) ) ;
#30122=CARTESIAN_POINT ( 'NONE',  ( 32.10490206750998965, 7.572278537213176008, 92.86731323645747693 ) ) ;
#30125=CARTESIAN_POINT ( 'NONE',  ( -0.5158933718595617446, 6.525180340836105763, -41.22077923227989515 ) ) ;
#30127=CARTESIAN_POINT ( 'NONE',  ( -118.6849742182705398, 41.92701402439733016, 13.36181871470159876 ) ) ;
#30128=CARTESIAN_POINT ( 'NONE',  ( 65.41496713438826305, 13.24164235279043389, -62.94294025472531473 ) ) ;
#30129=CARTESIAN_POINT ( 'NONE',  ( 126.8947007444828898, 37.37669340849691224, -19.48012531352281584 ) ) ;
#30131=CARTESIAN_POINT ( 'NONE',  ( -107.0751323097254470, 35.28386110859231906, -75.14699250370651384 ) ) ;
#30134=CARTESIAN_POINT ( 'NONE',  ( 63.01563776193091826, 12.67277567978495512, -89.40979201309708913 ) ) ;
#30144=CARTESIAN_POINT ( 'NONE',  ( -145.9095871962850595, 61.18682730038540285, -8.883549365152694222 ) ) ;
#30145=CARTESIAN_POINT ( 'NONE',  ( 199.3764173596862008, 100.9540560740992134, 4.553511661046183434 ) ) ;
#30149=CARTESIAN_POINT ( 'NONE',  ( 161.5974713863948011, 62.23003014314474513, 84.30540274493955621 ) ) ;
#30151=CARTESIAN_POINT ( 'NONE',  ( -55.54036735998992924, 15.85474597822063281, 18.47277718246749956 ) ) ;
#30153=CARTESIAN_POINT ( 'NONE',  ( -153.6994314938755224, 69.16570456337669270, 44.45659357967959124 ) ) ;
#30156=DIRECTION ( 'NONE',  ( -0.000000000000000000, 1.000000000000000000, -0.000000000000000000 ) ) ;
#30159=CARTESIAN_POINT ( 'NONE',  ( 57.07734607129818016, 11.37318329671159312, 32.70553640740841672 ) ) ;
#30162=CARTESIAN_POINT ( 'NONE',  ( -165.9121868482146454, 80.88751546905565704, 9.386801319154086443 ) ) ;
#30163=CARTESIAN_POINT ( 'NONE',  ( 20.36314374176837916, 6.689939636827348934, -75.82707789680702604 ) ) ;
#30166=CARTESIAN_POINT ( 'NONE',  ( -95.44494005344630239, 30.55403701725966670, 88.60368125266712980 ) ) ;
#30167=CARTESIAN_POINT ( 'NONE',  ( -75.43495400358861502, 22.18831810339349886, -49.38790907511541661 ) ) ;
#30168=ORIENTED_EDGE ( 'NONE', *, *, #32865, .F. ) ;
#30169=CARTESIAN_POINT ( 'NONE',  ( 209.6698611676811481, 115.2210955123518517, -65.03741327442061504 ) ) ;
#30170=CARTESIAN_POINT ( 'NONE',  ( 8.000000000000007105, 249.8719672152120381, -95.00000000000133582 ) ) ;
#30172=CARTESIAN_POINT ( 'NONE',  ( 114.6797682035589219, 32.10876583290006892, 31.04538199320165148 ) ) ;
#30174=CARTESIAN_POINT ( 'NONE',  ( 68.94948716683072121, 15.16699441119056146, -74.67836426230981317 ) ) ;
#30177=CARTESIAN_POINT ( 'NONE',  ( 11.79090982778180141, 7.411142935774506668, -90.30599167494429480 ) ) ;
#30180=CARTESIAN_POINT ( 'NONE',  ( -47.88880928231646550, 12.87693921808227770, -94.14315601767113151 ) ) ;
#30181=CARTESIAN_POINT ( 'NONE',  ( -54.62718114890975585, 15.60883832648648095, -88.90542517938722256 ) ) ;
#30183=CARTESIAN_POINT ( 'NONE',  ( 70.50376765786471367, 15.57629333413342998, -43.71097164717498629 ) ) ;
#30185=CARTESIAN_POINT ( 'NONE',  ( 204.6977192012829789, 106.3443248447423599, 56.05227132923312183 ) ) ;
#30188=CARTESIAN_POINT ( 'NONE',  ( -108.5248383251030333, 37.21456094989613206, 33.85788099656151218 ) ) ;
#30189=VERTEX_POINT ( 'NONE', #14875 ) ;
#30190=CARTESIAN_POINT ( 'NONE',  ( -32.41627406084104734, 9.753381371531503419, 18.32381523465870288 ) ) ;
#30191=CARTESIAN_POINT ( 'NONE',  ( 79.92842440418705507, 18.29578799637231512, 60.65141981179670694 ) ) ;
#30200=CARTESIAN_POINT ( 'NONE',  ( -12.40598104375063571, 8.242193636955557068, -36.95900104685619425 ) ) ;
#30204=ORIENTED_EDGE ( 'NONE', *, *, #41476, .F. ) ;
#30207=CARTESIAN_POINT ( 'NONE',  ( -173.1211646369891355, -170.0000000000000000, -88.40105834567734178 ) ) ;
#30208=CARTESIAN_POINT ( 'NONE',  ( -57.65574514524054450, 16.43983577669854768, 57.62394589512655330 ) ) ;
#30209=CARTESIAN_POINT ( 'NONE',  ( -189.4248691432192118, 107.3461292335514230, 9.845412498708020266 ) ) ;
#30212=CARTESIAN_POINT ( 'NONE',  ( -58.35379405639710626, 15.59115156255354329, -89.65743652648848183 ) ) ;
#30213=CARTESIAN_POINT ( 'NONE',  ( -38.55214349681829589, 10.86754840574842085, 35.28784456186913587 ) ) ;
#30214=CARTESIAN_POINT ( 'NONE',  ( 154.4435090467313501, 56.59612921827833532, -36.75824220859233549 ) ) ;
#30217=CARTESIAN_POINT ( 'NONE',  ( -155.1204242627070187, 70.44799358128194910, 60.08489091306021379 ) ) ;
#30218=CARTESIAN_POINT ( 'NONE',  ( -188.6739852773921200, 108.2139733222100375, 66.97274234833881223 ) ) ;
#30221=CARTESIAN_POINT ( 'NONE',  ( -175.9864315813574933, 91.91454246454364352, -76.00044308918302249 ) ) ;
#30225=CARTESIAN_POINT ( 'NONE',  ( 114.4640969196986191, 30.88424258798505306, 30.90719979216948943 ) ) ;
#30230=CARTESIAN_POINT ( 'NONE',  ( 203.1511228994173734, 104.2426341584999392, 29.32292381179308904 ) ) ;
#30232=CARTESIAN_POINT ( 'NONE',  ( 187.8965227056807521, 87.27289477191496303, 39.95742566600716827 ) ) ;
#30233=CARTESIAN_POINT ( 'NONE',  ( 140.9141742510256279, 47.05414327990545331, 7.575130398038848689 ) ) ;
#30234=FACE_OUTER_BOUND ( 'NONE', #44877, .T. ) ;
#30235=ORIENTED_EDGE ( 'NONE', *, *, #2569, .F. ) ;
#30236=CARTESIAN_POINT ( 'NONE',  ( 164.6598737201887843, 64.78038692612514637, -18.98586800582112133 ) ) ;
#30238=CARTESIAN_POINT ( 'NONE',  ( 8.000000000000007105, 249.8719672152120381, 94.99999999999866418 ) ) ;
#30239=CARTESIAN_POINT ( 'NONE',  ( 126.7968382499399809, 37.32194343744114207, 88.14309609214454611 ) ) ;
#30243=CARTESIAN_POINT ( 'NONE',  ( -149.5074843970971017, 64.17983161892348676, -61.65738112195564469 ) ) ;
#30245=VECTOR ( 'NONE', #56168, 1000.000000000000000 ) ;
#30246=CARTESIAN_POINT ( 'NONE',  ( 163.7607557204680404, 62.71181783708028235, -39.50859774029689930 ) ) ;
#30248=CARTESIAN_POINT ( 'NONE',  ( -99.10904156412044586, 32.31949011661293270, 17.98775302372827056 ) ) ;
#30251=CARTESIAN_POINT ( 'NONE',  ( 55.82249137702105202, 12.14481401622953527, 88.85236193575613584 ) ) ;
#30255=CARTESIAN_POINT ( 'NONE',  ( -171.0814041607219451, 84.88598211196838861, 31.09197369155747381 ) ) ;
#30256=CARTESIAN_POINT ( 'NONE',  ( 150.2794558856211324, 52.26944788078752424, 65.95378106583270039 ) ) ;
#30258=B_SPLINE_CURVE_WITH_KNOTS ( 'NONE', 3,
 ( #51211, #40998, #62454, #19184, #40638, #62098, #13914, #35376, #26199, #15981, #47979, #37784, #4734, #31820, #49012, #53940, #21602, #5763, #27222, #47635, #37431, #850, #27570, #63834, #53251, #26885, #22302, #58882, #43739, #10697, #65217, #37095, #59229, #15644, #32172, #53604, #64519, #11384, #58534, #6111, #36759, #48658, #31477, #64869, #10354 ),
 .UNSPECIFIED., .F., .F.,
 ( 4, 2, 2, 1, 2, 2, 2, 2, 2, 2, 2, 2, 2, 2, 2, 2, 2, 2, 2, 2, 2, 2, 4 ),
 ( 0.02345095402629350512, 0.02491692321306682514, 0.02564990780645348689, 0.02638289239984014517, 0.02711587699322680345, 0.02784886158661346520, 0.02931483077338677481, 0.03004781536677342962, 0.03078079996016008443, 0.03224676914693339058, 0.03297975374032004886, 0.03371273833370670020, 0.03517870752048000982, 0.03664467670725331944, 0.03737766130063997772, 0.03811064589402662905, 0.03957661508079991786, 0.04104258426757321360, 0.04250855345434650934, 0.04324153804773314680, 0.04397452264111979814, 0.04544049182789308694, 0.04690646101466637574 ),
 .UNSPECIFIED. ) ;
#30260=CARTESIAN_POINT ( 'NONE',  ( -96.45303203827901939, 31.03218867996498531, 69.61143926203455123 ) ) ;
#30261=CARTESIAN_POINT ( 'NONE',  ( -8.800520192024523070, 7.964629484975256801, 57.00751323463713760 ) ) ;
#30263=EDGE_CURVE ( 'NONE', #42164, #42704, #3227, .T. ) ;
#30264=CARTESIAN_POINT ( 'NONE',  ( 149.9883446984744637, 53.30011109831374227, -17.36738191414244170 ) ) ;
#30265=CARTESIAN_POINT ( 'NONE',  ( 39.40195752203892710, -170.0000000000000000, -96.80891864635512434 ) ) ;
#30266=CARTESIAN_POINT ( 'NONE',  ( 104.7042813665017462, 27.49927371769997464, 42.19190249457584940 ) ) ;
#30267=CARTESIAN_POINT ( 'NONE',  ( -0.9897066053608900571, 7.549089325901769065, 34.51982852159657256 ) ) ;
#30268=CARTESIAN_POINT ( 'NONE',  ( 63.68918951593933997, 12.82977143588412972, 83.52517258632475716 ) ) ;
#30269=CARTESIAN_POINT ( 'NONE',  ( 186.0827296088606602, 85.28826835108064586, 15.56026340398669916 ) ) ;
#30271=CARTESIAN_POINT ( 'NONE',  ( 177.0024338932393562, 74.57605685449961186, 16.27244958310170020 ) ) ;
#30272=CARTESIAN_POINT ( 'NONE',  ( -62.54085973597664605, 16.81797209566546414, 10.48152732957156630 ) ) ;
#30274=DIRECTION ( 'NONE',  ( 0.000000000000000000, 0.000000000000000000, 1.000000000000000000 ) ) ;
#30278=CARTESIAN_POINT ( 'NONE',  ( 46.80475532923159676, 10.50744084852536986, -17.50383325418069091 ) ) ;
#30279=EDGE_CURVE ( 'NONE', #39717, #55323, #47760, .T. ) ;
#30282=LINE ( 'NONE', #62974, #23268 ) ;
#30284=VERTEX_POINT ( 'NONE', #62989 ) ;
#30285=CARTESIAN_POINT ( 'NONE',  ( -71.16770070143911653, 19.60548673929831764, 64.23797182331117028 ) ) ;
#30286=CARTESIAN_POINT ( 'NONE',  ( -170.2801941679960294, 84.02053682015862535, 58.21222663911628104 ) ) ;
#30289=CARTESIAN_POINT ( 'NONE',  ( -154.0775378574013814, 68.15437918458553668, 44.18676606056580169 ) ) ;
#30291=CARTESIAN_POINT ( 'NONE',  ( 176.6214367443248250, 74.20967084876664899, -10.83384295640149730 ) ) ;
#30292=CARTESIAN_POINT ( 'NONE',  ( 105.7953515382196343, 27.97683113100023888, 70.01405529446219589 ) ) ;
#30295=CARTESIAN_POINT ( 'NONE',  ( 57.07246224906423748, 12.39953617563784327, -11.77494754054097470 ) ) ;
#30296=VERTEX_POINT ( 'NONE', #61944 ) ;
#30297=AXIS2_PLACEMENT_3D ( 'NONE', #52533, #4356, #31429 ) ;
#30299=EDGE_LOOP ( 'NONE', ( #27032, #61335 ) ) ;
#30300=CARTESIAN_POINT ( 'NONE',  ( 22.28556289340099994, 7.803548444155007147, -46.77340716559223210 ) ) ;
#30301=CARTESIAN_POINT ( 'NONE',  ( 8.478575283864731915, 7.382882227715640511, 66.05570129574820726 ) ) ;
#30302=CARTESIAN_POINT ( 'NONE',  ( 211.7451286015360665, 116.5372661580811098, 39.29095847353463711 ) ) ;
#30307=CARTESIAN_POINT ( 'NONE',  ( -132.8211701626061370, 52.46221387263234703, 94.70213310676591334 ) ) ;
#30308=CARTESIAN_POINT ( 'NONE',  ( 36.77024545412684375, 9.095083943590502429, -76.99170081823220357 ) ) ;
#30310=CARTESIAN_POINT ( 'NONE',  ( 8.452306438776274078, 6.376630025498653431, 89.60986528594584399 ) ) ;
#30312=CARTESIAN_POINT ( 'NONE',  ( 85.67138972405896880, 19.09593469918313247, -77.62004818985134591 ) ) ;
#30315=CARTESIAN_POINT ( 'NONE',  ( 197.6329787101074373, 98.74106466892206413, -46.36182222220342197 ) ) ;
#30317=CARTESIAN_POINT ( 'NONE',  ( -80.31691774066406708, 22.95709084517032395, 18.39362405332230566 ) ) ;
#30319=CARTESIAN_POINT ( 'NONE',  ( -81.00507684688699328, 23.22613445438387103, -62.32995080790337994 ) ) ;
#30323=CARTESIAN_POINT ( 'NONE',  ( 13.37820144534468625, 6.435512790162277952, -35.91245910506206940 ) ) ;
#30326=CARTESIAN_POINT ( 'NONE',  ( 19.53470118933707056, 6.649487981843464013, 4.168281182200566981 ) ) ;
#30329=CARTESIAN_POINT ( 'NONE',  ( -23.93384176999330037, 8.479327181248127232, 91.56969707628782373 ) ) ;
#30330=CARTESIAN_POINT ( 'NONE',  ( 174.4978817191264682, 73.57770570413207167, -74.16780078678564792 ) ) ;
#30332=CARTESIAN_POINT ( 'NONE',  ( -126.8016613879753862, 48.30316697011515004, -8.110637278710640885 ) ) ;
#30333=CARTESIAN_POINT ( 'NONE',  ( 103.0103829243729194, 25.67737053862328267, -41.37271453292686374 ) ) ;
#30334=DIRECTION ( 'NONE',  ( -0.000000000000000000, 1.000000000000000000, -0.000000000000000000 ) ) ;
#30335=CARTESIAN_POINT ( 'NONE',  ( -165.9719475799887221, 80.94902045251464529, -93.61803425850247606 ) ) ;
#30340=CARTESIAN_POINT ( 'NONE',  ( -80.32755469740935439, 24.04130076192507204, -62.14234554664773214 ) ) ;
#30341=CARTESIAN_POINT ( 'NONE',  ( -0.4996266546846072631, 6.524616273922395848, -95.00000000000133582 ) ) ;
#30344=CARTESIAN_POINT ( 'NONE',  ( 126.9201538765324386, 37.39093565120715112, 13.02954706411735053 ) ) ;
#30346=CARTESIAN_POINT ( 'NONE',  ( 210.8246821066057635, 116.9679728619736210, 94.73533617371974458 ) ) ;
#30350=EDGE_LOOP ( 'NONE', ( #66710, #25128 ) ) ;
#30351=CARTESIAN_POINT ( 'NONE',  ( 8.337549025192451779, 7.382630697225775585, -17.16211394505371146 ) ) ;
#30353=CARTESIAN_POINT ( 'NONE',  ( 203.1511228994173734, 104.2426341584999534, -24.36617736913426668 ) ) ;
#30354=VERTEX_POINT ( 'NONE', #56328 ) ;
#30357=CARTESIAN_POINT ( 'NONE',  ( 187.2384682876461852, 86.54721710842891014, -66.25374784196327482 ) ) ;
#30359=CARTESIAN_POINT ( 'NONE',  ( 65.40032188136231639, 13.23841673691966214, -23.49107392329795019 ) ) ;
#30361=CARTESIAN_POINT ( 'NONE',  ( -31.43908319763709969, 10.61114334766715572, 3.371903815725488585 ) ) ;
#30362=CARTESIAN_POINT ( 'NONE',  ( -107.0751323097254470, 35.28386110859231195, 5.386659267684521524 ) ) ;
#30363=CARTESIAN_POINT ( 'NONE',  ( 9.819093282782489496, 7.389085782749408970, -38.45181758483611389 ) ) ;
#30366=ORIENTED_EDGE ( 'NONE', *, *, #1920, .T. ) ;
#30369=CARTESIAN_POINT ( 'NONE',  ( -78.66644367742111399, 23.39876645725285798, 18.57365054920947500 ) ) ;
#30371=AXIS2_PLACEMENT_3D ( 'NONE', #28987, #45143, #44088 ) ;
#30372=CARTESIAN_POINT ( 'NONE',  ( 9.058156535714477542, 6.378495712187264743, 7.351094015256990133 ) ) ;
#30376=CARTESIAN_POINT ( 'NONE',  ( -177.5271152834790769, 92.16916858125013334, -36.12493601448592528 ) ) ;
#30377=CARTESIAN_POINT ( 'NONE',  ( 90.91465859190766707, 20.92790537681857188, -22.63697861787248655 ) ) ;
#30378=DIRECTION ( 'NONE',  ( 0.000000000000000000, 0.000000000000000000, 1.000000000000000000 ) ) ;
#30380=CARTESIAN_POINT ( 'NONE',  ( -54.08504625707234226, 14.42374043447187226, 72.11508717042879368 ) ) ;
#30381=CARTESIAN_POINT ( 'NONE',  ( -0.3249717932738297455, 6.518578686837482650, 64.94829995873614337 ) ) ;
#30385=DIRECTION ( 'NONE',  ( 0.000000000000000000, 0.000000000000000000, 1.000000000000000000 ) ) ;
#30386=CYLINDRICAL_SURFACE ( 'NONE', #44199, 7.500000000000013323 ) ;
#30389=CARTESIAN_POINT ( 'NONE',  ( -1.298947065946361112, 7.560777410219321482, 94.99999999999866418 ) ) ;
#30396=CARTESIAN_POINT ( 'NONE',  ( -7.825402957745085430, 6.891034867348153625, -89.10717191287116634 ) ) ;
#30397=CARTESIAN_POINT ( 'NONE',  ( -173.9548930713590948, 88.06040582145362805, -76.52175617720489242 ) ) ;
#30404=CARTESIAN_POINT ( 'NONE',  ( 60.40531521312255592, 13.11276739283242243, -50.25594387449618949 ) ) ;
#30405=CARTESIAN_POINT ( 'NONE',  ( -84.55783695959762269, 25.74181993349145259, 42.58591016297526721 ) ) ;
#30406=CARTESIAN_POINT ( 'NONE',  ( -29.50439180771547143, 10.29976981300626981, -23.23516915157700069 ) ) ;
#30407=CARTESIAN_POINT ( 'NONE',  ( 135.6842057900327063, 42.53841116629840258, 17.45434489297113956 ) ) ;
#30413=CARTESIAN_POINT ( 'NONE',  ( 11.21653854975268771, 6.397128675385707730, 70.32495166433241707 ) ) ;
#30418=CYLINDRICAL_SURFACE ( 'NONE', #57753, 7.500000000000020428 ) ;
#30423=B_SPLINE_CURVE_WITH_KNOTS ( 'NONE', 3,
 ( #42109, #58618, #53334, #10433, #48388, #5165, #10099, #21681, #64253, #52992, #21337, #37867, #32592, #41768, #4813, #37514, #37171, #15379, #20648, #224, #5845, #15033, #53687, #47370, #31554, #69177, #68825, #36491, #42784, #31903, #63567, #43130, #31224, #63908, #57942, #59315, #26961, #42451, #26627, #9762, #48062, #52655, #26281, #36839, #4480 ),
 .UNSPECIFIED., .F., .F.,
 ( 4, 2, 2, 2, 2, 2, 2, 2, 2, 2, 2, 1, 2, 2, 2, 2, 2, 2, 2, 2, 2, 2, 4 ),
 ( 1.430489624538199204E-17, 0.001502898956853375738, 0.002254348435280052656, 0.003005797913706729791, 0.004508696870560122659, 0.005260146348986836223, 0.006011595827413550655, 0.007514494784266991662, 0.009017393741120432668, 0.01052029269797387367, 0.01127174217640060198, 0.01202319165482733029, 0.01277464113325405687, 0.01352609061168078171, 0.01502898956853423486, 0.01578043904696096317, 0.01653188852538768974, 0.01803478748224114289, 0.01953768643909459257, 0.02028913591752131915, 0.02104058539594804572, 0.02254348435280153704, 0.02404638330965502488 ),
 .UNSPECIFIED. ) ;
#30424=CARTESIAN_POINT ( 'NONE',  ( -147.3614567344829140, 62.37986555269946365, 72.26553695328843219 ) ) ;
#30426=CARTESIAN_POINT ( 'NONE',  ( 198.3926538463959162, 98.07933330386025261, -66.56970357492031098 ) ) ;
#30427=CARTESIAN_POINT ( 'NONE',  ( 188.4937788906149763, 86.43336847120866651, -15.68169198850661417 ) ) ;
#30428=DIRECTION ( 'NONE',  ( 0.000000000000000000, 0.000000000000000000, 1.000000000000000000 ) ) ;
#30431=CARTESIAN_POINT ( 'NONE',  ( -48.70883077256304006, 14.10659259062419046, 33.80919071426065869 ) ) ;
#30432=ORIENTED_EDGE ( 'NONE', *, *, #17637, .T. ) ;
#30433=ORIENTED_EDGE ( 'NONE', *, *, #52765, .F. ) ;
#30434=EDGE_CURVE ( 'NONE', #33041, #4538, #19732, .T. ) ;
#30435=CARTESIAN_POINT ( 'NONE',  ( -108.0902552660050588, 36.97681740369922920, 6.405841544879333327 ) ) ;
#30436=CARTESIAN_POINT ( 'NONE',  ( 109.3047266816501093, 28.44977739115299187, 56.49988189436563601 ) ) ;
#30437=CARTESIAN_POINT ( 'NONE',  ( 102.7610798044536438, 25.57191189614546190, 91.42850727331421012 ) ) ;
#30438=CYLINDRICAL_SURFACE ( 'NONE', #3781, 7.500000000000013323 ) ;
#30443=CARTESIAN_POINT ( 'NONE',  ( -144.0382967194035473, 60.96512050924604864, 86.73872642800570532 ) ) ;
#30449=CARTESIAN_POINT ( 'NONE',  ( 67.92995549349548412, 13.86623459444478534, -48.90726067449875103 ) ) ;
#30452=VECTOR ( 'NONE', #12448, 1000.000000000000000 ) ;
#30453=CARTESIAN_POINT ( 'NONE',  ( -38.69449158134470679, 11.92067517118075237, -71.62430901259223504 ) ) ;
#30454=CARTESIAN_POINT ( 'NONE',  ( 31.96227686234408338, 7.558148489540042370, 63.27730136333553901 ) ) ;
#30455=CARTESIAN_POINT ( 'NONE',  ( 15.29899606819416569, 6.485153354884285903, -23.67439350822213839 ) ) ;
#30457=EDGE_LOOP ( 'NONE', ( #64606, #50999 ) ) ;
#30461=CARTESIAN_POINT ( 'NONE',  ( 66.08620257826612487, 13.40585338179126751, -63.21833551195629752 ) ) ;
#30462=CARTESIAN_POINT ( 'NONE',  ( 16.76400266940279948, 6.533513613209219528, 56.90669568735162898 ) ) ;
#30463=CARTESIAN_POINT ( 'NONE',  ( 22.89270809252618477, 7.840160460323052583, -13.75834395622513462 ) ) ;
#30464=CARTESIAN_POINT ( 'NONE',  ( 8.287863202055541834, 7.382585476140733682, 11.15840143617041669 ) ) ;
#30473=CARTESIAN_POINT ( 'NONE',  ( 188.0103583326377645, 87.39896620268123684, -40.83424593798813618 ) ) ;
#30480=EDGE_CURVE ( 'NONE', #36510, #34701, #35919, .T. ) ;
#30481=CARTESIAN_POINT ( 'NONE',  ( 164.7662527831195973, 64.87053726845202561, 88.85073695511873382 ) ) ;
#30482=EDGE_LOOP ( 'NONE', ( #35492, #62858 ) ) ;
#30483=CARTESIAN_POINT ( 'NONE',  ( 133.8566784816069344, 42.60093787723652525, -77.86786152285937135 ) ) ;
#30484=CARTESIAN_POINT ( 'NONE',  ( 132.0582325211145189, 40.34869848118183455, 44.30557495754532482 ) ) ;
#30485=CARTESIAN_POINT ( 'NONE',  ( -156.8773151811562343, 72.06122063279306644, 39.64036288611060854 ) ) ;
#30486=CARTESIAN_POINT ( 'NONE',  ( -95.21430597939259144, 29.33390900154322267, 35.45363162692691361 ) ) ;
#30487=DIRECTION ( 'NONE',  ( -0.8118923937861950435, -0.5838071093367415143, 0.000000000000000000 ) ) ;
#30495=CARTESIAN_POINT ( 'NONE',  ( 177.0027897064244371, 75.97676392242540544, 43.11708354611123895 ) ) ;
#30497=EDGE_CURVE ( 'NONE', #4217, #62345, #23365, .T. ) ;
#30498=CARTESIAN_POINT ( 'NONE',  ( 15.78827728214693416, -170.0000000000000000, -43.01894409868580027 ) ) ;
#30499=EDGE_LOOP ( 'NONE', ( #64703, #52601 ) ) ;
#30501=VECTOR ( 'NONE', #20085, 1000.000000000000000 ) ;
#30504=AXIS2_PLACEMENT_3D ( 'NONE', #35777, #56524, #30487 ) ;
#30505=CARTESIAN_POINT ( 'NONE',  ( -61.86845765289631061, 16.61548683002699889, -19.01154453034531500 ) ) ;
#30507=CARTESIAN_POINT ( 'NONE',  ( 135.6793972494603224, 43.71805072851431362, 29.72064904164495758 ) ) ;
#30508=CARTESIAN_POINT ( 'NONE',  ( 117.6853163455684665, 33.60747889659833021, 38.17223689839699574 ) ) ;
#30509=CARTESIAN_POINT ( 'NONE',  ( -132.6092625803567557, 52.31125232006264270, 14.62512562566566565 ) ) ;
#30510=CARTESIAN_POINT ( 'NONE',  ( 64.93224207568368911, 14.16036304753835218, -62.81019525340659726 ) ) ;
#30512=ORIENTED_EDGE ( 'NONE', *, *, #44296, .F. ) ;
#30514=CARTESIAN_POINT ( 'NONE',  ( 12.52293991431295872, 7.423284696525648485, -89.90348070406828640 ) ) ;
#30516=CARTESIAN_POINT ( 'NONE',  ( -172.7154982671752350, 86.67743928531949393, -49.71195716475002513 ) ) ;
#30519=EDGE_CURVE ( 'NONE', #31875, #62112, #36951, .T. ) ;
#30520=CARTESIAN_POINT ( 'NONE',  ( -53.98930025855998593, 14.39893220427481069, -88.97817567444977271 ) ) ;
#30524=CARTESIAN_POINT ( 'NONE',  ( 69.83617901654355364, 15.39919709983074547, -46.34986266313208603 ) ) ;
#30526=CARTESIAN_POINT ( 'NONE',  ( -165.9111709580270428, 79.44576090485631426, -66.96989664920324969 ) ) ;
#30528=CARTESIAN_POINT ( 'NONE',  ( -102.7494334820056849, 34.14986869751098908, 45.51907450641513009 ) ) ;
#30531=CARTESIAN_POINT ( 'NONE',  ( 85.67165909753197184, 20.15791549876376010, 71.51084241816450060 ) ) ;
#30533=CARTESIAN_POINT ( 'NONE',  ( -80.76833728594722572, 23.13302944128081151, -89.09247661525495232 ) ) ;
#30537=CARTESIAN_POINT ( 'NONE',  ( 31.91375106836930087, 7.553354707452900385, 10.08129055534168117 ) ) ;
#30538=CARTESIAN_POINT ( 'NONE',  ( -15.13464256769235838, 8.488509377255649468, -41.21959027930886066 ) ) ;
#30542=ORIENTED_EDGE ( 'NONE', *, *, #53551, .F. ) ;
#30543=CARTESIAN_POINT ( 'NONE',  ( -57.43251939610646417, 15.33203492375496957, 30.68838339410472926 ) ) ;
#30544=CARTESIAN_POINT ( 'NONE',  ( -56.97556689808916275, 16.24958672959845174, 71.91524354625708781 ) ) ;
#30545=CARTESIAN_POINT ( 'NONE',  ( -23.95096213915837069, 8.481591526885942756, 11.36064944404291843 ) ) ;
#30547=CARTESIAN_POINT ( 'NONE',  ( -60.99549137429562506, 16.35576463946026493, -91.82486495769101964 ) ) ;
#30549=CARTESIAN_POINT ( 'NONE',  ( 151.3136733342016953, 54.26417151662140270, -39.33353844295554325 ) ) ;
#30551=ORIENTED_EDGE ( 'NONE', *, *, #43748, .T. ) ;
#30554=FACE_OUTER_BOUND ( 'NONE', #46917, .T. ) ;
#30557=CARTESIAN_POINT ( 'NONE',  ( -124.1094910780272471, 45.33021696310841975, 30.83172109347568579 ) ) ;
#30558=CARTESIAN_POINT ( 'NONE',  ( -55.53469534616545644, 14.81076603075803710, -50.21632399845988459 ) ) ;
#30560=CARTESIAN_POINT ( 'NONE',  ( -180.4614954900547730, 97.28277348252827039, -70.62524901975936586 ) ) ;
#30562=CARTESIAN_POINT ( 'NONE',  ( 126.5464880001513137, 38.33492781348540746, 92.41540379265920535 ) ) ;
#30564=CARTESIAN_POINT ( 'NONE',  ( 115.7561705820728974, 31.51689401996057072, 32.00340604943662015 ) ) ;
#30566=CARTESIAN_POINT ( 'NONE',  ( -125.8938041572051389, -170.0000000000000000, -61.75825448869760237 ) ) ;
#30571=VERTEX_POINT ( 'NONE', #6314 ) ;
#30573=CARTESIAN_POINT ( 'NONE',  ( 117.7411475730015553, 32.50808475802732289, -70.80961951247346065 ) ) ;
#30574=CARTESIAN_POINT ( 'NONE',  ( 187.0788993276711949, 86.37277723143235164, 32.29480605614903510 ) ) ;
#30575=CARTESIAN_POINT ( 'NONE',  ( 140.2058232509808988, 46.59155168125934665, 14.18931278570159016 ) ) ;
#30580=DIRECTION ( 'NONE',  ( -0.8160245890732938934, -0.5780171883497599028, 0.000000000000000000 ) ) ;
#30581=VERTEX_POINT ( 'NONE', #66135 ) ;
#30583=CARTESIAN_POINT ( 'NONE',  ( 141.1678131691836029, 46.01782037724119334, 89.01741585174310956 ) ) ;
#30588=CARTESIAN_POINT ( 'NONE',  ( -178.5790738944854184, 93.41591512785082330, 43.47135350925507424 ) ) ;
#30592=ORIENTED_EDGE ( 'NONE', *, *, #59225, .T. ) ;
#30594=CARTESIAN_POINT ( 'NONE',  ( -102.2801239173131194, -170.0000000000000000, -88.70367844590326456 ) ) ;
#30595=CARTESIAN_POINT ( 'NONE',  ( 156.0367587612848013, 57.81183863259477818, -89.91473147631771212 ) ) ;
#30597=CARTESIAN_POINT ( 'NONE',  ( -178.2961695431413034, 94.64580896714811331, -90.45313625092560983 ) ) ;
#30598=CARTESIAN_POINT ( 'NONE',  ( 150.2076397309211870, 52.21780102759851871, 61.86243719087420345 ) ) ;
#30599=CARTESIAN_POINT ( 'NONE',  ( 94.14197848494937659, 23.19876128416614947, 37.22230832254705746 ) ) ;
#30603=EDGE_LOOP ( 'NONE', ( #16923, #18250, #16963, #30433 ) ) ;
#30605=CARTESIAN_POINT ( 'NONE',  ( 150.2060369882285613, 53.45752899907543565, -14.89401360268165497 ) ) ;
#30606=CARTESIAN_POINT ( 'NONE',  ( -52.58932868456671628, 14.03406530728571866, 84.39402770761704176 ) ) ;
#30607=CARTESIAN_POINT ( 'NONE',  ( 107.9342863085848165, 28.93180871323605174, 29.95979435419317127 ) ) ;
#30609=B_SPLINE_CURVE_WITH_KNOTS ( 'NONE', 3,
 ( #39669, #34752, #56188, #61124, #39327, #40360, #8004, #34412, #40698, #50919, #2733, #12594, #30166, #45986, #45643, #61808, #7322, #35085, #56537, #29813, #51275, #3087, #19244, #51615, #24884, #46321, #60769, #19596, #14331, #57587, #25236, #30854, #4798, #3766, #69159, #58261, #5144, #41746, #52971, #20287, #15361, #62863, #9395, #15701, #42433, #9742, #46674, #68808, #26263, #52300, #20981, #63207, #68149, #10079, #31539, #19957 ),
 .UNSPECIFIED., .F., .F.,
 ( 4, 2, 2, 2, 2, 2, 2, 2, 2, 2, 2, 2, 2, 2, 2, 2, 2, 2, 2, 2, 2, 2, 2, 2, 2, 2, 2, 4 ),
 ( 0.000000000000000000, 0.001986474333293954727, 0.002979711499940947920, 0.003972948666587941546, 0.004966185833234934739, 0.005959422999881927932, 0.006952660166528921125, 0.007945897333175914318, 0.008939134499822908378, 0.009932371666469900703, 0.01092560883311689303, 0.01191884599976388709, 0.01390532033305785092, 0.01489855749970483111, 0.01589179466635181129, 0.01688503183299879321, 0.01787826899964577165, 0.01986474333293978059, 0.02085798049958679373, 0.02185121766623380687, 0.02383769199952784357, 0.02582416633282188720, 0.02681740349946890381, 0.02781064066611592736, 0.02880387783276294397, 0.02979711499940996405, 0.03079035216605698413, 0.03178358933270400422 ),
 .UNSPECIFIED. ) ;
#30611=CARTESIAN_POINT ( 'NONE',  ( 55.59854697352604092, 11.07381680267640611, 89.83930078720294432 ) ) ;
#30613=CARTESIAN_POINT ( 'NONE',  ( 187.5165082312810227, 86.85340440641664372, 6.098473246464705788 ) ) ;
#30616=FACE_OUTER_BOUND ( 'NONE', #27305, .T. ) ;
#30621=B_SPLINE_CURVE_WITH_KNOTS ( 'NONE', 3,
 ( #58177, #57151, #9995, #31448, #19862, #41317, #47603, #41656, #42000, #69419, #14577, #9651, #57836, #30763, #31114, #69058, #42347, #63806, #15614, #58506, #823, #38807, #49331, #58855, #44058, #27896, #22271, #54615, #38094, #26856, #48282, #43367, #1163, #1509, #43706, #65539, #22974, #22618, #44418, #16638 ),
 .UNSPECIFIED., .F., .F.,
 ( 4, 2, 2, 2, 2, 2, 2, 2, 2, 2, 2, 2, 2, 2, 2, 2, 2, 2, 2, 4 ),
 ( 0.02472759712254455483, 0.02626001169882808198, 0.02779242627511161259, 0.02932484085139513974, 0.03009104813953689117, 0.03085725542767864260, 0.03238967000396211771, 0.03315587729210385526, 0.03392208458024560669, 0.03545449915652906792, 0.03698691373281254302, 0.03851932830909601813, 0.04005174288537948629, 0.04158415746166295446, 0.04311657203794642956, 0.04464898661422990467, 0.04541519390237164222, 0.04618140119051337977, 0.04771381576679688263, 0.04924623034308039243 ),
 .UNSPECIFIED. ) ;
#30622=CARTESIAN_POINT ( 'NONE',  ( 56.19513604272052731, 11.19349063094192864, -66.93610801037368674 ) ) ;
#30625=CARTESIAN_POINT ( 'NONE',  ( -12.88104669460377139, 7.273094923955126134, 85.75516146200649814 ) ) ;
#30627=CARTESIAN_POINT ( 'NONE',  ( -102.7447593990059147, 34.14748189312174276, -23.17002667451225761 ) ) ;
#30629=CARTESIAN_POINT ( 'NONE',  ( -75.64857587248467041, 21.19501514561449085, 71.63294696157397823 ) ) ;
#30630=CARTESIAN_POINT ( 'NONE',  ( 204.3728460619837222, 105.8991018586015684, -90.01503221354896311 ) ) ;
#30633=CARTESIAN_POINT ( 'NONE',  ( -157.0077369422017739, 70.81157624963286423, 37.93971990965763297 ) ) ;
#30640=EDGE_LOOP ( 'NONE', ( #6593, #66980, #64949, #8337 ) ) ;
#30641=CARTESIAN_POINT ( 'NONE',  ( 20.36233635256088448, 7.697399815318435756, -48.98271903251053772 ) ) ;
#30642=CARTESIAN_POINT ( 'NONE',  ( -146.7404675333698094, 63.17262273741976486, 45.19530540836205290 ) ) ;
#30643=CARTESIAN_POINT ( 'NONE',  ( 210.0292194063022180, 113.9511645670926470, 41.98791776798442754 ) ) ;
#30644=FACE_BOUND ( 'NONE', #38164, .T. ) ;
#30646=EDGE_CURVE ( 'NONE', #53693, #5113, #7018, .T. ) ;
#30648=VERTEX_POINT ( 'NONE', #1390 ) ;
#30649=CARTESIAN_POINT ( 'NONE',  ( -31.43908319763710679, -170.0000000000000000, 3.371903815725488585 ) ) ;
#30650=CARTESIAN_POINT ( 'NONE',  ( -126.2499057435234846, 47.93568886205795110, 84.31219562368272591 ) ) ;
#30652=CARTESIAN_POINT ( 'NONE',  ( -167.9889421625799457, 81.59140042431234008, -20.85682559493721655 ) ) ;
#30653=CARTESIAN_POINT ( 'NONE',  ( -149.5074843970971301, -170.0000000000000000, -61.65738112195564469 ) ) ;
#30654=CARTESIAN_POINT ( 'NONE',  ( 8.389070543067937535, 6.376531511354393444, 89.93455881902842464 ) ) ;
#30655=CARTESIAN_POINT ( 'NONE',  ( 80.73012746365746750, 17.49169339352361519, -65.50839743993871878 ) ) ;
#30659=CARTESIAN_POINT ( 'NONE',  ( -95.63568360745009045, 29.53168204475777259, 61.37563518862691581 ) ) ;
#30669=EDGE_LOOP ( 'NONE', ( #51480, #10071, #48165, #63699 ) ) ;
#30670=CARTESIAN_POINT ( 'NONE',  ( 13.14401442664830988, 6.430459733718341120, -35.99624556455200519 ) ) ;
#30674=B_SPLINE_CURVE_WITH_KNOTS ( 'NONE', 3,
 ( #13104, #8519, #35240, #29968, #51766, #35593, #34570, #8865, #2892, #67955, #7823, #46479, #51429, #66927, #62315, #67604, #40173, #30315, #3241, #56012, #56344, #28935, #25044, #13444, #2541, #34210, #45797, #3572, #34906, #19060, #40514, #23652, #19755, #50720, #61961, #7484, #14134, #29273, #50387, #19403, #41214, #45444, #18369, #12750, #55651, #42591, #20433, #57388, #62674, #36280 ),
 .UNSPECIFIED., .F., .F.,
 ( 4, 2, 2, 2, 2, 2, 2, 2, 2, 2, 2, 2, 2, 2, 2, 2, 2, 2, 2, 2, 2, 2, 2, 2, 4 ),
 ( 0.03296461860586801657, 0.03492857779726586676, 0.03689253698866371695, 0.03885649618006156714, 0.04082045537145942427, 0.04278441456285727446, 0.04376639415855620302, 0.04474837375425513852, 0.04573035334995407403, 0.04671233294565300259, 0.04720332274350246687, 0.04769431254135193810, 0.04867629213705086666, 0.04965827173274980216, 0.05064025132844873767, 0.05162223092414766623, 0.05260421051984659480, 0.05358619011554553030, 0.05456816971124446580, 0.05555014930694339437, 0.05653212890264232987, 0.05849608809404027721, 0.06046004728543821760, 0.06242400647683615800, 0.06438796566823409839 ),
 .UNSPECIFIED. ) ;
#30675=CARTESIAN_POINT ( 'NONE',  ( -38.56832981558923024, 10.87072789871799117, 93.82338543633802885 ) ) ;
#30676=CARTESIAN_POINT ( 'NONE',  ( 175.0634607207819045, 74.11351956991637735, -66.08984933419260699 ) ) ;
#30680=CYLINDRICAL_SURFACE ( 'NONE', #47856, 7.500000000000020428 ) ;
#30682=EDGE_LOOP ( 'NONE', ( #15936, #12284 ) ) ;
#30684=CARTESIAN_POINT ( 'NONE',  ( -85.75002235020440366, 26.23806300442548078, -66.98273671324270140 ) ) ;
#30685=CARTESIAN_POINT ( 'NONE',  ( 173.7225111622555005, 72.84868911716898765, 11.42765638463486333 ) ) ;
#30688=CARTESIAN_POINT ( 'NONE',  ( 133.3996297101684263, 41.14871796345731525, 17.66579024853170310 ) ) ;
#30689=CARTESIAN_POINT ( 'NONE',  ( -156.1462053606562677, 70.02140399657014314, 14.87619319211899516 ) ) ;
#30690=CARTESIAN_POINT ( 'NONE',  ( -118.8691191306315318, 43.21907118237575673, -66.61757324505178701 ) ) ;
#30691=CARTESIAN_POINT ( 'NONE',  ( 212.1488570093002011, 119.0116247937291689, 35.83619200126886994 ) ) ;
#30693=CARTESIAN_POINT ( 'NONE',  ( -109.7816385129979295, 36.75776661907239173, 37.51838681235415152 ) ) ;
#30697=CARTESIAN_POINT ( 'NONE',  ( -47.54597338633182346, 13.82996226214091173, 91.56377290884543640 ) ) ;
#30701=CARTESIAN_POINT ( 'NONE',  ( 63.01563776193090405, 13.70579113808096672, -89.40979201309708913 ) ) ;
#30704=DIRECTION ( 'NONE',  ( -0.000000000000000000, 0.000000000000000000, -1.000000000000000000 ) ) ;
#30705=DIRECTION ( 'NONE',  ( 0.000000000000000000, 0.000000000000000000, 1.000000000000000000 ) ) ;
#30706=CARTESIAN_POINT ( 'NONE',  ( 140.5958192060901695, 46.84598876498523623, -46.82504131882815557 ) ) ;
#30707=CARTESIAN_POINT ( 'NONE',  ( 36.99625334683020839, 8.108440754877198842, -50.24044060793853816 ) ) ;
#30710=CARTESIAN_POINT ( 'NONE',  ( 10.31616749326173554, 7.393414706728904662, -48.15370678270306826 ) ) ;
#30711=CARTESIAN_POINT ( 'NONE',  ( 127.6144785300460143, 37.78099129859914740, -47.68851779290559278 ) ) ;
#30724=ORIENTED_EDGE ( 'NONE', *, *, #58272, .T. ) ;
#30725=FACE_OUTER_BOUND ( 'NONE', #758, .T. ) ;
#30726=CARTESIAN_POINT ( 'NONE',  ( 174.1251613516843975, 71.84747073139212148, -67.71850567866349024 ) ) ;
#30729=CARTESIAN_POINT ( 'NONE',  ( -30.46358361599563835, 10.45190018822943578, 72.01312986667528548 ) ) ;
#30731=CARTESIAN_POINT ( 'NONE',  ( -51.77439426130688105, 13.82695438436702418, 71.41181520050716358 ) ) ;
#30736=EDGE_CURVE ( 'NONE', #33732, #27549, #11615, .T. ) ;
#30737=CARTESIAN_POINT ( 'NONE',  ( -173.1211646369891355, -170.0000000000000000, 3.977144016177345254 ) ) ;
#30738=CARTESIAN_POINT ( 'NONE',  ( -107.2385267828037172, 36.51474259889399576, -74.99142853021918143 ) ) ;
#30740=FACE_OUTER_BOUND ( 'NONE', #57159, .T. ) ;
#30746=VERTEX_POINT ( 'NONE', #67503 ) ;
#30750=CARTESIAN_POINT ( 'NONE',  ( 140.7279459667387869, 46.93224938917404643, -94.17646906148590347 ) ) ;
#30752=ORIENTED_EDGE ( 'NONE', *, *, #60527, .F. ) ;
#30756=CARTESIAN_POINT ( 'NONE',  ( 57.09527843067915143, 12.40436368789086963, -47.83156069688324408 ) ) ;
#30757=CARTESIAN_POINT ( 'NONE',  ( -83.51110947562234799, 25.31252704029287415, 32.18774550040605931 ) ) ;
#30758=CARTESIAN_POINT ( 'NONE',  ( -24.32776401346968598, 9.546905915310565760, -13.53957171349472510 ) ) ;
#30759=CARTESIAN_POINT ( 'NONE',  ( 141.0804878838241336, 45.96076546397619467, 12.25136187784951325 ) ) ;
#30763=CARTESIAN_POINT ( 'NONE',  ( 103.9685899589048432, 27.18106603025993095, -20.69423234284586499 ) ) ;
#30765=CARTESIAN_POINT ( 'NONE',  ( 14.08699529666005823, 6.452200550165255954, 71.66783672710508313 ) ) ;
#30766=CARTESIAN_POINT ( 'NONE',  ( -23.98747857548120876, 9.501432345103353327, 38.70170266760086264 ) ) ;
#30768=CARTESIAN_POINT ( 'NONE',  ( -125.8938041572051389, -170.0000000000000000, 45.61994787315711619 ) ) ;
#30771=CARTESIAN_POINT ( 'NONE',  ( 70.50376765786469946, 15.57629333413342820, 36.82268012421604197 ) ) ;
#30772=ORIENTED_EDGE ( 'NONE', *, *, #11506, .T. ) ;
#30779=CARTESIAN_POINT ( 'NONE',  ( -118.6849742182705256, 41.92701402439731595, 67.05091989562900778 ) ) ;
#30782=CARTESIAN_POINT ( 'NONE',  ( -52.67596829228261868, 15.09584868440940042, 30.68732742033287053 ) ) ;
#30785=B_SPLINE_CURVE_WITH_KNOTS ( 'NONE', 3,
 ( #43658, #48234, #16591, #22220, #410, #5680, #64432, #63756, #53521, #20834, #37020, #6025, #31733, #65137, #38047, #32774, #32084, #27487, #16931, #27141, #21519, #53168, #43309, #21865, #42963, #53861, #54202, #11653, #16243, #5001, #48926, #15565, #37695, #26465, #54563, #47902, #767, #59492, #21186, #58457, #6389, #27842, #58798, #5352 ),
 .UNSPECIFIED., .F., .F.,
 ( 4, 2, 2, 2, 2, 2, 2, 2, 2, 2, 2, 2, 2, 2, 2, 2, 2, 2, 2, 2, 2, 4 ),
 ( 0.000000000000000000, 0.001488594467279756757, 0.002232891700919623860, 0.002977188934559490963, 0.004465783401839205219, 0.005954377869118920343, 0.007442972336398633731, 0.008187269570038497798, 0.008931566803678360131, 0.01042016127095808480, 0.01190875573823781293, 0.01265305297187767700, 0.01339735020551753759, 0.01488594467279726052, 0.01563024190643714020, 0.01637453914007701988, 0.01786313360735677577, 0.01935172807463653513, 0.02009602530827639746, 0.02084032254191625633, 0.02232891700919594630, 0.02381751147647563280 ),
 .UNSPECIFIED. ) ;
#30786=CARTESIAN_POINT ( 'NONE',  ( -102.7494334820056139, 34.14986869751099618, 18.67452391595144334 ) ) ;
#30787=CARTESIAN_POINT ( 'NONE',  ( -83.69370847062543817, 25.38703975185372386, -48.18640663508916333 ) ) ;
#30788=CARTESIAN_POINT ( 'NONE',  ( 115.7655322686204755, 31.52170665051862031, 85.71478802353045978 ) ) ;
#30793=CARTESIAN_POINT ( 'NONE',  ( 164.8471526211111495, 63.62172173173267709, -69.08682052283407415 ) ) ;
#30798=CARTESIAN_POINT ( 'NONE',  ( -149.7268278745401631, 65.68859631971237434, -22.96827994102830317 ) ) ;
#30800=CARTESIAN_POINT ( 'NONE',  ( 68.63487067129265995, 14.04635751989139614, -38.22936938732106427 ) ) ;
#30806=CARTESIAN_POINT ( 'NONE',  ( 31.99894129856762603, 7.561773404408284271, 63.03122815760148256 ) ) ;
#30807=CARTESIAN_POINT ( 'NONE',  ( 45.98350631452262149, 9.356976075258891967, 94.71468413938886499 ) ) ;
#30809=CARTESIAN_POINT ( 'NONE',  ( 20.74561700410411191, 7.717362891868937425, 16.31941674212566795 ) ) ;
#30811=CARTESIAN_POINT ( 'NONE',  ( -119.2982054035570769, 42.30181775808005540, 7.695783488898820579 ) ) ;
#30812=CARTESIAN_POINT ( 'NONE',  ( -133.3122825023497171, 51.57669324886579432, -95.00000000000133582 ) ) ;
#30813=AXIS2_PLACEMENT_3D ( 'NONE', #60894, #55977, #13750 ) ;
#30814=CARTESIAN_POINT ( 'NONE',  ( 126.4754729582248132, 37.14269484129875565, -15.32358833706418011 ) ) ;
#30815=CARTESIAN_POINT ( 'NONE',  ( 20.36233635256087382, 7.697399815318433980, -22.13816844204684386 ) ) ;
#30816=CARTESIAN_POINT ( 'NONE',  ( 198.7084915431530305, 98.47675983942191635, 59.03003622776400761 ) ) ;
#30818=EDGE_CURVE ( 'NONE', #13481, #45287, #17246, .T. ) ;
#30819=VECTOR ( 'NONE', #53732, 1000.000000000000000 ) ;
#30824=CARTESIAN_POINT ( 'NONE',  ( 128.4157044224114088, 39.39296260757095069, -48.70813808969364089 ) ) ;
#30825=CARTESIAN_POINT ( 'NONE',  ( -130.1964689553233256, 49.39217932424205060, -36.25302896202752834 ) ) ;
#30826=CARTESIAN_POINT ( 'NONE',  ( -108.6944271866238978, 37.30738480893074893, -38.59587447743199817 ) ) ;
#30827=CARTESIAN_POINT ( 'NONE',  ( 188.4918087359957042, 87.93403732562659059, -44.93618865354876135 ) ) ;
#30829=ORIENTED_EDGE ( 'NONE', *, *, #25831, .F. ) ;
#30830=CARTESIAN_POINT ( 'NONE',  ( -26.50364027666003253, 8.832969329054188634, -21.64101123914544900 ) ) ;
#30836=CARTESIAN_POINT ( 'NONE',  ( -61.53550548562876088, 17.56596194025584978, 14.77635692923447053 ) ) ;
#30837=CARTESIAN_POINT ( 'NONE',  ( 133.8566784816069628, 41.42467568809806977, 44.51034083899536142 ) ) ;
#30838=CARTESIAN_POINT ( 'NONE',  ( -190.6985136298601731, 109.1272424661242582, 94.99999999999866418 ) ) ;
#30839=EDGE_CURVE ( 'NONE', #68152, #6290, #48466, .T. ) ;
#30841=CARTESIAN_POINT ( 'NONE',  ( -94.79534239005252516, 29.13842790650043568, 37.47587493899962396 ) ) ;
#30848=CARTESIAN_POINT ( 'NONE',  ( -125.0023254877051784, 45.90912477771775002, -23.02977023342388918 ) ) ;
#30851=CARTESIAN_POINT ( 'NONE',  ( -178.7483298110140311, 93.61800926271534706, -20.33199145141687225 ) ) ;
#30852=CARTESIAN_POINT ( 'NONE',  ( -129.3970594949620363, 50.06339481638102029, 58.31657860348069988 ) ) ;
#30854=CARTESIAN_POINT ( 'NONE',  ( -103.5135803422113980, 34.54427913530279426, 84.30440530529723731 ) ) ;
#30857=VERTEX_POINT ( 'NONE', #25640 ) ;
#30858=CARTESIAN_POINT ( 'NONE',  ( -58.32860549785898741, 15.58423118879329827, -22.62294191281809930 ) ) ;
#30861=CARTESIAN_POINT ( 'NONE',  ( -133.3220917939969752, 52.82057604964898445, -68.18860869838340477 ) ) ;
#30862=CARTESIAN_POINT ( 'NONE',  ( 57.01498327362266139, 11.36040931982467406, -92.39178327290893833 ) ) ;
#30865=CARTESIAN_POINT ( 'NONE',  ( 68.63585058221467250, 15.08566240483131438, -75.05603185210503625 ) ) ;
#30866=ORIENTED_EDGE ( 'NONE', *, *, #28738, .F. ) ;
#30868=CARTESIAN_POINT ( 'NONE',  ( -142.0084862216822899, 59.34995487985342777, -14.88985590709667228 ) ) ;
#30869=CARTESIAN_POINT ( 'NONE',  ( -171.0758681675584683, 84.87997360100517596, -34.98379575707922129 ) ) ;
#30872=CARTESIAN_POINT ( 'NONE',  ( -74.20136529587827567, 21.74007521413448885, 43.94919298524185791 ) ) ;
#30875=CARTESIAN_POINT ( 'NONE',  ( -149.2910611247328063, 63.99625741915658494, 45.72082123989907387 ) ) ;
#30877=CARTESIAN_POINT ( 'NONE',  ( 209.6525588430077960, 113.3929734759396695, 57.91716753057085754 ) ) ;
#30882=CARTESIAN_POINT ( 'NONE',  ( -36.37663950036513683, 10.45389057208228678, 16.53845768755774870 ) ) ;
#30884=CARTESIAN_POINT ( 'NONE',  ( -84.05562056347102384, 24.44784460338496501, -91.07024174204663325 ) ) ;
#30887=CARTESIAN_POINT ( 'NONE',  ( 32.46582151331404020, 7.608418548522501546, 13.45366444727946487 ) ) ;
#30888=CARTESIAN_POINT ( 'NONE',  ( -14.84903512415885274, 8.461292896365067762, -40.27624087600150915 ) ) ;
#30889=CARTESIAN_POINT ( 'NONE',  ( -38.16652041892308489, 11.81761816422915778, -19.32439935686155152 ) ) ;
#30891=DIRECTION ( 'NONE',  ( -0.000000000000000000, 1.000000000000000000, -0.000000000000000000 ) ) ;
#30894=CARTESIAN_POINT ( 'NONE',  ( -190.4968431727839118, 108.8425311198515004, 7.400362157239960936 ) ) ;
#30895=EDGE_CURVE ( 'NONE', #32175, #2381, #39299, .T. ) ;
#30897=CARTESIAN_POINT ( 'NONE',  ( -8.811275908848681837, 6.956777180392053062, -77.21364321485079074 ) ) ;
#30900=CARTESIAN_POINT ( 'NONE',  ( 150.2060369882285897, 53.45752899907544986, -41.73856419314534349 ) ) ;
#30907=CARTESIAN_POINT ( 'NONE',  ( -156.6644740249450081, 71.86407434531899696, 62.80635761803053896 ) ) ;
#30909=CARTESIAN_POINT ( 'NONE',  ( -103.2164890789475464, 34.39030697009943793, 72.31974941879711594 ) ) ;
#30910=CARTESIAN_POINT ( 'NONE',  ( -102.2801239173131194, -170.0000000000000000, 64.86362509687882039 ) ) ;
#30911=EDGE_LOOP ( 'NONE', ( #8150, #6313 ) ) ;
#30913=CARTESIAN_POINT ( 'NONE',  ( -176.3763474213711504, 92.36993073950281996, -75.82728650921367830 ) ) ;
#30914=CARTESIAN_POINT ( 'NONE',  ( 93.86680996363766383, 22.01878169039501998, 66.03955257416123459 ) ) ;
#30916=CARTESIAN_POINT ( 'NONE',  ( 115.0692128464502701, 31.17922615202198955, 42.87276276046937085 ) ) ;
#30918=DIRECTION ( 'NONE',  ( -0.000000000000000000, 1.000000000000000000, -0.000000000000000000 ) ) ;
#30920=CARTESIAN_POINT ( 'NONE',  ( -118.5043919384112030, 41.81711884544880320, -67.94780606738419237 ) ) ;
#30923=CARTESIAN_POINT ( 'NONE',  ( 197.8572563162090319, 97.41072138832259952, 39.79780622203359997 ) ) ;
#30924=CARTESIAN_POINT ( 'NONE',  ( 116.6734749296698936, 31.97209464358270026, -66.37505032600662958 ) ) ;
#30928=EDGE_CURVE ( 'NONE', #52659, #42507, #32560, .T. ) ;
#30933=CARTESIAN_POINT ( 'NONE',  ( -107.7893514267588273, 35.66840175773127442, -47.62729620103424821 ) ) ;
#30934=CARTESIAN_POINT ( 'NONE',  ( 140.0012045870120687, 45.26048451937214878, 94.99999999999866418 ) ) ;
#30935=CARTESIAN_POINT ( 'NONE',  ( -62.30100056228378946, 16.74548393487070541, 39.80882454632615719 ) ) ;
#30938=CARTESIAN_POINT ( 'NONE',  ( -179.9014775667593540, 95.00669833041663992, 35.10404331463944061 ) ) ;
#30940=CARTESIAN_POINT ( 'NONE',  ( 117.7442255600442422, 33.63739995216995737, -43.92135388644469174 ) ) ;
#30946=CARTESIAN_POINT ( 'NONE',  ( 139.2921620648437226, 44.80435067172500396, 58.66407138463905824 ) ) ;
#30948=CARTESIAN_POINT ( 'NONE',  ( -33.13098007862450345, 9.875138601866732202, -62.35103961865778643 ) ) ;
#30949=CARTESIAN_POINT ( 'NONE',  ( 133.8566784816069060, 41.42467568809810530, -77.86786152285937135 ) ) ;
#30950=ORIENTED_EDGE ( 'NONE', *, *, #54068, .F. ) ;
#30951=CARTESIAN_POINT ( 'NONE',  ( 41.33434189587761409, 9.684413566891871383, 17.82021384918356688 ) ) ;
#30955=CARTESIAN_POINT ( 'NONE',  ( -62.55951243933055395, 16.82361985462172171, 91.56887453183679781 ) ) ;
#30958=CARTESIAN_POINT ( 'NONE',  ( 110.2429982417149574, 29.99119854320846201, 29.61121420573730489 ) ) ;
#30959=CARTESIAN_POINT ( 'NONE',  ( -0.3740447803642803493, 7.527031846085010969, 36.63165479535449975 ) ) ;
#30961=CARTESIAN_POINT ( 'NONE',  ( 187.8965227056808089, 87.27289477191501987, 13.11287507554345488 ) ) ;
#30964=CARTESIAN_POINT ( 'NONE',  ( 176.6258282025054882, 74.21441092921637050, 3.928463118842791424 ) ) ;
#30967=FACE_OUTER_BOUND ( 'NONE', #37616, .T. ) ;
#30969=ORIENTED_EDGE ( 'NONE', *, *, #27850, .F. ) ;
#30971=CARTESIAN_POINT ( 'NONE',  ( 60.62939143133407072, 12.13148391928981162, -77.19219116658004509 ) ) ;
#30974=CARTESIAN_POINT ( 'NONE',  ( 16.28382582968307091, 7.523443033994206885, 45.01470767270525641 ) ) ;
#30975=CARTESIAN_POINT ( 'NONE',  ( -105.8683518445188838, 35.77995342500075537, -22.27314921212501275 ) ) ;
#30979=EDGE_LOOP ( 'NONE', ( #2930, #17163 ) ) ;
#30984=CARTESIAN_POINT ( 'NONE',  ( 179.4207200232661705, 76.93724985992179199, -9.516548198904395406 ) ) ;
#30987=ADVANCED_FACE ( 'NONE', ( #18882 ), #41026, .F. ) ;
#30990=CARTESIAN_POINT ( 'NONE',  ( -133.0835080491125098, 52.64966140620843049, 35.96838589234516093 ) ) ;
#30992=CARTESIAN_POINT ( 'NONE',  ( 212.0180052085437694, 116.9552462415714871, 11.52689105391897861 ) ) ;
#30993=CARTESIAN_POINT ( 'NONE',  ( 10.15118267943872077, 7.391905976536033762, 59.40606955087935148 ) ) ;
#30994=CARTESIAN_POINT ( 'NONE',  ( 212.1707951106656935, 117.1901534358506041, 37.36565939486786192 ) ) ;
#31000=CARTESIAN_POINT ( 'NONE',  ( -120.6576327989070450, 44.32766273560634573, 86.43031013461866507 ) ) ;
#31002=CARTESIAN_POINT ( 'NONE',  ( 38.90907126433564400, 9.359889524363179447, -62.46436805589143404 ) ) ;
#31004=CARTESIAN_POINT ( 'NONE',  ( 22.25657943806483274, 6.793941046373902282, 94.99999999999866418 ) ) ;
#31006=CARTESIAN_POINT ( 'NONE',  ( 81.04675113612954362, 17.59091904316106181, -65.13359550991796709 ) ) ;
#31014=CARTESIAN_POINT ( 'NONE',  ( -96.02415295709708687, 29.71480036090584420, 60.71932897351158687 ) ) ;
#31016=CARTESIAN_POINT ( 'NONE',  ( -79.62258606008208517, 22.68765733708494281, 3.619629083515957468 ) ) ;
#31017=ORIENTED_EDGE ( 'NONE', *, *, #13490, .T. ) ;
#31018=B_SPLINE_CURVE_WITH_KNOTS ( 'NONE', 3,
 ( #26207, #30116, #24830, #9692, #47642, #62810, #9338, #57189, #51567, #9004, #14954, #20927, #42381, #51900, #52249, #31157, #63844, #36418 ),
 .UNSPECIFIED., .F., .F.,
 ( 4, 2, 2, 2, 2, 2, 2, 2, 4 ),
 ( 0.01023491291840469483, 0.01150387722361230318, 0.01277284152881991153, 0.01404180583402751814, 0.01531077013923512649, 0.01657973444444273484, 0.01784869874965034145, 0.01911766305485795153, 0.02038662736006555815 ),
 .UNSPECIFIED. ) ;
#31021=ORIENTED_EDGE ( 'NONE', *, *, #6828, .F. ) ;
#31023=CARTESIAN_POINT ( 'NONE',  ( 13.37366753069833791, 6.435102282077984626, -50.13664276337100034 ) ) ;
#31024=CARTESIAN_POINT ( 'NONE',  ( -177.5271152834791337, 92.16916858125016176, 71.25326634736879328 ) ) ;
#31025=CARTESIAN_POINT ( 'NONE',  ( 132.9440032680863055, 40.87616997986730638, 56.40712532407142987 ) ) ;
#31027=CARTESIAN_POINT ( 'NONE',  ( -38.85807996819452370, 10.92741605234837188, 92.55207049280542719 ) ) ;
#31028=CARTESIAN_POINT ( 'NONE',  ( 173.6700117628886915, 72.79957362875116189, -69.39913175793722644 ) ) ;
#31030=CARTESIAN_POINT ( 'NONE',  ( 109.7774723066848566, 28.66666416591279898, -50.92243756565371626 ) ) ;
#31033=ORIENTED_EDGE ( 'NONE', *, *, #21133, .T. ) ;
#31035=CARTESIAN_POINT ( 'NONE',  ( -84.53753601793928851, 25.73343139558517123, -74.15369040441258619 ) ) ;
#31036=CARTESIAN_POINT ( 'NONE',  ( 173.5836858989432017, 72.71885240881783830, 10.25081972939208441 ) ) ;
#31039=CARTESIAN_POINT ( 'NONE',  ( 128.0568017572569488, 38.03085713813913316, 5.383796554812978918 ) ) ;
#31040=CARTESIAN_POINT ( 'NONE',  ( 35.46869960875725525, 7.930278842742511713, -90.40974432087365642 ) ) ;
#31041=CARTESIAN_POINT ( 'NONE',  ( -122.1940143064357187, 45.29738883755585732, -62.73011510844082750 ) ) ;
#31043=CARTESIAN_POINT ( 'NONE',  ( 211.8382652195006699, 118.5282575235989952, 39.02422649141074373 ) ) ;
#31044=CARTESIAN_POINT ( 'NONE',  ( -82.33596576276350731, 24.83688096733768447, 71.32179102043865271 ) ) ;
#31045=CARTESIAN_POINT ( 'NONE',  ( -109.3553681454883844, 36.52260784104392854, 35.47894457937506019 ) ) ;
#31047=CIRCLE ( 'NONE', #23155, 243.4957430088094839 ) ;
#31050=CARTESIAN_POINT ( 'NONE',  ( -48.41612563322100016, 14.03642305406760471, 94.99999999999866418 ) ) ;
#31052=DIRECTION ( 'NONE',  ( -0.000000000000000000, 1.000000000000000000, -0.000000000000000000 ) ) ;
#31054=CARTESIAN_POINT ( 'NONE',  ( 17.72748965151693668, 7.577488030789625739, -62.61435461240134970 ) ) ;
#31056=CARTESIAN_POINT ( 'NONE',  ( -172.7173255566597163, 88.18461381371096763, 30.82169460664102800 ) ) ;
#31058=CARTESIAN_POINT ( 'NONE',  ( 134.7708899521911121, 43.15864772107692460, -50.97092526706858706 ) ) ;
#31060=CARTESIAN_POINT ( 'NONE',  ( -7.825402957745081878, 7.899365992529268965, 3.271030448983517580 ) ) ;
#31062=CARTESIAN_POINT ( 'NONE',  ( 212.1700216741374447, 117.1889356120871213, -71.39816962747791251 ) ) ;
#31066=VERTEX_POINT ( 'NONE', #56867 ) ;
#31068=B_SPLINE_CURVE_WITH_KNOTS ( 'NONE', 3,
 ( #45770, #29577, #35560, #18690, #46102, #30286, #45413, #3540, #50692, #45061, #3212, #35906, #46444, #2856, #19028, #34874, #67572, #13751, #13073, #39795, #19371, #40480, #57019, #67925, #35209, #61926, #61599, #8485, #40829, #41182, #66547, #57359, #56313, #9170, #29933, #51045, #8836, #51400, #61253, #2512, #25706, #46799, #26041, #26386, #64011, #4919 ),
 .UNSPECIFIED., .F., .F.,
 ( 4, 2, 2, 2, 2, 2, 2, 2, 2, 2, 2, 2, 2, 2, 2, 2, 2, 2, 2, 2, 2, 2, 4 ),
 ( 0.02989107162308291682, 0.03170280136394029724, 0.03351453110479767072, 0.03532626084565505115, 0.03713799058651242463, 0.03894972032736980505, 0.03985558519779850567, 0.04076145006822720629, 0.04166731493865591385, 0.04257317980908461447, 0.04347904467951332202, 0.04438490954994202264, 0.04529077442037073020, 0.04619663929079943776, 0.04710250416122813838, 0.04800836903165683900, 0.04891423390208554656, 0.04982009877251425412, 0.05163182851337159290, 0.05344355825422893169, 0.05525528799508627742, 0.05706701773594362315, 0.05887874747680096194 ),
 .UNSPECIFIED. ) ;
#31069=CARTESIAN_POINT ( 'NONE',  ( 173.5958500711059571, 72.73022245412229836, 91.08498831883019875 ) ) ;
#31072=CARTESIAN_POINT ( 'NONE',  ( -24.19091603582231542, 8.513464105188679909, -67.71881203971585705 ) ) ;
#31076=CARTESIAN_POINT ( 'NONE',  ( 15.78827728214693416, 6.500811158483284835, 3.170157082241545687 ) ) ;
#31080=CARTESIAN_POINT ( 'NONE',  ( -173.5394735271662512, 87.59446374803710000, -49.71195716474999671 ) ) ;
#31082=CARTESIAN_POINT ( 'NONE',  ( -173.1211646369891071, 87.12891641440859303, 18.97714401617737678 ) ) ;
#31083=CARTESIAN_POINT ( 'NONE',  ( 204.6977192012829789, 106.3443248447423599, -78.17048162308530834 ) ) ;
#31084=CARTESIAN_POINT ( 'NONE',  ( -52.66507163626135934, 14.05394608175175364, 71.78805517841820460 ) ) ;
#31085=ORIENTED_EDGE ( 'NONE', *, *, #51775, .T. ) ;
#31086=CARTESIAN_POINT ( 'NONE',  ( 130.7457207912710828, 40.74300766298682674, 3.325828997484891580 ) ) ;
#31088=CARTESIAN_POINT ( 'NONE',  ( -54.56685407443680447, 15.59259313022788085, 72.16187836339487660 ) ) ;
#31089=CYLINDRICAL_SURFACE ( 'NONE', #35473, 7.500000000000013323 ) ;
#31090=CARTESIAN_POINT ( 'NONE',  ( -53.14475157111024828, 14.17819596930906734, -49.97361403301091087 ) ) ;
#31092=DIRECTION ( 'NONE',  ( 0.000000000000000000, 0.000000000000000000, 1.000000000000000000 ) ) ;
#31096=CARTESIAN_POINT ( 'NONE',  ( -55.54058841405666413, 14.81234591756537711, 72.16187836339486239 ) ) ;
#31100=CARTESIAN_POINT ( 'NONE',  ( 31.91241427070456993, 8.564321958137947277, 91.88119559238364786 ) ) ;
#31103=ORIENTED_EDGE ( 'NONE', *, *, #41160, .F. ) ;
#31107=CARTESIAN_POINT ( 'NONE',  ( 33.44527180510250020, 7.709232309484722379, -20.85868167691871733 ) ) ;
#31108=CARTESIAN_POINT ( 'NONE',  ( 173.7225111622555005, 72.84868911716898765, -42.26144479629255102 ) ) ;
#31109=AXIS2_PLACEMENT_3D ( 'NONE', #63089, #62045, #31092 ) ;
#31111=CARTESIAN_POINT ( 'NONE',  ( 93.92280655489132357, 22.03989931749466535, 35.44608963825557169 ) ) ;
#31114=CARTESIAN_POINT ( 'NONE',  ( 103.8325688302027459, 27.12251147381400784, -20.47917175127302869 ) ) ;
#31116=CARTESIAN_POINT ( 'NONE',  ( 8.336882341125873452, 6.376438415325263342, 63.37576547410991878 ) ) ;
#31118=CARTESIAN_POINT ( 'NONE',  ( 197.2847860006354495, 98.30530166401516112, 35.55649062842450547 ) ) ;
#31119=CARTESIAN_POINT ( 'NONE',  ( -71.43567564266649583, 20.76245642981890427, 89.58950873541245130 ) ) ;
#31122=CARTESIAN_POINT ( 'NONE',  ( 157.4703587214989398, -170.0000000000000000, 63.75401806271707983 ) ) ;
#31124=EDGE_CURVE ( 'NONE', #17942, #66072, #56115, .T. ) ;
#31127=CARTESIAN_POINT ( 'NONE',  ( 116.6436511186860514, 33.08230081168870385, -66.34972720225196952 ) ) ;
#31130=CARTESIAN_POINT ( 'NONE',  ( 181.0840389613909736, 78.60582251573006829, 71.15314469597512925 ) ) ;
#31133=CARTESIAN_POINT ( 'NONE',  ( -86.15466590221103615, 26.40813842494317498, -15.27875085681931999 ) ) ;
#31134=CARTESIAN_POINT ( 'NONE',  ( 18.19980344696536889, 6.589834367837005047, -23.28036388989822925 ) ) ;
#31136=CARTESIAN_POINT ( 'NONE',  ( -152.5067928559255961, 66.76529500553621688, -49.20136729112984142 ) ) ;
#31141=EDGE_CURVE ( 'NONE', #26264, #26262, #20853, .T. ) ;
#31143=CARTESIAN_POINT ( 'NONE',  ( 110.6184472392236700, 29.05585583753637735, 83.30291117284286884 ) ) ;
#31144=CARTESIAN_POINT ( 'NONE',  ( -149.5074843970971017, 65.50121172469319220, 18.87627064943540134 ) ) ;
#31147=CARTESIAN_POINT ( 'NONE',  ( 181.5127080940606561, 79.03904173130084132, -36.22505766587960352 ) ) ;
#31149=CARTESIAN_POINT ( 'NONE',  ( -156.7943706409895412, 71.98431607767156493, 93.71821196632575379 ) ) ;
#31155=CARTESIAN_POINT ( 'NONE',  ( -80.55742067659893735, 23.05042616197515670, 57.48945466102705382 ) ) ;
#31157=CARTESIAN_POINT ( 'NONE',  ( 103.3213573731405290, 25.80935123464501046, -94.19314425201019958 ) ) ;
#31159=CARTESIAN_POINT ( 'NONE',  ( -37.52119286077851967, 11.69341290629617802, -74.05703107814400710 ) ) ;
#31160=CARTESIAN_POINT ( 'NONE',  ( -150.3898662070192245, 64.92828409760431896, -7.968279941028269420 ) ) ;
#31162=CARTESIAN_POINT ( 'NONE',  ( 38.42020198992004509, 8.283430712587442457, 56.80691058368965685 ) ) ;
#31163=CARTESIAN_POINT ( 'NONE',  ( 11.82322073186613487, 6.406156243758799107, -22.54526628955453660 ) ) ;
#31165=CARTESIAN_POINT ( 'NONE',  ( -7.330690860789850660, 6.858814156830897346, -35.41807073194382838 ) ) ;
#31167=CARTESIAN_POINT ( 'NONE',  ( -125.4481990864045002, 46.20056605584954923, 3.775397282693378820 ) ) ;
#31168=CARTESIAN_POINT ( 'NONE',  ( 69.50572373348798294, 14.27208627753790005, -66.27431351737995158 ) ) ;
#31169=CARTESIAN_POINT ( 'NONE',  ( 131.6005058089755835, 40.07838125795770878, -23.84668524735129225 ) ) ;
#31170=B_SPLINE_CURVE_WITH_KNOTS ( 'NONE', 3,
 ( #495, #43396, #31817, #38123, #5077, #47976, #9681, #63485, #52579, #21258, #15300, #36755, #64166, #37429, #4398, #52909, #4731, #55701, #6473, #54993, #28626, #28983, #12802, #44446, #59566, #6814, #11382, #32850, #50078, #28264, #7171, #23000, #65935, #50430, #12447, #33906 ),
 .UNSPECIFIED., .F., .F.,
 ( 4, 2, 2, 2, 2, 2, 2, 2, 2, 2, 2, 2, 2, 2, 2, 2, 2, 4 ),
 ( 3.469446951953614189E-18, 0.001545474820159053976, 0.003090949640318104482, 0.004636424460477154771, 0.006181899280636205495, 0.007727374100795257085, 0.008500111510874769002, 0.009272848920954281787, 0.01081832374111331256, 0.01236379856127234160, 0.01390927338143137064, 0.01545474820159039968, 0.01700022302174943045, 0.01854569784190845602, 0.02009117266206748506, 0.02163664748222651410, 0.02318212230238553273, 0.02472759712254455483 ),
 .UNSPECIFIED. ) ;
#31171=CARTESIAN_POINT ( 'NONE',  ( 17.72748965151693312, 7.577488030789624851, -8.925253431473967325 ) ) ;
#31172=CARTESIAN_POINT ( 'NONE',  ( 8.336237313193164411, 7.382629160459398321, 11.64778143086688011 ) ) ;
#31175=DIRECTION ( 'NONE',  ( -0.000000000000000000, 1.000000000000000000, -0.000000000000000000 ) ) ;
#31177=CARTESIAN_POINT ( 'NONE',  ( 173.9413349464226997, 71.67637800842355489, 34.50366122527430690 ) ) ;
#31179=CARTESIAN_POINT ( 'NONE',  ( 42.03492317486904994, 8.766487167902388578, -76.99122434333160925 ) ) ;
#31180=CARTESIAN_POINT ( 'NONE',  ( 184.9757174666827382, 84.09845285279334348, -50.14020102364498399 ) ) ;
#31183=CARTESIAN_POINT ( 'NONE',  ( -24.70911172866234295, 8.583078995053023519, -19.31926905173414966 ) ) ;
#31184=CARTESIAN_POINT ( 'NONE',  ( 200.8303160266299301, 102.8412051751308809, 16.30336876723097106 ) ) ;
#31186=CARTESIAN_POINT ( 'NONE',  ( 113.8748103246145575, 30.59837980920004696, 70.53553382418881768 ) ) ;
#31188=CARTESIAN_POINT ( 'NONE',  ( -133.3122825023497171, -170.0000000000000000, -95.00000000000133582 ) ) ;
#31194=ORIENTED_EDGE ( 'NONE', *, *, #33532, .F. ) ;
#31197=VERTEX_POINT ( 'NONE', #44116 ) ;
#31199=CARTESIAN_POINT ( 'NONE',  ( -119.1795380580999790, 42.22910606512925114, -18.92106183394395202 ) ) ;
#31201=CARTESIAN_POINT ( 'NONE',  ( -175.1920326508032701, 89.46239303019291356, -22.58843696369808285 ) ) ;
#31203=CARTESIAN_POINT ( 'NONE',  ( -131.2955621888335429, 51.38237199780174080, 59.73917619575056648 ) ) ;
#31205=CARTESIAN_POINT ( 'NONE',  ( 62.53356220515463093, 13.59349015304564467, 2.968410348757589023 ) ) ;
#31212=CARTESIAN_POINT ( 'NONE',  ( -126.8016613879753578, 48.30316697011514293, -61.79973845963801438 ) ) ;
#31213=DIRECTION ( 'NONE',  ( -0.000000000000000000, 0.000000000000000000, -1.000000000000000000 ) ) ;
#31214=DIRECTION ( 'NONE',  ( -0.000000000000000000, 1.000000000000000000, -0.000000000000000000 ) ) ;
#31222=CARTESIAN_POINT ( 'NONE',  ( -190.6985136298601731, 109.1272424661242582, 94.99999999999866418 ) ) ;
#31224=CARTESIAN_POINT ( 'NONE',  ( 80.72161230109726660, 17.48902961068030137, 32.56519435810803742 ) ) ;
#31225=CARTESIAN_POINT ( 'NONE',  ( -143.2464978228200039, 59.04559547356111437, 42.35829187257395745 ) ) ;
#31226=CARTESIAN_POINT ( 'NONE',  ( 15.78827728214693416, -170.0000000000000000, -62.36349468914946925 ) ) ;
#31227=CARTESIAN_POINT ( 'NONE',  ( -165.7143741370937278, 79.24519349471960084, -70.27428026180706411 ) ) ;
#31228=ORIENTED_EDGE ( 'NONE', *, *, #64969, .T. ) ;
#31229=CARTESIAN_POINT ( 'NONE',  ( -109.7290872258107157, 36.72869630780160577, -16.68929740702757769 ) ) ;
#31231=CARTESIAN_POINT ( 'NONE',  ( 80.92695752160176426, 18.60786019495465027, -92.06836682371273639 ) ) ;
#31236=DIRECTION ( 'NONE',  ( -0.8118923937861950435, -0.5838071093367415143, 0.000000000000000000 ) ) ;
#31238=CARTESIAN_POINT ( 'NONE',  ( 36.99625334683018707, 8.108440754877204171, 3.448660572988824669 ) ) ;
#31240=CARTESIAN_POINT ( 'NONE',  ( -35.99414836699283882, 11.40630460607620122, -21.95128177927970725 ) ) ;
#31242=VECTOR ( 'NONE', #62056, 1000.000000000000000 ) ;
#31243=CARTESIAN_POINT ( 'NONE',  ( -122.1170451552604277, 45.24844212239635510, -89.61962605176735508 ) ) ;
#31246=CARTESIAN_POINT ( 'NONE',  ( 8.288696687633803961, 7.382586467017839382, -70.36437873598936221 ) ) ;
#31247=CARTESIAN_POINT ( 'NONE',  ( -23.98903001682803904, 8.486614814224626713, 9.877694052388251933 ) ) ;
#31248=CARTESIAN_POINT ( 'NONE',  ( 211.7634543339367781, -170.0000000000000000, -95.00000000000133582 ) ) ;
#31249=CARTESIAN_POINT ( 'NONE',  ( -11.57808265946730231, 7.164483090579921942, -76.26091628640612896 ) ) ;
#31250=CARTESIAN_POINT ( 'NONE',  ( -95.50384525802330415, 29.46973564057718065, -12.44541413338938440 ) ) ;
#31253=CARTESIAN_POINT ( 'NONE',  ( 156.5993887774280324, 58.24868799840906064, -51.07665877090285989 ) ) ;
#31258=CARTESIAN_POINT ( 'NONE',  ( 176.6238742729555611, 75.60943990211369226, -22.92894773880436077 ) ) ;
#31260=CARTESIAN_POINT ( 'NONE',  ( -55.05276343752910151, 14.68156374112636264, -50.21632399845989170 ) ) ;
#31262=DIRECTION ( 'NONE',  ( 0.000000000000000000, 0.000000000000000000, 1.000000000000000000 ) ) ;
#31263=CARTESIAN_POINT ( 'NONE',  ( -0.5158933718595597462, 6.525180340836103099, -14.37622864181621374 ) ) ;
#31264=CARTESIAN_POINT ( 'NONE',  ( 201.5987353083855567, 103.8544727311227263, -23.82465923633973048 ) ) ;
#31265=CARTESIAN_POINT ( 'NONE',  ( -148.5360305860837116, 63.35984549844194902, 84.46819988047289485 ) ) ;
#31267=CARTESIAN_POINT ( 'NONE',  ( 139.3067271572849677, 44.81402783181198402, 42.16869312922494117 ) ) ;
#31270=CARTESIAN_POINT ( 'NONE',  ( 113.4351684956570097, 30.38657459074489253, -77.07004752621021737 ) ) ;
#31271=CARTESIAN_POINT ( 'NONE',  ( 181.0840389613909736, 80.03940679743415387, 44.30859410551141764 ) ) ;
#31272=CARTESIAN_POINT ( 'NONE',  ( 156.5993887774280324, 58.24868799840906064, 29.45699300048817193 ) ) ;
#31276=CARTESIAN_POINT ( 'NONE',  ( 176.6238742729555327, 75.60943990211367804, 57.60470403258671013 ) ) ;
#31279=CARTESIAN_POINT ( 'NONE',  ( -76.32962633615589709, 21.44528079176261670, -22.90158379948196199 ) ) ;
#31280=CARTESIAN_POINT ( 'NONE',  ( 70.25990036603477051, 14.47042233282418700, -68.10757834462343396 ) ) ;
#31281=CARTESIAN_POINT ( 'NONE',  ( -56.02027488966933078, 14.94257193099086045, 45.27018892150354645 ) ) ;
#31282=CARTESIAN_POINT ( 'NONE',  ( 150.2941978382489197, 53.52137138947625061, 7.867929705122802986 ) ) ;
#31284=CARTESIAN_POINT ( 'NONE',  ( -180.0175713311536470, 95.14770835574078944, 35.35984136943162071 ) ) ;
#31293=CARTESIAN_POINT ( 'NONE',  ( 140.4897729434290170, 45.57634363643750675, 67.39407047049898836 ) ) ;
#31294=DIRECTION ( 'NONE',  ( -0.000000000000000000, 1.000000000000000000, -0.000000000000000000 ) ) ;
#31303=CARTESIAN_POINT ( 'NONE',  ( 211.8345664497466316, 118.5225165986914533, -19.30918099180828307 ) ) ;
#31304=CARTESIAN_POINT ( 'NONE',  ( 103.0124792097646491, 26.77148435100181345, 35.05276459316780091 ) ) ;
#31307=CARTESIAN_POINT ( 'NONE',  ( 187.8973304652193690, 87.27378997243177139, 6.817108339809598405 ) ) ;
#31308=CARTESIAN_POINT ( 'NONE',  ( 205.5105258529713410, 107.4632495673648691, -36.35903942194123317 ) ) ;
#31313=CARTESIAN_POINT ( 'NONE',  ( -73.80418150970712077, 21.59712875466424009, 59.03090319298773636 ) ) ;
#31316=CARTESIAN_POINT ( 'NONE',  ( 55.61382797299290104, 11.07686102552915486, -71.30009820847813273 ) ) ;
#31319=CARTESIAN_POINT ( 'NONE',  ( -2.101755354351193539, 6.585774088635568901, 86.44700550218486512 ) ) ;
#31322=CARTESIAN_POINT ( 'NONE',  ( 164.9547823171479877, 65.03046442419432083, -71.02841637048652501 ) ) ;
#31325=CARTESIAN_POINT ( 'NONE',  ( 200.2082720696348588, 100.3848492891406750, -91.49428350888068451 ) ) ;
#31329=DIRECTION ( 'NONE',  ( -1.000000000000000000, 0.000000000000000000, 0.000000000000000000 ) ) ;
#31333=CARTESIAN_POINT ( 'NONE',  ( -131.3096895243910751, 51.39228038925230635, 43.33102018556300550 ) ) ;
#31334=EDGE_LOOP ( 'NONE', ( #49714, #7266, #19075, #28788 ) ) ;
#31335=CARTESIAN_POINT ( 'NONE',  ( 15.78827728214693416, 7.507518794609589818, -50.51894409868581448 ) ) ;
#31336=CARTESIAN_POINT ( 'NONE',  ( 11.81843724556920883, 7.412394300769734379, 70.72722298566459642 ) ) ;
#31339=VERTEX_POINT ( 'NONE', #8244 ) ;
#31343=CARTESIAN_POINT ( 'NONE',  ( -132.6811329440527061, 52.36246882380746115, 94.99999999999866418 ) ) ;
#31344=CARTESIAN_POINT ( 'NONE',  ( -166.3188283541501846, 79.86268666707378827, -18.53829102832942510 ) ) ;
#31346=CARTESIAN_POINT ( 'NONE',  ( 67.92995549349549833, 13.86623459444476758, 31.62639109689230921 ) ) ;
#31347=CARTESIAN_POINT ( 'NONE',  ( 8.368703124675214156, 7.382636543903409176, 89.92552182398135585 ) ) ;
#31348=B_SPLINE_CURVE_WITH_KNOTS ( 'NONE', 3,
 ( #8553, #24038, #55335, #39518, #13143, #44796, #39179, #51464, #28974, #19094, #12791, #61661, #40548, #28619, #60622, #34607, #7860, #2240, #22992, #50759, #50068, #45479, #45832, #29308, #44436, #39861, #65925, #12438, #18068, #60966, #61999, #67308, #2580, #1899, #66961, #8202, #55691, #24390, #23689, #23353, #34940, #56381, #51115, #13815, #33897 ),
 .UNSPECIFIED., .F., .F.,
 ( 4, 2, 2, 2, 2, 2, 2, 2, 1, 2, 2, 2, 2, 2, 2, 2, 2, 2, 2, 2, 2, 2, 4 ),
 ( 1.734723475976807094E-18, 0.001467747071934204835, 0.002201620607901308771, 0.002935494143868413140, 0.004403241215802621011, 0.005870988287736829750, 0.007338735359671038488, 0.008072608895638135051, 0.008806482431605229880, 0.009540355967572328177, 0.01027422950353942301, 0.01174197657547363521, 0.01247585011144074219, 0.01320972364740784742, 0.01467747071934208045, 0.01541134425530918742, 0.01614521779127629092, 0.01761296486321051874, 0.01908071193514474656, 0.01981458547111185353, 0.02054845900707896744, 0.02201620607901318832, 0.02348395315094740227 ),
 .UNSPECIFIED. ) ;
#31352=CARTESIAN_POINT ( 'NONE',  ( -99.98930671699733352, 31.63190627461931470, 57.70662428919617071 ) ) ;
#31354=CARTESIAN_POINT ( 'NONE',  ( -83.52505811737952968, 24.23179517241435121, 5.338914906993961651 ) ) ;
#31357=B_SPLINE_CURVE_WITH_KNOTS ( 'NONE', 3,
 ( #40957, #46572, #37391, #48972, #21560, #43357, #45016, #18290, #27183, #59186, #21229, #48615, #64831, #13030, #26504, #43004, #64478, #38086, #50307, #16292, #11008, #12669, #66158, #59530, #23238, #5724, #64130, #15946, #32471, #17949, #39749, #11348, #34134, #61204, #39400, #53212, #53904, #60849, #58845, #48275, #5042, #47941, #16630, #10659, #26849, #21910, #103 ),
 .UNSPECIFIED., .F., .F.,
 ( 4, 2, 2, 2, 2, 2, 2, 2, 2, 2, 2, 2, 1, 2, 2, 2, 2, 2, 2, 2, 2, 2, 2, 4 ),
 ( 0.000000000000000000, 0.001493793014771646350, 0.002240689522157466706, 0.002987586029543287496, 0.004481379044314894380, 0.005228275551700687848, 0.005975172059086479581, 0.007468965073858052639, 0.008215861581243833964, 0.008962758088629617023, 0.01045655110340117273, 0.01120344761078695232, 0.01195034411817272844, 0.01269724062555850803, 0.01344413713294428762, 0.01493793014771584333, 0.01568482665510159690, 0.01643172316248735221, 0.01792551617725889404, 0.01941930919203043934, 0.02016620569941620852, 0.02091310220680198811, 0.02240689522157354729, 0.02390068823634510647 ),
 .UNSPECIFIED. ) ;
#31358=VERTEX_POINT ( 'NONE', #28661 ) ;
#31360=CARTESIAN_POINT ( 'NONE',  ( -124.9915686518654638, 47.10215472274615678, 18.77539728269343300 ) ) ;
#31361=CARTESIAN_POINT ( 'NONE',  ( -178.2381786520593323, 93.01028335822120141, 70.65477212569948051 ) ) ;
#31362=CARTESIAN_POINT ( 'NONE',  ( 19.11168290073778664, 6.629794975642856691, 17.39810640889013982 ) ) ;
#31367=CARTESIAN_POINT ( 'NONE',  ( -25.76662357285300686, 8.728786737612503899, 86.48839091911142418 ) ) ;
#31368=CARTESIAN_POINT ( 'NONE',  ( 150.0889146124742979, 52.13243511955543852, 35.55320488847186766 ) ) ;
#31372=CARTESIAN_POINT ( 'NONE',  ( -29.51060362117876679, 9.282716514427262311, 30.46451046403358731 ) ) ;
#31373=CARTESIAN_POINT ( 'NONE',  ( -146.5309471467635944, 62.99917515507669208, -62.26958893730678568 ) ) ;
#31374=ORIENTED_EDGE ( 'NONE', *, *, #27295, .F. ) ;
#31376=CARTESIAN_POINT ( 'NONE',  ( -82.33596576276349310, 24.83688096733768447, -62.90096193187974194 ) ) ;
#31379=DIRECTION ( 'NONE',  ( 0.000000000000000000, 0.000000000000000000, 1.000000000000000000 ) ) ;
#31380=CARTESIAN_POINT ( 'NONE',  ( 133.8566784816069628, 41.42467568809806977, 17.66579024853170310 ) ) ;
#31381=CARTESIAN_POINT ( 'NONE',  ( -157.0069704378501854, 70.81086990254190994, 11.95845096291080800 ) ) ;
#31382=CARTESIAN_POINT ( 'NONE',  ( -124.9915686518654496, 47.10215472274615678, -61.75825448869760237 ) ) ;
#31383=CARTESIAN_POINT ( 'NONE',  ( 63.49940197359695304, 12.78497925206075614, 2.968410348757586803 ) ) ;
#31385=CARTESIAN_POINT ( 'NONE',  ( -109.0297561673456386, 36.34391931706015555, 41.29912065558960421 ) ) ;
#31387=CARTESIAN_POINT ( 'NONE',  ( -51.71962244998664460, 14.85104855202525087, 84.78028665116053730 ) ) ;
#31390=ORIENTED_EDGE ( 'NONE', *, *, #61830, .F. ) ;
#31392=DIRECTION ( 'NONE',  ( 0.000000000000000000, 0.000000000000000000, 1.000000000000000000 ) ) ;
#31394=CARTESIAN_POINT ( 'NONE',  ( -171.5023337025455703, 86.83681590836894770, 30.98698263294540922 ) ) ;
#31395=CARTESIAN_POINT ( 'NONE',  ( 64.69649025047539226, 13.06878919510321069, -23.68941227953380491 ) ) ;
#31398=VECTOR ( 'NONE', #17400, 1000.000000000000000 ) ;
#31399=CARTESIAN_POINT ( 'NONE',  ( 138.5684226926155134, 45.53585076428271350, -37.66822987502320785 ) ) ;
#31400=CARTESIAN_POINT ( 'NONE',  ( 38.90894112122322213, 8.345444037631240874, -35.61981746542777216 ) ) ;
#31401=CARTESIAN_POINT ( 'NONE',  ( 150.2809931605061990, 52.27058242113232467, -45.77730096997402853 ) ) ;
#31404=FACE_OUTER_BOUND ( 'NONE', #37310, .T. ) ;
#31407=CARTESIAN_POINT ( 'NONE',  ( 174.1490454011869247, 73.24869551604541584, 87.53382120110444475 ) ) ;
#31409=CARTESIAN_POINT ( 'NONE',  ( -168.0052514572427071, 83.06849406765624622, -9.877606560333585861 ) ) ;
#31416=CARTESIAN_POINT ( 'NONE',  ( 92.21267147730743829, 21.40196534721317079, -11.44563081337609134 ) ) ;
#31419=CARTESIAN_POINT ( 'NONE',  ( 163.1313205310724754, 63.49733392291052780, 68.67987254822025989 ) ) ;
#31421=CARTESIAN_POINT ( 'NONE',  ( 127.4669243510812890, 38.85312661085429653, 14.12496005488912054 ) ) ;
#31424=CARTESIAN_POINT ( 'NONE',  ( -108.1180879163843400, 36.99199941971029659, -64.62439509494042511 ) ) ;
#31425=CARTESIAN_POINT ( 'NONE',  ( -47.55235941796721022, 12.79790236059689512, -42.47865514628445993 ) ) ;
#31427=CARTESIAN_POINT ( 'NONE',  ( -0.5066725584836090368, 7.531654729013470551, 89.63377582999561355 ) ) ;
#31429=DIRECTION ( 'NONE',  ( 0.000000000000000000, 0.000000000000000000, 1.000000000000000000 ) ) ;
#31434=CARTESIAN_POINT ( 'NONE',  ( 33.22375030330210421, 8.697783996218335645, 86.83782710728377197 ) ) ;
#31435=CARTESIAN_POINT ( 'NONE',  ( -180.5231752320737826, 95.76423526868923375, -67.80882487326303476 ) ) ;
#31436=CARTESIAN_POINT ( 'NONE',  ( 140.1190804604727589, 46.53525738079846263, -93.06488777412555180 ) ) ;
#31441=CARTESIAN_POINT ( 'NONE',  ( 34.45817031441433187, 7.817703378455679086, -21.93692879055299016 ) ) ;
#31442=DIRECTION ( 'NONE',  ( -0.8118923937861950435, -0.5838071093367415143, 0.000000000000000000 ) ) ;
#31448=CARTESIAN_POINT ( 'NONE',  ( 108.3942953861066485, 29.14039925067523740, -23.86156525699782094 ) ) ;
#31451=CARTESIAN_POINT ( 'NONE',  ( 9.045716588192249219, 7.384596431530733973, 40.83588045389161891 ) ) ;
#31452=CARTESIAN_POINT ( 'NONE',  ( 197.2199569260504006, 98.22436319491367840, 37.37150111065846403 ) ) ;
#31454=CARTESIAN_POINT ( 'NONE',  ( -85.59501769175496122, 26.17305447445046696, 88.66329033029090567 ) ) ;
#31459=ORIENTED_EDGE ( 'NONE', *, *, #65093, .F. ) ;
#31460=CARTESIAN_POINT ( 'NONE',  ( 115.7612476187724013, 32.64200929566224119, -65.16402729089644197 ) ) ;
#31461=CYLINDRICAL_SURFACE ( 'NONE', #12071, 7.500000000000013323 ) ;
#31464=FACE_OUTER_BOUND ( 'NONE', #13113, .T. ) ;
#31465=CARTESIAN_POINT ( 'NONE',  ( 151.7819978880463907, 53.35998893001568177, -75.36307041061454015 ) ) ;
#31467=CARTESIAN_POINT ( 'NONE',  ( -154.2585856850055848, 68.31650218414630160, -48.12096048054596764 ) ) ;
#31472=CARTESIAN_POINT ( 'NONE',  ( -79.14094329813315198, 23.58034730000058588, -50.11545063171793402 ) ) ;
#31473=CARTESIAN_POINT ( 'NONE',  ( 164.0298848570286907, 62.93631132702880393, 67.42917240860492711 ) ) ;
#31475=CARTESIAN_POINT ( 'NONE',  ( -156.9919426121902575, 72.16759471857101005, 11.93913789850172336 ) ) ;
#31477=CARTESIAN_POINT ( 'NONE',  ( 16.77391662606471456, 6.533867394142991003, 44.96609377977839728 ) ) ;
#31481=ORIENTED_EDGE ( 'NONE', *, *, #68150, .F. ) ;
#31484=CARTESIAN_POINT ( 'NONE',  ( 34.82939798935584719, 8.870855050008909615, -37.15461301836749186 ) ) ;
#31487=CARTESIAN_POINT ( 'NONE',  ( -38.16652041892308489, 11.81761816422914535, -73.01350053778892857 ) ) ;
#31488=CARTESIAN_POINT ( 'NONE',  ( 197.3756653044964082, 98.41886189307119537, 61.92014655920272759 ) ) ;
#31492=CARTESIAN_POINT ( 'NONE',  ( 46.48120921213031664, 9.436135543404052584, 88.60415001228606968 ) ) ;
#31494=CARTESIAN_POINT ( 'NONE',  ( 16.77104078056616387, 7.540619757007626767, 18.12152667333544898 ) ) ;
#31495=CARTESIAN_POINT ( 'NONE',  ( 181.0840389613909736, 78.60582251573003987, 56.15314469597509373 ) ) ;
#31497=CARTESIAN_POINT ( 'NONE',  ( -84.22570405563702423, 24.51726571826274537, -37.55730470497496754 ) ) ;
#31498=CARTESIAN_POINT ( 'NONE',  ( 128.0568017572569488, 38.03085713813911184, -21.46075403565069450 ) ) ;
#31500=CARTESIAN_POINT ( 'NONE',  ( 10.31616749326173910, 7.393414706728907326, 5.535394398224304346 ) ) ;
#31501=VERTEX_POINT ( 'NONE', #59087 ) ;
#31502=CARTESIAN_POINT ( 'NONE',  ( 185.5572090022886016, 83.24697331286186852, 16.00218672843412548 ) ) ;
#31505=CARTESIAN_POINT ( 'NONE',  ( 176.4367926094705297, 74.03315361639847936, 30.91700671302049841 ) ) ;
#31507=CARTESIAN_POINT ( 'NONE',  ( -106.7004823116342607, 36.22460663120047997, -36.43660411563737966 ) ) ;
#31508=DIRECTION ( 'NONE',  ( -0.000000000000000000, 1.000000000000000000, -0.000000000000000000 ) ) ;
#31509=EDGE_LOOP ( 'NONE', ( #34744, #24988, #33253, #36670 ) ) ;
#31512=ADVANCED_FACE ( 'NONE', ( #41633 ), #42903, .F. ) ;
#31515=CARTESIAN_POINT ( 'NONE',  ( 173.8519557319370392, 71.59321990351749321, 88.50132255048274033 ) ) ;
#31516=ORIENTED_EDGE ( 'NONE', *, *, #12627, .T. ) ;
#31518=CARTESIAN_POINT ( 'NONE',  ( 114.6890011751076202, 30.99337387307414815, 70.01517709306831705 ) ) ;
#31519=B_SPLINE_CURVE_WITH_KNOTS ( 'NONE', 3,
 ( #43381, #64851, #49344, #38820, #32836, #16651, #44431, #50062, #45825, #56373, #65917, #33891, #56037, #50753, #60268, #12086, #29300, #7516, #61654, #22987, #60616, #18060, #29643, #33553, #7853, #55328, #51108, #1892, #2573, #6797, #2917, #44789, #23346, #66270, #34931, #24030, #28248, #24381, #67302, #13136, #1524, #7152, #49694 ),
 .UNSPECIFIED., .F., .F.,
 ( 4, 2, 2, 2, 2, 2, 2, 2, 2, 2, 2, 2, 1, 2, 2, 2, 2, 2, 2, 2, 2, 4 ),
 ( 0.02390068823634510300, 0.02538837671117074798, 0.02613222094858357047, 0.02687606518599639296, 0.02836375366082206223, 0.02985144213564773150, 0.03059528637306055399, 0.03133913061047337995, 0.03282681908529903186, 0.03431450756012468378, 0.03580219603495033570, 0.03654604027236316166, 0.03728988450977598068, 0.03803372874718881358, 0.03877757298460163260, 0.04026526145942728452, 0.04175294993425293644, 0.04324063840907858836, 0.04398448264649141431, 0.04472832688390424027, 0.04621601535872986444, 0.04770370383355549554 ),
 .UNSPECIFIED. ) ;
#31525=CARTESIAN_POINT ( 'NONE',  ( 163.8800397297740972, 62.81151592172381726, -93.41319794146498623 ) ) ;
#31526=CARTESIAN_POINT ( 'NONE',  ( 93.63037639125410294, 21.92981100938040484, -40.61996566342161685 ) ) ;
#31528=VERTEX_POINT ( 'NONE', #36013 ) ;
#31531=VERTEX_POINT ( 'NONE', #5623 ) ;
#31532=CARTESIAN_POINT ( 'NONE',  ( -118.4622862908118606, 41.79153065058244465, -14.52264416072287112 ) ) ;
#31535=CARTESIAN_POINT ( 'NONE',  ( -180.3158531669105855, 95.51092859788508349, -17.50723337383704958 ) ) ;
#31536=ADVANCED_FACE ( 'NONE', ( #30740 ), #46910, .F. ) ;
#31537=CARTESIAN_POINT ( 'NONE',  ( -145.3109762780891288, 60.69959559383372749, -36.07957426329402750 ) ) ;
#31538=ORIENTED_EDGE ( 'NONE', *, *, #56638, .F. ) ;
#31539=CARTESIAN_POINT ( 'NONE',  ( -109.1625286449147296, 37.56522729164488084, 94.70638889232425583 ) ) ;
#31541=CARTESIAN_POINT ( 'NONE',  ( -59.56523643198717366, 15.93788386494078502, -9.876116202400169186 ) ) ;
#31542=CARTESIAN_POINT ( 'NONE',  ( -132.8150886319751578, 52.45790550853838141, -72.15884298396014174 ) ) ;
#31543=CARTESIAN_POINT ( 'NONE',  ( 56.67004931728209982, 11.28989923258780159, 94.99999999999866418 ) ) ;
#31546=ORIENTED_EDGE ( 'NONE', *, *, #61214, .F. ) ;
#31547=EDGE_LOOP ( 'NONE', ( #9297, #3223, #25867, #55481 ) ) ;
#31549=CARTESIAN_POINT ( 'NONE',  ( 188.4389256074243804, 86.37278721358583766, -69.07214298238083927 ) ) ;
#31550=CARTESIAN_POINT ( 'NONE',  ( -165.6210506643949429, 79.15024150453837137, -41.91068780496413382 ) ) ;
#31553=CARTESIAN_POINT ( 'NONE',  ( -71.23176719684944658, 20.69188312694500809, 38.93799383707774098 ) ) ;
#31554=CARTESIAN_POINT ( 'NONE',  ( 79.19132716134491545, 17.01584750883627351, 36.21715455800038086 ) ) ;
#31555=CARTESIAN_POINT ( 'NONE',  ( 63.01563776193090405, 13.70579113808098271, -35.72069083216973695 ) ) ;
#31556=CARTESIAN_POINT ( 'NONE',  ( -118.5151419614604720, 43.00218563933589877, 39.48948330295599618 ) ) ;
#31559=ORIENTED_EDGE ( 'NONE', *, *, #46604, .T. ) ;
#31563=CARTESIAN_POINT ( 'NONE',  ( -15.32550079334878923, 7.496023944924841587, -43.15998724655409546 ) ) ;
#31565=CARTESIAN_POINT ( 'NONE',  ( 94.06416612695404922, 23.16920323269610194, 65.07509206730203744 ) ) ;
#31566=CARTESIAN_POINT ( 'NONE',  ( 152.3102623290680242, 53.74757787434987932, -11.33146698698797472 ) ) ;
#31567=CARTESIAN_POINT ( 'NONE',  ( 32.38493285958205803, 8.611594965040678673, 7.909991613938172961 ) ) ;
#31569=CARTESIAN_POINT ( 'NONE',  ( 34.84173759613682364, 7.859847277726514925, -63.98992801080245840 ) ) ;
#31570=CARTESIAN_POINT ( 'NONE',  ( -96.76336539645315327, 31.18045094643428428, -74.46404432994987133 ) ) ;
#31572=CARTESIAN_POINT ( 'NONE',  ( -34.74563762132953570, 11.17960945723135424, -9.236443799584387548 ) ) ;
#31574=CARTESIAN_POINT ( 'NONE',  ( -7.825402957745081878, 7.899365992529270741, 56.96013162991089018 ) ) ;
#31575=VERTEX_POINT ( 'NONE', #14892 ) ;
#31577=CARTESIAN_POINT ( 'NONE',  ( -190.3074740493606782, 108.5764897054613272, 7.695633288411995565 ) ) ;
#31578=LINE ( 'NONE', #63251, #40087 ) ;
#31579=CARTESIAN_POINT ( 'NONE',  ( -5.885876544836659896, 6.772369038004113939, 30.36654913812938261 ) ) ;
#31581=CARTESIAN_POINT ( 'NONE',  ( 152.8373718734505076, 55.38925997611394081, -37.70618783639333316 ) ) ;
#31585=CARTESIAN_POINT ( 'NONE',  ( 177.7964363391245115, 76.75162026635256041, -23.63659886028308676 ) ) ;
#31586=CARTESIAN_POINT ( 'NONE',  ( -104.1225399044495674, 34.86084180570099278, 57.58965421403807028 ) ) ;
#31592=CARTESIAN_POINT ( 'NONE',  ( -2.174378755909792460, 6.588636630831475216, -11.11814556240371132 ) ) ;
#31593=CARTESIAN_POINT ( 'NONE',  ( 199.2049631873262854, 100.7347227143600321, -11.86830923348487055 ) ) ;
#31595=CARTESIAN_POINT ( 'NONE',  ( -142.1931036653837737, 58.21544485181838269, 90.21602549727161602 ) ) ;
#31597=CARTESIAN_POINT ( 'NONE',  ( 141.2811136745703493, 46.09188267874203859, 35.91509209166238747 ) ) ;
#31599=DIRECTION ( 'NONE',  ( 1.000000000000000000, 0.000000000000000000, -0.000000000000000000 ) ) ;
#31600=CARTESIAN_POINT ( 'NONE',  ( 84.05289558242220949, 19.61733656419351846, 3.319883102769282335 ) ) ;
#31601=CARTESIAN_POINT ( 'NONE',  ( 164.9706294237033717, 65.04392654036657007, 9.790795167083055972 ) ) ;
#31611=CARTESIAN_POINT ( 'NONE',  ( -104.5827168854524416, 33.96561401163047123, -49.66786823832703135 ) ) ;
#31614=FACE_OUTER_BOUND ( 'NONE', #50388, .T. ) ;
#31617=CARTESIAN_POINT ( 'NONE',  ( -175.9970298498767534, 90.38640259140139221, 31.38186942925006662 ) ) ;
#31620=CARTESIAN_POINT ( 'NONE',  ( 113.8724110608469005, 31.71510301790680941, -50.00321340998061714 ) ) ;
#31621=ORIENTED_EDGE ( 'NONE', *, *, #41778, .T. ) ;
#31624=CYLINDRICAL_SURFACE ( 'NONE', #16780, 7.500000000000013323 ) ;
#31625=CARTESIAN_POINT ( 'NONE',  ( -31.93184248720558926, 9.672312402099827011, -62.16174795566553257 ) ) ;
#31626=CARTESIAN_POINT ( 'NONE',  ( 188.0081045302010807, 85.89855126821615272, -19.77675329002309468 ) ) ;
#31632=CARTESIAN_POINT ( 'NONE',  ( -59.75659776108101084, 15.99281909568473026, 85.62955986424741184 ) ) ;
#31635=CARTESIAN_POINT ( 'NONE',  ( 67.07698108884261501, 13.65136238353903408, 84.68817323788672979 ) ) ;
#31644=CARTESIAN_POINT ( 'NONE',  ( 57.39674746172462250, 11.43903079040059012, -65.07340723825461737 ) ) ;
#31646=CARTESIAN_POINT ( 'NONE',  ( -121.5928001448268958, 44.91559452735375402, 71.12660519080166921 ) ) ;
#31647=CARTESIAN_POINT ( 'NONE',  ( 23.23965501943000334, 7.861749956303023978, 36.53097551103099505 ) ) ;
#31649=CARTESIAN_POINT ( 'NONE',  ( 164.8433205901838789, 64.93586312665799198, -69.06606882681678883 ) ) ;
#31650=VERTEX_POINT ( 'NONE', #28125 ) ;
#31653=CARTESIAN_POINT ( 'NONE',  ( -72.78737098446266884, 20.16853011470089285, 60.07899134986872269 ) ) ;
#31654=CARTESIAN_POINT ( 'NONE',  ( 198.8923184520479026, 98.70864400575095488, -92.76185446744425178 ) ) ;
#31659=B_SPLINE_CURVE_WITH_KNOTS ( 'NONE', 3,
 ( #63855, #15664, #4755, #43761, #58554, #26562, #20937, #47999, #32875, #10717, #10371, #5784, #31837, #31497, #54307, #65232, #32191, #53273, #38497, #26218, #42393, #47657, #69462, #53623, #26902, #21281, #48328, #42730, #37447, #64186, #58901, #21620, #27241, #43066, #16347, #517, #21967, #60304, #33237, #54668, #65955, #44109, #6496, #56076, #38864, #55016, #23721 ),
 .UNSPECIFIED., .F., .F.,
 ( 4, 2, 2, 2, 2, 2, 2, 2, 2, 2, 2, 2, 1, 2, 2, 2, 2, 2, 2, 2, 2, 2, 2, 4 ),
 ( 0.000000000000000000, 0.001520400357568958694, 0.002280600536353455388, 0.003040800715137951648, 0.004561201072706938531, 0.005321401251491414408, 0.006081601430275891153, 0.007602001787844816887, 0.008362201966629284958, 0.009122402145413752161, 0.01064280250298270565, 0.01140300268176718326, 0.01216320286055166087, 0.01292340303933613849, 0.01368360321812061610, 0.01520400357568958000, 0.01596420375447405934, 0.01672440393325854216, 0.01824480429082751820, 0.01976520464839649424, 0.02052540482718098400, 0.02128560500596547028, 0.02280600536353445673, 0.02432640572110343624 ),
 .UNSPECIFIED. ) ;
#31668=CARTESIAN_POINT ( 'NONE',  ( -132.8257891167039304, 52.46553896898736014, 40.99495158203683332 ) ) ;
#31670=CARTESIAN_POINT ( 'NONE',  ( 38.43102714813441878, 9.298961820315048143, -23.72831626942832628 ) ) ;
#31671=CARTESIAN_POINT ( 'NONE',  ( -148.6471085600700235, 64.76880961642446266, 30.75770659792187800 ) ) ;
#31672=CARTESIAN_POINT ( 'NONE',  ( 205.1049299651096760, 106.9023875785546664, 44.20772073876946706 ) ) ;
#31681=CARTESIAN_POINT ( 'NONE',  ( -170.2801941679960578, 84.02053682015871061, -22.32142513227474367 ) ) ;
#31685=CARTESIAN_POINT ( 'NONE',  ( 8.639536176317964333, 7.383242619405921303, 93.49568538271768148 ) ) ;
#31688=CARTESIAN_POINT ( 'NONE',  ( -94.89192151156326815, 29.18342430963126688, 63.54748444646997285 ) ) ;
#31690=CARTESIAN_POINT ( 'NONE',  ( -81.90020664963799391, 23.57971581008656514, 4.302302874625238083 ) ) ;
#31691=ORIENTED_EDGE ( 'NONE', *, *, #35993, .F. ) ;
#31695=CARTESIAN_POINT ( 'NONE',  ( -119.5404913382140109, 43.63271406506959238, 7.281364596653088661 ) ) ;
#31697=CARTESIAN_POINT ( 'NONE',  ( -177.1540936177022445, 91.73126115633625943, 58.82771625204114940 ) ) ;
#31699=CARTESIAN_POINT ( 'NONE',  ( 126.6576865394846152, 37.24426596493988484, 65.97471202277128555 ) ) ;
#31703=CARTESIAN_POINT ( 'NONE',  ( -34.85922420997363957, 10.17769528929257561, 84.72309154256973329 ) ) ;
#31704=CARTESIAN_POINT ( 'NONE',  ( 149.9552318559266837, 52.03645904563048674, 36.93262037564134914 ) ) ;
#31706=CARTESIAN_POINT ( 'NONE',  ( 103.4696172145934838, 25.87254488218943749, -40.19200279096821760 ) ) ;
#31707=CARTESIAN_POINT ( 'NONE',  ( 138.1901928158493149, 45.29454828899441310, -64.22858801807878137 ) ) ;
#31713=CARTESIAN_POINT ( 'NONE',  ( 179.4074606910091347, 78.34362448405026669, 17.32480475505861506 ) ) ;
#31715=DIRECTION ( 'NONE',  ( 0.000000000000000000, 0.000000000000000000, 1.000000000000000000 ) ) ;
#31717=CARTESIAN_POINT ( 'NONE',  ( -156.0300823189602397, 69.91528270335481920, 7.635611034400681341 ) ) ;
#31718=CARTESIAN_POINT ( 'NONE',  ( -121.5928001448268816, 44.91559452735373981, -63.09614776151676097 ) ) ;
#31719=CARTESIAN_POINT ( 'NONE',  ( 68.63487067129261732, 14.04635751989138726, 15.45973179360630922 ) ) ;
#31720=CARTESIAN_POINT ( 'NONE',  ( -85.90077524418997257, 26.30132018890135370, 66.75733766280808368 ) ) ;
#31721=CARTESIAN_POINT ( 'NONE',  ( -108.6634958860518338, 36.14357436892402831, 41.96444054384087252 ) ) ;
#31725=ORIENTED_EDGE ( 'NONE', *, *, #15095, .F. ) ;
#31728=CARTESIAN_POINT ( 'NONE',  ( 22.72762739171800206, 7.830015800126070680, -66.98700550285960276 ) ) ;
#31730=CARTESIAN_POINT ( 'NONE',  ( -148.6426892915312123, 64.76241938621076599, 72.56537183036277838 ) ) ;
#31731=CARTESIAN_POINT ( 'NONE',  ( 70.51601918574517924, 14.53832276813547608, -16.13771727979073489 ) ) ;
#31733=CARTESIAN_POINT ( 'NONE',  ( -49.13048465129992337, 14.20828170588045936, -64.93260343570349846 ) ) ;
#31738=EDGE_LOOP ( 'NONE', ( #50263, #53525, #22739, #41982 ) ) ;
#31742=CARTESIAN_POINT ( 'NONE',  ( 127.3613131747807472, 38.79352689838291468, -93.43917518758931351 ) ) ;
#31743=PRODUCT_DEFINITION_CONTEXT ( 'detailed design', #50279, 'design' ) ;
#31744=AXIS2_PLACEMENT_3D ( 'NONE', #22376, #6553, #31897 ) ;
#31745=CARTESIAN_POINT ( 'NONE',  ( 69.01423235029108127, 15.18386996031285996, -92.38905430490223125 ) ) ;
#31747=CARTESIAN_POINT ( 'NONE',  ( 185.5412249395995730, 84.70425786165998261, -22.91669308973334651 ) ) ;
#31751=CARTESIAN_POINT ( 'NONE',  ( -174.7800083645696532, 88.99302808536934606, -49.53816181598559609 ) ) ;
#31752=CARTESIAN_POINT ( 'NONE',  ( 88.99522780200243233, 20.24180937454203644, -9.355914456664107703 ) ) ;
#31756=LINE ( 'NONE', #32452, #58010 ) ;
#31760=EDGE_CURVE ( 'NONE', #9029, #63051, #55994, .T. ) ;
#31762=CARTESIAN_POINT ( 'NONE',  ( -123.4416615615272832, 44.90042688650405012, -35.32212343775866970 ) ) ;
#31765=CARTESIAN_POINT ( 'NONE',  ( 154.0281735872262630, 56.28213428456460576, 70.42142694816533322 ) ) ;
#31766=CARTESIAN_POINT ( 'NONE',  ( -7.825402957745087207, -170.0000000000000000, 64.46013162991090439 ) ) ;
#31768=CARTESIAN_POINT ( 'NONE',  ( 151.3309484205704791, 53.03078371058071383, 14.38017068174847246 ) ) ;
#31769=CARTESIAN_POINT ( 'NONE',  ( -12.11199156453544923, 8.217753791142426323, 85.14174289210440350 ) ) ;
#31777=CARTESIAN_POINT ( 'NONE',  ( 136.9816124143867455, 44.53086385938545533, -90.39170542592599134 ) ) ;
#31781=CARTESIAN_POINT ( 'NONE',  ( -0.3255842968951676020, 7.525381170773408179, 11.26331030618680096 ) ) ;
#31783=CARTESIAN_POINT ( 'NONE',  ( 173.6007744016332879, 72.73482010729019009, -43.14319336715800546 ) ) ;
#31785=CARTESIAN_POINT ( 'NONE',  ( -149.7268278745401631, 65.68859631971241697, -76.65738112195569443 ) ) ;
#31788=ORIENTED_EDGE ( 'NONE', *, *, #64793, .T. ) ;
#31792=CARTESIAN_POINT ( 'NONE',  ( 15.29912143387263512, 7.491799981865496783, 30.01470767270521733 ) ) ;
#31793=CARTESIAN_POINT ( 'NONE',  ( 198.8752826725511511, 100.3130050945023726, 31.97338715271266096 ) ) ;
#31794=CARTESIAN_POINT ( 'NONE',  ( 79.13491102535617472, 16.99860516843601133, 90.45089180137320284 ) ) ;
#31803=CARTESIAN_POINT ( 'NONE',  ( -31.43908319763709969, 10.61114334766715928, 57.06100499665286208 ) ) ;
#31807=CARTESIAN_POINT ( 'NONE',  ( 154.4550750032601911, 55.34393534448157226, -63.59772041800123787 ) ) ;
#31810=CYLINDRICAL_SURFACE ( 'NONE', #9326, 7.500000000000013323 ) ;
#31812=VERTEX_POINT ( 'NONE', #25305 ) ;
#31813=CARTESIAN_POINT ( 'NONE',  ( 70.26936813788617542, 15.51386666370915535, -18.34636768599548517 ) ) ;
#31814=CARTESIAN_POINT ( 'NONE',  ( -83.51110947562234799, 25.31252704029287059, -48.34590627098496896 ) ) ;
#31816=CARTESIAN_POINT ( 'NONE',  ( 161.7209903610254571, 61.03262545641846515, 69.95060923550748555 ) ) ;
#31817=CARTESIAN_POINT ( 'NONE',  ( 111.1829448509513298, 30.43012797723691776, -9.122365715518217399 ) ) ;
#31819=CARTESIAN_POINT ( 'NONE',  ( 185.5572090022886300, 83.24697331286185431, -37.68691445249324801 ) ) ;
#31820=CARTESIAN_POINT ( 'NONE',  ( 21.42484406671928454, 6.746536496442161912, 32.56092050209711886 ) ) ;
#31821=CARTESIAN_POINT ( 'NONE',  ( -156.4791144138197296, 71.69273398181533707, 94.69527957875486379 ) ) ;
#31826=CARTESIAN_POINT ( 'NONE',  ( -155.2836587093738956, 70.59655508952972980, -20.25880271682157385 ) ) ;
#31827=CARTESIAN_POINT ( 'NONE',  ( 32.29578462738145817, 8.602609172809794202, -40.70879380640250389 ) ) ;
#31828=CARTESIAN_POINT ( 'NONE',  ( 176.6214367443247681, 74.20967084876663478, 69.69980881498953806 ) ) ;
#31832=CARTESIAN_POINT ( 'NONE',  ( 37.46254810722765427, 8.164772623042711786, 56.99704862271182293 ) ) ;
#31833=CARTESIAN_POINT ( 'NONE',  ( 8.480442907658517271, 6.376693431076494889, -14.46955541742294038 ) ) ;
#31835=CARTESIAN_POINT ( 'NONE',  ( 183.9986899696430669, 81.60141257362812439, 56.72931473510586642 ) ) ;
#31837=CARTESIAN_POINT ( 'NONE',  ( -83.69653436244855982, 24.30167057287990673, -37.04694618773496018 ) ) ;
#31848=CARTESIAN_POINT ( 'NONE',  ( 174.1251613516844543, 71.84747073139212148, 39.65969668319120700 ) ) ;
#31850=CARTESIAN_POINT ( 'NONE',  ( -105.8683518445188270, 35.77995342500074827, -49.11769980258868884 ) ) ;
#31852=CARTESIAN_POINT ( 'NONE',  ( 58.47885130911550533, 12.69429933094348506, -76.05780093763492289 ) ) ;
#31853=ORIENTED_EDGE ( 'NONE', *, *, #68145, .T. ) ;
#31855=ORIENTED_EDGE ( 'NONE', *, *, #17068, .T. ) ;
#31857=CARTESIAN_POINT ( 'NONE',  ( -29.02794087136070544, 9.207646203414356023, -8.854141498921386244 ) ) ;
#31859=CARTESIAN_POINT ( 'NONE',  ( 201.9721407532275350, 104.3507814346148308, 16.86238661557147367 ) ) ;
#31863=ORIENTED_EDGE ( 'NONE', *, *, #45566, .T. ) ;
#31869=CARTESIAN_POINT ( 'NONE',  ( -95.61819996182569525, 29.52346081122273347, 41.47345898016966004 ) ) ;
#31870=CARTESIAN_POINT ( 'NONE',  ( 87.58098510096633049, 19.74745174099416900, -50.77640564174353699 ) ) ;
#31871=CARTESIAN_POINT ( 'NONE',  ( -7.825402957745087207, -170.0000000000000000, -69.76262132240751157 ) ) ;
#31873=EDGE_CURVE ( 'NONE', #10603, #18346, #20720, .T. ) ;
#31874=ORIENTED_EDGE ( 'NONE', *, *, #30480, .T. ) ;
#31875=VERTEX_POINT ( 'NONE', #47415 ) ;
#31876=CARTESIAN_POINT ( 'NONE',  ( -120.1259246007803512, 42.81147313035990010, -10.74822668097895928 ) ) ;
#31879=CARTESIAN_POINT ( 'NONE',  ( -179.5082312244189211, 94.53075638132058600, -19.30745591354370205 ) ) ;
#31880=CARTESIAN_POINT ( 'NONE',  ( -167.4860113959265391, 82.52233889531187572, -64.10065570822085590 ) ) ;
#31881=CARTESIAN_POINT ( 'NONE',  ( -143.2471548081023514, 59.04577938365764567, -46.47464696708835419 ) ) ;
#31885=CARTESIAN_POINT ( 'NONE',  ( -133.3765738414514601, 51.62252165471731757, 38.69660473656405486 ) ) ;
#31886=CARTESIAN_POINT ( 'NONE',  ( -56.72814287166055891, 15.13700122306437557, -8.557341907245762158 ) ) ;
#31887=CARTESIAN_POINT ( 'NONE',  ( 82.14449817946437804, 17.93919511903896691, -10.46065494932177842 ) ) ;
#31890=DIRECTION ( 'NONE',  ( -0.000000000000000000, 1.000000000000000000, -0.000000000000000000 ) ) ;
#31895=AXIS2_PLACEMENT_3D ( 'NONE', #2000, #40647, #62103 ) ;
#31896=CARTESIAN_POINT ( 'NONE',  ( 188.0081045302011944, 85.89855126821616693, -73.46585447095047527 ) ) ;
#31897=DIRECTION ( 'NONE',  ( 0.000000000000000000, 0.000000000000000000, 1.000000000000000000 ) ) ;
#31901=CARTESIAN_POINT ( 'NONE',  ( 106.6322547488295385, 28.34756922280615399, -76.85819378913427613 ) ) ;
#31903=CARTESIAN_POINT ( 'NONE',  ( 79.93126905972556528, 17.24332478304276961, 33.82846076375348332 ) ) ;
#31904=CARTESIAN_POINT ( 'NONE',  ( 66.30230369578302430, 14.49551544185123930, -49.96661566441417079 ) ) ;
#31906=CARTESIAN_POINT ( 'NONE',  ( 46.23304607317101755, 10.41544405387738692, -46.22577417019589063 ) ) ;
#31907=CARTESIAN_POINT ( 'NONE',  ( 210.5178985598939221, 114.6803933586780886, 68.28892203333299449 ) ) ;
#31911=FACE_OUTER_BOUND ( 'NONE', #44101, .T. ) ;
#31913=CARTESIAN_POINT ( 'NONE',  ( -14.55390976651257162, 7.422979442794212623, -46.24041557031399918 ) ) ;
#31916=CARTESIAN_POINT ( 'NONE',  ( 79.22872707466393649, 18.07970189365809688, 65.29920498983847210 ) ) ;
#31917=CARTESIAN_POINT ( 'NONE',  ( 91.11019107624154856, 22.06959540317787116, 70.07588725628826865 ) ) ;
#31918=CARTESIAN_POINT ( 'NONE',  ( 151.6351261592328683, 53.25263237790400694, -12.06117684806004675 ) ) ;
#31920=CARTESIAN_POINT ( 'NONE',  ( 37.00112095025831138, 8.109340230899350743, -62.85478614795575680 ) ) ;
#31927=DIRECTION ( 'NONE',  ( -0.000000000000000000, 1.000000000000000000, -0.000000000000000000 ) ) ;
#31928=CARTESIAN_POINT ( 'NONE',  ( 10.31616749326172844, 7.393414706728908214, -74.99825737316675145 ) ) ;
#31929=CARTESIAN_POINT ( 'NONE',  ( -28.35330809568272770, 9.105138953156437509, 17.71201881402830836 ) ) ;
#31930=DIRECTION ( 'NONE',  ( 0.000000000000000000, -1.000000000000000000, 0.000000000000000000 ) ) ;
#31934=CARTESIAN_POINT ( 'NONE',  ( 79.26839340764567510, 18.09188476209940433, 89.42367620941877249 ) ) ;
#31939=CARTESIAN_POINT ( 'NONE',  ( -153.6994314938755508, 69.16570456337670691, 71.30114417014331707 ) ) ;
#31940=CARTESIAN_POINT ( 'NONE',  ( 174.2468109002381880, 73.34092405459587383, -13.78573923642201393 ) ) ;
#31941=CARTESIAN_POINT ( 'NONE',  ( -104.5740066103013106, 35.09687312794778080, 57.71916911584846588 ) ) ;
#31942=CARTESIAN_POINT ( 'NONE',  ( -132.2161740628506266, 52.03204870034953444, -46.45640934042872061 ) ) ;
#31945=CARTESIAN_POINT ( 'NONE',  ( -0.5780275525703851836, 6.527356703336896437, -18.01939305138792591 ) ) ;
#31947=CARTESIAN_POINT ( 'NONE',  ( -156.4787762129735711, 70.32547257834129084, 94.69602752494165543 ) ) ;
#31951=PLANE ( 'NONE',  #50314 ) ;
#31953=CARTESIAN_POINT ( 'NONE',  ( 164.8908506817023749, 64.97619709085122963, 11.18946311072333799 ) ) ;
#31956=ORIENTED_EDGE ( 'NONE', *, *, #52779, .F. ) ;
#31957=EDGE_CURVE ( 'NONE', #66812, #6692, #4335, .T. ) ;
#31958=CARTESIAN_POINT ( 'NONE',  ( 173.6007744016332595, 72.73482010729017588, 64.23500899469674152 ) ) ;
#31960=EDGE_LOOP ( 'NONE', ( #13703, #11386 ) ) ;
#31961=CARTESIAN_POINT ( 'NONE',  ( -103.2129897037411013, 33.25684593987700310, -35.05838499450624113 ) ) ;
#31964=CARTESIAN_POINT ( 'NONE',  ( -61.38706483483512244, 16.47181058798475917, 41.84068912785072314 ) ) ;
#31967=CARTESIAN_POINT ( 'NONE',  ( -179.5178913137216909, 94.54206947403388028, 42.27584261177923253 ) ) ;
#31969=DIRECTION ( 'NONE',  ( 0.000000000000000000, -1.000000000000000000, 0.000000000000000000 ) ) ;
#31970=EDGE_LOOP ( 'NONE', ( #53423, #57744, #13084, #4945 ) ) ;
#31974=CARTESIAN_POINT ( 'NONE',  ( 130.7457207912710828, 40.74300766298685517, 57.01493017841226418 ) ) ;
#31976=CARTESIAN_POINT ( 'NONE',  ( 43.96062659677685502, 10.06332325923985671, 16.54484489615712306 ) ) ;
#31981=CARTESIAN_POINT ( 'NONE',  ( -57.24414243706566197, 15.27981560285317109, 84.32688172081668654 ) ) ;
#31983=CARTESIAN_POINT ( 'NONE',  ( -156.8764584803562059, 70.69066846313526753, -70.58134442723202540 ) ) ;
#31984=CARTESIAN_POINT ( 'NONE',  ( -108.1183077156918841, 35.84680167036558629, 86.98961108605696779 ) ) ;
#31989=ORIENTED_EDGE ( 'NONE', *, *, #30109, .F. ) ;
#31991=CARTESIAN_POINT ( 'NONE',  ( -101.8638894403611204, 33.69766868189126541, -88.70367844590323614 ) ) ;
#31994=CARTESIAN_POINT ( 'NONE',  ( -71.15374617000810531, 20.66492714610675918, 64.77291441092350510 ) ) ;
#31995=CARTESIAN_POINT ( 'NONE',  ( 211.1200456646896555, 115.5868795682033721, -66.78691274028477665 ) ) ;
#31996=CARTESIAN_POINT ( 'NONE',  ( 42.71247067544611298, 9.879726907348445053, -23.00956250308817275 ) ) ;
#31998=CARTESIAN_POINT ( 'NONE',  ( -73.79615177260656367, 20.52570924097572203, 16.79824538533793543 ) ) ;
#31999=CARTESIAN_POINT ( 'NONE',  ( -120.1650841064594033, 44.02024060322521848, 69.81157495390961287 ) ) ;
#32001=CARTESIAN_POINT ( 'NONE',  ( 23.28809538736929241, 7.864824219997537114, 38.00689959157113407 ) ) ;
#32002=CARTESIAN_POINT ( 'NONE',  ( 199.0123542265578180, 98.86010591893334265, 85.49239298808598164 ) ) ;
#32004=FACE_OUTER_BOUND ( 'NONE', #63836, .T. ) ;
#32012=CARTESIAN_POINT ( 'NONE',  ( -26.88635117726413881, 9.904687797303051155, -63.68164643894200339 ) ) ;
#32013=CARTESIAN_POINT ( 'NONE',  ( 55.76066037845575352, 11.10616952318089545, -45.18587298604916924 ) ) ;
#32017=CARTESIAN_POINT ( 'NONE',  ( -146.1260528621668300, 61.36307454672304118, 4.665803956922211171 ) ) ;
#32021=CARTESIAN_POINT ( 'NONE',  ( -126.3495878770406478, 48.00153794568857535, 45.61994787315711619 ) ) ;
#32024=CARTESIAN_POINT ( 'NONE',  ( 181.0840389613909736, 80.03940679743415387, -89.91415884680696990 ) ) ;
#32025=CARTESIAN_POINT ( 'NONE',  ( 58.48209831743721310, 11.66636741727081805, 70.15205218717414937 ) ) ;
#32029=ORIENTED_EDGE ( 'NONE', *, *, #67134, .T. ) ;
#32032=CARTESIAN_POINT ( 'NONE',  ( -172.7154982671752350, 86.67743928531946551, -22.86740657428632417 ) ) ;
#32034=CARTESIAN_POINT ( 'NONE',  ( 68.63487067129263153, 14.04635751989139258, 42.30428238407001373 ) ) ;
#32035=CARTESIAN_POINT ( 'NONE',  ( 9.446081536138994039, 7.386671790239061508, 87.18713865022354526 ) ) ;
#32037=CARTESIAN_POINT ( 'NONE',  ( -94.79166046756731134, 29.13671350128076654, 65.35457784805571180 ) ) ;
#32039=CARTESIAN_POINT ( 'NONE',  ( -76.31381168750412769, 21.43908608416556660, 45.05567668390800407 ) ) ;
#32043=CARTESIAN_POINT ( 'NONE',  ( 9.058156535714475766, 6.378495712187264743, -46.33800716567037625 ) ) ;
#32044=LINE ( 'NONE', #42261, #67 ) ;
#32045=CARTESIAN_POINT ( 'NONE',  ( 128.9253503890652155, 38.52561778336669818, 58.19870550832551004 ) ) ;
#32052=CARTESIAN_POINT ( 'NONE',  ( 150.5550643769628891, 52.46819381604269239, 33.99397750223288028 ) ) ;
#32058=CARTESIAN_POINT ( 'NONE',  ( -146.7404675333698378, 63.17262273741972223, -62.18289695349267276 ) ) ;
#32060=FACE_BOUND ( 'NONE', #30979, .T. ) ;
#32063=CARTESIAN_POINT ( 'NONE',  ( 113.2864006930874297, 30.31414150890303816, -90.21175991542801853 ) ) ;
#32064=CARTESIAN_POINT ( 'NONE',  ( -120.4666325602655945, 44.20829586446608772, -47.59616471546328142 ) ) ;
#32065=CARTESIAN_POINT ( 'NONE',  ( -85.73740570227380431, 26.23277384689414049, 8.560564749426776032 ) ) ;
#32067=CARTESIAN_POINT ( 'NONE',  ( -150.3898662070191961, 64.92828409760429054, 18.87627064943540134 ) ) ;
#32068=CARTESIAN_POINT ( 'NONE',  ( -75.37104758724677822, 21.09346139657355579, -89.55357651485830672 ) ) ;
#32069=ADVANCED_FACE ( 'NONE', ( #22773 ), #48783, .F. ) ;
#32070=CARTESIAN_POINT ( 'NONE',  ( 63.01563776193091826, 12.67277567978500308, 2.968410348757589023 ) ) ;
#32072=CARTESIAN_POINT ( 'NONE',  ( 45.20420770554357404, 10.25329097499119513, -92.03875038294617639 ) ) ;
#32074=CARTESIAN_POINT ( 'NONE',  ( -36.38071096718370967, 11.47804921491337282, 16.53490236032401839 ) ) ;
#32078=LINE ( 'NONE', #21513, #6226 ) ;
#32083=CARTESIAN_POINT ( 'NONE',  ( 137.3861614007145704, 44.78548268714477132, -36.90154586889402566 ) ) ;
#32084=CARTESIAN_POINT ( 'NONE',  ( -48.23766733091051151, 13.99378332280059212, -66.41992323350672223 ) ) ;
#32087=ORIENTED_EDGE ( 'NONE', *, *, #36448, .F. ) ;
#32100=CARTESIAN_POINT ( 'NONE',  ( -14.76369756425704871, 7.442560416198674034, 67.33920332730103553 ) ) ;
#32101=CARTESIAN_POINT ( 'NONE',  ( -84.22570405563701001, 24.51726571826273826, -10.71275411451128434 ) ) ;
#32104=CARTESIAN_POINT ( 'NONE',  ( 45.04360969585142271, 9.210232288266690048, -11.30927456569269651 ) ) ;
#32105=CARTESIAN_POINT ( 'NONE',  ( -7.825402957745087207, -170.0000000000000000, 71.96013162991091860 ) ) ;
#32106=FACE_OUTER_BOUND ( 'NONE', #9375, .T. ) ;
#32111=ORIENTED_EDGE ( 'NONE', *, *, #2104, .F. ) ;
#32113=CYLINDRICAL_SURFACE ( 'NONE', #59699, 7.500000000000013323 ) ;
#32119=LINE ( 'NONE', #9636, #3330 ) ;
#32123=CARTESIAN_POINT ( 'NONE',  ( 38.10887197045263264, 9.258695140773173904, 83.70795236904210412 ) ) ;
#32125=CARTESIAN_POINT ( 'NONE',  ( 140.3402251947021000, 46.67919788697790295, -93.41835240302059162 ) ) ;
#32126=ORIENTED_EDGE ( 'NONE', *, *, #37814, .T. ) ;
#32128=CARTESIAN_POINT ( 'NONE',  ( 32.28603806442400526, 7.590310383548725781, -18.69525418143827267 ) ) ;
#32129=CARTESIAN_POINT ( 'NONE',  ( 181.0840389613909736, 80.03940679743416808, -51.22505766587963905 ) ) ;
#32131=CARTESIAN_POINT ( 'NONE',  ( 91.49345572560145001, 21.13836538408681776, 31.49813976496750811 ) ) ;
#32134=CARTESIAN_POINT ( 'NONE',  ( -48.23766733091052572, 13.99378332280059212, -39.57537264304307456 ) ) ;
#32138=CARTESIAN_POINT ( 'NONE',  ( 15.78827728214693416, 7.507518794609589818, 30.01470767270522089 ) ) ;
#32141=CIRCLE ( 'NONE', #10796, 242.4895526022646379 ) ;
#32144=ORIENTED_EDGE ( 'NONE', *, *, #43753, .F. ) ;
#32149=CARTESIAN_POINT ( 'NONE',  ( -166.1020662756963588, 81.08306215305039188, 94.67661392444711055 ) ) ;
#32153=EDGE_CURVE ( 'NONE', #16002, #26339, #43864, .T. ) ;
#32157=CARTESIAN_POINT ( 'NONE',  ( -13.77312480593389310, 8.361845410302541026, -20.64904994316430376 ) ) ;
#32158=CARTESIAN_POINT ( 'NONE',  ( 151.7956716830627215, 53.36999433148316285, -65.55858710784085019 ) ) ;
#32159=DIRECTION ( 'NONE',  ( -0.000000000000000000, 1.000000000000000000, -0.000000000000000000 ) ) ;
#32162=CARTESIAN_POINT ( 'NONE',  ( -150.3791492925491582, 64.92185203933371440, -49.77484619116003017 ) ) ;
#32165=CARTESIAN_POINT ( 'NONE',  ( 63.98689050258325750, 13.93365232918668006, -8.923645743953048992 ) ) ;
#32166=CARTESIAN_POINT ( 'NONE',  ( -85.36298448216592760, 26.07611629625834127, -39.20033059854998214 ) ) ;
#32167=CARTESIAN_POINT ( 'NONE',  ( 117.6673027744877658, 32.47081449954681887, 89.68066879645499512 ) ) ;
#32169=CARTESIAN_POINT ( 'NONE',  ( -156.9232798886536955, 72.10386843399172108, 10.21938759049889178 ) ) ;
#32171=CARTESIAN_POINT ( 'NONE',  ( 184.0013086981202832, 81.60415045669144263, -36.80231263419718601 ) ) ;
#32172=CARTESIAN_POINT ( 'NONE',  ( 20.74852474914888845, 6.709938988646749536, 43.16143151702989655 ) ) ;
#32175=VERTEX_POINT ( 'NONE', #55121 ) ;
#32176=ORIENTED_EDGE ( 'NONE', *, *, #57908, .F. ) ;
#32177=CARTESIAN_POINT ( 'NONE',  ( -8.807541152391511474, 6.956521193351526300, 18.22245856944851283 ) ) ;
#32178=CARTESIAN_POINT ( 'NONE',  ( 33.77444274891859521, 8.756048688386682599, -48.08388456350459705 ) ) ;
#32185=EDGE_CURVE ( 'NONE', #46840, #50390, #22335, .T. ) ;
#32187=CARTESIAN_POINT ( 'NONE',  ( -152.9119739516381458, 67.12135129037710612, 58.36714245934808787 ) ) ;
#32188=CARTESIAN_POINT ( 'NONE',  ( 21.44191228441539465, 7.755009954762318358, 5.717230818571867879 ) ) ;
#32191=CARTESIAN_POINT ( 'NONE',  ( -85.09761763353364472, 24.87634954265998388, -38.74851144219385191 ) ) ;
#32192=CARTESIAN_POINT ( 'NONE',  ( 22.53041628628729143, 6.810083298012985509, 67.68129265094559344 ) ) ;
#32194=CARTESIAN_POINT ( 'NONE',  ( 13.84120792123769128, 6.445822122644895735, -77.12289573830005907 ) ) ;
#32200=CARTESIAN_POINT ( 'NONE',  ( 174.9042454172880525, 72.57746269938725447, 41.08881398978587640 ) ) ;
#32201=CARTESIAN_POINT ( 'NONE',  ( -129.6165111262477296, 48.99406349865699895, -48.92884824319389736 ) ) ;
#32202=CARTESIAN_POINT ( 'NONE',  ( 43.96465529479667822, 9.046527005589323878, -75.93720877633131749 ) ) ;
#32208=CARTESIAN_POINT ( 'NONE',  ( -29.49620345460275317, 9.280093073089039635, -8.712006218224214393 ) ) ;
#32209=CARTESIAN_POINT ( 'NONE',  ( 197.2199569260504006, 98.22436319491367840, 10.52695052019480570 ) ) ;
#32212=CARTESIAN_POINT ( 'NONE',  ( 150.6633721218480275, 53.78936049964467259, 93.76803445655194480 ) ) ;
#32214=CARTESIAN_POINT ( 'NONE',  ( 127.2107679985236217, 38.70844091144995502, -66.85294649915745424 ) ) ;
#32216=CARTESIAN_POINT ( 'NONE',  ( 136.9822423813093337, 44.53121110416874018, 57.03315645636024556 ) ) ;
#32217=CARTESIAN_POINT ( 'NONE',  ( 110.2429982417149432, 29.99119854320847267, 2.766663615273645682 ) ) ;
#32218=CARTESIAN_POINT ( 'NONE',  ( 163.9881357112706723, 62.90166026738586424, -93.59647863210024354 ) ) ;
#32219=CARTESIAN_POINT ( 'NONE',  ( 94.12988949694084795, 22.11811104795076588, -43.08587400594926464 ) ) ;
#32222=ORIENTED_EDGE ( 'NONE', *, *, #17625, .T. ) ;
#32223=CARTESIAN_POINT ( 'NONE',  ( -166.5742238910466142, 81.57147158222488770, 7.807693272540740637 ) ) ;
#32226=CARTESIAN_POINT ( 'NONE',  ( -177.1540936177023582, 91.73126115633628785, -21.70593551934987886 ) ) ;
#32227=CARTESIAN_POINT ( 'NONE',  ( -165.7149569557575433, 80.68479365246972179, -67.83569924512404725 ) ) ;
#32230=CARTESIAN_POINT ( 'NONE',  ( 55.51637278631174865, 12.08345311280958789, 9.958762847333103352 ) ) ;
#32232=CARTESIAN_POINT ( 'NONE',  ( -128.7650348665116837, 48.41336321950710442, 45.05237689147213587 ) ) ;
#32234=EDGE_CURVE ( 'NONE', #46420, #52493, #24837, .T. ) ;
#32236=ADVANCED_FACE ( 'NONE', ( #9374 ), #53643, .F. ) ;
#32237=CARTESIAN_POINT ( 'NONE',  ( 84.27368848767928000, 18.63026910897604438, -23.61379479314351570 ) ) ;
#32239=CARTESIAN_POINT ( 'NONE',  ( 93.70675391435743506, 21.95852801827563283, -72.66083171198076229 ) ) ;
#32242=CARTESIAN_POINT ( 'NONE',  ( -154.7844486873554217, 68.78754123322237035, -90.65283450566464296 ) ) ;
#32244=ORIENTED_EDGE ( 'NONE', *, *, #40760, .T. ) ;
#32247=CARTESIAN_POINT ( 'NONE',  ( 187.5272808203428099, 85.37192123373904451, -74.44646421899427935 ) ) ;
#32253=CARTESIAN_POINT ( 'NONE',  ( -73.10086105983764071, 21.34631349770505082, -64.40865245798021022 ) ) ;
#32256=CARTESIAN_POINT ( 'NONE',  ( 46.90170507415071199, 10.52318308703818239, -42.62448673664831489 ) ) ;
#32257=CARTESIAN_POINT ( 'NONE',  ( 210.6741002223296562, 114.9147155784838219, 68.09108095163148278 ) ) ;
#32259=CARTESIAN_POINT ( 'NONE',  ( -109.5025362253418706, 36.60371748273998094, -13.58337307779724767 ) ) ;
#32261=CARTESIAN_POINT ( 'NONE',  ( -8.320652113663529192, 6.923290556636830573, -35.41807073194381417 ) ) ;
#32263=CARTESIAN_POINT ( 'NONE',  ( -85.69951099329024657, 25.12635487938836931, 88.98224730508108848 ) ) ;
#32264=CARTESIAN_POINT ( 'NONE',  ( 91.67776154311749792, 22.27748043241297538, 69.60850208772687608 ) ) ;
#32265=CARTESIAN_POINT ( 'NONE',  ( 150.7926588734435427, 52.63999027731881597, -13.35493234247606154 ) ) ;
#32266=CARTESIAN_POINT ( 'NONE',  ( 31.95163392065794739, 8.568192436298476267, 9.577667117831884624 ) ) ;
#32267=CARTESIAN_POINT ( 'NONE',  ( -96.02159028238561689, 30.82695531378849196, -65.21878469105446641 ) ) ;
#32272=CARTESIAN_POINT ( 'NONE',  ( 211.7624483073558110, 116.5638334585939333, 92.92243069068229033 ) ) ;
#32273=CARTESIAN_POINT ( 'NONE',  ( 8.000000000000007105, 249.8719672152120381, 94.99999999999866418 ) ) ;
#32278=CARTESIAN_POINT ( 'NONE',  ( 46.90170507415071910, 10.52318308703818062, -69.46903732711203361 ) ) ;
#32281=CARTESIAN_POINT ( 'NONE',  ( 80.34841469379381351, 18.42674688750400946, 94.99999999999866418 ) ) ;
#32284=CARTESIAN_POINT ( 'NONE',  ( -190.4968431727838833, 108.8425311198514720, -19.44418843322370805 ) ) ;
#32285=CARTESIAN_POINT ( 'NONE',  ( -130.6002960060536964, 49.67125682092490990, 5.415878727382473556 ) ) ;
#32286=CARTESIAN_POINT ( 'NONE',  ( -103.2061297292849531, 34.38496953192504435, 57.40642899071801963 ) ) ;
#32287=CARTESIAN_POINT ( 'NONE',  ( -132.4896623150434323, 52.22616402022728721, -38.83446270130018974 ) ) ;
#32288=ORIENTED_EDGE ( 'NONE', *, *, #25989, .T. ) ;
#32289=FACE_OUTER_BOUND ( 'NONE', #32831, .T. ) ;
#32290=CARTESIAN_POINT ( 'NONE',  ( 93.63037639125413136, 21.92981100938040484, 66.75823669843309460 ) ) ;
#32292=B_SPLINE_CURVE_WITH_KNOTS ( 'NONE', 3,
 ( #20612, #64215, #31870, #38174, #42072, #189, #69141, #59616, #15690, #11430, #21647, #63536, #59276, #37482, #11094, #5477, #32557, #53299, #15350, #42420, #63880, #53987, #10066, #32219, #37138, #5812, #27266, #48706, #58582, #36806, #31526, #26590, #48027, #60332, #12153, #43787, #39920, #22696, #49760, #49063, #12856, #33619, #55047, #38525, #2300, #1244 ),
 .UNSPECIFIED., .F., .F.,
 ( 4, 2, 2, 2, 2, 2, 2, 2, 2, 2, 2, 2, 2, 2, 2, 2, 2, 2, 2, 2, 2, 2, 4 ),
 ( 0.02404638330965502488, 0.02555608299537557443, 0.02631093283823585441, 0.02706578268109613092, 0.02857548236681668741, 0.02933033220967695698, 0.03008518205253722655, 0.03159488173825776569, 0.03310458142397830483, 0.03385943126683858134, 0.03461428110969885785, 0.03612398079541943863, 0.03687883063827972208, 0.03763368048114001246, 0.03838853032400030285, 0.03914338016686058630, 0.04065307985258116708, 0.04216277953830173397, 0.04367247922402230781, 0.04518217890974288165, 0.04593702875260315122, 0.04669187859546342079, 0.04820157828118395993 ),
 .UNSPECIFIED. ) ;
#32294=CARTESIAN_POINT ( 'NONE',  ( -149.0738659721762076, 63.81256528267484640, 84.41759755226209450 ) ) ;
#32297=CARTESIAN_POINT ( 'NONE',  ( 140.9169160367233076, 45.85398962664667977, 39.59428667614358233 ) ) ;
#32298=ORIENTED_EDGE ( 'NONE', *, *, #49351, .T. ) ;
#32300=CARTESIAN_POINT ( 'NONE',  ( 79.22872707466396491, 18.07970189365808622, 11.61010380891110572 ) ) ;
#32303=DIRECTION ( 'NONE',  ( 0.000000000000000000, 0.000000000000000000, 1.000000000000000000 ) ) ;
#32309=CARTESIAN_POINT ( 'NONE',  ( -73.63346300764936814, 20.46798018699518451, -21.33674241584527920 ) ) ;
#32311=CARTESIAN_POINT ( 'NONE',  ( 70.26722489419888973, 14.47234958177330455, -72.04276696937047575 ) ) ;
#32315=CARTESIAN_POINT ( 'NONE',  ( 164.9709596662455056, 63.72607097915132357, 37.17312740752070965 ) ) ;
#32318=VERTEX_POINT ( 'NONE', #22690 ) ;
#32322=CARTESIAN_POINT ( 'NONE',  ( -166.7049310409072405, 80.25944422923581101, 42.21435027861289768 ) ) ;
#32323=CARTESIAN_POINT ( 'NONE',  ( 133.4058733589413634, 42.32720528873925048, 56.35489142945903751 ) ) ;
#32329=FACE_OUTER_BOUND ( 'NONE', #1389, .T. ) ;
#32330=CARTESIAN_POINT ( 'NONE',  ( -107.0544991134679691, 36.41543129049375693, 5.385398075284562047 ) ) ;
#32332=CARTESIAN_POINT ( 'NONE',  ( -156.4841188516943191, 70.33041971808555104, -71.92384636904367312 ) ) ;
#32334=CARTESIAN_POINT ( 'NONE',  ( 69.36122620657974380, 14.23458312296499528, 94.99999999999866418 ) ) ;
#32338=ORIENTED_EDGE ( 'NONE', *, *, #35097, .T. ) ;
#32343=CARTESIAN_POINT ( 'NONE',  ( 211.7419975634645368, 116.5322580952101532, -73.32492906585233072 ) ) ;
#32348=CARTESIAN_POINT ( 'NONE',  ( 23.09590709048883994, 7.852755081912510704, 39.22044207619089917 ) ) ;
#32349=CARTESIAN_POINT ( 'NONE',  ( 197.8045642144698206, 97.34517417643259307, 93.35912461664177897 ) ) ;
#32351=LINE ( 'NONE', #48153, #33330 ) ;
#32352=ORIENTED_EDGE ( 'NONE', *, *, #60104, .F. ) ;
#32357=VERTEX_POINT ( 'NONE', #65617 ) ;
#32358=CARTESIAN_POINT ( 'NONE',  ( -29.50439180771548564, 10.29976981300624850, -76.92427033250436352 ) ) ;
#32359=CARTESIAN_POINT ( 'NONE',  ( 58.09436971064712907, 11.58462396079456980, -37.53989357320173781 ) ) ;
#32360=CARTESIAN_POINT ( 'NONE',  ( -24.32937228292060894, 8.531905774118440533, 62.12288946467717210 ) ) ;
#32363=B_SPLINE_CURVE_WITH_KNOTS ( 'NONE', 3,
 ( #38786, #45088, #50382, #50024, #34208, #12398, #28572, #1858, #55644, #2198, #2537, #66574, #34566, #31006, #30655, #4269, #46131, #57385, #29606, #40509, #66921, #18716, #57047, #56341, #19057, #14127, #61957, #62312, #41553, #14477, #61625, #46474, #34902, #2885, #62670, #36273, #25040, #13777, #35237, #56692, #24694, #63007, #30312, #40168, #35933 ),
 .UNSPECIFIED., .F., .F.,
 ( 4, 2, 2, 2, 2, 2, 2, 2, 2, 2, 2, 1, 2, 2, 2, 2, 2, 2, 2, 2, 2, 2, 4 ),
 ( 1.430489624538199204E-17, 0.001502898956853363811, 0.002254348435280040513, 0.003005797913706716781, 0.004508696870560108781, 0.005260146348986821478, 0.006011595827413535043, 0.007514494784267020284, 0.009017393741120507261, 0.01052029269797399164, 0.01127174217640075117, 0.01202319165482751070, 0.01277464113325426677, 0.01352609061168102457, 0.01502898956853450201, 0.01578043904696122338, 0.01653188852538794301, 0.01803478748224135106, 0.01953768643909475911, 0.02028913591752146486, 0.02104058539594816715, 0.02254348435280160989, 0.02404638330965504917 ),
 .UNSPECIFIED. ) ;
#32365=VERTEX_POINT ( 'NONE', #49409 ) ;
#32366=CARTESIAN_POINT ( 'NONE',  ( -128.9863978264385196, 49.78205252558957739, 44.95660336865451967 ) ) ;
#32367=ORIENTED_EDGE ( 'NONE', *, *, #39061, .T. ) ;
#32369=CARTESIAN_POINT ( 'NONE',  ( -142.8492950481059438, 60.01492924994603584, 34.75812731920188270 ) ) ;
#32370=CARTESIAN_POINT ( 'NONE',  ( 55.90536342106781831, 11.13510150712953362, 61.72041802730606719 ) ) ;
#32379=CARTESIAN_POINT ( 'NONE',  ( -171.4814970982679938, 85.32124710276288226, -8.037032661340148820 ) ) ;
#32380=FACE_OUTER_BOUND ( 'NONE', #52321, .T. ) ;
#32381=CARTESIAN_POINT ( 'NONE',  ( 70.51601918574517924, 14.53832276813547608, 37.55138390113663149 ) ) ;
#32382=CARTESIAN_POINT ( 'NONE',  ( 8.621086886543794847, 7.383195413572584798, 88.96999900602391165 ) ) ;
#32387=CARTESIAN_POINT ( 'NONE',  ( 82.14449817946437804, 17.93919511903896336, 16.38389564114189412 ) ) ;
#32391=CARTESIAN_POINT ( 'NONE',  ( -75.64857587248467041, 21.19501514561449440, 44.78839637111028082 ) ) ;
#32396=CARTESIAN_POINT ( 'NONE',  ( -121.5680658099884113, 44.89994870382101055, 5.130273036901130901 ) ) ;
#32397=CARTESIAN_POINT ( 'NONE',  ( -179.0654441437004323, 93.99779465816534696, 60.58611069645034775 ) ) ;
#32398=DIRECTION ( 'NONE',  ( -0.8118923937861950435, -0.5838071093367415143, 0.000000000000000000 ) ) ;
#32400=CARTESIAN_POINT ( 'NONE',  ( 157.4703587214989113, 57.65129005721576050, -9.279633708673953763 ) ) ;
#32401=CARTESIAN_POINT ( 'NONE',  ( 151.6351261592328683, 53.25263237790399273, 41.62792433286728766 ) ) ;
#32402=CARTESIAN_POINT ( 'NONE',  ( 69.49112875363883290, 15.30845942322121367, 33.52089747499180561 ) ) ;
#32407=CARTESIAN_POINT ( 'NONE',  ( 136.9654665832767932, 44.52067472585214603, -63.53847950313026871 ) ) ;
#32408=CARTESIAN_POINT ( 'NONE',  ( -142.3187766126154941, 59.59460822661993973, -71.36695520502316015 ) ) ;
#32410=VERTEX_POINT ( 'NONE', #39229 ) ;
#32411=FACE_BOUND ( 'NONE', #18407, .T. ) ;
#32412=CARTESIAN_POINT ( 'NONE',  ( -5.885876544836655455, 6.772369038004113939, -77.01165322372530397 ) ) ;
#32413=CARTESIAN_POINT ( 'NONE',  ( -179.2128128997734109, 95.75254520622991095, 60.76269154493880364 ) ) ;
#32415=CARTESIAN_POINT ( 'NONE',  ( -118.4106078162223668, 42.93830006159888768, -41.84395280496732283 ) ) ;
#32416=CARTESIAN_POINT ( 'NONE',  ( -82.32006615997345023, 24.83050031643766431, 4.505854562011677444 ) ) ;
#32418=CARTESIAN_POINT ( 'NONE',  ( -153.5002794404625774, 67.64160439471098130, 5.023374128941582306 ) ) ;
#32419=CARTESIAN_POINT ( 'NONE',  ( -6.843910203392212566, 7.836697961436722260, -8.622009400863452910 ) ) ;
#32420=CARTESIAN_POINT ( 'NONE',  ( 70.38121398871578549, 14.50253776029980557, 11.94555559055825711 ) ) ;
#32421=CARTESIAN_POINT ( 'NONE',  ( -86.16710354151693707, 26.41338104675949339, 64.99724543193327975 ) ) ;
#32422=CARTESIAN_POINT ( 'NONE',  ( 91.11019107624154856, 22.06959540317787827, -10.45776451510279159 ) ) ;
#32424=CARTESIAN_POINT ( 'NONE',  ( -35.17296606710972640, 11.25626711331309160, 4.348805324083214074 ) ) ;
#32427=ORIENTED_EDGE ( 'NONE', *, *, #62455, .T. ) ;
#32428=CARTESIAN_POINT ( 'NONE',  ( 19.54326199789021246, 7.657220834818548205, -76.36046258218678418 ) ) ;
#32429=CARTESIAN_POINT ( 'NONE',  ( 108.6949225693525847, 29.27769766909357330, 83.45484555132844662 ) ) ;
#32430=CARTESIAN_POINT ( 'NONE',  ( -146.5230751932348596, 62.99205605665029850, 58.17019016430769796 ) ) ;
#32431=CARTESIAN_POINT ( 'NONE',  ( 68.95451040317564662, 14.12887482153123031, -11.76939062271155656 ) ) ;
#32432=CARTESIAN_POINT ( 'NONE',  ( -29.03891846981456126, 10.22741474064059020, -49.93962856602705358 ) ) ;
#32433=CARTESIAN_POINT ( 'NONE',  ( 208.0011962801381458, 112.7551321982796111, -90.77262215979118309 ) ) ;
#32434=CARTESIAN_POINT ( 'NONE',  ( -71.48055013538424873, 20.77798539480599160, -94.11067968272816131 ) ) ;
#32435=CARTESIAN_POINT ( 'NONE',  ( -124.9915686518654638, 47.10215472274616388, -8.069153307770244865 ) ) ;
#32438=CARTESIAN_POINT ( 'NONE',  ( 37.45439421541016145, 9.177432671831372346, 71.51784865638920508 ) ) ;
#32439=CARTESIAN_POINT ( 'NONE',  ( -173.1211646369891355, 88.63826465341152527, 72.66624519710475738 ) ) ;
#32446=CARTESIAN_POINT ( 'NONE',  ( 188.4374648754671284, 87.87346242052439038, -18.38533621105863958 ) ) ;
#32450=CARTESIAN_POINT ( 'NONE',  ( 209.4789161463551181, 113.1367444519304115, -22.76410597263823377 ) ) ;
#32452=CARTESIAN_POINT ( 'NONE',  ( -149.5074843970971301, -170.0000000000000000, 3.876270649435373805 ) ) ;
#32454=DIRECTION ( 'NONE',  ( -0.000000000000000000, 0.000000000000000000, -1.000000000000000000 ) ) ;
#32456=CARTESIAN_POINT ( 'NONE',  ( -48.71337292867759317, 14.10768470390587659, 68.67724857654715720 ) ) ;
#32458=DIRECTION ( 'NONE',  ( 0.000000000000000000, 0.000000000000000000, 1.000000000000000000 ) ) ;
#32461=CARTESIAN_POINT ( 'NONE',  ( 61.33627421985470818, 12.28939706835343237, 17.78195680140521162 ) ) ;
#32466=CARTESIAN_POINT ( 'NONE',  ( 46.90632335736349745, 10.52393368783804561, 90.89396992506641482 ) ) ;
#32469=CARTESIAN_POINT ( 'NONE',  ( 103.8093541423578898, 26.01745837747064982, 33.22445973737408309 ) ) ;
#32471=CARTESIAN_POINT ( 'NONE',  ( -62.30463872474476972, 16.74658165105247321, -71.53854161899334940 ) ) ;
#32473=CARTESIAN_POINT ( 'NONE',  ( 32.56927464314650678, 7.618924692399903442, -19.37770249060224614 ) ) ;
#32474=CARTESIAN_POINT ( 'NONE',  ( 175.5498284945444709, 74.57669191966280664, -48.81277339523749959 ) ) ;
#32475=CARTESIAN_POINT ( 'NONE',  ( 164.6177656728407044, 63.42876281302249453, 88.29515807379765135 ) ) ;
#32478=CARTESIAN_POINT ( 'NONE',  ( -50.14523569787233725, 14.45648954445650780, -48.40948618845168738 ) ) ;
#32480=CARTESIAN_POINT ( 'NONE',  ( 11.20486344102687326, 7.403248964808830657, 43.47161425690537584 ) ) ;
#32483=CIRCLE ( 'NONE', #61714, 242.4895526022646379 ) ;
#32485=CARTESIAN_POINT ( 'NONE',  ( -85.35521056349260505, 26.07297753498038873, 94.99999999999866418 ) ) ;
#32487=ORIENTED_EDGE ( 'NONE', *, *, #52728, .T. ) ;
#32490=VERTEX_POINT ( 'NONE', #46221 ) ;
#32491=CARTESIAN_POINT ( 'NONE',  ( -14.66033866466834823, 7.432913330382389105, -19.17095739190610004 ) ) ;
#32492=FACE_OUTER_BOUND ( 'NONE', #24686, .T. ) ;
#32495=CARTESIAN_POINT ( 'NONE',  ( -36.38071096718371678, 11.47804921491337993, 70.22400354125137767 ) ) ;
#32496=CARTESIAN_POINT ( 'NONE',  ( -11.56945424397728672, 8.173256823723106024, -22.57675618948779217 ) ) ;
#32498=CARTESIAN_POINT ( 'NONE',  ( 16.77391662606470391, 6.533867394142986562, -8.723007401148960227 ) ) ;
#32500=CARTESIAN_POINT ( 'NONE',  ( 63.01563776193091826, -170.0000000000000000, -16.37614024170606797 ) ) ;
#32503=CARTESIAN_POINT ( 'NONE',  ( 67.55199883153193241, 14.80832170058782715, -22.36842963500835069 ) ) ;
#32505=CARTESIAN_POINT ( 'NONE',  ( -24.14271535429456605, 9.522144728394469126, 89.63976553000811975 ) ) ;
#32507=CARTESIAN_POINT ( 'NONE',  ( -157.0079874970173535, 72.18249880494043680, 11.64991257542693859 ) ) ;
#32510=CARTESIAN_POINT ( 'NONE',  ( -156.2646585454849344, 71.49501546611418235, 88.63874933570780001 ) ) ;
#32516=CARTESIAN_POINT ( 'NONE',  ( -38.15923928782688535, 10.79140400702258695, 67.90023288991038442 ) ) ;
#32518=CARTESIAN_POINT ( 'NONE',  ( 197.2847860006354495, 98.30530166401517533, 62.40104121888823130 ) ) ;
#32520=CARTESIAN_POINT ( 'NONE',  ( 188.4918087359956189, 87.93403732562654795, 62.44201370830596431 ) ) ;
#32521=CARTESIAN_POINT ( 'NONE',  ( -153.6931187576189188, 67.81270084382354923, 58.83762594297919435 ) ) ;
#32525=CARTESIAN_POINT ( 'NONE',  ( 103.8317086684999992, 26.02720265156212776, 14.16654748491671256 ) ) ;
#32534=CARTESIAN_POINT ( 'NONE',  ( 179.4207200232660853, 76.93724985992177778, 44.17255298202294256 ) ) ;
#32535=CARTESIAN_POINT ( 'NONE',  ( -133.0808647576834289, 51.41195281028756625, -40.25360747411231443 ) ) ;
#32538=CARTESIAN_POINT ( 'NONE',  ( 181.9295958320008708, 80.90438706151873305, -51.18938441524608152 ) ) ;
#32539=ORIENTED_EDGE ( 'NONE', *, *, #10463, .T. ) ;
#32542=CARTESIAN_POINT ( 'NONE',  ( -78.66644367742111399, -170.0000000000000000, 72.26275173013684139 ) ) ;
#32543=CARTESIAN_POINT ( 'NONE',  ( 174.8714394078361352, 72.54688047260668782, 94.71445689663468670 ) ) ;
#32545=ORIENTED_EDGE ( 'NONE', *, *, #7043, .F. ) ;
#32549=VERTEX_POINT ( 'NONE', #24783 ) ;
#32550=CARTESIAN_POINT ( 'NONE',  ( 117.3145357257065911, 33.41973663092564806, 66.50590971767826431 ) ) ;
#32552=CARTESIAN_POINT ( 'NONE',  ( 141.1220430186942565, 47.19066702031173577, 65.73481338491475867 ) ) ;
#32553=CARTESIAN_POINT ( 'NONE',  ( -71.22878586122430988, 19.62649588091171893, -41.61736384448404635 ) ) ;
#32556=CARTESIAN_POINT ( 'NONE',  ( 86.23158543793178410, 19.28538367132613374, -89.51066537983908233 ) ) ;
#32557=CARTESIAN_POINT ( 'NONE',  ( 93.32502112557683915, 21.81526022999039327, -46.73702075745129036 ) ) ;
#32558=B_SPLINE_CURVE_WITH_KNOTS ( 'NONE', 3,
 ( #2007, #3042, #66383, #2347, #39971, #55808, #44901, #8317, #24504, #7630, #46275, #19196, #40657, #67752, #19552, #26212, #41699, #52592, #57194, #47303, #42041, #4075, #14620, #36422, #30454, #30806, #68764, #14957, #25539, #41012, #68101, #25193, #15313, #46975, #47652, #46626, #20931, #10035, #26557, #63164, #4749, #31832, #31162, #9012, #5097 ),
 .UNSPECIFIED., .F., .F.,
 ( 4, 2, 2, 2, 2, 2, 2, 2, 1, 2, 2, 2, 2, 2, 2, 2, 2, 2, 2, 2, 2, 2, 4 ),
 ( 0.000000000000000000, 0.001470449819620697676, 0.002205674729431036755, 0.002940899639241375402, 0.004411349458862033612, 0.005881799278482692690, 0.007352249098103350901, 0.008087474007913679139, 0.008822698917724009979, 0.009557923827534337349, 0.01029314873734466819, 0.01176359855696528650, 0.01249882346677559479, 0.01323404837658590308, 0.01470449819620656823, 0.01543972310601690427, 0.01617494801582724032, 0.01764539783544789159, 0.01911584765506854633, 0.01985107256487888411, 0.02058629747468921842, 0.02205674729430988704, 0.02352719711393055566 ),
 .UNSPECIFIED. ) ;
#32560=B_SPLINE_CURVE_WITH_KNOTS ( 'NONE', 3,
 ( #37902, #7289, #22763, #54053, #59683, #1311, #43511, #22069, #16783, #28385, #17120, #32972, #60401, #12564, #5877, #59349, #65690, #17479, #49127, #50196, #38958, #54405, #12216, #44572, #33684, #28744, #27336, #38597, #21716, #55113, #43162, #64637, #16450, #11160, #48774, #6935, #49832, #6230, #17842, #32626, #612, #968, #22417, #43856, #65332, #60039 ),
 .UNSPECIFIED., .F., .F.,
 ( 4, 2, 2, 2, 2, 2, 2, 2, 2, 2, 2, 2, 2, 2, 2, 2, 2, 2, 2, 2, 2, 2, 4 ),
 ( 1.387778780781445676E-17, 0.003635178948345826107, 0.005452768422518705117, 0.007270357896691583693, 0.008179152633778011272, 0.009087947370864437116, 0.01090553684503733911, 0.01181433158212381353, 0.01272312631921028968, 0.01363192105629676409, 0.01454071579338324025, 0.01544951053046971640, 0.01635830526755619255, 0.01726710000464266523, 0.01817589474172914138, 0.01908468947881561753, 0.01999348421590209368, 0.02090227895298856983, 0.02181107369007504251, 0.02362866316424793584, 0.02544625263842082569, 0.02726384211259371554, 0.02908143158676660886 ),
 .UNSPECIFIED. ) ;
#32561=ORIENTED_EDGE ( 'NONE', *, *, #54469, .F. ) ;
#32566=CARTESIAN_POINT ( 'NONE',  ( -142.8556048422594813, 60.01994222009839319, -38.83800050151604921 ) ) ;
#32567=CARTESIAN_POINT ( 'NONE',  ( -167.6566265204789943, 82.70140535081095834, -63.91361994493567522 ) ) ;
#32568=CARTESIAN_POINT ( 'NONE',  ( -143.7151964745329451, 59.41799441280377891, -47.08409988814416636 ) ) ;
#32570=CYLINDRICAL_SURFACE ( 'NONE', #504, 7.500000000000013323 ) ;
#32575=CARTESIAN_POINT ( 'NONE',  ( -142.1381007084227122, 58.17237452544241449, 63.64461756446542040 ) ) ;
#32578=CARTESIAN_POINT ( 'NONE',  ( 82.34195123877073286, 18.00239921638039675, -10.31852367068890430 ) ) ;
#32579=CARTESIAN_POINT ( 'NONE',  ( 91.67571176799441446, 21.20498955963029530, -75.71976116502800380 ) ) ;
#32580=CARTESIAN_POINT ( 'NONE',  ( 203.1511228994173734, 104.2426341584999250, 2.478373221329412068 ) ) ;
#32582=CARTESIAN_POINT ( 'NONE',  ( -96.00016893459645928, 29.70347032303886436, -65.25124674057008178 ) ) ;
#32584=ORIENTED_EDGE ( 'NONE', *, *, #25906, .F. ) ;
#32585=VECTOR ( 'NONE', #43572, 1000.000000000000000 ) ;
#32586=CARTESIAN_POINT ( 'NONE',  ( 186.2722199822849802, 84.01218714714249813, -65.13350658560696615 ) ) ;
#32591=LINE ( 'NONE', #26279, #42282 ) ;
#32592=CARTESIAN_POINT ( 'NONE',  ( 81.57482918025355900, 17.75786713398421668, 42.75847996119852468 ) ) ;
#32594=CARTESIAN_POINT ( 'NONE',  ( 39.89582146299186860, 9.488756994579082615, -35.61981746542775795 ) ) ;
#32597=CARTESIAN_POINT ( 'NONE',  ( -25.48750459758502274, 9.705678256319574260, 6.281801299306986053 ) ) ;
#32599=CARTESIAN_POINT ( 'NONE',  ( -13.47680110791658059, 7.324966777230639714, -47.87354606939886281 ) ) ;
#32601=DIRECTION ( 'NONE',  ( -0.000000000000000000, 1.000000000000000000, -0.000000000000000000 ) ) ;
#32602=B_SPLINE_CURVE_WITH_KNOTS ( 'NONE', 3,
 ( #37530, #10798, #8315, #38940, #34708, #12546, #29761, #50177, #3040, #61427, #35045, #24149, #2346, #34363, #55093, #44899, #61079, #45938, #7274, #55441, #2683, #44554, #55806, #28727, #45591, #67072, #23799, #39284, #66382, #2006, #12904, #60386, #56145, #39624, #34006, #6918 ),
 .UNSPECIFIED., .F., .F.,
 ( 4, 2, 2, 2, 2, 2, 2, 2, 2, 2, 2, 2, 2, 2, 2, 2, 2, 4 ),
 ( 1.734723475976807094E-18, 0.001548367318450188240, 0.003096734636900374746, 0.004645101955350561251, 0.006193469273800747757, 0.007741836592250927324, 0.008516020251476004096, 0.009290203910701080869, 0.01083857122915123268, 0.01238693854760138449, 0.01393530586605153804, 0.01548367318450169158, 0.01703204050295184513, 0.01858040782140199521, 0.02012877513985214528, 0.02167714245830229536, 0.02322550977675244543, 0.02477387709520258857 ),
 .UNSPECIFIED. ) ;
#32603=CARTESIAN_POINT ( 'NONE',  ( 152.8430172091323129, 54.14068524174420816, -22.68681308951628850 ) ) ;
#32605=CARTESIAN_POINT ( 'NONE',  ( -97.86516199987806885, 31.71158167298307617, -75.44090550092165870 ) ) ;
#32608=ORIENTED_EDGE ( 'NONE', *, *, #56294, .F. ) ;
#32612=ORIENTED_EDGE ( 'NONE', *, *, #50686, .T. ) ;
#32613=CARTESIAN_POINT ( 'NONE',  ( 56.29445224195349340, 12.24017809212663010, 60.79306025269804792 ) ) ;
#32615=CARTESIAN_POINT ( 'NONE',  ( -27.48703802937315288, 8.975952825337598640, 17.25091243039942057 ) ) ;
#32617=CARTESIAN_POINT ( 'NONE',  ( -0.7174461528505738928, 6.532311451815524528, 40.02128953067827410 ) ) ;
#32618=CARTESIAN_POINT ( 'NONE',  ( -105.4556185321791162, 34.42302275449792859, -62.54804870380231563 ) ) ;
#32619=CARTESIAN_POINT ( 'NONE',  ( 80.86930862966734423, 18.59011988975001728, 86.08600358295961996 ) ) ;
#32620=EDGE_CURVE ( 'NONE', #61020, #33777, #62054, .T. ) ;
#32624=DIRECTION ( 'NONE',  ( 0.000000000000000000, 0.000000000000000000, 1.000000000000000000 ) ) ;
#32625=CARTESIAN_POINT ( 'NONE',  ( -126.3508039230932809, 46.79479538767115798, 18.77539728269342234 ) ) ;
#32626=CARTESIAN_POINT ( 'NONE',  ( -169.8885678771098071, 85.07765565657317097, -48.99404913829265951 ) ) ;
#32628=CARTESIAN_POINT ( 'NONE',  ( -130.1938957973835329, 50.61368074696266461, -48.57623976542650013 ) ) ;
#32631=CARTESIAN_POINT ( 'NONE',  ( -3.857727530059801513, 6.665032499723450243, -9.704207997736320479 ) ) ;
#32633=CARTESIAN_POINT ( 'NONE',  ( -156.7916867929804994, 70.61267366697164505, 93.72828952245049550 ) ) ;
#32639=CARTESIAN_POINT ( 'NONE',  ( 82.14396250120408638, 18.99560174459422157, 4.351623306195690155 ) ) ;
#32642=CARTESIAN_POINT ( 'NONE',  ( 174.6242782760050147, 73.69713439533578025, 67.47305218060527920 ) ) ;
#32645=CARTESIAN_POINT ( 'NONE',  ( 179.0091171455096912, 77.94933395983139235, 29.58847966245846095 ) ) ;
#32646=FACE_OUTER_BOUND ( 'NONE', #5049, .T. ) ;
#32647=FACE_OUTER_BOUND ( 'NONE', #20139, .T. ) ;
#32649=CARTESIAN_POINT ( 'NONE',  ( 163.7464701930790341, 62.69993100427431898, 32.77245788678815330 ) ) ;
#32651=CARTESIAN_POINT ( 'NONE',  ( 8.000000000000007105, 249.8719672152120381, 94.99999999999866418 ) ) ;
#32657=( GEOMETRIC_REPRESENTATION_CONTEXT ( 3 ) GLOBAL_UNCERTAINTY_ASSIGNED_CONTEXT ( ( #52169 ) ) GLOBAL_UNIT_ASSIGNED_CONTEXT ( ( #7025, #40080, #61536 ) ) REPRESENTATION_CONTEXT ( 'NONE', 'WORKASPACE' ) );
#32659=CARTESIAN_POINT ( 'NONE',  ( -144.7329995847092050, 61.52689957297653223, -90.21374520017691623 ) ) ;
#32661=CARTESIAN_POINT ( 'NONE',  ( -33.13098007862451055, 9.875138601866705557, -8.661938437730437812 ) ) ;
#32662=CARTESIAN_POINT ( 'NONE',  ( -178.5750994113944898, 94.98114813978521909, 33.14926202597649763 ) ) ;
#32663=CARTESIAN_POINT ( 'NONE',  ( 132.2818448028687328, 41.65267246304671289, 56.51853981166434693 ) ) ;
#32664=VERTEX_POINT ( 'NONE', #52200 ) ;
#32665=VERTEX_POINT ( 'NONE', #10313 ) ;
#32669=CARTESIAN_POINT ( 'NONE',  ( -48.07236379518559488, 12.92027279314125288, 88.68666546384376659 ) ) ;
#32671=CARTESIAN_POINT ( 'NONE',  ( -154.7998111145352880, 68.80117179139331540, -74.49316838609406943 ) ) ;
#32672=CARTESIAN_POINT ( 'NONE',  ( 70.39075050212761653, 14.50499482275434460, 92.52271767195246355 ) ) ;
#32678=ORIENTED_EDGE ( 'NONE', *, *, #1920, .F. ) ;
#32680=CARTESIAN_POINT ( 'NONE',  ( 183.1865184929770294, 80.75677158533821398, 29.60613287127756621 ) ) ;
#32682=CARTESIAN_POINT ( 'NONE',  ( -71.59086462055192612, 19.75139532313339785, 8.573663426099198404 ) ) ;
#32685=CARTESIAN_POINT ( 'NONE',  ( 200.7308788951040697, 101.0577854064628980, 84.00080373449807780 ) ) ;
#32686=CARTESIAN_POINT ( 'NONE',  ( 150.0501577908836737, 52.10460126680130344, -42.49831103806872079 ) ) ;
#32693=CARTESIAN_POINT ( 'NONE',  ( -86.06016868996613312, 25.27707703029501474, 39.20171598925913514 ) ) ;
#32694=CARTESIAN_POINT ( 'NONE',  ( 156.5993887774280324, 58.24868799840905353, -77.92120936136656439 ) ) ;
#32696=CARTESIAN_POINT ( 'NONE',  ( -23.95096213915836714, 8.481591526885939203, 65.04975062497030081 ) ) ;
#32697=EDGE_CURVE ( 'NONE', #40620, #24801, #13421, .T. ) ;
#32699=B_SPLINE_CURVE_WITH_KNOTS ( 'NONE', 3,
 ( #59615, #32556, #69487, #64568, #21305, #42754, #5811, #64213, #16026, #64919, #16377, #10748, #53649, #27265, #54338, #39235, #23054, #28677, #59970, #38524 ),
 .UNSPECIFIED., .F., .F.,
 ( 4, 2, 2, 2, 2, 2, 2, 2, 2, 4 ),
 ( 0.01005966960094808842, 0.01130938760903082291, 0.01255910561711355913, 0.01380882362519629536, 0.01505854163327902985, 0.01568340063732039796, 0.01630825964136176781, 0.01755797764944450404, 0.01880769565752724026, 0.02005741366560997996 ),
 .UNSPECIFIED. ) ;
#32705=CARTESIAN_POINT ( 'NONE',  ( 36.77024545412684375, 9.095083943590502429, -23.30259963730480877 ) ) ;
#32708=CARTESIAN_POINT ( 'NONE',  ( 56.66775172211443135, 11.28938863449063135, 68.15943088655339466 ) ) ;
#32709=CARTESIAN_POINT ( 'NONE',  ( 137.7927399796681414, 45.04243838361963270, 84.30735228466484443 ) ) ;
#32710=EDGE_CURVE ( 'NONE', #10586, #54090, #59192, .T. ) ;
#32713=VECTOR ( 'NONE', #38263, 1000.000000000000000 ) ;
#32719=ADVANCED_FACE ( 'NONE', ( #52869 ), #15605, .F. ) ;
#32722=FACE_OUTER_BOUND ( 'NONE', #10018, .T. ) ;
#32724=CARTESIAN_POINT ( 'NONE',  ( 136.9798231265810102, 43.34196232604179500, -77.20246944962947566 ) ) ;
#32725=CARTESIAN_POINT ( 'NONE',  ( 69.50572373348801136, 14.27208627753790893, 41.10388884447479541 ) ) ;
#32728=CARTESIAN_POINT ( 'NONE',  ( 84.97343609940683962, 18.86260005312943022, 17.68632826205469399 ) ) ;
#32730=CARTESIAN_POINT ( 'NONE',  ( -76.10397364431021572, 21.36211154336729834, 30.86549673594327814 ) ) ;
#32732=ORIENTED_EDGE ( 'NONE', *, *, #58048, .F. ) ;
#32733=DIRECTION ( 'NONE',  ( 0.000000000000000000, 0.000000000000000000, 1.000000000000000000 ) ) ;
#32737=EDGE_CURVE ( 'NONE', #34992, #3775, #32483, .T. ) ;
#32740=CARTESIAN_POINT ( 'NONE',  ( 151.1607415860635513, 52.90668588398090577, 32.82304110344981041 ) ) ;
#32741=CARTESIAN_POINT ( 'NONE',  ( -174.7903139851460139, 90.53182997092835649, -34.88798999700193804 ) ) ;
#32745=EDGE_LOOP ( 'NONE', ( #68187, #42519, #39396, #26358 ) ) ;
#32746=CARTESIAN_POINT ( 'NONE',  ( 136.1037846510193390, 43.98155406734453265, -63.19752277197763846 ) ) ;
#32750=FACE_BOUND ( 'NONE', #11387, .T. ) ;
#32751=FACE_OUTER_BOUND ( 'NONE', #20951, .T. ) ;
#32754=CARTESIAN_POINT ( 'NONE',  ( -83.53167274806556009, 25.32068190668984187, 16.80234616661474334 ) ) ;
#32756=B_SPLINE_CURVE_WITH_KNOTS ( 'NONE', 3,
 ( #39620, #45586, #61073, #67067, #12541, #66029, #18862, #54741, #40310, #22744, #7625, #23456, #44179, #65668, #55801, #6912, #1636, #34001, #44894, #38934, #44548, #60382, #17822, #55437, #66376, #40649, #14953, #51898, #47298, #35737, #29757, #41356, #3374, #41693, #46971, #46269, #57874, #62808, #19190, #57187, #9002, #36417, #13921, #31155, #36073, #19544, #67746 ),
 .UNSPECIFIED., .F., .F.,
 ( 4, 2, 2, 2, 2, 2, 2, 2, 2, 2, 2, 2, 1, 2, 2, 2, 2, 2, 2, 2, 2, 2, 2, 4 ),
 ( 0.000000000000000000, 0.001520400357568927252, 0.002280600536353409851, 0.003040800715137892234, 0.004561201072706856999, 0.005321401251491323335, 0.006081601430275789671, 0.007602001787844721477, 0.008362201966629198222, 0.009122402145413675834, 0.01064280250298263106, 0.01140300268176712775, 0.01216320286055162618, 0.01292340303933612461, 0.01368360321812062477, 0.01520400357568962683, 0.01596420375447412179, 0.01672440393325861502, 0.01824480429082758065, 0.01976520464839655322, 0.02052540482718103604, 0.02128560500596551885, 0.02280600536353448102, 0.02432640572110344665 ),
 .UNSPECIFIED. ) ;
#32757=CARTESIAN_POINT ( 'NONE',  ( -150.3791492925491298, 64.92185203933371440, 3.914254989767345094 ) ) ;
#32758=CARTESIAN_POINT ( 'NONE',  ( -120.6420427933462349, 44.31795133507807094, -74.61821363998994627 ) ) ;
#32759=AXIS2_PLACEMENT_3D ( 'NONE', #26779, #53491, #43630 ) ;
#32762=CARTESIAN_POINT ( 'NONE',  ( 159.6725804802005655, 59.38339663535510482, 17.24836648525045035 ) ) ;
#32763=CARTESIAN_POINT ( 'NONE',  ( 94.02499804464933675, 23.15433260743126453, -15.20501225471814877 ) ) ;
#32765=CARTESIAN_POINT ( 'NONE',  ( -36.89224332184166855, 11.57404295377975600, 5.717042333022100742 ) ) ;
#32767=FACE_OUTER_BOUND ( 'NONE', #50606, .T. ) ;
#32768=CARTESIAN_POINT ( 'NONE',  ( 83.38619203015947789, 19.39783821526630803, -76.94561659048915203 ) ) ;
#32769=CARTESIAN_POINT ( 'NONE',  ( 117.3315207373142215, 33.42838861910006898, 88.32577119086282380 ) ) ;
#32773=CARTESIAN_POINT ( 'NONE',  ( -26.49928411671542960, 9.848831533840670005, -37.15254042537868173 ) ) ;
#32774=CARTESIAN_POINT ( 'NONE',  ( -48.34500911884041585, 14.01939034823941732, -66.19665500006401260 ) ) ;
#32775=B_SPLINE_CURVE_WITH_KNOTS ( 'NONE', 3,
 ( #52924, #36423, #62817, #4750, #47304, #36083, #4413, #20932, #15659, #24835, #57540, #20580, #41700, #19908, #3715, #26213, #58549, #41364, #68435, #31833, #10367, #52254, #51906, #46276, #25878, #63165, #9342, #47653, #14284, #57879, #67753, #63851, #19553, #4076, #31163, #62467, #35743, #68765, #42042, #9013, #69107, #30455, #25540 ),
 .UNSPECIFIED., .F., .F.,
 ( 4, 2, 2, 2, 2, 2, 2, 2, 1, 2, 2, 2, 2, 2, 2, 2, 2, 2, 2, 2, 2, 4 ),
 ( 0.000000000000000000, 0.001465684626643344503, 0.002198526939965016972, 0.002931369253286689007, 0.004397053879930033944, 0.005862738506573378014, 0.007328423133216722084, 0.008061265446538396287, 0.008794107759860073092, 0.009526950073181746428, 0.01025979238650342150, 0.01172547701314677338, 0.01319116163979012525, 0.01465684626643347713, 0.01538968857975514873, 0.01612253089307682033, 0.01758821551972016353, 0.01905390014636350327, 0.01978674245968517140, 0.02051958477300683953, 0.02198526939965017579, 0.02345095402629350512 ),
 .UNSPECIFIED. ) ;
#32777=CARTESIAN_POINT ( 'NONE',  ( 104.0290905220488469, 26.11184870228230892, 94.99999999999866418 ) ) ;
#32781=CARTESIAN_POINT ( 'NONE',  ( 34.83823433017387572, 8.871835168107974567, 58.28624973792864239 ) ) ;
#32782=CARTESIAN_POINT ( 'NONE',  ( -171.4943428135322847, 86.82484920477511992, 72.53627115242575485 ) ) ;
#32784=CARTESIAN_POINT ( 'NONE',  ( -168.0003605155415016, 83.06333427281268200, -20.85263118173764951 ) ) ;
#32788=CARTESIAN_POINT ( 'NONE',  ( 187.5165082312810227, 86.85340440641657267, -20.74607734399896231 ) ) ;
#32791=CARTESIAN_POINT ( 'NONE',  ( -78.66644367742109978, 23.39876645725289706, -88.80455181264524356 ) ) ;
#32792=CARTESIAN_POINT ( 'NONE',  ( 46.70715146412976537, 9.472433765546997009, -17.99120794428602821 ) ) ;
#32793=CARTESIAN_POINT ( 'NONE',  ( 210.4897348480408255, 114.6382060222044714, -21.75249441828651698 ) ) ;
#32794=CYLINDRICAL_SURFACE ( 'NONE', #54228, 7.500000000000020428 ) ;
#32795=CARTESIAN_POINT ( 'NONE',  ( 160.9099843287284841, 61.67000084894968381, 57.07340599545204185 ) ) ;
#32798=EDGE_LOOP ( 'NONE', ( #11210, #1875 ) ) ;
#32799=EDGE_CURVE ( 'NONE', #8782, #30746, #12250, .T. ) ;
#32801=CARTESIAN_POINT ( 'NONE',  ( -31.43908319763709969, 9.591432048623765638, 57.06100499665286208 ) ) ;
#32803=CARTESIAN_POINT ( 'NONE',  ( -51.34562532494749831, 14.75613283840035983, 71.19973610574378142 ) ) ;
#32806=CARTESIAN_POINT ( 'NONE',  ( -15.23124449227264066, 8.497728762338836006, 89.95007870748302992 ) ) ;
#32808=CARTESIAN_POINT ( 'NONE',  ( 59.72897338775215559, 11.93428797217974591, 3.722467926232761126 ) ) ;
#32809=CARTESIAN_POINT ( 'NONE',  ( -56.97107423601134712, 15.20373812575556194, 57.39529982396223318 ) ) ;
#32814=LINE ( 'NONE', #6065, #1839 ) ;
#32815=CARTESIAN_POINT ( 'NONE',  ( 104.7034219878852213, 26.40210929103715998, 32.03102971527638232 ) ) ;
#32816=EDGE_LOOP ( 'NONE', ( #27018, #55823 ) ) ;
#32819=VECTOR ( 'NONE', #67524, 1000.000000000000000 ) ;
#32820=CARTESIAN_POINT ( 'NONE',  ( 86.62931800182293784, -170.0000000000000000, -16.47701360844803986 ) ) ;
#32825=CARTESIAN_POINT ( 'NONE',  ( -51.13576748034041231, 14.70354244225167584, -49.11681489039352044 ) ) ;
#32827=CARTESIAN_POINT ( 'NONE',  ( 13.37708032728285623, 7.441924986912762385, 30.40862419550404994 ) ) ;
#32829=CARTESIAN_POINT ( 'NONE',  ( 79.29307999139646768, 17.04697453199588963, 92.49707517143880864 ) ) ;
#32831=EDGE_LOOP ( 'NONE', ( #10882, #3573, #7016, #36322 ) ) ;
#32834=CARTESIAN_POINT ( 'NONE',  ( -15.32550079334879278, 7.496023944924841587, -16.31543665609040872 ) ) ;
#32835=CYLINDRICAL_SURFACE ( 'NONE', #42800, 7.500000000000013323 ) ;
#32836=CARTESIAN_POINT ( 'NONE',  ( -53.14475157111026249, 14.17819596930906556, -23.12906344254722413 ) ) ;
#32838=CARTESIAN_POINT ( 'NONE',  ( -34.52542994698664813, 11.14027065218089518, 71.40085072621459972 ) ) ;
#32840=CARTESIAN_POINT ( 'NONE',  ( 150.9184679586219886, 52.73111408630724384, -66.80947418898379908 ) ) ;
#32841=CARTESIAN_POINT ( 'NONE',  ( 23.28869764673362042, 6.856674305776599532, -15.68603375068130390 ) ) ;
#32848=CARTESIAN_POINT ( 'NONE',  ( -59.10270545739309966, 16.85145316017989714, -90.07846592657732288 ) ) ;
#32849=CARTESIAN_POINT ( 'NONE',  ( -24.30908968323081254, 9.544419512845170317, 93.82125383429070098 ) ) ;
#32850=CARTESIAN_POINT ( 'NONE',  ( 115.0606351894211627, 32.29586232625067765, -22.34698907665701384 ) ) ;
#32853=CARTESIAN_POINT ( 'NONE',  ( -108.6634958860518196, 36.14357436892402831, 15.11988995337718933 ) ) ;
#32855=CARTESIAN_POINT ( 'NONE',  ( 141.0792860804899362, 47.16255757051794006, -18.76987349801746774 ) ) ;
#32856=ORIENTED_EDGE ( 'NONE', *, *, #9778, .T. ) ;
#32857=ORIENTED_EDGE ( 'NONE', *, *, #11573, .F. ) ;
#32858=EDGE_CURVE ( 'NONE', #31501, #34735, #52479, .T. ) ;
#32862=CARTESIAN_POINT ( 'NONE',  ( -156.8728827992624133, 72.05711009495556141, -16.91073671683209056 ) ) ;
#32864=CARTESIAN_POINT ( 'NONE',  ( 88.59828180051356128, 21.16853032775269838, -89.76271995981053919 ) ) ;
#32865=EDGE_CURVE ( 'NONE', #49747, #65764, #34217, .T. ) ;
#32867=CARTESIAN_POINT ( 'NONE',  ( -35.17686701826945495, 10.23452050416468140, 71.08151450555706674 ) ) ;
#32868=CARTESIAN_POINT ( 'NONE',  ( -149.5074843970971017, 64.17983161892348676, -22.96827994102829962 ) ) ;
#32872=CARTESIAN_POINT ( 'NONE',  ( -6.125624616441583292, 7.794071945221091369, -35.60914887735208367 ) ) ;
#32873=CARTESIAN_POINT ( 'NONE',  ( 102.8111940033033989, 25.59308899183600872, 11.30835609773350647 ) ) ;
#32874=FACE_OUTER_BOUND ( 'NONE', #52264, .T. ) ;
#32875=CARTESIAN_POINT ( 'NONE',  ( -82.32750425780473336, 23.74963782027935011, -36.05213690621574329 ) ) ;
#32876=CARTESIAN_POINT ( 'NONE',  ( 19.11168290073777598, 6.629794975642855803, 71.08720758981752397 ) ) ;
#32878=CARTESIAN_POINT ( 'NONE',  ( 12.46277766093406569, 6.416700641561363661, -63.12311374513074469 ) ) ;
#32880=VERTEX_POINT ( 'NONE', #61634 ) ;
#32883=CARTESIAN_POINT ( 'NONE',  ( -132.0958200534847435, 50.71531800824805458, -73.48295987508291205 ) ) ;
#32884=CARTESIAN_POINT ( 'NONE',  ( -132.6161619568759136, 51.08240647571219739, -45.74966482454154715 ) ) ;
#32885=CARTESIAN_POINT ( 'NONE',  ( 45.49006904354232006, 9.279592366778887325, -74.35131477850875115 ) ) ;
#32887=ORIENTED_EDGE ( 'NONE', *, *, #25102, .F. ) ;
#32891=ORIENTED_EDGE ( 'NONE', *, *, #19929, .F. ) ;
#32893=CARTESIAN_POINT ( 'NONE',  ( 176.0745160362858428, 73.68684431790050837, -38.13833935887404891 ) ) ;
#32897=CARTESIAN_POINT ( 'NONE',  ( 139.1306635769909121, 45.89653412152168954, 58.51687394488192950 ) ) ;
#32898=CARTESIAN_POINT ( 'NONE',  ( -71.37402418445425667, 19.67651958824262337, -44.38599607864244945 ) ) ;
#32900=CARTESIAN_POINT ( 'NONE',  ( 164.6046919270428930, 63.41782451559755174, -95.00000000000133582 ) ) ;
#32903=CARTESIAN_POINT ( 'NONE',  ( -48.58279704072701577, 14.07632445131079457, -12.07026367287715019 ) ) ;
#32906=CARTESIAN_POINT ( 'NONE',  ( -123.6619986853278306, 45.04188181212062148, -8.405249343855505373 ) ) ;
#32908=CARTESIAN_POINT ( 'NONE',  ( -143.4048679855200703, 60.45763799613827416, -37.94565703660070000 ) ) ;
#32910=CARTESIAN_POINT ( 'NONE',  ( -142.0081215801269536, 58.07066293384866640, -42.61264745997317505 ) ) ;
#32912=CARTESIAN_POINT ( 'NONE',  ( 57.41085175769455873, 12.46982565415947519, 5.478706012108088608 ) ) ;
#32914=EDGE_LOOP ( 'NONE', ( #61292, #16173, #41723, #34327 ) ) ;
#32915=CARTESIAN_POINT ( 'NONE',  ( -128.9925397612933580, 48.56800623462828526, 31.28606989344878642 ) ) ;
#32921=CARTESIAN_POINT ( 'NONE',  ( 94.11746922806581495, 22.11341285603780449, -69.67410109035120058 ) ) ;
#32923=CARTESIAN_POINT ( 'NONE',  ( -95.61819996182569525, 29.52346081122274413, 14.62890838970597329 ) ) ;
#32924=CARTESIAN_POINT ( 'NONE',  ( -149.5074843970970733, 65.50121172469319220, -34.81283053149196149 ) ) ;
#32927=CARTESIAN_POINT ( 'NONE',  ( 41.35041461497707616, 8.670465437677201237, 44.67304901252469307 ) ) ;
#32928=CARTESIAN_POINT ( 'NONE',  ( 12.03317402819681625, 6.409531826169460267, 31.01780596777689425 ) ) ;
#32931=CARTESIAN_POINT ( 'NONE',  ( 207.4566510040494904, 111.9649643341356580, -50.80316001813071125 ) ) ;
#32934=CARTESIAN_POINT ( 'NONE',  ( 43.96062659677685502, 10.06332325923986204, -37.14425628477024333 ) ) ;
#32936=ORIENTED_EDGE ( 'NONE', *, *, #15518, .F. ) ;
#32937=CARTESIAN_POINT ( 'NONE',  ( -102.2801239173131052, 32.78103895658057354, -23.17002667451225406 ) ) ;
#32940=CARTESIAN_POINT ( 'NONE',  ( -10.23402954931276732, 7.059791383763807993, -35.81110276668997017 ) ) ;
#32941=VECTOR ( 'NONE', #21880, 1000.000000000000000 ) ;
#32942=CARTESIAN_POINT ( 'NONE',  ( -190.6985136298601731, 109.1272424661242582, 94.99999999999866418 ) ) ;
#32943=CARTESIAN_POINT ( 'NONE',  ( 90.91356992076218546, 21.99794663086831648, 70.21725602554428747 ) ) ;
#32944=CARTESIAN_POINT ( 'NONE',  ( 155.2910738464913152, 55.97560547655804442, -23.97026548063870521 ) ) ;
#32948=ADVANCED_FACE ( 'NONE', ( #1867 ), #56704, .F. ) ;
#32949=CARTESIAN_POINT ( 'NONE',  ( 113.2766812233866318, 31.42710996230401577, -90.24119829850059205 ) ) ;
#32951=B_SPLINE_CURVE_WITH_KNOTS ( 'NONE', 3,
 ( #55671, #7504, #44419, #28957, #29288, #39842, #18045, #50402, #66943, #44778, #28237, #33540, #13123, #40195, #49682, #55317, #6446, #27897, #2219, #23668, #49332, #45112, #66595, #60254, #34591, #38808, #50741, #54968, #2561, #1510, #33879, #22975, #17702, #39161, #12421, #67292, #57067, #47183, #62338, #3256, #46491, #8880, #67624, #13461 ),
 .UNSPECIFIED., .F., .F.,
 ( 4, 2, 2, 2, 2, 2, 2, 2, 2, 2, 2, 2, 2, 2, 2, 2, 2, 2, 2, 2, 2, 4 ),
 ( 0.000000000000000000, 0.001488594467279762395, 0.002232891700919633834, 0.002977188934559505274, 0.004465783401839225168, 0.005954377869118944629, 0.007442972336398671895, 0.008187269570038539432, 0.008931566803678405234, 0.01042016127095814551, 0.01190875573823788405, 0.01265305297187775332, 0.01339735020551761913, 0.01488594467279734899, 0.01563024190643721653, 0.01637453914007708233, 0.01786313360735681047, 0.01935172807463653513, 0.02009602530827639399, 0.02084032254191624939, 0.02232891700919594630, 0.02381751147647563627 ),
 .UNSPECIFIED. ) ;
#32952=CARTESIAN_POINT ( 'NONE',  ( 211.9998916201001293, 116.9275145151761990, 92.12172642968158698 ) ) ;
#32954=ORIENTED_EDGE ( 'NONE', *, *, #42849, .F. ) ;
#32955=CARTESIAN_POINT ( 'NONE',  ( 62.04382205963241859, 13.48099884269679904, 71.61031193528864947 ) ) ;
#32957=CARTESIAN_POINT ( 'NONE',  ( -11.13714165684778301, 8.138643170880696331, 4.037354935646943588 ) ) ;
#32959=DIRECTION ( 'NONE',  ( 0.000000000000000000, 0.000000000000000000, 1.000000000000000000 ) ) ;
#32960=CARTESIAN_POINT ( 'NONE',  ( -1.314022807222072098, 6.554273999800675377, 41.36949670402924539 ) ) ;
#32963=CARTESIAN_POINT ( 'NONE',  ( 90.66938301215044760, 21.90914557174533073, 84.57376703108099036 ) ) ;
#32964=AXIS2_PLACEMENT_3D ( 'NONE', #38601, #59354, #27690 ) ;
#32966=VERTEX_POINT ( 'NONE', #18375 ) ;
#32969=CARTESIAN_POINT ( 'NONE',  ( -189.2826425734429563, 107.1493800926106275, -14.39297977970899112 ) ) ;
#32970=CARTESIAN_POINT ( 'NONE',  ( -126.8005235842505840, 47.09307471149451629, 18.73398224919106880 ) ) ;
#32972=CARTESIAN_POINT ( 'NONE',  ( -166.9992034932275828, 82.01285191063138313, -37.84924264257025328 ) ) ;
#32973=CARTESIAN_POINT ( 'NONE',  ( -180.5370160906538786, 95.78117245680181213, 90.87545911180488645 ) ) ;
#32977=CARTESIAN_POINT ( 'NONE',  ( 201.9721407532274782, 104.3507814346148024, -9.982163974892198866 ) ) ;
#32978=CARTESIAN_POINT ( 'NONE',  ( -1.866625526081663322, 7.583073082893625028, -65.18153374896648700 ) ) ;
#32982=CARTESIAN_POINT ( 'NONE',  ( 80.15818551272217007, 18.36718314243336181, 14.19107730079274887 ) ) ;
#32983=B_SPLINE_CURVE_WITH_KNOTS ( 'NONE', 3,
 ( #46340, #25608, #68501, #3108, #36841, #46006, #41770, #35455, #15037, #24570, #41079, #58280, #24908, #36493, #10101, #52657, #8736, #25940, #67818, #31556, #47372, #20651, #67472, #19267, #62540, #10435, #43480, #37870, #48390, #5509, #934, #59317, #21008, #26963, #52994, #16753, #42786, #11130, #63910, #64957, #226, #58620, #58968, #43824, #47719, #37173 ),
 .UNSPECIFIED., .F., .F.,
 ( 4, 2, 2, 2, 2, 2, 2, 2, 2, 2, 2, 2, 2, 2, 2, 2, 2, 2, 2, 2, 2, 2, 4 ),
 ( 6.938893903907228378E-18, 0.003192770216278346951, 0.003990962770347930219, 0.004789155324417513487, 0.006385540432556660942, 0.007183732986626248547, 0.007981925540695836152, 0.009578310648835011362, 0.01037650320290461198, 0.01117469575697421086, 0.01197288831104380974, 0.01277108086511340862, 0.01436746597325258383, 0.01596385108139175904, 0.01676204363546133710, 0.01756023618953091170, 0.01835842874360048976, 0.01915662129767006783, 0.02075300640580923089, 0.02234939151394839396, 0.02394577662208756050, 0.02474396917615714203, 0.02554216173022672010 ),
 .UNSPECIFIED. ) ;
#32984=CARTESIAN_POINT ( 'NONE',  ( -95.20053778133916467, 30.43887292928078381, 35.49128386806113866 ) ) ;
#32986=CARTESIAN_POINT ( 'NONE',  ( 114.6797682035588934, 32.10876583290006892, 4.200831402737990494 ) ) ;
#32995=CARTESIAN_POINT ( 'NONE',  ( 157.4703587214989113, 57.65129005721575339, -89.81328548006499091 ) ) ;
#32999=LINE ( 'NONE', #54084, #33928 ) ;
#33005=VECTOR ( 'NONE', #53463, 1000.000000000000000 ) ;
#33007=CARTESIAN_POINT ( 'NONE',  ( -32.41627406084104734, 9.753381371531506971, -8.520735355804967881 ) ) ;
#33008=CARTESIAN_POINT ( 'NONE',  ( 156.7474413564702616, 57.09079859174879346, -89.83946617008655267 ) ) ;
#33010=CARTESIAN_POINT ( 'NONE',  ( 126.4633682455862100, 38.28837286275645369, 65.14279228220068774 ) ) ;
#33020=EDGE_CURVE ( 'NONE', #65087, #44762, #54203, .T. ) ;
#33022=CARTESIAN_POINT ( 'NONE',  ( -47.97412431374925035, 13.93110604348564685, 89.00688050077388880 ) ) ;
#33026=CARTESIAN_POINT ( 'NONE',  ( -97.72846716802192191, 31.64568465353664806, -90.23871114884526889 ) ) ;
#33027=EDGE_LOOP ( 'NONE', ( #15411, #23045, #20838, #2132 ) ) ;
#33028=ORIENTED_EDGE ( 'NONE', *, *, #47177, .F. ) ;
#33029=CARTESIAN_POINT ( 'NONE',  ( 184.3941060377212011, 82.01604625189465025, 30.06399996121712093 ) ) ;
#33032=CARTESIAN_POINT ( 'NONE',  ( -31.43908319763710679, -170.0000000000000000, -50.31719736520186359 ) ) ;
#33033=CARTESIAN_POINT ( 'NONE',  ( -38.61120365219831996, 10.87907113164045469, -94.14611914679960591 ) ) ;
#33034=CARTESIAN_POINT ( 'NONE',  ( 22.15926701483428829, 7.796117250416236821, 41.47971552668069251 ) ) ;
#33041=VERTEX_POINT ( 'NONE', #15357 ) ;
#33045=CARTESIAN_POINT ( 'NONE',  ( -83.12901536265223967, 24.07178615860086168, 43.95099611738770307 ) ) ;
#33048=CARTESIAN_POINT ( 'NONE',  ( -28.13852122803040956, 9.072484007196644384, 57.80876482626037216 ) ) ;
#33049=CIRCLE ( 'NONE', #3881, 243.4957430088094839 ) ;
#33050=CARTESIAN_POINT ( 'NONE',  ( 128.0848616812662613, 38.04676222636084049, -11.86342996178354703 ) ) ;
#33054=ORIENTED_EDGE ( 'NONE', *, *, #9525, .T. ) ;
#33055=ADVANCED_FACE ( 'NONE', ( #68476 ), #66853, .F. ) ;
#33060=CARTESIAN_POINT ( 'NONE',  ( -190.6985136298601731, 109.1272424661242582, -95.00000000000133582 ) ) ;
#33061=CARTESIAN_POINT ( 'NONE',  ( 188.0298970627777635, 87.42051935455698697, -94.54416634815818554 ) ) ;
#33063=CARTESIAN_POINT ( 'NONE',  ( 206.3125232506203304, 108.5822159704962075, 44.04308254722315041 ) ) ;
#33069=CARTESIAN_POINT ( 'NONE',  ( -125.4481990864045287, 46.20056605584957765, -76.75825448869764500 ) ) ;
#33078=CARTESIAN_POINT ( 'NONE',  ( 79.23200707685333555, 17.02828389812517429, 11.62992474421185385 ) ) ;
#33080=CARTESIAN_POINT ( 'NONE',  ( -71.26675986148646302, 19.63956187826085298, 39.16646718081778289 ) ) ;
#33087=ORIENTED_EDGE ( 'NONE', *, *, #9062, .T. ) ;
#33090=EDGE_CURVE ( 'NONE', #16235, #29084, #13710, .T. ) ;
#33094=CARTESIAN_POINT ( 'NONE',  ( -129.6165111262478149, 48.99406349865698473, -22.08429765273019996 ) ) ;
#33097=B_SPLINE_CURVE_WITH_KNOTS ( 'NONE', 3,
 ( #69233, #9472, #31961, #57660, #279, #15776, #14739, #63962, #37222, #52376, #68556, #10489, #52705, #4871, #5559, #48444, #58331, #20709, #4197, #10149, #26340, #25661, #47093, #4533, #20359, #36894, #37574, #48113, #30933, #42837, #26682, #21065, #53388, #31611, #41826, #63281, #42165, #67028 ),
 .UNSPECIFIED., .F., .F.,
 ( 4, 2, 2, 2, 2, 2, 2, 2, 2, 2, 2, 2, 2, 2, 2, 2, 2, 2, 4 ),
 ( 1.551583845779545699E-17, 0.001559859933532273648, 0.003119719867064531683, 0.004679579800596789067, 0.006239439734129047753, 0.007799299667661305571, 0.008579229634427429710, 0.009359159601193552114, 0.01091901953472580039, 0.01169894950149191065, 0.01247887946825801918, 0.01403873940179021888, 0.01559859933532241859, 0.01715845926885461656, 0.01871831920238681626, 0.02027817913591901597, 0.02183803906945121567, 0.02339789900298341538, 0.02495775893651561508 ),
 .UNSPECIFIED. ) ;
#33098=ORIENTED_EDGE ( 'NONE', *, *, #65770, .T. ) ;
#33102=FACE_BOUND ( 'NONE', #24465, .T. ) ;
#33105=CARTESIAN_POINT ( 'NONE',  ( -180.2188652555596491, 96.98354576637423463, 62.72563788181442845 ) ) ;
#33108=CARTESIAN_POINT ( 'NONE',  ( -81.90760111942957167, 24.66532273091449667, 17.85392087365031344 ) ) ;
#33112=CARTESIAN_POINT ( 'NONE',  ( -125.6703656163502529, 47.55170550253217954, -76.75825448869768763 ) ) ;
#33116=CARTESIAN_POINT ( 'NONE',  ( 163.7607557204680404, 62.71181783708028235, 14.18050344063046886 ) ) ;
#33118=CARTESIAN_POINT ( 'NONE',  ( 42.79263376053064860, 9.891365420389709229, -90.11595853705047432 ) ) ;
#33125=CARTESIAN_POINT ( 'NONE',  ( 81.04027388895737261, 18.64386073872847760, -65.14085334647751324 ) ) ;
#33126=CARTESIAN_POINT ( 'NONE',  ( 103.6609592836012439, 27.04873813663200721, 94.41228810559154283 ) ) ;
#33127=CARTESIAN_POINT ( 'NONE',  ( -143.2498117110515352, 60.33382252735061257, 60.92286773224797969 ) ) ;
#33128=CARTESIAN_POINT ( 'NONE',  ( 69.49862690228275142, 14.27023134440515051, -20.17942441373172358 ) ) ;
#33129=CARTESIAN_POINT ( 'NONE',  ( -24.32776401346968242, 9.546905915310563984, -40.38412230395840652 ) ) ;
#33130=CARTESIAN_POINT ( 'NONE',  ( 211.7634543339367781, 118.4123239814494610, -95.00000000000133582 ) ) ;
#33131=CARTESIAN_POINT ( 'NONE',  ( -73.58789645738433194, 21.51976592945687727, -90.76835761085054344 ) ) ;
#33132=CARTESIAN_POINT ( 'NONE',  ( -125.4463376280758666, 47.40387005565908396, -23.05918939656154265 ) ) ;
#33135=CARTESIAN_POINT ( 'NONE',  ( 33.46033188299907835, 8.722678254080102889, 59.67493974660781930 ) ) ;
#33143=CARTESIAN_POINT ( 'NONE',  ( 94.11733320392089297, 23.18939451097127957, 9.873858910156306123 ) ) ;
#33144=CARTESIAN_POINT ( 'NONE',  ( -14.32241591711280115, 7.401556312061830845, 68.21502159609927674 ) ) ;
#33145=CARTESIAN_POINT ( 'NONE',  ( -81.00507684688699328, 23.22613445438386748, -8.640849626975995790 ) ) ;
#33146=FACE_OUTER_BOUND ( 'NONE', #65775, .T. ) ;
#33147=CARTESIAN_POINT ( 'NONE',  ( 42.49453823366105354, 8.831814337191476127, -9.438221642302703884 ) ) ;
#33148=CARTESIAN_POINT ( 'NONE',  ( 211.7419975634644800, 116.5322580952101674, -19.63582788492490394 ) ) ;
#33149=FACE_BOUND ( 'NONE', #3253, .T. ) ;
#33151=CARTESIAN_POINT ( 'NONE',  ( -61.86403937395562025, 16.61416349803655734, -39.56707441162413375 ) ) ;
#33154=CARTESIAN_POINT ( 'NONE',  ( -109.6829043543429236, 37.85329552808669717, -95.00000000000133582 ) ) ;
#33155=CARTESIAN_POINT ( 'NONE',  ( 93.32756701508621688, 22.89083686918420568, -39.91087544770613249 ) ) ;
#33157=DIRECTION ( 'NONE',  ( -0.000000000000000000, 1.000000000000000000, -0.000000000000000000 ) ) ;
#33158=DIRECTION ( 'NONE',  ( -0.000000000000000000, 1.000000000000000000, -0.000000000000000000 ) ) ;
#33164=CARTESIAN_POINT ( 'NONE',  ( 55.76066037845578194, 11.10616952318092032, 8.503228194878166946 ) ) ;
#33171=CARTESIAN_POINT ( 'NONE',  ( 107.2672065034543039, 27.52931006625852817, 30.22273792253545466 ) ) ;
#33175=CARTESIAN_POINT ( 'NONE',  ( 157.9121974517528599, 59.27335488206247760, 29.40946747225336821 ) ) ;
#33176=CARTESIAN_POINT ( 'NONE',  ( -156.0204364459164594, 71.27041535366184632, -65.42916888645565621 ) ) ;
#33178=CARTESIAN_POINT ( 'NONE',  ( 70.51583798635768119, 15.57951509147424041, 10.22650159239598544 ) ) ;
#33183=CARTESIAN_POINT ( 'NONE',  ( 39.40195752203891999, 9.424259417798149130, 44.91383430596327742 ) ) ;
#33186=CARTESIAN_POINT ( 'NONE',  ( 63.42461771757965039, 12.76763389977390695, -89.40979201309708913 ) ) ;
#33187=CARTESIAN_POINT ( 'NONE',  ( 88.27986429602357532, 19.99062825313306391, 83.57789623867044781 ) ) ;
#33190=VERTEX_POINT ( 'NONE', #7753 ) ;
#33191=ORIENTED_EDGE ( 'NONE', *, *, #66589, .F. ) ;
#33192=CARTESIAN_POINT ( 'NONE',  ( -15.26524495591509556, 7.490231452641286758, -17.05327951355247151 ) ) ;
#33193=CARTESIAN_POINT ( 'NONE',  ( -54.08504625707234226, 14.42374043447185272, 45.27053657996511049 ) ) ;
#33195=DIRECTION ( 'NONE',  ( -0.000000000000000000, 1.000000000000000000, -0.000000000000000000 ) ) ;
#33197=CARTESIAN_POINT ( 'NONE',  ( -59.58556642339446086, 16.99097764963621771, -36.72105999418167244 ) ) ;
#33198=CARTESIAN_POINT ( 'NONE',  ( -14.84452950307166219, 8.460866451887694595, -18.72723383062862368 ) ) ;
#33210=CARTESIAN_POINT ( 'NONE',  ( -60.12227522086160292, 17.14774203938726416, -90.87396971807878288 ) ) ;
#33215=CARTESIAN_POINT ( 'NONE',  ( -108.9136445001389575, 36.28030794288191885, 14.68305003638678841 ) ) ;
#33218=CARTESIAN_POINT ( 'NONE',  ( 141.2801018238827453, 47.29457739955285689, -15.57642269469550200 ) ) ;
#33221=VECTOR ( 'NONE', #50142, 1000.000000000000000 ) ;
#33222=ORIENTED_EDGE ( 'NONE', *, *, #65793, .T. ) ;
#33223=CARTESIAN_POINT ( 'NONE',  ( 86.62931800182293784, -170.0000000000000000, -8.977013608448027426 ) ) ;
#33224=AXIS2_PLACEMENT_3D ( 'NONE', #5407, #37070, #5739 ) ;
#33225=CARTESIAN_POINT ( 'NONE',  ( -157.0079874970173250, 72.18249880494039417, -15.19463801503674460 ) ) ;
#33226=CARTESIAN_POINT ( 'NONE',  ( 39.40195752203892710, 8.409560354027375340, -77.46436805589148378 ) ) ;
#33229=CARTESIAN_POINT ( 'NONE',  ( -38.54881010929333485, 10.86689971295296431, 66.99878871782735246 ) ) ;
#33231=ORIENTED_EDGE ( 'NONE', *, *, #41778, .F. ) ;
#33232=CARTESIAN_POINT ( 'NONE',  ( 63.01563776193091826, 12.67277567978498709, -62.56524142263340593 ) ) ;
#33233=CARTESIAN_POINT ( 'NONE',  ( -154.6171773099879658, 68.63761944777705537, 70.56064342458570593 ) ) ;
#33235=CARTESIAN_POINT ( 'NONE',  ( -4.071369321747702053, 7.682719369516287422, -36.40674159414955113 ) ) ;
#33237=CARTESIAN_POINT ( 'NONE',  ( -82.53770812813171176, 23.83403279300014432, -49.04362026007095920 ) ) ;
#33241=CARTESIAN_POINT ( 'NONE',  ( 12.03194517566456412, 6.409266703743583982, -63.35348225446327319 ) ) ;
#33242=B_SPLINE_CURVE_WITH_KNOTS ( 'NONE', 3,
 ( #40247, #19473, #8238, #25116, #8592, #2965, #36350, #40933, #20169, #34972, #30040, #57803, #13516, #9622, #52178, #14547, #29686, #35666, #51502, #36007, #24072, #56416, #62392, #51151, #67339, #45515, #14883, #66999, #24425, #24765, #45867, #67678, #57120, #46548, #62036, #19127, #30731, #40581, #31084, #14207, #30380, #51832, #3641 ),
 .UNSPECIFIED., .F., .F.,
 ( 4, 2, 2, 2, 2, 2, 2, 2, 2, 2, 2, 2, 1, 2, 2, 2, 2, 2, 2, 2, 2, 4 ),
 ( 0.02390068823634511341, 0.02538837671117072023, 0.02613222094858352190, 0.02687606518599632011, 0.02836375366082194427, 0.02985144213564756843, 0.03059528637306038745, 0.03133913061047320647, 0.03282681908529885145, 0.03431450756012450337, 0.03580219603495014835, 0.03654604027236297431, 0.03728988450977580027, 0.03803372874718861929, 0.03877757298460144525, 0.04026526145942713186, 0.04175294993425281154, 0.04324063840907849815, 0.04398448264649133799, 0.04472832688390418476, 0.04621601535872985056, 0.04770370383355551636 ),
 .UNSPECIFIED. ) ;
#33245=CARTESIAN_POINT ( 'NONE',  ( -133.3958821919892728, 51.63629593114584537, -69.77245200765010225 ) ) ;
#33250=ORIENTED_EDGE ( 'NONE', *, *, #31124, .T. ) ;
#33251=LINE ( 'NONE', #54685, #31398 ) ;
#33253=ORIENTED_EDGE ( 'NONE', *, *, #66326, .T. ) ;
#33256=CARTESIAN_POINT ( 'NONE',  ( 174.1251613516845111, 71.84747073139213569, -40.87395508819982126 ) ) ;
#33260=CARTESIAN_POINT ( 'NONE',  ( 136.1215428813736992, 43.99260314811117212, 56.69008934874803174 ) ) ;
#33261=CARTESIAN_POINT ( 'NONE',  ( -77.02372450489323796, 21.70271995013165167, -49.93720601098491585 ) ) ;
#33266=CARTESIAN_POINT ( 'NONE',  ( -189.2442476610617916, 107.0963225822736007, 38.85773244000630910 ) ) ;
#33269=VECTOR ( 'NONE', #18388, 1000.000000000000000 ) ;
#33272=CARTESIAN_POINT ( 'NONE',  ( 113.8568724296587789, 30.58972477291343850, -50.01180695322363334 ) ) ;
#33274=EDGE_CURVE ( 'NONE', #10310, #24054, #37011, .T. ) ;
#33276=CARTESIAN_POINT ( 'NONE',  ( 41.80536115778105000, 8.734184316430663841, -50.22851050661703454 ) ) ;
#33277=CARTESIAN_POINT ( 'NONE',  ( -167.4844853368928170, 82.52074065752736942, -74.01054566969028770 ) ) ;
#33278=CARTESIAN_POINT ( 'NONE',  ( -129.5125723098807384, 48.92280137375520610, 85.23347960619950925 ) ) ;
#33280=LINE ( 'NONE', #22015, #34214 ) ;
#33282=VERTEX_POINT ( 'NONE', #53992 ) ;
#33283=CARTESIAN_POINT ( 'NONE',  ( -130.6002960060536395, 49.67125682092491701, 32.26042931784617451 ) ) ;
#33286=CARTESIAN_POINT ( 'NONE',  ( 89.87840278991589571, 21.62393877508910833, 30.44804967038920651 ) ) ;
#33289=CARTESIAN_POINT ( 'NONE',  ( 92.19920907511534836, 21.39700525884450855, -75.21216531110735559 ) ) ;
#33290=CARTESIAN_POINT ( 'NONE',  ( -28.53262343748519214, 9.132042770041840285, -89.57910440806035979 ) ) ;
#33293=EDGE_CURVE ( 'NONE', #22683, #48695, #7135, .T. ) ;
#33296=CARTESIAN_POINT ( 'NONE',  ( 46.90222083990963853, 9.503928413859240365, 37.65402312257223372 ) ) ;
#33300=CARTESIAN_POINT ( 'NONE',  ( 211.7318474105134669, 118.3631723164074714, -46.44534482335959069 ) ) ;
#33301=CARTESIAN_POINT ( 'NONE',  ( -78.19438069111004097, 23.21811806230640585, -76.96000122218163142 ) ) ;
#33303=CARTESIAN_POINT ( 'NONE',  ( 157.4703587214989398, -170.0000000000000000, -16.77963370867396975 ) ) ;
#33304=CARTESIAN_POINT ( 'NONE',  ( 162.6190874793280727, 61.76782592053313437, -75.92743616221932257 ) ) ;
#33307=CARTESIAN_POINT ( 'NONE',  ( -23.93933407965396043, 9.495050561681672718, 11.36750298520080626 ) ) ;
#33311=CARTESIAN_POINT ( 'NONE',  ( -84.20019048342901158, 24.50704008690495428, 86.53502039815329283 ) ) ;
#33313=CARTESIAN_POINT ( 'NONE',  ( 133.4058733589413066, 42.32720528873923627, 29.51034083899532590 ) ) ;
#33314=CARTESIAN_POINT ( 'NONE',  ( 8.000000000000007105, 249.8719672152120381, 94.99999999999866418 ) ) ;
#33316=DIRECTION ( 'NONE',  ( -0.000000000000000000, 1.000000000000000000, -0.000000000000000000 ) ) ;
#33322=ORIENTED_EDGE ( 'NONE', *, *, #3794, .T. ) ;
#33324=CARTESIAN_POINT ( 'NONE',  ( 56.52205390515079131, 12.28646189164058988, 67.94243928922777798 ) ) ;
#33329=CARTESIAN_POINT ( 'NONE',  ( 87.30556659420746257, 20.71715946144239950, 83.42470827707606418 ) ) ;
#33330=VECTOR ( 'NONE', #26037, 1000.000000000000000 ) ;
#33334=CARTESIAN_POINT ( 'NONE',  ( -127.6861178856153174, 47.68458428355327072, 18.57198835803803050 ) ) ;
#33335=CARTESIAN_POINT ( 'NONE',  ( -125.8938041572051389, -170.0000000000000000, 3.775397282693376155 ) ) ;
#33337=CARTESIAN_POINT ( 'NONE',  ( -133.2787743207941276, 52.78950725740544669, -41.07782338636832975 ) ) ;
#33339=CARTESIAN_POINT ( 'NONE',  ( -119.5576859660651508, 42.46117483543971360, -46.43479381264184980 ) ) ;
#33342=CARTESIAN_POINT ( 'NONE',  ( -6.843910203392210789, 7.836697961436722260, -62.31111058179082818 ) ) ;
#33345=CARTESIAN_POINT ( 'NONE',  ( 163.8779926341230748, 64.12131166777415103, -93.39151763476601786 ) ) ;
#33346=CARTESIAN_POINT ( 'NONE',  ( 197.6145711261845008, 97.10888456119690204, -46.37243094951851674 ) ) ;
#33348=CARTESIAN_POINT ( 'NONE',  ( -101.3502439362134879, 33.43728945125134544, 30.56238026629964466 ) ) ;
#33349=CARTESIAN_POINT ( 'NONE',  ( 22.80839748737787787, 6.826915557457470030, -45.67001842980409521 ) ) ;
#33350=CARTESIAN_POINT ( 'NONE',  ( 113.4402889550712672, 31.50582881646777622, 17.06772458018410177 ) ) ;
#33359=CARTESIAN_POINT ( 'NONE',  ( -35.47785446961778177, 11.31170061832250973, -90.17238499101478055 ) ) ;
#33361=CARTESIAN_POINT ( 'NONE',  ( -10.24974837193994581, 8.069704751038630164, -62.64850511569373737 ) ) ;
#33362=ORIENTED_EDGE ( 'NONE', *, *, #60960, .T. ) ;
#33364=EDGE_CURVE ( 'NONE', #8399, #21982, #24459, .T. ) ;
#33366=DIRECTION ( 'NONE',  ( -0.000000000000000000, 1.000000000000000000, -0.000000000000000000 ) ) ;
#33372=CARTESIAN_POINT ( 'NONE',  ( -38.92726670956013635, 10.94099576009806718, -16.46139659267618427 ) ) ;
#33373=CARTESIAN_POINT ( 'NONE',  ( -174.7903139851460423, 90.53182997092832807, 45.64566177438910444 ) ) ;
#33375=CARTESIAN_POINT ( 'NONE',  ( 20.74185656603722450, 7.717159106492281317, 58.70619541278092157 ) ) ;
#33376=EDGE_CURVE ( 'NONE', #58488, #66136, #5562, .T. ) ;
#33377=B_SPLINE_CURVE_WITH_KNOTS ( 'NONE', 3,
 ( #37540, #69206, #48415, #21706, #31579, #4842, #21362, #42809, #16441, #956, #64277, #58991, #64626, #603, #11152, #47742, #15746, #37195, #53359, #17112, #11487, #53015, #37895, #59675, #26312, #59340, #54398, #5869, #32617, #5195, #22408, #32960, #21030, #43155, #42475, #26650, #248, #48085, #54044, #43848, #22059, #27325, #63935, #58640, #48766 ),
 .UNSPECIFIED., .F., .F.,
 ( 4, 2, 2, 1, 2, 2, 2, 2, 2, 2, 2, 2, 2, 2, 2, 2, 2, 2, 2, 2, 2, 2, 4 ),
 ( 0.02348395315094740227, 0.02495010856601299204, 0.02568318627354578693, 0.02641626398107858181, 0.02714934168861137670, 0.02788241939614417159, 0.02934857481120974748, 0.03008165251874254584, 0.03081473022627534419, 0.03228088564134092009, 0.03301396334887372191, 0.03374704105640652374, 0.03521319647147211351, 0.03667935188653771716, 0.03741242959407050511, 0.03814550730160329306, 0.03961166271666886896, 0.04107781813173444485, 0.04254397354680002075, 0.04327705125433281563, 0.04401012896186559664, 0.04547628437693117254, 0.04694243979199674843 ),
 .UNSPECIFIED. ) ;
#33378=ORIENTED_EDGE ( 'NONE', *, *, #26592, .T. ) ;
#33379=VERTEX_POINT ( 'NONE', #68396 ) ;
#33381=DIRECTION ( 'NONE',  ( 1.000000000000000000, 0.000000000000000000, -0.000000000000000000 ) ) ;
#33382=CARTESIAN_POINT ( 'NONE',  ( -104.7956873821848944, 35.21322275870666374, 4.105111570260970844 ) ) ;
#33383=CARTESIAN_POINT ( 'NONE',  ( -35.38560449531984631, 10.27249159032102099, -49.19954030868971984 ) ) ;
#33384=DIRECTION ( 'NONE',  ( -0.000000000000000000, 1.000000000000000000, -0.000000000000000000 ) ) ;
#33387=CARTESIAN_POINT ( 'NONE',  ( -71.17846906053300415, 20.67346400882179935, -16.26539829717355801 ) ) ;
#33388=CARTESIAN_POINT ( 'NONE',  ( 81.04675113612957205, 17.59091904316105826, 69.08915744240043466 ) ) ;
#33392=CARTESIAN_POINT ( 'NONE',  ( 207.4867844023103487, 110.2451255333963474, -63.69630056086449343 ) ) ;
#33394=CARTESIAN_POINT ( 'NONE',  ( -71.21970990337015905, 19.62334883444992428, 10.04748825087579434 ) ) ;
#33395=CARTESIAN_POINT ( 'NONE',  ( -118.4470345550925714, 42.96051736048244152, 63.92217194901178345 ) ) ;
#33396=CARTESIAN_POINT ( 'NONE',  ( -49.62489392740901906, 13.29305723289024499, 5.791284796356666043 ) ) ;
#33402=CARTESIAN_POINT ( 'NONE',  ( -190.6985136298601731, 109.1272424661242582, 87.66052266422059347 ) ) ;
#33404=FACE_OUTER_BOUND ( 'NONE', #12919, .T. ) ;
#33406=ORIENTED_EDGE ( 'NONE', *, *, #68760, .F. ) ;
#33407=CARTESIAN_POINT ( 'NONE',  ( -82.32931163805224628, 23.75065981441939655, 31.36902022954703995 ) ) ;
#33408=CARTESIAN_POINT ( 'NONE',  ( -27.49195330402087833, 9.993776132065308460, -76.04372912499586334 ) ) ;
#33409=CARTESIAN_POINT ( 'NONE',  ( 46.23304607317103176, 10.41544405387738514, 34.30787760119516605 ) ) ;
#33410=CARTESIAN_POINT ( 'NONE',  ( -29.04258984626622819, 9.210213971636685315, 57.44998931435969780 ) ) ;
#33411=CARTESIAN_POINT ( 'NONE',  ( -146.1142527948576060, 61.35394402951020254, 18.06864745197337285 ) ) ;
#33412=VECTOR ( 'NONE', #3907, 1000.000000000000000 ) ;
#33417=CARTESIAN_POINT ( 'NONE',  ( 31.91383250562745388, 8.564461488296997160, -15.78690365252851535 ) ) ;
#33420=CARTESIAN_POINT ( 'NONE',  ( 140.1490313966874908, 46.55482389929059650, 86.60343140016868801 ) ) ;
#33422=CARTESIAN_POINT ( 'NONE',  ( 197.6319840686292082, 98.73992647122672395, -95.00000000000133582 ) ) ;
#33427=CARTESIAN_POINT ( 'NONE',  ( -120.1497954511983721, 42.82624472369558788, -74.10732019003926041 ) ) ;
#33433=CARTESIAN_POINT ( 'NONE',  ( 136.7507824285648894, 44.38599729999915411, 17.08875733851226997 ) ) ;
#33435=VERTEX_POINT ( 'NONE', #8964 ) ;
#33436=EDGE_CURVE ( 'NONE', #29969, #48053, #14603, .T. ) ;
#33441=ORIENTED_EDGE ( 'NONE', *, *, #11513, .T. ) ;
#33442=CARTESIAN_POINT ( 'NONE',  ( 129.8795108792701569, 39.07419932312295430, -90.84173050637812707 ) ) ;
#33443=EDGE_LOOP ( 'NONE', ( #56650, #56536 ) ) ;
#33446=CARTESIAN_POINT ( 'NONE',  ( 90.91465859190772392, 20.92790537681857543, 4.207571972591185983 ) ) ;
#33453=CARTESIAN_POINT ( 'NONE',  ( 32.89501968360929851, 8.663558833820822258, 41.17552703169613437 ) ) ;
#33454=CARTESIAN_POINT ( 'NONE',  ( -178.5848962563133568, 94.99295350784007042, -37.04987916691930394 ) ) ;
#33459=VERTEX_POINT ( 'NONE', #114 ) ;
#33460=CARTESIAN_POINT ( 'NONE',  ( 140.0820590176526252, 46.51134312115247127, -74.55802468919154080 ) ) ;
#33463=EDGE_LOOP ( 'NONE', ( #51270, #62486 ) ) ;
#33466=FACE_BOUND ( 'NONE', #22016, .T. ) ;
#33468=CARTESIAN_POINT ( 'NONE',  ( -0.3249717932738296899, 6.518578686837487979, -69.27445299358225839 ) ) ;
#33470=CARTESIAN_POINT ( 'NONE',  ( -144.3939084932120807, 61.25241660819418144, -9.976470740476594656 ) ) ;
#33471=CARTESIAN_POINT ( 'NONE',  ( -125.8938041572051389, 47.69968343338778283, -49.91370389823397602 ) ) ;
#33472=CARTESIAN_POINT ( 'NONE',  ( -2.869721780807576561, 7.625909776230886727, 43.26631488255254254 ) ) ;
#33475=CARTESIAN_POINT ( 'NONE',  ( -7.330587818645180498, 7.867004275019543691, -8.573520141480125645 ) ) ;
#33476=CARTESIAN_POINT ( 'NONE',  ( -14.93280618462406828, 8.469244267267917792, 40.02294218869200648 ) ) ;
#33477=CARTESIAN_POINT ( 'NONE',  ( 117.0065308422768453, 32.13872219870569324, 7.015794843079218523 ) ) ;
#33483=CARTESIAN_POINT ( 'NONE',  ( 86.62931800182293784, 20.48449268398423939, -77.66611478937542756 ) ) ;
#33484=CARTESIAN_POINT ( 'NONE',  ( 102.7475671010530220, 26.65887778672039587, 90.36044456738673603 ) ) ;
#33485=DIRECTION ( 'NONE',  ( 0.000000000000000000, 0.000000000000000000, 1.000000000000000000 ) ) ;
#33486=CARTESIAN_POINT ( 'NONE',  ( -15.14442107647020563, 7.478650287766785532, 89.63505923903740324 ) ) ;
#33487=CARTESIAN_POINT ( 'NONE',  ( -26.88234027341226096, 9.904106450608203716, -48.79416700654920902 ) ) ;
#33488=CYLINDRICAL_SURFACE ( 'NONE', #49003, 7.500000000000013323 ) ;
#33489=CARTESIAN_POINT ( 'NONE',  ( -72.44920908684991900, 21.11636224409796370, -92.10391607065253083 ) ) ;
#33493=CARTESIAN_POINT ( 'NONE',  ( 31.90247004928964358, 8.563336936370815167, 63.75499471202854096 ) ) ;
#33496=CARTESIAN_POINT ( 'NONE',  ( -167.0073208999198755, 82.02183861952781285, 60.81400106796706240 ) ) ;
#33499=EDGE_LOOP ( 'NONE', ( #10904, #11007 ) ) ;
#33500=CARTESIAN_POINT ( 'NONE',  ( 94.11595392909971736, 23.18887043179185170, 10.88183017804118435 ) ) ;
#33501=CARTESIAN_POINT ( 'NONE',  ( 23.09590709048884349, 7.852755081912510704, -41.31320969520013620 ) ) ;
#33502=CARTESIAN_POINT ( 'NONE',  ( -86.10361028793438720, 25.29528064050656866, -16.77258119596484320 ) ) ;
#33503=CARTESIAN_POINT ( 'NONE',  ( -81.96414466956503020, 24.68804580838119733, -89.55477965345060909 ) ) ;
#33505=CARTESIAN_POINT ( 'NONE',  ( 209.5118425285948831, 113.1852661712287471, -11.22590986498565790 ) ) ;
#33506=ADVANCED_FACE ( 'NONE', ( #15615 ), #64841, .F. ) ;
#33507=FACE_BOUND ( 'NONE', #44068, .T. ) ;
#33508=CARTESIAN_POINT ( 'NONE',  ( -62.15324028806258383, 16.70091357159900980, -40.25091533774048003 ) ) ;
#33513=CARTESIAN_POINT ( 'NONE',  ( 132.0249343950657135, 41.49728247212333798, 17.49763525730703506 ) ) ;
#33516=FACE_OUTER_BOUND ( 'NONE', #26408, .T. ) ;
#33517=CARTESIAN_POINT ( 'NONE',  ( 154.0293889979056701, 55.02370422818217577, 3.384461364915644754 ) ) ;
#33530=CARTESIAN_POINT ( 'NONE',  ( 106.6228877857910788, 27.24245963308693419, 43.69709372667754366 ) ) ;
#33532=EDGE_CURVE ( 'NONE', #8631, #50694, #52757, .T. ) ;
#33533=VERTEX_POINT ( 'NONE', #65186 ) ;
#33534=CARTESIAN_POINT ( 'NONE',  ( -7.825402957745087207, -170.0000000000000000, 45.11558103944722120 ) ) ;
#33535=CARTESIAN_POINT ( 'NONE',  ( 162.8034185388970911, 63.22443559329414597, 31.61437189098316480 ) ) ;
#33539=CARTESIAN_POINT ( 'NONE',  ( -49.43836229152576323, 14.28302414152159727, -47.71376574487467792 ) ) ;
#33540=CARTESIAN_POINT ( 'NONE',  ( -49.44484229820454857, 14.28460989390479341, 15.97695875002632881 ) ) ;
#33541=CARTESIAN_POINT ( 'NONE',  ( -128.9863978264384912, 49.78205252558954896, -8.732497812272862703 ) ) ;
#33543=CARTESIAN_POINT ( 'NONE',  ( 70.05403699894507952, 14.41597870224753208, -94.18588356900310998 ) ) ;
#33548=ADVANCED_FACE ( 'NONE', ( #37067 ), #42348, .F. ) ;
#33551=CARTESIAN_POINT ( 'NONE',  ( -13.47680110791658237, 7.324966777230637049, -21.02899547893517607 ) ) ;
#33552=CARTESIAN_POINT ( 'NONE',  ( -167.7367320859366941, 82.78554475141790192, 86.78082447994947302 ) ) ;
#33553=CARTESIAN_POINT ( 'NONE',  ( -47.61380558691495679, 12.81230778489787880, -14.88474268100918607 ) ) ;
#33556=CARTESIAN_POINT ( 'NONE',  ( -62.50103539982530521, 17.85731685071835173, -43.72722077931214812 ) ) ;
#33558=VECTOR ( 'NONE', #20688, 1000.000000000000000 ) ;
#33561=VERTEX_POINT ( 'NONE', #824 ) ;
#33568=CARTESIAN_POINT ( 'NONE',  ( -29.23649411797835995, 10.25826775638764943, 84.22912791894023599 ) ) ;
#33569=CARTESIAN_POINT ( 'NONE',  ( -94.79534239005252516, 29.13842790650044279, -43.05777683239141140 ) ) ;
#33573=CARTESIAN_POINT ( 'NONE',  ( 136.9654665832767932, 44.52067472585215313, -9.849378322202888114 ) ) ;
#33578=CARTESIAN_POINT ( 'NONE',  ( -14.32241591711281714, 7.401556312061831733, 14.52592041517191035 ) ) ;
#33580=CARTESIAN_POINT ( 'NONE',  ( 56.30011474572733476, 11.21470186335419150, -19.72478589053048381 ) ) ;
#33585=CARTESIAN_POINT ( 'NONE',  ( -157.0069704378501569, 70.81086990254190994, 65.64755214383821169 ) ) ;
#33586=CARTESIAN_POINT ( 'NONE',  ( -0.5178428571329642960, 7.532057582089303871, -41.21203124799237116 ) ) ;
#33590=FACE_BOUND ( 'NONE', #10914, .T. ) ;
#33595=CARTESIAN_POINT ( 'NONE',  ( -132.2199390322348620, 50.80243550247267592, -65.19852263477184806 ) ) ;
#33596=CARTESIAN_POINT ( 'NONE',  ( -103.2061297292849531, 34.38496953192503724, -76.81632396160040344 ) ) ;
#33597=CARTESIAN_POINT ( 'NONE',  ( 45.90693067088658808, 9.344800815249323378, -66.19927155725260093 ) ) ;
#33601=CARTESIAN_POINT ( 'NONE',  ( -126.7195977354785867, 47.03939704596392346, -88.63674059282946871 ) ) ;
#33603=CARTESIAN_POINT ( 'NONE',  ( 176.5082832158485360, 74.10150673151672152, 84.54631382975011888 ) ) ;
#33606=CARTESIAN_POINT ( 'NONE',  ( 175.8963338753314360, 73.51705463274393537, -38.30295033125676696 ) ) ;
#33615=CARTESIAN_POINT ( 'NONE',  ( 140.4641697461913168, 46.75994457266056514, 67.44143240493572478 ) ) ;
#33616=CARTESIAN_POINT ( 'NONE',  ( -78.19460645047367109, 22.14203592077027949, -50.11545063171791270 ) ) ;
#33619=CARTESIAN_POINT ( 'NONE',  ( 88.53517449242353621, 20.08005703101045114, -36.06378951590050974 ) ) ;
#33620=CARTESIAN_POINT ( 'NONE',  ( -48.34250119710922888, 14.01879126850789348, -19.23099893068116373 ) ) ;
#33621=EDGE_LOOP ( 'NONE', ( #17613, #36413, #62866, #50306 ) ) ;
#33622=CARTESIAN_POINT ( 'NONE',  ( 116.0773578185793298, 31.67580513411749621, -48.16155069270497080 ) ) ;
#33623=CARTESIAN_POINT ( 'NONE',  ( -71.42546113164834765, 20.75891408601219368, 13.09244254408361741 ) ) ;
#33624=CARTESIAN_POINT ( 'NONE',  ( -142.0729208125266894, 59.40063722436774896, -41.17521488854814748 ) ) ;
#33626=CARTESIAN_POINT ( 'NONE',  ( -121.3504824331598826, 43.57435154345014894, 85.83401817385978916 ) ) ;
#33628=CARTESIAN_POINT ( 'NONE',  ( 55.76255201544532270, 12.13275766515751641, 8.496681876347771833 ) ) ;
#33631=CARTESIAN_POINT ( 'NONE',  ( -55.05276343752909440, 14.68156374112638929, -23.37177340799619785 ) ) ;
#33635=CARTESIAN_POINT ( 'NONE',  ( 181.0840389613909736, 78.60582251573003987, -24.38050707541595230 ) ) ;
#33636=CARTESIAN_POINT ( 'NONE',  ( 139.6359093656973585, 45.02518919224741012, -11.89209978307138904 ) ) ;
#33637=DIRECTION ( 'NONE',  ( 0.000000000000000000, 0.000000000000000000, 1.000000000000000000 ) ) ;
#33638=CARTESIAN_POINT ( 'NONE',  ( 93.33480479917545836, 21.81892021443993457, -66.76901901691363150 ) ) ;
#33639=CARTESIAN_POINT ( 'NONE',  ( -28.14167211390615009, 9.073095087475770981, -89.75665694410322715 ) ) ;
#33641=ORIENTED_EDGE ( 'NONE', *, *, #60011, .T. ) ;
#33643=VERTEX_POINT ( 'NONE', #17337 ) ;
#33644=CARTESIAN_POINT ( 'NONE',  ( 42.49453823366106775, 8.831814337191479680, 44.25087953862465184 ) ) ;
#33649=CARTESIAN_POINT ( 'NONE',  ( 210.5008983495071959, 116.4753531594350733, -39.06839114615122099 ) ) ;
#33650=CARTESIAN_POINT ( 'NONE',  ( 110.2429982417149290, 28.88204397445231209, -77.76698815611739235 ) ) ;
#33651=CARTESIAN_POINT ( 'NONE',  ( -105.8879439778144587, 34.65133284149109727, 58.27111540278865931 ) ) ;
#33652=CARTESIAN_POINT ( 'NONE',  ( -24.33435124463266419, 8.532637995283115728, -40.40188971294399778 ) ) ;
#33655=CARTESIAN_POINT ( 'NONE',  ( -30.94745021534355800, 10.53010394565407637, 18.37190381572551345 ) ) ;
#33658=DIRECTION ( 'NONE',  ( -0.000000000000000000, 1.000000000000000000, -0.000000000000000000 ) ) ;
#33660=DIRECTION ( 'NONE',  ( 0.000000000000000000, 0.000000000000000000, 1.000000000000000000 ) ) ;
#33663=CARTESIAN_POINT ( 'NONE',  ( -102.2801239173131194, -170.0000000000000000, 30.51907450641510522 ) ) ;
#33666=CARTESIAN_POINT ( 'NONE',  ( -166.2425995121691642, 81.22826102820870631, 94.99999999999866418 ) ) ;
#33667=CARTESIAN_POINT ( 'NONE',  ( 209.0273569836735419, 112.4716286368275462, 84.24349562760866661 ) ) ;
#33669=ORIENTED_EDGE ( 'NONE', *, *, #18421, .T. ) ;
#33670=CARTESIAN_POINT ( 'NONE',  ( 55.52751777340357364, 12.08567914268656374, 64.64719063402279176 ) ) ;
#33673=EDGE_CURVE ( 'NONE', #49905, #65743, #17977, .T. ) ;
#33677=CARTESIAN_POINT ( 'NONE',  ( 133.8566784816069060, 42.60093787723652525, -9.178760341931967659 ) ) ;
#33678=EDGE_CURVE ( 'NONE', #12095, #17473, #55725, .T. ) ;
#33679=ORIENTED_EDGE ( 'NONE', *, *, #63110, .F. ) ;
#33684=CARTESIAN_POINT ( 'NONE',  ( -165.7690020878297901, 80.74028011998679233, -43.72344623212075021 ) ) ;
#33685=CARTESIAN_POINT ( 'NONE',  ( -165.6309143132208987, 79.16027303391220471, 91.58517648874418171 ) ) ;
#33687=CARTESIAN_POINT ( 'NONE',  ( -125.8938041572051105, 46.49392987655492959, -49.91370389823397602 ) ) ;
#33690=CARTESIAN_POINT ( 'NONE',  ( -0.7211439451572416726, 7.539282923622936394, -67.34605877822407649 ) ) ;
#33694=CARTESIAN_POINT ( 'NONE',  ( -61.76386578474846090, 17.63453064612501109, 7.588056654894035802 ) ) ;
#33695=CARTESIAN_POINT ( 'NONE',  ( 198.8687991397276278, 98.67887821384414337, -48.55222848310017270 ) ) ;
#33697=CARTESIAN_POINT ( 'NONE',  ( -95.86163447241558799, 30.75089131639703410, 34.10712415686030852 ) ) ;
#33699=CARTESIAN_POINT ( 'NONE',  ( 22.81270948571150115, 6.827178363529887939, -40.37925852579917319 ) ) ;
#33700=CARTESIAN_POINT ( 'NONE',  ( 111.1829448509513298, 30.43012797723691776, 17.72218487494545514 ) ) ;
#33701=ORIENTED_EDGE ( 'NONE', *, *, #48713, .F. ) ;
#33705=CARTESIAN_POINT ( 'NONE',  ( -71.37402418445427088, 19.67651958824263048, -17.54144548817878402 ) ) ;
#33707=CARTESIAN_POINT ( 'NONE',  ( -13.29455179262033226, 8.319166883236668752, -74.90053121910786160 ) ) ;
#33709=CARTESIAN_POINT ( 'NONE',  ( 164.4615316623334991, 63.29763980349832764, 34.18048905360906531 ) ) ;
#33715=CARTESIAN_POINT ( 'NONE',  ( -38.55214349681828168, 10.86754840574842262, -18.40125661905821630 ) ) ;
#33716=CARTESIAN_POINT ( 'NONE',  ( 113.4402889550712530, 31.50582881646776912, 43.91227517064776009 ) ) ;
#33717=CARTESIAN_POINT ( 'NONE',  ( -131.2955621888335713, 51.38237199780174080, 6.050075014823135255 ) ) ;
#33718=CARTESIAN_POINT ( 'NONE',  ( 23.03546163277112413, 7.848986635155161373, 66.30567845553197515 ) ) ;
#33721=VERTEX_POINT ( 'NONE', #8184 ) ;
#33722=CARTESIAN_POINT ( 'NONE',  ( 211.0271454480929663, 115.4465235294104986, -93.48507865360365088 ) ) ;
#33725=CARTESIAN_POINT ( 'NONE',  ( -35.99019277275121453, 10.38248800679341954, -36.83593714842513123 ) ) ;
#33726=CARTESIAN_POINT ( 'NONE',  ( -95.72254973812390233, 29.57223513374536594, 88.01148943108383094 ) ) ;
#33728=CARTESIAN_POINT ( 'NONE',  ( -190.6985136298601731, 109.1272424661242582, -46.56223028809779407 ) ) ;
#33729=CARTESIAN_POINT ( 'NONE',  ( -72.21889834709580214, 21.03534256744169539, -11.90770200485403940 ) ) ;
#33732=VERTEX_POINT ( 'NONE', #25413 ) ;
#33733=CARTESIAN_POINT ( 'NONE',  ( 32.46582151331404731, 7.608418548522502434, 40.29821503774315516 ) ) ;
#33736=CARTESIAN_POINT ( 'NONE',  ( 188.2988323915788271, 86.21831227955478028, 38.87825967812030825 ) ) ;
#33739=CARTESIAN_POINT ( 'NONE',  ( -51.35181696773307891, 13.72007042346227479, 4.431000077818415761 ) ) ;
#33743=CARTESIAN_POINT ( 'NONE',  ( 163.1370549780984049, 63.50181104276889243, -75.40761482696586882 ) ) ;
#33746=CARTESIAN_POINT ( 'NONE',  ( 204.6977192012829789, -170.0000000000000000, -43.82593103262159673 ) ) ;
#33754=EDGE_CURVE ( 'NONE', #38092, #59735, #63024, .T. ) ;
#33755=CARTESIAN_POINT ( 'NONE',  ( 39.89582146299186860, 9.488756994579086168, 44.91383430596328452 ) ) ;
#33761=ORIENTED_EDGE ( 'NONE', *, *, #14611, .T. ) ;
#33762=CARTESIAN_POINT ( 'NONE',  ( -55.05276343752910151, -170.0000000000000000, -69.56087458892355357 ) ) ;
#33763=DIRECTION ( 'NONE',  ( 1.000000000000000000, 0.000000000000000000, -0.000000000000000000 ) ) ;
#33764=CARTESIAN_POINT ( 'NONE',  ( 141.3354458183166287, 47.33100220280247328, 90.10713329041466579 ) ) ;
#33775=CARTESIAN_POINT ( 'NONE',  ( 139.3067271572849677, 44.81402783181202665, -65.20950923262978449 ) ) ;
#33777=VERTEX_POINT ( 'NONE', #40530 ) ;
#33783=DIRECTION ( 'NONE',  ( -0.000000000000000000, 1.000000000000000000, -0.000000000000000000 ) ) ;
#33785=CARTESIAN_POINT ( 'NONE',  ( 93.70675391435744928, 21.95852801827565770, 7.872820059410217119 ) ) ;
#33787=ORIENTED_EDGE ( 'NONE', *, *, #68677, .F. ) ;
#33790=CARTESIAN_POINT ( 'NONE',  ( 36.98541457540710553, 9.120571655722420346, 44.53055877612269597 ) ) ;
#33791=CARTESIAN_POINT ( 'NONE',  ( 66.30230369578305272, 14.49551544185123753, 30.56703610697686102 ) ) ;
#33792=CARTESIAN_POINT ( 'NONE',  ( -125.8938041572051105, 46.49392987655492959, -23.06915330777029638 ) ) ;
#33793=CARTESIAN_POINT ( 'NONE',  ( -146.3604280344345909, 61.55502468262317706, -89.18082157871309334 ) ) ;
#33794=CARTESIAN_POINT ( 'NONE',  ( 133.3996297101683979, 41.14871796345731525, -62.86786152285935003 ) ) ;
#33800=CARTESIAN_POINT ( 'NONE',  ( -0.5183605925911991541, 6.525266619725957007, -71.47052751656273983 ) ) ;
#33801=CARTESIAN_POINT ( 'NONE',  ( -37.37206033059242571, 11.66494618096613145, 33.12183574046159151 ) ) ;
#33802=CARTESIAN_POINT ( 'NONE',  ( -144.7530445311634821, 61.54314312182905411, -21.27383361102199189 ) ) ;
#33805=CYLINDRICAL_SURFACE ( 'NONE', #54616, 7.500000000000013323 ) ;
#33808=CARTESIAN_POINT ( 'NONE',  ( -2.873329055852802405, 7.626065826870667586, -21.72791809929673690 ) ) ;
#33809=CARTESIAN_POINT ( 'NONE',  ( -11.13714165684777946, 8.138643170880698108, 30.88190552611061435 ) ) ;
#33810=CARTESIAN_POINT ( 'NONE',  ( 116.1021807117071631, 31.68810634233422263, 14.97497448979273571 ) ) ;
#33813=CARTESIAN_POINT ( 'NONE',  ( -101.8140949286062380, 33.67224128592402366, -35.01457726497591239 ) ) ;
#33816=CARTESIAN_POINT ( 'NONE',  ( 79.13041963748371188, 18.04952109592811382, -70.68632447848128209 ) ) ;
#33817=CARTESIAN_POINT ( 'NONE',  ( 104.1111664609392022, 27.24250349207208899, 86.46839379475228782 ) ) ;
#33825=CARTESIAN_POINT ( 'NONE',  ( -118.8691191306315460, 43.21907118237575673, -12.92847206412439220 ) ) ;
#33832=CARTESIAN_POINT ( 'NONE',  ( 46.47744650267831190, 9.435478116178785513, -94.18279426279515576 ) ) ;
#33834=CARTESIAN_POINT ( 'NONE',  ( -125.8938041572051389, -170.0000000000000000, 38.11994787315708777 ) ) ;
#33839=CARTESIAN_POINT ( 'NONE',  ( 87.59078297315400619, 20.81577753000345155, 2.914042839113803129 ) ) ;
#33840=CARTESIAN_POINT ( 'NONE',  ( 23.23965501943000334, 7.861749956303022202, -44.00267626036002611 ) ) ;
#33841=CARTESIAN_POINT ( 'NONE',  ( 15.78827728214693416, 7.507518794609588042, 56.85925826316891829 ) ) ;
#33844=FACE_BOUND ( 'NONE', #44590, .T. ) ;
#33845=CARTESIAN_POINT ( 'NONE',  ( 161.7006237583813117, 62.31514460450498660, 57.54382807939717992 ) ) ;
#33846=EDGE_CURVE ( 'NONE', #3228, #964, #52471, .T. ) ;
#33847=ORIENTED_EDGE ( 'NONE', *, *, #22312, .F. ) ;
#33852=CARTESIAN_POINT ( 'NONE',  ( 153.4268936273268196, 54.57409659828383752, 3.743913822929773705 ) ) ;
#33859=ORIENTED_EDGE ( 'NONE', *, *, #7636, .T. ) ;
#33864=CARTESIAN_POINT ( 'NONE',  ( 89.88147981065576175, 21.62466191578946706, -63.39067841512786572 ) ) ;
#33865=ORIENTED_EDGE ( 'NONE', *, *, #2659, .F. ) ;
#33868=CARTESIAN_POINT ( 'NONE',  ( 39.89582146299186860, 9.488756994579084392, 71.75838489642696061 ) ) ;
#33870=CARTESIAN_POINT ( 'NONE',  ( -151.2511071212631464, 67.00426547928869070, -61.84963319502005419 ) ) ;
#33871=CARTESIAN_POINT ( 'NONE',  ( 69.35866309798980467, 15.27376159675663736, 14.47800203215017056 ) ) ;
#33873=AXIS2_PLACEMENT_3D ( 'NONE', #46661, #20275, #9382 ) ;
#33879=CARTESIAN_POINT ( 'NONE',  ( -48.70883077256302585, 14.10659259062419046, 6.964640123796999482 ) ) ;
#33881=CARTESIAN_POINT ( 'NONE',  ( -156.4859261060826157, 71.69908252863689313, -93.24215537093068917 ) ) ;
#33882=CARTESIAN_POINT ( 'NONE',  ( 113.4351684956570239, 30.38657459074491030, -23.38094634528284743 ) ) ;
#33883=CARTESIAN_POINT ( 'NONE',  ( 93.28163122584956568, 21.79878316975275965, 94.43086186953131289 ) ) ;
#33885=ORIENTED_EDGE ( 'NONE', *, *, #25827, .T. ) ;
#33891=CARTESIAN_POINT ( 'NONE',  ( -49.62489392740900485, 13.29305723289023966, -21.05326579410700560 ) ) ;
#33894=CARTESIAN_POINT ( 'NONE',  ( -38.45778834351242637, 11.87434869453506892, 67.21600681512579456 ) ) ;
#33896=CARTESIAN_POINT ( 'NONE',  ( -71.96390573417174608, 19.88067451234327621, -66.05669224067524681 ) ) ;
#33897=CARTESIAN_POINT ( 'NONE',  ( -7.825402957745083654, 6.891034867348166060, 30.11558103944718923 ) ) ;
#33901=ORIENTED_EDGE ( 'NONE', *, *, #19860, .T. ) ;
#33902=EDGE_LOOP ( 'NONE', ( #17342, #63373, #15000, #33701 ) ) ;
#33903=CARTESIAN_POINT ( 'NONE',  ( -142.0070007485041117, 59.34878529741514086, 11.10676733467697730 ) ) ;
#33904=CARTESIAN_POINT ( 'NONE',  ( -61.00567534907362699, 17.40801984996452489, -91.82290913100322882 ) ) ;
#33905=CARTESIAN_POINT ( 'NONE',  ( -38.02163356681019479, 11.78964455120423693, 94.99999999999866418 ) ) ;
#33906=CARTESIAN_POINT ( 'NONE',  ( 110.2429982417149432, 29.99119854320847267, -24.07788697519002596 ) ) ;
#33908=LINE ( 'NONE', #7173, #35944 ) ;
#33909=CARTESIAN_POINT ( 'NONE',  ( 135.6793972494602940, 43.71805072851429230, -23.96845213928238039 ) ) ;
#33916=DIRECTION ( 'NONE',  ( -0.000000000000000000, 1.000000000000000000, -0.000000000000000000 ) ) ;
#33917=CARTESIAN_POINT ( 'NONE',  ( 31.90184941268615759, 7.552181687745349592, -70.20641173465664053 ) ) ;
#33918=CARTESIAN_POINT ( 'NONE',  ( 59.72897338775215559, 11.93428797217974768, -23.12208266423090919 ) ) ;
#33923=CARTESIAN_POINT ( 'NONE',  ( -54.57280099357649306, 14.55288945003959888, 30.31732777293113656 ) ) ;
#33926=CARTESIAN_POINT ( 'NONE',  ( -58.76099769480629220, 16.75353773354895281, -63.03723493735800787 ) ) ;
#33928=VECTOR ( 'NONE', #5570, 1000.000000000000000 ) ;
#33929=CARTESIAN_POINT ( 'NONE',  ( -0.5658006089934872751, 7.533733779014707643, -44.86461209534569861 ) ) ;
#33931=CARTESIAN_POINT ( 'NONE',  ( -168.7187482717114051, 82.35796501763486788, 5.386810785733501028 ) ) ;
#33933=FACE_BOUND ( 'NONE', #63687, .T. ) ;
#33934=CARTESIAN_POINT ( 'NONE',  ( -189.3696967735686485, 107.2697815289672718, 90.68589341612421606 ) ) ;
#33935=VECTOR ( 'NONE', #19877, 1000.000000000000000 ) ;
#33937=VECTOR ( 'NONE', #26690, 1000.000000000000000 ) ;
#33938=ORIENTED_EDGE ( 'NONE', *, *, #24887, .F. ) ;
#33940=CARTESIAN_POINT ( 'NONE',  ( -127.6861178856153174, 47.68458428355325651, -61.96166341335298000 ) ) ;
#33941=CYLINDRICAL_SURFACE ( 'NONE', #63535, 7.500000000000013323 ) ;
#33948=CARTESIAN_POINT ( 'NONE',  ( 178.9572806431051788, 76.48101739820698697, 83.28229297188985925 ) ) ;
#33951=CARTESIAN_POINT ( 'NONE',  ( 173.7246046907419554, 71.47482343504563573, -42.25086531254567745 ) ) ;
#33952=CARTESIAN_POINT ( 'NONE',  ( 150.4722669492348643, 53.65054032737663192, 34.19824095576758083 ) ) ;
#33955=CARTESIAN_POINT ( 'NONE',  ( 111.1865443042261603, 30.43181341527237649, 56.50051719710833709 ) ) ;
#33956=CARTESIAN_POINT ( 'NONE',  ( -178.2381786520593607, 93.01028335822124404, 16.96567094477213189 ) ) ;
#33959=FACE_OUTER_BOUND ( 'NONE', #54815, .T. ) ;
#33960=CARTESIAN_POINT ( 'NONE',  ( -47.55316895016325418, 13.83165595246916801, -15.36910518223855426 ) ) ;
#33962=CARTESIAN_POINT ( 'NONE',  ( -123.4416615615273258, 44.90042688650401459, -8.477572847294975844 ) ) ;
#33963=CARTESIAN_POINT ( 'NONE',  ( -71.22896441287282698, 20.69091426169409687, 10.07455366818023279 ) ) ;
#33964=CARTESIAN_POINT ( 'NONE',  ( -145.5195986658808920, 62.16746116576787529, -48.66889029199882799 ) ) ;
#33966=CARTESIAN_POINT ( 'NONE',  ( -133.3249632897631614, 51.58572645347020824, 90.73949300795004547 ) ) ;
#33968=CARTESIAN_POINT ( 'NONE',  ( 79.92465405224848496, 17.24122384219593940, -39.92366204608148195 ) ) ;
#33973=CARTESIAN_POINT ( 'NONE',  ( 86.14890207173841929, 20.31981596387579714, 44.71208757247934074 ) ) ;
#33975=CARTESIAN_POINT ( 'NONE',  ( 93.43270425363546394, 22.93046121381056324, 34.04559475132371205 ) ) ;
#33977=CARTESIAN_POINT ( 'NONE',  ( 134.7770330630252715, 41.98246829846534922, -9.221158025336912090 ) ) ;
#33979=CARTESIAN_POINT ( 'NONE',  ( 20.11619980831799737, 7.685075536026321430, -90.56824105099134670 ) ) ;
#33983=B_SPLINE_CURVE_WITH_KNOTS ( 'NONE', 3,
 ( #37645, #48185, #47850, #4604, #69316, #21468, #21142, #42585, #64041, #11, #56571, #36501, #29838, #20316, #8393, #18942, #24580, #8747, #41780, #25951, #25268, #14694 ),
 .UNSPECIFIED., .F., .F.,
 ( 4, 2, 2, 2, 2, 2, 2, 2, 2, 2, 4 ),
 ( 9.309503074677274191E-17, 0.001318139496345288294, 0.001977209244517854486, 0.002636278992690420462, 0.003954418489035491265, 0.005272557985380562501, 0.005931627733553119369, 0.006590697481725675370, 0.007908836978070793444, 0.009226976474415910651, 0.01054511597076102612 ),
 .UNSPECIFIED. ) ;
#33984=ORIENTED_EDGE ( 'NONE', *, *, #58575, .F. ) ;
#33987=CYLINDRICAL_SURFACE ( 'NONE', #52033, 7.500000000000013323 ) ;
#33990=CARTESIAN_POINT ( 'NONE',  ( 204.6977192012829505, 108.0580384837234931, -51.32593103262161094 ) ) ;
#33993=CARTESIAN_POINT ( 'NONE',  ( -23.95096213915836714, 8.481591526885946308, -42.32845173688443907 ) ) ;
#33999=CYLINDRICAL_SURFACE ( 'NONE', #12833, 7.500000000000020428 ) ;
#34001=CARTESIAN_POINT ( 'NONE',  ( -85.34215807311493052, 24.97769003780924280, 68.19029523188604003 ) ) ;
#34002=CARTESIAN_POINT ( 'NONE',  ( 126.3681350380371242, 38.23508791628619718, 37.50295032406403095 ) ) ;
#34003=CARTESIAN_POINT ( 'NONE',  ( 8.000000000000007105, 249.8719672152120381, 94.99999999999866418 ) ) ;
#34006=CARTESIAN_POINT ( 'NONE',  ( -101.8187363387487210, 33.67461140603126779, -23.17002667451226472 ) ) ;
#34007=CARTESIAN_POINT ( 'NONE',  ( 57.57684776206770749, 12.50442334002048206, 32.14292840263019002 ) ) ;
#34008=CARTESIAN_POINT ( 'NONE',  ( 35.07461521969879215, 7.885994798980979326, 84.96838794907451131 ) ) ;
#34013=CARTESIAN_POINT ( 'NONE',  ( -190.4966031023458299, 108.8421921967458701, -37.93375413894162307 ) ) ;
#34015=CARTESIAN_POINT ( 'NONE',  ( -109.7078892845591298, 36.71702188566217018, -68.28782286830018222 ) ) ;
#34016=CARTESIAN_POINT ( 'NONE',  ( -96.04542865839948718, 29.72476396586411340, -92.00996532311685883 ) ) ;
#34020=CARTESIAN_POINT ( 'NONE',  ( -189.9554299271397895, 108.0836897899587825, -12.03754007755143718 ) ) ;
#34024=DIRECTION ( 'NONE',  ( -0.000000000000000000, 1.000000000000000000, -0.000000000000000000 ) ) ;
#34026=LINE ( 'NONE', #65336, #47000 ) ;
#34028=CARTESIAN_POINT ( 'NONE',  ( -3.244108878396733786, 6.635632329121485817, -10.11498957647276598 ) ) ;
#34033=VECTOR ( 'NONE', #23014, 1000.000000000000000 ) ;
#34036=CARTESIAN_POINT ( 'NONE',  ( 164.1849564601154441, 64.37948657927526597, -93.96497455420622202 ) ) ;
#34040=CARTESIAN_POINT ( 'NONE',  ( 16.76400266940279948, 6.533513613209221305, -50.47150667450311090 ) ) ;
#34043=CARTESIAN_POINT ( 'NONE',  ( 61.09275639403235658, 12.23448398202910248, 30.04748534290944662 ) ) ;
#34046=CARTESIAN_POINT ( 'NONE',  ( -125.4859928193505567, 46.22544753638531034, -88.60280507916128556 ) ) ;
#34047=CARTESIAN_POINT ( 'NONE',  ( -78.66644367742111399, -170.0000000000000000, 64.76275173013681297 ) ) ;
#34048=CARTESIAN_POINT ( 'NONE',  ( -11.78188048797445298, 8.190559674012732216, -76.13891883678253691 ) ) ;
#34054=EDGE_LOOP ( 'NONE', ( #7642, #69282 ) ) ;
#34055=CARTESIAN_POINT ( 'NONE',  ( 207.2640160519426615, 111.6867652229576322, -77.72071523413366378 ) ) ;
#34057=CARTESIAN_POINT ( 'NONE',  ( -109.6829043543429236, -170.0000000000000000, -95.00000000000133582 ) ) ;
#34058=EDGE_CURVE ( 'NONE', #49097, #5706, #59113, .T. ) ;
#34060=CARTESIAN_POINT ( 'NONE',  ( -179.2210908201800805, 95.76260491022611632, 42.71376849300861522 ) ) ;
#34061=CARTESIAN_POINT ( 'NONE',  ( 132.9453095272139365, 42.04754713161464252, 71.35489142945908725 ) ) ;
#34062=CARTESIAN_POINT ( 'NONE',  ( 16.27775141556968919, 7.523247835309962106, 56.85925826316893961 ) ) ;
#34070=AXIS2_PLACEMENT_3D ( 'NONE', #43819, #28352, #7946 ) ;
#34071=CARTESIAN_POINT ( 'NONE',  ( -35.17600017528511813, 10.23461991275926941, -49.32454204471093107 ) ) ;
#34072=CARTESIAN_POINT ( 'NONE',  ( -98.59957010994544646, 30.95006567008976717, 85.16634146005831951 ) ) ;
#34074=VECTOR ( 'NONE', #4028, 1000.000000000000000 ) ;
#34076=CARTESIAN_POINT ( 'NONE',  ( -61.68940124183719576, 17.61226241086874467, 94.99999999999866418 ) ) ;
#34077=EDGE_CURVE ( 'NONE', #3372, #8866, #41524, .T. ) ;
#34082=CARTESIAN_POINT ( 'NONE',  ( 36.76746179515745183, 8.081433644308903652, 44.44018405963787188 ) ) ;
#34088=EDGE_CURVE ( 'NONE', #62698, #26121, #23088, .T. ) ;
#34091=CARTESIAN_POINT ( 'NONE',  ( -8.314488422519710653, 7.931352979988683494, -50.41807073194384969 ) ) ;
#34092=AXIS2_PLACEMENT_3D ( 'NONE', #23785, #56133, #6901 ) ;
#34093=CARTESIAN_POINT ( 'NONE',  ( 151.6192474229129630, 53.24103268919210308, -48.32307074035101380 ) ) ;
#34095=VERTEX_POINT ( 'NONE', #19688 ) ;
#34098=ORIENTED_EDGE ( 'NONE', *, *, #29858, .T. ) ;
#34101=DIRECTION ( 'NONE',  ( -0.000000000000000000, 1.000000000000000000, -0.000000000000000000 ) ) ;
#34102=EDGE_LOOP ( 'NONE', ( #6876, #6628 ) ) ;
#34103=CARTESIAN_POINT ( 'NONE',  ( -86.10361028793440141, 25.29528064050660419, 36.91651998496248410 ) ) ;
#34104=CARTESIAN_POINT ( 'NONE',  ( -10.46803069297985900, 7.077485182625207649, -62.73931412836061838 ) ) ;
#34105=CARTESIAN_POINT ( 'NONE',  ( 41.80372346091801461, 9.750024116765237281, 44.52309710506295204 ) ) ;
#34106=CARTESIAN_POINT ( 'NONE',  ( 140.0614732283738704, 45.29930344725071478, -47.74382409638028690 ) ) ;
#34109=VERTEX_POINT ( 'NONE', #35175 ) ;
#34112=CARTESIAN_POINT ( 'NONE',  ( -5.417282889646091171, 7.753782747238993522, 17.87817252730139828 ) ) ;
#34113=CARTESIAN_POINT ( 'NONE',  ( -1.328627985309865034, 7.561890325089884790, 60.70477836359661694 ) ) ;
#34115=CARTESIAN_POINT ( 'NONE',  ( 198.4963257495732023, 99.83071316188434707, -93.29099697683768966 ) ) ;
#34121=CARTESIAN_POINT ( 'NONE',  ( 164.6406716478537646, 63.44801348349338355, -18.99558380653978418 ) ) ;
#34124=CARTESIAN_POINT ( 'NONE',  ( 63.98009977735161158, 12.89803120691696314, 56.70387718321437376 ) ) ;
#34125=CARTESIAN_POINT ( 'NONE',  ( 136.1310312718402429, 42.81430973242788696, -63.20608120636161686 ) ) ;
#34128=ORIENTED_EDGE ( 'NONE', *, *, #59778, .F. ) ;
#34130=VERTEX_POINT ( 'NONE', #24293 ) ;
#34132=CARTESIAN_POINT ( 'NONE',  ( 10.83046137699561484, 6.392429922561258415, 43.16356064574667073 ) ) ;
#34134=CARTESIAN_POINT ( 'NONE',  ( -61.52143283897137138, 16.51181063611438304, -73.36460479103185151 ) ) ;
#34138=ORIENTED_EDGE ( 'NONE', *, *, #68835, .T. ) ;
#34139=CARTESIAN_POINT ( 'NONE',  ( -147.3641864666714980, 62.38213854487952403, -76.35815727694746613 ) ) ;
#34140=CARTESIAN_POINT ( 'NONE',  ( 89.21005684773506061, 20.31770592753387206, 3.321479991859375591 ) ) ;
#34146=CARTESIAN_POINT ( 'NONE',  ( 62.38471166598394291, 13.55946638994290154, 83.52142562900598932 ) ) ;
#34147=CARTESIAN_POINT ( 'NONE',  ( 37.46876540261052924, 9.179568636624026112, 30.16313010050332011 ) ) ;
#34148=CARTESIAN_POINT ( 'NONE',  ( -180.6158171975815208, 97.47361786002628037, -42.53633187762700629 ) ) ;
#34150=CARTESIAN_POINT ( 'NONE',  ( -133.3392045760936639, 51.59583146030205825, -16.62341006324014359 ) ) ;
#34151=CARTESIAN_POINT ( 'NONE',  ( -143.7563954441272926, 59.45082218538873065, -91.18228907187790355 ) ) ;
#34155=CARTESIAN_POINT ( 'NONE',  ( 141.2801018238827169, 47.29457739955284268, -69.26552387562287549 ) ) ;
#34157=ORIENTED_EDGE ( 'NONE', *, *, #46843, .F. ) ;
#34158=EDGE_CURVE ( 'NONE', #61600, #28307, #47354, .T. ) ;
#34159=CARTESIAN_POINT ( 'NONE',  ( -157.0079874970173250, 72.18249880494042259, -42.03918860550044911 ) ) ;
#34160=CARTESIAN_POINT ( 'NONE',  ( 208.5884523568772124, 113.6152425727545108, -10.55554601564709749 ) ) ;
#34161=CARTESIAN_POINT ( 'NONE',  ( -33.85171821065139852, 11.02091558840053942, 44.83441027425075731 ) ) ;
#34162=CARTESIAN_POINT ( 'NONE',  ( -169.1041038606267080, 82.76530082651281361, -48.56111750552656048 ) ) ;
#34163=CARTESIAN_POINT ( 'NONE',  ( 86.62931800182293784, -170.0000000000000000, -43.32156419891173016 ) ) ;
#34164=CARTESIAN_POINT ( 'NONE',  ( -13.72143910172259318, 7.346845691402125844, -91.95266834806231770 ) ) ;
#34165=CARTESIAN_POINT ( 'NONE',  ( -50.13771638889892301, 13.41835215703893702, -63.87468226647597902 ) ) ;
#34166=CARTESIAN_POINT ( 'NONE',  ( -0.5783162822156591165, 7.534184941292927817, -14.12672653011558488 ) ) ;
#34167=CARTESIAN_POINT ( 'NONE',  ( -15.32584732649904247, 8.506915958926390076, 38.10398657133274014 ) ) ;
#34168=CARTESIAN_POINT ( 'NONE',  ( 117.6865880453675999, 32.48051379280607165, 9.211411928219352063 ) ) ;
#34172=CARTESIAN_POINT ( 'NONE',  ( -94.83794676023109105, 30.26879337035744655, -41.45177952449644465 ) ) ;
#34176=CARTESIAN_POINT ( 'NONE',  ( 84.27937148876360141, 19.69225537006224869, -77.29251801931836496 ) ) ;
#34182=CARTESIAN_POINT ( 'NONE',  ( 56.31655686453512288, 12.24428004209404897, -93.43573692067893433 ) ) ;
#34184=VERTEX_POINT ( 'NONE', #36567 ) ;
#34187=B_SPLINE_CURVE_WITH_KNOTS ( 'NONE', 3,
 ( #3293, #23706, #66628, #13499, #66982, #18424, #45850, #39877, #34956, #8223, #29671, #13158, #34623, #67325, #56061, #7876, #51133, #40230, #51484, #2949, #29326, #45497, #24751, #14193, #8917, #19111, #51819, #62018, #13837, #35300, #42970, #52509, #21525, #5006, #41956, #63418, #69373, #26472, #15222, #58463, #14869, #53177, #3982, #68, #36688, #47221, #9256, #4661, #53529, #58135, #9951, #31407, #46891, #64441, #25793, #52837, #52165, #15911, #31069, #25452, #47909, #5358, #4332, #63065, #36337, #26812, #37025, #26123, #16251 ),
 .UNSPECIFIED., .F., .F.,
 ( 4, 2, 2, 2, 2, 2, 1, 2, 2, 2, 2, 2, 2, 2, 2, 2, 2, 2, 2, 2, 2, 2, 2, 2, 2, 2, 2, 2, 2, 2, 2, 2, 2, 2, 4 ),
 ( 0.000000000000000000, 0.001221101243989660551, 0.001831651865984463287, 0.002442202487979266024, 0.003663303731968859788, 0.004273854353963660140, 0.004884404975958460925, 0.005494955597953261710, 0.006105506219948060760, 0.007326607463937678810, 0.007937158085932474391, 0.008547708707927269972, 0.009768809951916843787, 0.01098991119590641587, 0.01221101243989598968, 0.01343211368388556523, 0.01465321492787513905, 0.01709541741585432484, 0.01831651865984389171, 0.01953761990383345165, 0.02197982239181260622, 0.02320092363580220085, 0.02442202487979178854, 0.02564312612378137970, 0.02686422736777097434, 0.02930642985575018095, 0.03174863234372939103, 0.03296973358771899260, 0.03358028420971379685, 0.03419083483170859417, 0.03541193607569825125, 0.03602248669769304856, 0.03663303731968785282, 0.03785413856367740582, 0.03907523980766696575 ),
 .UNSPECIFIED. ) ;
#34189=CARTESIAN_POINT ( 'NONE',  ( 175.5493994043409032, 73.18740965572595769, 68.72061911442422399 ) ) ;
#34190=CARTESIAN_POINT ( 'NONE',  ( 43.35276089251598819, 8.955376472641077612, -90.37929691252209352 ) ) ;
#34191=CARTESIAN_POINT ( 'NONE',  ( 102.7983318509014623, 26.68040613344513545, 62.90955133405510935 ) ) ;
#34193=CARTESIAN_POINT ( 'NONE',  ( -166.5742238910466142, 81.57147158222490191, -19.03685731792293012 ) ) ;
#34196=CARTESIAN_POINT ( 'NONE',  ( 88.98820631332498010, 21.30618275724810573, 3.231923812655122852 ) ) ;
#34197=CARTESIAN_POINT ( 'NONE',  ( -14.66033866466834645, 7.432913330382390882, 61.36269437948495664 ) ) ;
#34198=CARTESIAN_POINT ( 'NONE',  ( 12.91653430408660874, 7.431946598423014194, 57.41795537130889215 ) ) ;
#34201=FACE_BOUND ( 'NONE', #32816, .T. ) ;
#34206=CARTESIAN_POINT ( 'NONE',  ( -178.2328124332056234, 94.56955476227571467, 5.969047184286479180 ) ) ;
#34207=CARTESIAN_POINT ( 'NONE',  ( 206.2957331585309362, 110.2946564621822887, 56.17913581376664212 ) ) ;
#34208=CARTESIAN_POINT ( 'NONE',  ( 84.74140601443113496, 18.78541996275572856, -62.90364757930472450 ) ) ;
#34209=ORIENTED_EDGE ( 'NONE', *, *, #54445, .T. ) ;
#34210=CARTESIAN_POINT ( 'NONE',  ( 197.1975259970232344, 98.19639476549652102, -43.49939252954278146 ) ) ;
#34212=CARTESIAN_POINT ( 'NONE',  ( 108.7067726706416977, 29.28183711776652132, -89.72851832208228018 ) ) ;
#34214=VECTOR ( 'NONE', #49425, 1000.000000000000000 ) ;
#34217=LINE ( 'NONE', #28585, #6626 ) ;
#34220=CARTESIAN_POINT ( 'NONE',  ( 38.91493890549797641, 8.346224043800601677, -23.77526687496409963 ) ) ;
#34222=CARTESIAN_POINT ( 'NONE',  ( -155.7457403566965297, 71.01814553754120141, -73.35110919937355334 ) ) ;
#34223=CARTESIAN_POINT ( 'NONE',  ( 66.94365390260637128, 14.65531706601758977, 4.074685676838114112 ) ) ;
#34224=CARTESIAN_POINT ( 'NONE',  ( 152.6804161981488619, 55.27286404993338209, 4.288696971359757804 ) ) ;
#34225=VERTEX_POINT ( 'NONE', #10162 ) ;
#34228=ADVANCED_FACE ( 'NONE', ( #53522 ), #31624, .F. ) ;
#34232=CARTESIAN_POINT ( 'NONE',  ( -133.3220917939969183, 52.82057604964899866, -14.49950751745602950 ) ) ;
#34234=CARTESIAN_POINT ( 'NONE',  ( 115.7746371641014775, 31.52600568297705408, -11.48978713420478925 ) ) ;
#34235=CARTESIAN_POINT ( 'NONE',  ( 94.12361176368516169, 22.11573381981098052, 90.45082768725070821 ) ) ;
#34239=ADVANCED_FACE ( 'NONE', ( #9835 ), #15791, .F. ) ;
#34241=CARTESIAN_POINT ( 'NONE',  ( 42.70988075781782101, 8.862408058333491212, 3.820616178905913873 ) ) ;
#34242=CARTESIAN_POINT ( 'NONE',  ( -180.6289110087067797, 97.48982472183162429, 92.17219495999866297 ) ) ;
#34243=LINE ( 'NONE', #2233, #4196 ) ;
#34244=CARTESIAN_POINT ( 'NONE',  ( 104.3805245147141676, 26.26278144139197934, -21.28214446120828285 ) ) ;
#34245=CARTESIAN_POINT ( 'NONE',  ( 198.4017331595409246, 98.09114638179336509, 5.778807527766608665 ) ) ;
#34246=CARTESIAN_POINT ( 'NONE',  ( -55.05276343752909440, 15.72344139423349141, -35.21632399845986328 ) ) ;
#34248=CARTESIAN_POINT ( 'NONE',  ( -72.20490592113145567, 19.96451062593610004, -65.62012688376218250 ) ) ;
#34249=CARTESIAN_POINT ( 'NONE',  ( 8.000000000000007105, 249.8719672152120381, -95.00000000000133582 ) ) ;
#34253=ORIENTED_EDGE ( 'NONE', *, *, #63113, .F. ) ;
#34254=EDGE_CURVE ( 'NONE', #69216, #49946, #64052, .T. ) ;
#34256=CARTESIAN_POINT ( 'NONE',  ( 181.0840389613909736, 80.03940679743416808, -78.06960825634331513 ) ) ;
#34257=CARTESIAN_POINT ( 'NONE',  ( -166.2053056899075045, 81.18967388993343093, 35.40543396571913348 ) ) ;
#34258=CARTESIAN_POINT ( 'NONE',  ( -99.98930671699736195, 31.63190627461932891, -49.67157807265856917 ) ) ;
#34261=CARTESIAN_POINT ( 'NONE',  ( 140.4641697461913168, 46.75994457266055093, -13.09221936645533368 ) ) ;
#34268=LINE ( 'NONE', #13839, #17646 ) ;
#34269=CARTESIAN_POINT ( 'NONE',  ( 93.85477471612979627, 23.08982334209078147, -95.00000000000133582 ) ) ;
#34272=CARTESIAN_POINT ( 'NONE',  ( 199.9103251464699440, 101.6434290204575603, 69.33018220824747857 ) ) ;
#34276=CARTESIAN_POINT ( 'NONE',  ( -60.98168946575806615, 17.40090852531920618, -64.94124262262964464 ) ) ;
#34277=CARTESIAN_POINT ( 'NONE',  ( 197.2199163281727863, 98.22431253015348318, -71.33388331724441400 ) ) ;
#34278=CARTESIAN_POINT ( 'NONE',  ( -179.5178913137216909, 94.54206947403388028, -38.25780915961179574 ) ) ;
#34279=CARTESIAN_POINT ( 'NONE',  ( 102.8066580714140485, 25.59117171226998266, 9.258329190121406427 ) ) ;
#34280=CARTESIAN_POINT ( 'NONE',  ( -170.2801941679961146, 84.02053682015869640, 4.523125458188938630 ) ) ;
#34281=CARTESIAN_POINT ( 'NONE',  ( -173.1211646369891355, 88.63826465341151106, -22.86740657428632773 ) ) ;
#34282=FACE_BOUND ( 'NONE', #16921, .T. ) ;
#34283=B_SPLINE_CURVE_WITH_KNOTS ( 'NONE', 3,
 ( #49531, #44263, #66104, #62185, #35813, #15043, #56565, #36498, #14690, #24913, #4148, #8742, #51303, #67477, #46699, #35461, #20312, #57950 ),
 .UNSPECIFIED., .F., .F.,
 ( 4, 2, 2, 2, 2, 2, 2, 2, 4 ),
 ( 0.01368524652304596405, 0.01545087154706958552, 0.01721649657109320872, 0.02074774661914039961, 0.02251337164316399506, 0.02427899666718758703, 0.02604462169121118595, 0.02692743420322298367, 0.02781024671523478140 ),
 .UNSPECIFIED. ) ;
#34284=CARTESIAN_POINT ( 'NONE',  ( -189.3456113063706709, 107.2364438114461791, 93.44106408251658991 ) ) ;
#34287=CARTESIAN_POINT ( 'NONE',  ( -0.5780275525703854056, 6.527356703336898214, 62.51425872000311301 ) ) ;
#34293=CARTESIAN_POINT ( 'NONE',  ( 59.72647370436682479, 12.96353798836696214, -63.32053846355550775 ) ) ;
#34297=DIRECTION ( 'NONE',  ( -0.000000000000000000, 1.000000000000000000, -0.000000000000000000 ) ) ;
#34302=CARTESIAN_POINT ( 'NONE',  ( 173.6718135456487175, 71.42581476597410983, -42.54376570200113150 ) ) ;
#34303=CARTESIAN_POINT ( 'NONE',  ( 150.4542242713869484, 53.63744268572195750, 39.57349238810517988 ) ) ;
#34306=FACE_OUTER_BOUND ( 'NONE', #44891, .T. ) ;
#34308=CARTESIAN_POINT ( 'NONE',  ( -0.7215816834507559063, 6.532459459468096696, 8.353057134836445741 ) ) ;
#34309=CARTESIAN_POINT ( 'NONE',  ( -55.05276343752910151, -170.0000000000000000, -77.06087458892358200 ) ) ;
#34310=CARTESIAN_POINT ( 'NONE',  ( -28.13128612339709278, 10.08889185338652972, -9.223690606770793110 ) ) ;
#34311=CARTESIAN_POINT ( 'NONE',  ( -51.34542473642584781, 14.75635007918830155, -22.39598248981539541 ) ) ;
#34314=EDGE_CURVE ( 'NONE', #57172, #58537, #40511, .T. ) ;
#34317=CARTESIAN_POINT ( 'NONE',  ( -75.43495400358860081, 22.18831810339350952, 4.301192105811935562 ) ) ;
#34319=CARTESIAN_POINT ( 'NONE',  ( -166.3205068063721512, 81.30869308872871670, -72.23115024874353196 ) ) ;
#34321=CARTESIAN_POINT ( 'NONE',  ( -123.1591800884025218, 44.71875343686618010, 84.80057340962032697 ) ) ;
#34322=EDGE_LOOP ( 'NONE', ( #51514, #39923, #30551, #6113 ) ) ;
#34323=CARTESIAN_POINT ( 'NONE',  ( 82.34195123877070444, 18.00239921638038965, -37.16307426115260171 ) ) ;
#34327=ORIENTED_EDGE ( 'NONE', *, *, #2055, .T. ) ;
#34329=CARTESIAN_POINT ( 'NONE',  ( 80.71682498289315788, 18.54204664833076066, 41.85293259918689301 ) ) ;
#34343=CARTESIAN_POINT ( 'NONE',  ( 102.8066580714140343, 25.59117171227001464, 62.94743037104881722 ) ) ;
#34344=CARTESIAN_POINT ( 'NONE',  ( 162.7921669283190909, 61.91024532638674316, 58.46359787650868611 ) ) ;
#34346=EDGE_CURVE ( 'NONE', #39218, #30581, #20446, .T. ) ;
#34351=CARTESIAN_POINT ( 'NONE',  ( -109.5142642360664667, 36.61018064014777451, 62.81589927390022865 ) ) ;
#34352=CYLINDRICAL_SURFACE ( 'NONE', #39598, 7.500000000000020428 ) ;
#34353=DIRECTION ( 'NONE',  ( -0.8160245890732938934, -0.5780171883497599028, 0.000000000000000000 ) ) ;
#34355=ORIENTED_EDGE ( 'NONE', *, *, #46120, .T. ) ;
#34356=VERTEX_POINT ( 'NONE', #45653 ) ;
#34358=CARTESIAN_POINT ( 'NONE',  ( -74.60184650407219920, 20.81479667884462614, 85.29625918890103264 ) ) ;
#34360=CARTESIAN_POINT ( 'NONE',  ( 130.7457207912710828, 40.74300766298683385, 30.17037958794855257 ) ) ;
#34363=CARTESIAN_POINT ( 'NONE',  ( -95.63694837622350065, 30.64472169584720618, -12.17974421549104314 ) ) ;
#34364=CARTESIAN_POINT ( 'NONE',  ( 57.39233401791016576, 12.46575990788836918, 42.29982551114518685 ) ) ;
#34370=CARTESIAN_POINT ( 'NONE',  ( -15.27594996066616773, 8.502079791899641137, 9.781629159753414626 ) ) ;
#34372=CARTESIAN_POINT ( 'NONE',  ( -102.7456062648101636, 33.01749955571779083, -76.85912785543966663 ) ) ;
#34373=CARTESIAN_POINT ( 'NONE',  ( 126.4757069339777473, 38.29528077539270470, -18.03564317929428285 ) ) ;
#34379=CARTESIAN_POINT ( 'NONE',  ( -189.5325095384513929, 107.4952257375067290, -13.13692968654411786 ) ) ;
#34382=CARTESIAN_POINT ( 'NONE',  ( -167.9337388826115784, 81.53346785675708475, 86.55874306617425873 ) ) ;
#34385=CARTESIAN_POINT ( 'NONE',  ( 23.09119322872580682, 7.852465917941087170, -95.00000000000133582 ) ) ;
#34388=CARTESIAN_POINT ( 'NONE',  ( -142.0081215801269536, 58.07066293384865929, -15.76809686950948830 ) ) ;
#34390=CARTESIAN_POINT ( 'NONE',  ( -2.873329055852807290, 7.626065826870673803, -75.41701928022413881 ) ) ;
#34391=EDGE_CURVE ( 'NONE', #29060, #29497, #51282, .T. ) ;
#34396=CARTESIAN_POINT ( 'NONE',  ( 197.3707490726350215, 96.80690576410104597, -42.19351181672752205 ) ) ;
#34398=CARTESIAN_POINT ( 'NONE',  ( 19.75784582661440680, 6.660183274347837745, -36.65081142605392728 ) ) ;
#34399=CARTESIAN_POINT ( 'NONE',  ( 110.7167338301703694, 30.21148223254618159, 17.76666361527367499 ) ) ;
#34402=CARTESIAN_POINT ( 'NONE',  ( 57.39083379741711610, 11.43779987330584724, 32.32724278055570721 ) ) ;
#34404=EDGE_LOOP ( 'NONE', ( #27853, #4715 ) ) ;
#34406=ORIENTED_EDGE ( 'NONE', *, *, #62455, .F. ) ;
#34407=CARTESIAN_POINT ( 'NONE',  ( 173.8623159076320235, 72.97967239795021044, 34.76400434874135215 ) ) ;
#34408=CARTESIAN_POINT ( 'NONE',  ( 18.21423326326598158, 6.590134686181414736, -62.74990453328492634 ) ) ;
#34409=ADVANCED_FACE ( 'NONE', ( #67803 ), #67461, .F. ) ;
#34410=CARTESIAN_POINT ( 'NONE',  ( -8.800520192024519517, 7.964629484975260354, -77.21523971768127126 ) ) ;
#34411=ORIENTED_EDGE ( 'NONE', *, *, #48102, .F. ) ;
#34412=CARTESIAN_POINT ( 'NONE',  ( -94.82531008173683063, 30.26290669250042598, 90.82179001772281879 ) ) ;
#34413=DIRECTION ( 'NONE',  ( 0.000000000000000000, -0.000000000000000000, -1.000000000000000000 ) ) ;
#34414=CARTESIAN_POINT ( 'NONE',  ( -71.15374617000811952, 20.66492714610676273, -42.60528795093121346 ) ) ;
#34417=CARTESIAN_POINT ( 'NONE',  ( 206.3053863259450509, 110.3084416756849464, -63.29990767306989596 ) ) ;
#34419=DIRECTION ( 'NONE',  ( -0.000000000000000000, 1.000000000000000000, -0.000000000000000000 ) ) ;
#34421=CARTESIAN_POINT ( 'NONE',  ( 128.0540543950622805, 39.18660671946771146, 68.63333648139733612 ) ) ;
#34435=CARTESIAN_POINT ( 'NONE',  ( -142.4991775570125583, 58.45550857435407011, 40.94546928456825441 ) ) ;
#34437=CARTESIAN_POINT ( 'NONE',  ( -78.66644367742111399, 23.39876645725285798, -8.270900041254197532 ) ) ;
#34440=CARTESIAN_POINT ( 'NONE',  ( 83.60262962804348774, 18.41036205028015615, 57.19024780777382944 ) ) ;
#34441=B_SPLINE_CURVE_WITH_KNOTS ( 'NONE', 3,
 ( #10969, #32435, #41951, #63414, #47905, #21188, #63062, #27143, #42635, #37022, #20152, #36683, #41603, #58460, #36332, #20837, #33825, #48928, #6393, #60895, #43660, #414, #1823, #7448, #28904, #65488, #39115, #44011, #23282, #21867, #27845, #44728, #39444, #38049, #65139, #49993, #17647, #27490, #59494, #43312, #770, #28545, #64788, #33132, #49281, #54566 ),
 .UNSPECIFIED., .F., .F.,
 ( 4, 2, 2, 2, 2, 2, 2, 2, 2, 2, 2, 2, 2, 2, 2, 2, 2, 2, 2, 2, 2, 2, 4 ),
 ( 7.152448122690996019E-18, 0.003192770216278319195, 0.003990962770347897259, 0.004789155324417473589, 0.006385540432556618441, 0.007183732986626203444, 0.007981925540695787580, 0.009578310648834957586, 0.01037650320290455300, 0.01117469575697414667, 0.01197288831104374382, 0.01277108086511333750, 0.01436746597325252658, 0.01596385108139171741, 0.01676204363546130241, 0.01756023618953088741, 0.01835842874360046895, 0.01915662129767005395, 0.02075300640580922049, 0.02234939151394838702, 0.02394577662208755703, 0.02474396917615713856, 0.02554216173022672010 ),
 .UNSPECIFIED. ) ;
#34443=CARTESIAN_POINT ( 'NONE',  ( 31.96227686234411181, 7.558148489540045922, 36.43275077287186292 ) ) ;
#34450=CARTESIAN_POINT ( 'NONE',  ( -48.99162761293256096, 13.13973062091724664, 6.548506681903217164 ) ) ;
#34453=CARTESIAN_POINT ( 'NONE',  ( -102.2801239173131052, 32.78103895658057354, -88.70367844590326456 ) ) ;
#34459=VERTEX_POINT ( 'NONE', #4468 ) ;
#34461=CARTESIAN_POINT ( 'NONE',  ( 150.7770046255792238, 53.87214803240240713, -67.07469974738161511 ) ) ;
#34462=CARTESIAN_POINT ( 'NONE',  ( -38.87848244732137459, 10.93141945332450327, 36.73303816849150394 ) ) ;
#34463=CARTESIAN_POINT ( 'NONE',  ( 140.1999945597798671, 45.38880890490928977, -47.53303235619388545 ) ) ;
#34466=CARTESIAN_POINT ( 'NONE',  ( -121.5677746760273834, 43.71038933438993013, 44.26482168794601790 ) ) ;
#34468=CARTESIAN_POINT ( 'NONE',  ( 31.90247004928964358, 8.563336936370816943, -16.77865705936252994 ) ) ;
#34469=CARTESIAN_POINT ( 'NONE',  ( -55.05276343752909440, 15.72344139423348430, 30.31732777293113301 ) ) ;
#34470=CARTESIAN_POINT ( 'NONE',  ( -7.330587818645180498, 7.867004275019547244, 18.27103044898354156 ) ) ;
#34471=CARTESIAN_POINT ( 'NONE',  ( 135.4635403382140737, 43.58489979881251486, 83.36700200578437148 ) ) ;
#34473=CARTESIAN_POINT ( 'NONE',  ( 200.2036606579482338, 102.0234725140079632, -91.49788894171744857 ) ) ;
#34477=VERTEX_POINT ( 'NONE', #31543 ) ;
#34478=CARTESIAN_POINT ( 'NONE',  ( 163.1495034066983862, 62.20479872133083887, -11.85475170272490608 ) ) ;
#34481=CARTESIAN_POINT ( 'NONE',  ( 70.45466089417031696, 14.52203022703029944, 65.14393066459052761 ) ) ;
#34482=CARTESIAN_POINT ( 'NONE',  ( -129.8719378883314164, 50.39084145585431429, -89.73039419715394160 ) ) ;
#34488=CARTESIAN_POINT ( 'NONE',  ( 164.9700808964341547, 65.04346068891115351, -16.49089399958545954 ) ) ;
#34490=ORIENTED_EDGE ( 'NONE', *, *, #63779, .T. ) ;
#34492=CARTESIAN_POINT ( 'NONE',  ( 67.55199883153196083, 14.80832170058782360, 58.16522213638270955 ) ) ;
#34494=EDGE_CURVE ( 'NONE', #54444, #8166, #60695, .T. ) ;
#34496=EDGE_LOOP ( 'NONE', ( #13657, #16247 ) ) ;
#34497=CARTESIAN_POINT ( 'NONE',  ( -144.9287131874381771, 60.39056348581542721, -63.19771770627043139 ) ) ;
#34501=VERTEX_POINT ( 'NONE', #36479 ) ;
#34503=CARTESIAN_POINT ( 'NONE',  ( 67.88615656271203136, 14.89310733039355306, 85.25998462581451065 ) ) ;
#34505=CARTESIAN_POINT ( 'NONE',  ( 80.15818551272215586, 18.36718314243335470, -12.65347328967094498 ) ) ;
#34506=CARTESIAN_POINT ( 'NONE',  ( -129.3963145237380843, 48.84337839101544176, -8.933155718294752745 ) ) ;
#34507=CARTESIAN_POINT ( 'NONE',  ( 151.6351261592328967, 53.25263237790400694, 68.47247492333102059 ) ) ;
#34508=CARTESIAN_POINT ( 'NONE',  ( 126.5710838895481345, 37.19597237024179037, -72.16778413864886943 ) ) ;
#34509=EDGE_LOOP ( 'NONE', ( #69003, #17140, #45484, #15824 ) ) ;
#34510=CARTESIAN_POINT ( 'NONE',  ( -96.77705718164443738, 31.18700926299571208, 69.98325796537412202 ) ) ;
#34511=CARTESIAN_POINT ( 'NONE',  ( -14.84452950307166219, 8.460866451887699924, 61.80641794076242945 ) ) ;
#34513=CARTESIAN_POINT ( 'NONE',  ( -156.8728827992624417, 72.05711009495558983, -43.75528730729580218 ) ) ;
#34516=FACE_OUTER_BOUND ( 'NONE', #41727, .T. ) ;
#34517=CARTESIAN_POINT ( 'NONE',  ( -10.71904918402348805, 7.096480526292664237, -89.67472281983359039 ) ) ;
#34518=ADVANCED_FACE ( 'NONE', ( #9750 ), #48050, .T. ) ;
#34521=CARTESIAN_POINT ( 'NONE',  ( -10.69547592951791160, 8.103864096836391084, 30.67361113490947488 ) ) ;
#34522=CARTESIAN_POINT ( 'NONE',  ( -62.30100056228381078, 16.74548393487071607, 12.96427395586250952 ) ) ;
#34526=CARTESIAN_POINT ( 'NONE',  ( -94.83091526606385457, 30.26550147229321652, -43.53056186647030756 ) ) ;
#34531=CARTESIAN_POINT ( 'NONE',  ( 46.70715146412977248, 9.472433765546997009, 62.54244382710503913 ) ) ;
#34533=CARTESIAN_POINT ( 'NONE',  ( -14.91909499790562954, 7.457200389278945352, 93.82548247898083105 ) ) ;
#34536=CARTESIAN_POINT ( 'NONE',  ( 133.8566784816069344, -170.0000000000000000, 37.01034083899534721 ) ) ;
#34544=CARTESIAN_POINT ( 'NONE',  ( 106.6322547488295243, 28.34756922280614688, 57.36455916318408299 ) ) ;
#34546=CARTESIAN_POINT ( 'NONE',  ( 110.2429982417149574, -170.0000000000000000, -89.61153874658103291 ) ) ;
#34547=CARTESIAN_POINT ( 'NONE',  ( 59.72647370436681769, 12.96353798836696747, -9.631437282628132479 ) ) ;
#34548=VERTEX_POINT ( 'NONE', #63898 ) ;
#34549=CARTESIAN_POINT ( 'NONE',  ( 86.62931800182293784, 20.48449268398422518, 2.867536982015617575 ) ) ;
#34550=EDGE_CURVE ( 'NONE', #14016, #40816, #25595, .T. ) ;
#34551=CARTESIAN_POINT ( 'NONE',  ( -7.825402957745083654, 6.891034867348165172, 56.96013162991089018 ) ) ;
#34553=B_SPLINE_CURVE_WITH_KNOTS ( 'NONE', 3,
 ( #11755, #44103, #17380, #56072, #13511, #18436, #24066, #56410, #45862, #45158, #1557, #19121, #7889, #17750, #1927, #66638, #7187, #55366, #28645, #61687, #50449, #23386, #50786, #34277, #23019, #29335, #39891, #40241, #66994, #51144, #6833, #50098, #2607, #8232, #61348, #62030, #60649, #2269, #40576, #45510, #67333, #2960, #44471, #23716, #13167, #66305, #65952, #18092, #34635, #44824 ),
 .UNSPECIFIED., .F., .F.,
 ( 4, 2, 2, 2, 2, 2, 2, 2, 2, 2, 2, 2, 2, 2, 2, 2, 2, 2, 2, 2, 2, 2, 2, 2, 4 ),
 ( 0.03296461860586797493, 0.03492857779726588757, 0.03689253698866380021, 0.03885649618006171979, 0.04082045537145963243, 0.04278441456285754507, 0.04376639415855652221, 0.04474837375425549935, 0.04573035334995447648, 0.04671233294565345362, 0.04720332274350291790, 0.04769431254135237525, 0.04867629213705129687, 0.04965827173275022544, 0.05064025132844915400, 0.05162223092414808256, 0.05260421051984700419, 0.05358619011554593276, 0.05456816971124485438, 0.05555014930694378295, 0.05653212890264271151, 0.05849608809404054782, 0.06046004728543838413, 0.06242400647683622739, 0.06438796566823407064 ),
 .UNSPECIFIED. ) ;
#34555=CARTESIAN_POINT ( 'NONE',  ( 205.5105258529713126, 107.4632495673648123, -9.514488831477544650 ) ) ;
#34556=FACE_BOUND ( 'NONE', #11519, .T. ) ;
#34563=CARTESIAN_POINT ( 'NONE',  ( 33.31166872005965729, 8.707041209322234465, -74.34829994818775845 ) ) ;
#34565=CARTESIAN_POINT ( 'NONE',  ( 210.6584452238134588, 116.7138338345753965, 58.97358617813433312 ) ) ;
#34566=CARTESIAN_POINT ( 'NONE',  ( 81.57482918025354479, 17.75786713398421313, -64.61972240065618678 ) ) ;
#34570=CARTESIAN_POINT ( 'NONE',  ( 201.5987353083855567, 103.8544727311227263, -50.66920982680341012 ) ) ;
#34575=CARTESIAN_POINT ( 'NONE',  ( -81.01337222286376516, 23.22902179892324881, -76.59940889876602910 ) ) ;
#34576=DIRECTION ( 'NONE',  ( -0.000000000000000000, 1.000000000000000000, -0.000000000000000000 ) ) ;
#34577=CARTESIAN_POINT ( 'NONE',  ( 92.21252738308862718, 22.47457138983957137, -75.19816570723047278 ) ) ;
#34581=EDGE_CURVE ( 'NONE', #56862, #22146, #262, .T. ) ;
#34583=CARTESIAN_POINT ( 'NONE',  ( 43.14565945994675644, 9.942782559600560788, 57.75492960358775463 ) ) ;
#34586=CARTESIAN_POINT ( 'NONE',  ( 21.42484406671928454, 6.746536496442160136, 5.716369911633448986 ) ) ;
#34591=CARTESIAN_POINT ( 'NONE',  ( -47.65155309726505806, 13.85482731128120193, 9.734102492370531934 ) ) ;
#34592=CARTESIAN_POINT ( 'NONE',  ( -132.0738857626834317, 51.93126104279146915, -19.82589294571803507 ) ) ;
#34593=CARTESIAN_POINT ( 'NONE',  ( 111.1767565371974484, 29.31586421952250632, -24.03438127329443219 ) ) ;
#34594=CARTESIAN_POINT ( 'NONE',  ( 88.90509360958570539, 20.20992759522961180, 83.74746512799291054 ) ) ;
#34595=CARTESIAN_POINT ( 'NONE',  ( -166.4833234777584323, 81.47689702327105010, -92.37364644444049588 ) ) ;
#34598=VERTEX_POINT ( 'NONE', #54004 ) ;
#34599=CARTESIAN_POINT ( 'NONE',  ( 46.90222083990963853, 9.503928413859236812, 10.80947253210855052 ) ) ;
#34600=DIRECTION ( 'NONE',  ( 0.000000000000000000, 0.000000000000000000, 1.000000000000000000 ) ) ;
#34602=CARTESIAN_POINT ( 'NONE',  ( 103.0026233023293116, 25.67408295205788349, -18.60120070009467241 ) ) ;
#34603=CARTESIAN_POINT ( 'NONE',  ( 199.3743599161302882, 99.31857334527873604, 15.17104788207974231 ) ) ;
#34604=CARTESIAN_POINT ( 'NONE',  ( 199.9883293275698293, 101.7441989053914426, 84.55131181239630678 ) ) ;
#34606=DIRECTION ( 'NONE',  ( 0.000000000000000000, 0.000000000000000000, 1.000000000000000000 ) ) ;
#34607=CARTESIAN_POINT ( 'NONE',  ( -14.55425570676091773, 7.423011834016146615, 40.93716450737882440 ) ) ;
#34609=CARTESIAN_POINT ( 'NONE',  ( 8.478575283864733692, 7.382882227715640511, -14.47795047564284410 ) ) ;
#34611=B_SPLINE_CURVE_WITH_KNOTS ( 'NONE', 3,
 ( #35846, #9111, #52363, #9804, #4179, #63267, #31264, #25980, #18970, #51336, #38247, #48780, #68867, #59008, #58317, #21046, #16101, #63950, #64293, #43517, #16455, #5883, #10136, #59690, #58657, #10476, #22076, #42149, #42494, #10826, #26325, #37909, #42822, #64996, #6238, #47412, #11502, #31593, #27342, #59355, #37556, #16789, #20690, #21721, #32977, #53375, #53033, #47762, #4859, #11166 ),
 .UNSPECIFIED., .F., .F.,
 ( 4, 2, 2, 2, 2, 2, 2, 2, 2, 2, 2, 2, 2, 2, 2, 2, 2, 2, 2, 2, 2, 2, 2, 2, 4 ),
 ( 0.03296461860586794718, 0.03492857779726583900, 0.03689253698866373082, 0.03885649618006162265, 0.04082045537145951447, 0.04278441456285740629, 0.04376639415855634874, 0.04474837375425529118, 0.04573035334995423362, 0.04671233294565317606, 0.04720332274350264035, 0.04769431254135211157, 0.04867629213705104707, 0.04965827173274998951, 0.05064025132844893196, 0.05162223092414787440, 0.05260421051984681684, 0.05358619011554575928, 0.05456816971124470173, 0.05555014930694364417, 0.05653212890264258661, 0.05849608809404044374, 0.06046004728543829393, 0.06242400647683614412, 0.06438796566823400125 ),
 .UNSPECIFIED. ) ;
#34613=CARTESIAN_POINT ( 'NONE',  ( -148.0058283997321098, 64.22864592525512251, 4.024936692211257494 ) ) ;
#34615=CARTESIAN_POINT ( 'NONE',  ( -165.7690020878297901, 80.74028011998679233, 36.81020553927029226 ) ) ;
#34617=CARTESIAN_POINT ( 'NONE',  ( -31.43908319763710679, 10.61114334766713796, -89.00629854612920155 ) ) ;
#34618=CARTESIAN_POINT ( 'NONE',  ( 14.81290967676422277, 7.477658233646010899, -50.47154902647776709 ) ) ;
#34619=DIRECTION ( 'NONE',  ( -0.000000000000000000, 1.000000000000000000, -0.000000000000000000 ) ) ;
#34623=CARTESIAN_POINT ( 'NONE',  ( 188.5871124577482192, 88.04033245483464043, 90.77543754304032575 ) ) ;
#34624=CARTESIAN_POINT ( 'NONE',  ( -7.825402957745083654, 6.891034867348166060, 3.271030448983516692 ) ) ;
#34626=CARTESIAN_POINT ( 'NONE',  ( 58.09607305250595743, 11.58497620657515270, -22.05889382308176039 ) ) ;
#34631=VERTEX_POINT ( 'NONE', #45128 ) ;
#34633=CARTESIAN_POINT ( 'NONE',  ( 46.51377856795992471, 10.46037936279324576, -67.53287648513382635 ) ) ;
#34634=CARTESIAN_POINT ( 'NONE',  ( -60.64199216239840240, 17.30050036439948258, -74.56797183276353280 ) ) ;
#34635=CARTESIAN_POINT ( 'NONE',  ( 204.3091227790963558, 107.5190503136783065, -63.17048162308529413 ) ) ;
#34636=CARTESIAN_POINT ( 'NONE',  ( -177.1539090641757923, 91.73101548694627638, -35.87291332312106817 ) ) ;
#34638=CARTESIAN_POINT ( 'NONE',  ( -165.7689197919845014, 79.30072199592277116, 12.98792212612636732 ) ) ;
#34639=CARTESIAN_POINT ( 'NONE',  ( -61.68940124183720286, -170.0000000000000000, 94.99999999999866418 ) ) ;
#34640=FACE_BOUND ( 'NONE', #26110, .T. ) ;
#34641=CARTESIAN_POINT ( 'NONE',  ( 133.8566784816069344, 42.60093787723652525, 56.35489142945903751 ) ) ;
#34642=ADVANCED_FACE ( 'NONE', ( #5833 ), #43464, .F. ) ;
#34645=CARTESIAN_POINT ( 'NONE',  ( -5.871577929436014642, 6.771181646175757685, 71.71801545187251747 ) ) ;
#34649=CARTESIAN_POINT ( 'NONE',  ( 157.4703587214989113, 58.92748579479258808, 56.25401806271706562 ) ) ;
#34650=DIRECTION ( 'NONE',  ( -0.8160245890732938934, -0.5780171883497599028, 0.000000000000000000 ) ) ;
#34655=ORIENTED_EDGE ( 'NONE', *, *, #44042, .F. ) ;
#34658=CARTESIAN_POINT ( 'NONE',  ( 151.7783534118502189, 54.60545177578661935, 41.79957158508126014 ) ) ;
#34660=EDGE_CURVE ( 'NONE', #68705, #67501, #24588, .T. ) ;
#34662=FACE_OUTER_BOUND ( 'NONE', #9877, .T. ) ;
#34663=CARTESIAN_POINT ( 'NONE',  ( -180.4654253355436992, 95.69358270527506249, 9.926583934681923793 ) ) ;
#34664=CARTESIAN_POINT ( 'NONE',  ( -1.314022807222076983, 6.554273999800675377, 14.52494611356557641 ) ) ;
#34666=CARTESIAN_POINT ( 'NONE',  ( 150.1480464045414180, 52.17471502308665521, 92.38535431822143096 ) ) ;
#34670=CARTESIAN_POINT ( 'NONE',  ( 112.5721302457195208, 29.97407549554797868, -36.27765895070014324 ) ) ;
#34671=CARTESIAN_POINT ( 'NONE',  ( -71.23176719684943237, 20.69188312694498677, 12.09344324661407377 ) ) ;
#34672=CARTESIAN_POINT ( 'NONE',  ( 43.35980717318838629, 8.957244490220878319, -36.74440757935403923 ) ) ;
#34681=CARTESIAN_POINT ( 'NONE',  ( 84.97658021689284169, 19.92447159015899416, 29.89253886502025637 ) ) ;
#34684=CARTESIAN_POINT ( 'NONE',  ( 140.4897729434290454, 45.57634363643752806, -13.13958130089202392 ) ) ;
#34686=CARTESIAN_POINT ( 'NONE',  ( -180.6158171975815492, 97.47361786002628037, -15.69178128716336040 ) ) ;
#34687=CARTESIAN_POINT ( 'NONE',  ( -154.6171773099879658, 68.63761944777705537, -36.81755893726905526 ) ) ;
#34691=CARTESIAN_POINT ( 'NONE',  ( 164.9697211531229755, 63.72502658717164792, 63.45721136982654542 ) ) ;
#34695=CARTESIAN_POINT ( 'NONE',  ( 187.8959968237854525, 85.77553094678185630, -46.87483139314726088 ) ) ;
#34696=CARTESIAN_POINT ( 'NONE',  ( -104.5827168854524558, 33.96561401163047833, 57.71033412352771563 ) ) ;
#34701=VERTEX_POINT ( 'NONE', #56732 ) ;
#34703=FACE_OUTER_BOUND ( 'NONE', #67148, .T. ) ;
#34705=CARTESIAN_POINT ( 'NONE',  ( 132.2818448028687897, 41.65267246304672000, 29.67398922120065663 ) ) ;
#34707=CARTESIAN_POINT ( 'NONE',  ( -55.05276343752909440, 15.72344139423348430, 30.31732777293113301 ) ) ;
#34708=CARTESIAN_POINT ( 'NONE',  ( -99.99439884168255332, 32.75762661251356889, -8.511024296776820819 ) ) ;
#34709=CARTESIAN_POINT ( 'NONE',  ( 59.29474530993685732, 12.86968658439547930, 43.82944600131264679 ) ) ;
#34710=CARTESIAN_POINT ( 'NONE',  ( 37.45083697588171390, 8.163195152810535760, 83.83898265753474277 ) ) ;
#34714=CARTESIAN_POINT ( 'NONE',  ( -14.33060720034883673, 8.412649192293191192, 7.006307883328436681 ) ) ;
#34715=CARTESIAN_POINT ( 'NONE',  ( -144.9287131874381771, 60.39056348581540590, 17.33593406512061819 ) ) ;
#34717=CARTESIAN_POINT ( 'NONE',  ( 197.3685896092616474, 96.80423329231983587, 61.92891938233814386 ) ) ;
#34719=CARTESIAN_POINT ( 'NONE',  ( 127.4992165631961569, 38.87141012667720474, -20.68911966244177947 ) ) ;
#34722=EDGE_CURVE ( 'NONE', #8386, #12944, #3269, .T. ) ;
#34723=CARTESIAN_POINT ( 'NONE',  ( 126.3580464630938707, 38.22944795020833908, -43.82392713467700673 ) ) ;
#34724=CARTESIAN_POINT ( 'NONE',  ( -38.80621516088653067, 11.94263260276895622, -41.34864224206805261 ) ) ;
#34727=CARTESIAN_POINT ( 'NONE',  ( -188.6739852773920347, 108.2139733222100517, -43.81670758250005093 ) ) ;
#34728=ORIENTED_EDGE ( 'NONE', *, *, #17928, .T. ) ;
#34730=B_SPLINE_CURVE_WITH_KNOTS ( 'NONE', 3,
 ( #10420, #37499, #25594, #4467, #58953, #51960, #47357, #20632, #46679, #26610, #19964, #3770, #25243, #15015, #63897, #62868, #63556, #31542, #14668, #52979, #4802, #15365, #41415, #68813, #36133, #30861, #47029, #20291, #48049, #5152, #36828, #52305, #26266, #58604, #36478, #69504, #52643, #4125, #15708, #20990, #68486, #21324, #41755, #57930, #9749, #31212, #25926, #58266 ),
 .UNSPECIFIED., .F., .F.,
 ( 4, 2, 2, 2, 2, 2, 2, 2, 2, 2, 2, 2, 2, 2, 2, 2, 2, 2, 2, 2, 2, 2, 2, 4 ),
 ( 0.02554216173022674438, 0.02715505844859233270, 0.02796150680777515288, 0.02876795516695797306, 0.03038085188532354056, 0.03199374860368910806, 0.03360664532205467903, 0.03441309368123745410, 0.03521954204042023612, 0.03602599039960301119, 0.03683243875878579321, 0.03844533547715135030, 0.03925178383633415313, 0.04005823219551694903, 0.04086468055469975186, 0.04167112891388255469, 0.04247757727306535058, 0.04328402563224814648, 0.04489692235061378683, 0.04650981906897942025, 0.04731626742816222309, 0.04812271578734503286, 0.04973561250571071485, 0.05134850922407639684 ),
 .UNSPECIFIED. ) ;
#34732=CARTESIAN_POINT ( 'NONE',  ( 204.6977192012829505, 108.0580384837234931, 2.363170148305746565 ) ) ;
#34733=CARTESIAN_POINT ( 'NONE',  ( 159.9309212402495461, 60.87908227903663771, 83.50715383507403544 ) ) ;
#34734=EDGE_CURVE ( 'NONE', #8399, #33379, #22074, .T. ) ;
#34735=VERTEX_POINT ( 'NONE', #43641 ) ;
#34736=CARTESIAN_POINT ( 'NONE',  ( -56.96436614829622869, 16.24647150911285820, 3.716444753663429523 ) ) ;
#34741=LINE ( 'NONE', #7992, #53907 ) ;
#34742=CARTESIAN_POINT ( 'NONE',  ( 79.14129363775930415, 17.00055658855363205, 9.874494824056680997 ) ) ;
#34744=ORIENTED_EDGE ( 'NONE', *, *, #55497, .T. ) ;
#34745=CARTESIAN_POINT ( 'NONE',  ( 58.09607305250595033, 11.58497620657515803, 31.63020735784560600 ) ) ;
#34748=CARTESIAN_POINT ( 'NONE',  ( -171.4943428135323131, 86.82484920477511992, 18.84716997149836359 ) ) ;
#34749=DIRECTION ( 'NONE',  ( 0.000000000000000000, 0.000000000000000000, 1.000000000000000000 ) ) ;
#34750=CARTESIAN_POINT ( 'NONE',  ( -14.56631729561072319, 8.434645566888200108, -66.43805081226972220 ) ) ;
#34751=ORIENTED_EDGE ( 'NONE', *, *, #43644, .T. ) ;
#34752=CARTESIAN_POINT ( 'NONE',  ( -95.25262505162312721, 30.46326104480063890, 94.40935392145755145 ) ) ;
#34753=CARTESIAN_POINT ( 'NONE',  ( -24.61094659556677655, 9.585225265507407499, 40.82880548562345524 ) ) ;
#34757=CARTESIAN_POINT ( 'NONE',  ( 211.7357196141372242, 118.3691710715567211, -68.06136091401778287 ) ) ;
#34758=CYLINDRICAL_SURFACE ( 'NONE', #15125, 7.500000000000013323 ) ;
#34760=LINE ( 'NONE', #55867, #6666 ) ;
#34761=DIRECTION ( 'NONE',  ( -0.000000000000000000, 1.000000000000000000, -0.000000000000000000 ) ) ;
#34765=ORIENTED_EDGE ( 'NONE', *, *, #44143, .F. ) ;
#34766=LINE ( 'NONE', #6978, #62076 ) ;
#34769=CARTESIAN_POINT ( 'NONE',  ( -52.34571669801462690, 13.97238103161367562, -89.40772904822969736 ) ) ;
#34774=CARTESIAN_POINT ( 'NONE',  ( -71.97171223898807568, 20.94894057408424359, -12.35306980544747546 ) ) ;
#34776=CARTESIAN_POINT ( 'NONE',  ( -108.6622665321723105, 37.28993738537006664, 34.07158365272115219 ) ) ;
#34777=EDGE_LOOP ( 'NONE', ( #69038, #52836, #23194, #33938 ) ) ;
#34779=CARTESIAN_POINT ( 'NONE',  ( 36.31593203568480277, 8.028139509847019184, 30.57375986728627026 ) ) ;
#34782=CARTESIAN_POINT ( 'NONE',  ( 183.1910712700538397, 80.76073941711160842, 44.01936912216330455 ) ) ;
#34785=CARTESIAN_POINT ( 'NONE',  ( -123.6618353044034535, 46.23845779494349273, 57.78952661695447546 ) ) ;
#34786=CARTESIAN_POINT ( 'NONE',  ( -47.80193682758676488, 12.85650137125659143, 8.992210446493192677 ) ) ;
#34787=CARTESIAN_POINT ( 'NONE',  ( 151.1607415860635797, 52.90668588398090577, -47.71061066794121075 ) ) ;
#34799=CARTESIAN_POINT ( 'NONE',  ( -97.49219489034499020, 30.41416107059308871, -21.46345111338298750 ) ) ;
#34801=CARTESIAN_POINT ( 'NONE',  ( -25.80058235236790765, 8.733375263008326783, 69.53065690646717201 ) ) ;
#34806=CARTESIAN_POINT ( 'NONE',  ( -85.23209958216042992, 26.02162889534598733, -92.67245568390785593 ) ) ;
#34807=CARTESIAN_POINT ( 'NONE',  ( -123.6619986853277879, 45.04188181212061437, 45.28385183707185746 ) ) ;
#34810=CARTESIAN_POINT ( 'NONE',  ( 184.3941060377211443, 82.01604625189460762, 3.219449370753451944 ) ) ;
#34817=CARTESIAN_POINT ( 'NONE',  ( 164.4615316623334991, 63.29763980349831343, -19.50861212731829752 ) ) ;
#34819=CARTESIAN_POINT ( 'NONE',  ( 70.38121440378671423, 14.50253793787158685, 65.63465686359772633 ) ) ;
#34824=AXIS2_PLACEMENT_3D ( 'NONE', #51764, #51076, #40172 ) ;
#34828=CARTESIAN_POINT ( 'NONE',  ( 159.2325040199866919, 60.31699144791974021, -9.434136353667053498 ) ) ;
#34833=B_SPLINE_CURVE_WITH_KNOTS ( 'NONE', 3,
 ( #62326, #35603, #57061, #56354, #8175, #30323, #30670, #19071, #8529, #51777, #29976, #52117, #25056, #51439, #3250, #67964, #3935, #61293, #19765, #41224, #25406, #39833, #57747, #4960, #36293, #20794, #68308, #32043, #58087, #26424, #9558, #58759, #42260, #9906, #41907, #27099, #63017, #15178, #31023, #53131, #42921, #52789, #14819 ),
 .UNSPECIFIED., .F., .F.,
 ( 4, 2, 2, 2, 2, 2, 2, 2, 1, 2, 2, 2, 2, 2, 2, 2, 2, 2, 2, 2, 2, 4 ),
 ( 0.000000000000000000, 0.001465684626643313062, 0.002198526939964969701, 0.002931369253286626123, 0.004397053879929952412, 0.005862738506573278267, 0.007328423133216604123, 0.008061265446538276591, 0.008794107759859948192, 0.009526950073181621528, 0.01025979238650329313, 0.01172547701314665541, 0.01319116163979001770, 0.01465684626643337998, 0.01538968857975506026, 0.01612253089307674053, 0.01758821551972008027, 0.01905390014636342694, 0.01978674245968510548, 0.02051958477300678402, 0.02198526939965014457, 0.02345095402629350512 ),
 .UNSPECIFIED. ) ;
#34834=ORIENTED_EDGE ( 'NONE', *, *, #24955, .F. ) ;
#34835=CARTESIAN_POINT ( 'NONE',  ( -142.3178993725748853, 58.31327888234795864, -66.94886755203597772 ) ) ;
#34839=LINE ( 'NONE', #8089, #51888 ) ;
#34841=CARTESIAN_POINT ( 'NONE',  ( -101.8187363387486641, 33.67461140603122516, 3.674523915951410480 ) ) ;
#34842=CARTESIAN_POINT ( 'NONE',  ( 65.60747156646080214, 14.32439394919076570, 83.95651089761803121 ) ) ;
#34843=CARTESIAN_POINT ( 'NONE',  ( 152.6567222595844555, 55.25503842111547925, -91.54794413222496985 ) ) ;
#34844=CARTESIAN_POINT ( 'NONE',  ( 79.33384730094455506, 18.11203072455033336, -18.23467331857458262 ) ) ;
#34847=CARTESIAN_POINT ( 'NONE',  ( 131.6189313563687620, 40.08924984825279125, -63.19450288702588381 ) ) ;
#34849=CARTESIAN_POINT ( 'NONE',  ( 181.0840389613909736, 78.60582251573003987, 56.15314469597509373 ) ) ;
#34855=CARTESIAN_POINT ( 'NONE',  ( -34.74563762132952860, 11.17960945723135779, 44.45265738134296640 ) ) ;
#34856=DIRECTION ( 'NONE',  ( -0.000000000000000000, 1.000000000000000000, -0.000000000000000000 ) ) ;
#34858=CARTESIAN_POINT ( 'NONE',  ( -52.68007207639882239, 14.05813534436550682, -76.67980032479178476 ) ) ;
#34859=CARTESIAN_POINT ( 'NONE',  ( -0.7076388175553618431, 7.538734751903870546, -18.48788273639771162 ) ) ;
#34860=CARTESIAN_POINT ( 'NONE',  ( 173.7227242028390606, 71.47307702680406294, 8.499494705527911975 ) ) ;
#34861=CARTESIAN_POINT ( 'NONE',  ( -62.45356936877016807, 16.79156452995240301, 9.731492733239218040 ) ) ;
#34864=CARTESIAN_POINT ( 'NONE',  ( -99.98584758882476820, 32.75338129098884110, -49.67063086737493904 ) ) ;
#34866=CARTESIAN_POINT ( 'NONE',  ( 102.8111940033034273, 25.59308899183601582, -69.22529567365751291 ) ) ;
#34867=CARTESIAN_POINT ( 'NONE',  ( 46.23113030541875190, 10.41513832761375902, -13.16521276663865692 ) ) ;
#34868=CARTESIAN_POINT ( 'NONE',  ( 43.14356474118744700, 8.925336319666904217, 57.73968773710988245 ) ) ;
#34871=VECTOR ( 'NONE', #61029, 1000.000000000000000 ) ;
#34873=CARTESIAN_POINT ( 'NONE',  ( -173.1211646369891071, 87.12891641440859303, -22.86740657428632773 ) ) ;
#34874=CARTESIAN_POINT ( 'NONE',  ( -166.3188283541502415, 79.86268666707375985, 61.99536074306163869 ) ) ;
#34880=CARTESIAN_POINT ( 'NONE',  ( 44.67156470120503542, 9.152591717284639827, -91.40705571865771617 ) ) ;
#34881=CARTESIAN_POINT ( 'NONE',  ( -171.5023337025455135, 86.83681590836893349, 57.83153322340911018 ) ) ;
#34886=CARTESIAN_POINT ( 'NONE',  ( 61.33840119549017089, 13.32121602003047123, -23.69023232728272887 ) ) ;
#34889=CARTESIAN_POINT ( 'NONE',  ( 22.72762739171800561, 7.830015800126072456, -40.14245491239596930 ) ) ;
#34890=CARTESIAN_POINT ( 'NONE',  ( -81.67992981004168485, 23.49232121719082400, -22.64303255023387962 ) ) ;
#34892=FACE_BOUND ( 'NONE', #18667, .T. ) ;
#34896=FACE_OUTER_BOUND ( 'NONE', #66373, .T. ) ;
#34899=CARTESIAN_POINT ( 'NONE',  ( 23.26352157766197948, 6.855087657142792779, 91.89523032385697832 ) ) ;
#34901=EDGE_CURVE ( 'NONE', #55648, #42077, #48958, .T. ) ;
#34902=CARTESIAN_POINT ( 'NONE',  ( 80.72161230109723817, 17.48902961068032980, -74.81300800374665982 ) ) ;
#34903=ORIENTED_EDGE ( 'NONE', *, *, #17864, .F. ) ;
#34906=CARTESIAN_POINT ( 'NONE',  ( 197.3700262219430783, 98.41176242030789467, -42.19614285301155832 ) ) ;
#34910=CARTESIAN_POINT ( 'NONE',  ( -82.32931163805226049, 23.75065981441938234, -76.00918213230767151 ) ) ;
#34911=CARTESIAN_POINT ( 'NONE',  ( -55.53456145826333312, 15.85318253404851063, -23.37177340799620140 ) ) ;
#34912=CARTESIAN_POINT ( 'NONE',  ( 90.51709546286272712, 21.85407654229979357, -76.58433341987911547 ) ) ;
#34916=CARTESIAN_POINT ( 'NONE',  ( -108.5076394317819677, 37.20503715172082337, -91.99933385091648574 ) ) ;
#34917=CARTESIAN_POINT ( 'NONE',  ( 22.89634831467701659, 6.832298124325686395, 13.07552592342019260 ) ) ;
#34920=CARTESIAN_POINT ( 'NONE',  ( 180.2494929075577375, 79.18888319146951460, -63.06960825634327961 ) ) ;
#34921=CARTESIAN_POINT ( 'NONE',  ( -129.3970594949620363, 50.06339481638100608, -22.21707316791037456 ) ) ;
#34923=CARTESIAN_POINT ( 'NONE',  ( 79.37778929114111293, 18.12554302172300780, -41.34262384610868679 ) ) ;
#34929=CARTESIAN_POINT ( 'NONE',  ( 46.90141780929663895, 9.503798448769785523, 10.06464778740114774 ) ) ;
#34931=CARTESIAN_POINT ( 'NONE',  ( -51.13073217147959326, 13.66490163179657102, -9.474297845703558707 ) ) ;
#34933=CARTESIAN_POINT ( 'NONE',  ( 140.1272987153004124, 45.34167505388539610, -93.07698992894040657 ) ) ;
#34934=CARTESIAN_POINT ( 'NONE',  ( -26.06927550048145292, 8.771279580068128467, -91.25299760957113904 ) ) ;
#34935=CARTESIAN_POINT ( 'NONE',  ( 211.8616541147234784, 118.5646031478490414, 88.16756572905163125 ) ) ;
#34938=DIRECTION ( 'NONE',  ( -0.000000000000000000, 1.000000000000000000, -0.000000000000000000 ) ) ;
#34940=CARTESIAN_POINT ( 'NONE',  ( -10.23867141318105922, 7.059827648235817321, 30.49746343403691995 ) ) ;
#34943=CARTESIAN_POINT ( 'NONE',  ( 8.480977594057447888, 7.382886909400594000, -17.88117617556033423 ) ) ;
#34947=CARTESIAN_POINT ( 'NONE',  ( 184.5867277229703518, 83.68414666546580349, -63.93399993165346729 ) ) ;
#34948=CARTESIAN_POINT ( 'NONE',  ( -38.31648305663216547, 11.84679862791310079, 94.41515645623105968 ) ) ;
#34953=CARTESIAN_POINT ( 'NONE',  ( 131.6189313563687335, 40.08924984825279125, -36.34995229656220772 ) ) ;
#34956=CARTESIAN_POINT ( 'NONE',  ( 188.3569538602032480, 87.78382372060060845, 92.37220588221737216 ) ) ;
#34959=CARTESIAN_POINT ( 'NONE',  ( -27.48703802937314933, 8.975952825337623509, -63.28273934099161124 ) ) ;
#34962=B_SPLINE_CURVE_WITH_KNOTS ( 'NONE', 3,
 ( #26900, #16345, #54666, #1560, #38143, #48326, #6494, #21618, #15996, #22668, #21965, #160, #59583, #59249, #32525, #53953, #11399, #44107, #17383, #38862, #32873, #54305, #6127, #27589, #49028, #34279, #50790, #55368, #34969, #18438, #55728, #18095, #3301, #2962, #56769, #35310, #29338, #19124, #29683, #61350, #40578, #2609, #1930, #60652 ),
 .UNSPECIFIED., .F., .F.,
 ( 4, 2, 2, 2, 2, 2, 2, 2, 2, 2, 2, 2, 2, 2, 2, 2, 2, 2, 2, 2, 2, 4 ),
 ( 0.000000000000000000, 0.001533942663855616256, 0.003067885327711232513, 0.004601827991566848769, 0.005368799323494655162, 0.006135770655422460688, 0.007669713319278092557, 0.008436684651205906757, 0.009203655983133721824, 0.01073759864698933982, 0.01150456997891714794, 0.01227154131084495781, 0.01303851264277276420, 0.01380548397470057233, 0.01533942663855619552, 0.01687336930241181698, 0.01840731196626744018, 0.01994125463012305990, 0.02070822596205087324, 0.02147519729397868657, 0.02300913995783434793, 0.02454308262169001276 ),
 .UNSPECIFIED. ) ;
#34966=CARTESIAN_POINT ( 'NONE',  ( -56.01329802674224112, 15.98369420723829570, -77.01488154601142355 ) ) ;
#34969=CARTESIAN_POINT ( 'NONE',  ( 103.1567541746301657, 25.73937982110325606, 7.758240586775330350 ) ) ;
#34970=CARTESIAN_POINT ( 'NONE',  ( -30.94745021534356511, 10.53010394565407637, 72.06100499665291181 ) ) ;
#34972=CARTESIAN_POINT ( 'NONE',  ( -50.52927270563906603, 13.51486287463704450, 58.65938854185318263 ) ) ;
#34974=CARTESIAN_POINT ( 'NONE',  ( -1.728570918131774325, 6.570609986804655023, 60.08533143854203473 ) ) ;
#34975=ORIENTED_EDGE ( 'NONE', *, *, #12627, .F. ) ;
#34978=CARTESIAN_POINT ( 'NONE',  ( -128.9925397612932443, 48.56800623462826394, -76.09213246840596412 ) ) ;
#34981=CARTESIAN_POINT ( 'NONE',  ( -0.3508015596286013227, 7.526244656639662800, 90.60611482011238138 ) ) ;
#34989=FACE_OUTER_BOUND ( 'NONE', #35392, .T. ) ;
#34990=CARTESIAN_POINT ( 'NONE',  ( 150.5538013146980347, 53.70974888488126453, 39.82180283041768831 ) ) ;
#34992=VERTEX_POINT ( 'NONE', #65829 ) ;
#34994=CARTESIAN_POINT ( 'NONE',  ( -176.3791001330699260, 90.82833141237287577, 18.24710418921203114 ) ) ;
#34995=CARTESIAN_POINT ( 'NONE',  ( -3.857727530059801513, 6.665032499723451132, 17.14034259272734317 ) ) ;
#34996=CIRCLE ( 'NONE', #38342, 243.4957430088094839 ) ;
#34999=CARTESIAN_POINT ( 'NONE',  ( -23.93933407965395688, 9.495050561681670942, -15.47704760526285916 ) ) ;
#35000=CARTESIAN_POINT ( 'NONE',  ( 140.0614732283738704, 45.29930344725075031, 5.945277084547093693 ) ) ;
#35001=ORIENTED_EDGE ( 'NONE', *, *, #22596, .T. ) ;
#35002=CARTESIAN_POINT ( 'NONE',  ( 116.9200705848630264, 32.09536795999728298, -39.96847962606891258 ) ) ;
#35003=CARTESIAN_POINT ( 'NONE',  ( -71.57660578921959882, 20.81129687646278725, 13.57068704725283581 ) ) ;
#35005=DIRECTION ( 'NONE',  ( -0.000000000000000000, 1.000000000000000000, -0.000000000000000000 ) ) ;
#35008=CARTESIAN_POINT ( 'NONE',  ( 80.16939877002759829, 17.31693935407228935, -39.47914003811105488 ) ) ;
#35012=CARTESIAN_POINT ( 'NONE',  ( 82.73618382051373032, 19.18661415186669572, 43.62715597890617403 ) ) ;
#35015=EDGE_CURVE ( 'NONE', #58406, #52035, #18318, .T. ) ;
#35016=CARTESIAN_POINT ( 'NONE',  ( -124.3331814159187587, 45.47486189329072204, 57.62516324564902703 ) ) ;
#35017=CARTESIAN_POINT ( 'NONE',  ( -86.16710354151695128, 26.41338104675949694, -15.53640633945776273 ) ) ;
#35019=ADVANCED_FACE ( 'NONE', ( #18673 ), #29562, .F. ) ;
#35021=VERTEX_POINT ( 'NONE', #17262 ) ;
#35023=EDGE_CURVE ( 'NONE', #46840, #6856, #3392, .T. ) ;
#35025=CARTESIAN_POINT ( 'NONE',  ( 108.3906473026529653, 28.03385344351494268, 71.23839387606832929 ) ) ;
#35026=CARTESIAN_POINT ( 'NONE',  ( 164.6406716478538215, 63.44801348349341197, 61.53806796485126540 ) ) ;
#35027=CARTESIAN_POINT ( 'NONE',  ( -189.4223925288096666, 107.3427006758676043, 66.98796678033512819 ) ) ;
#35030=DIRECTION ( 'NONE',  ( -0.000000000000000000, 1.000000000000000000, -0.000000000000000000 ) ) ;
#35039=CARTESIAN_POINT ( 'NONE',  ( -73.83891297820638044, 20.54113601143295753, 85.85888820351974005 ) ) ;
#35041=EDGE_CURVE ( 'NONE', #30746, #30581, #25344, .T. ) ;
#35042=CARTESIAN_POINT ( 'NONE',  ( 67.55134213333077753, 13.77030723107741039, -49.21396399478243922 ) ) ;
#35044=CARTESIAN_POINT ( 'NONE',  ( -58.33157376762796531, 16.63098604184963847, 44.56701505676580410 ) ) ;
#35045=CARTESIAN_POINT ( 'NONE',  ( -96.45303203827903360, 31.03218867996497821, -10.92221250935651966 ) ) ;
#35047=CARTESIAN_POINT ( 'NONE',  ( 31.89767103975184881, 7.551769522480730856, 90.89116849545793286 ) ) ;
#35051=CARTESIAN_POINT ( 'NONE',  ( -102.2801239173131052, 32.78103895658057354, -76.85912785543962400 ) ) ;
#35052=CARTESIAN_POINT ( 'NONE',  ( -189.7987719395349018, 107.8653664616570467, -39.23015726446638496 ) ) ;
#35053=DIRECTION ( 'NONE',  ( -0.000000000000000000, 1.000000000000000000, -0.000000000000000000 ) ) ;
#35054=CARTESIAN_POINT ( 'NONE',  ( 22.90619343622340764, 7.840927939412482672, -18.58827641307582468 ) ) ;
#35055=CARTESIAN_POINT ( 'NONE',  ( 201.6034029841262338, 102.1956603101140644, 70.39772623200110502 ) ) ;
#35056=EDGE_LOOP ( 'NONE', ( #7696, #57667, #16248, #51724 ) ) ;
#35057=CARTESIAN_POINT ( 'NONE',  ( 133.4058733589413919, 42.32720528873925048, -51.02331093239570237 ) ) ;
#35058=CARTESIAN_POINT ( 'NONE',  ( -38.87871322265797858, 11.95691939779334767, -41.83587164630765187 ) ) ;
#35060=CARTESIAN_POINT ( 'NONE',  ( -165.6130566995026356, 79.14211131649287267, 92.14615457014019739 ) ) ;
#35062=CARTESIAN_POINT ( 'NONE',  ( 126.3681350380370958, 38.23508791628619008, 10.65839973360038684 ) ) ;
#35063=CARTESIAN_POINT ( 'NONE',  ( -149.2910611247328063, 63.99625741915658494, -7.968279941028271196 ) ) ;
#35066=CARTESIAN_POINT ( 'NONE',  ( 150.1360066839118304, 53.40685429604861412, 92.17743685337597981 ) ) ;
#35067=EDGE_LOOP ( 'NONE', ( #335, #25530, #38676, #6039 ) ) ;
#35068=CARTESIAN_POINT ( 'NONE',  ( -62.29496909743954092, 17.79481128341708285, 12.93814815294244269 ) ) ;
#35069=CARTESIAN_POINT ( 'NONE',  ( 127.4750938923429402, 37.70245908594343121, 33.06177329601652559 ) ) ;
#35070=CARTESIAN_POINT ( 'NONE',  ( -155.7455325080991315, 71.01834415181987481, 42.39273526441780859 ) ) ;
#35071=VECTOR ( 'NONE', #25988, 1000.000000000000000 ) ;
#35078=CARTESIAN_POINT ( 'NONE',  ( 63.01563776193090405, 12.67277567978497643, 44.81296093922130552 ) ) ;
#35080=ORIENTED_EDGE ( 'NONE', *, *, #32737, .T. ) ;
#35081=CARTESIAN_POINT ( 'NONE',  ( -166.7050147108375313, 81.70694330787516435, 15.40055725785405727 ) ) ;
#35082=CARTESIAN_POINT ( 'NONE',  ( 17.72992212664810197, 6.570588738776104165, -77.11196272085689429 ) ) ;
#35083=CARTESIAN_POINT ( 'NONE',  ( -132.9126122820979390, 52.52752252041128145, 62.30792293928088554 ) ) ;
#35085=CARTESIAN_POINT ( 'NONE',  ( -96.88714137552827310, 31.24002647487883522, 86.48642051269072795 ) ) ;
#35089=CARTESIAN_POINT ( 'NONE',  ( 180.3998223972066910, 79.34418886440140284, -89.93734709859124621 ) ) ;
#35091=CARTESIAN_POINT ( 'NONE',  ( 134.7720294983483598, 43.15885542353189663, 44.46810067847044223 ) ) ;
#35092=CARTESIAN_POINT ( 'NONE',  ( 117.7442255600442422, 33.63739995216995737, 36.61229788494631521 ) ) ;
#35093=CARTESIAN_POINT ( 'NONE',  ( -130.5904357464317229, 50.88938808445627160, 17.14299821243472977 ) ) ;
#35094=CARTESIAN_POINT ( 'NONE',  ( 65.62985354949974237, 14.32996029952553840, -63.03137781880401036 ) ) ;
#35097=EDGE_CURVE ( 'NONE', #61600, #69216, #52406, .T. ) ;
#35098=CARTESIAN_POINT ( 'NONE',  ( -145.3246383987844297, 62.00818849034183700, -21.69799560209030531 ) ) ;
#35102=CARTESIAN_POINT ( 'NONE',  ( -142.3393481102175713, 58.33014244976926932, 35.99748335774498287 ) ) ;
#35103=CARTESIAN_POINT ( 'NONE',  ( -129.4098618459771615, 48.85263848239743822, 58.33566833192991652 ) ) ;
#35104=CARTESIAN_POINT ( 'NONE',  ( -169.1005390226459042, 82.76152663947081578, -62.70965392198332466 ) ) ;
#35113=CARTESIAN_POINT ( 'NONE',  ( 134.3182571105338923, 42.88121222759020412, 71.35489142945908725 ) ) ;
#35117=CARTESIAN_POINT ( 'NONE',  ( -15.13211202216340823, 8.488266782358833140, -44.62742559165378253 ) ) ;
#35118=AXIS2_PLACEMENT_3D ( 'NONE', #66498, #17596, #39747 ) ;
#35120=CARTESIAN_POINT ( 'NONE',  ( 152.8430172091322561, 54.14068524174418684, -49.53136367997995393 ) ) ;
#35123=CARTESIAN_POINT ( 'NONE',  ( -109.6829043543429236, 36.70322915510440254, -95.00000000000133582 ) ) ;
#35125=DIRECTION ( 'NONE',  ( -0.000000000000000000, 1.000000000000000000, -0.000000000000000000 ) ) ;
#35126=CARTESIAN_POINT ( 'NONE',  ( -62.50103539982530521, 17.85731685071834818, 63.65098158254257754 ) ) ;
#35128=ORIENTED_EDGE ( 'NONE', *, *, #3444, .F. ) ;
#35130=CARTESIAN_POINT ( 'NONE',  ( -10.23402954931276554, 7.059791383763807993, -62.65565335715368889 ) ) ;
#35131=CARTESIAN_POINT ( 'NONE',  ( -37.38262509017738466, 10.64263598035110547, 42.31726256907158756 ) ) ;
#35136=B_SPLINE_CURVE_WITH_KNOTS ( 'NONE', 3,
 ( #40494, #49646, #44742, #60564, #66559, #51059, #13426, #45075, #45781, #18348, #39810, #55991, #50706, #61264, #13087, #67256, #34889, #23976, #19042, #33501, #54929, #1474, #12381, #33840, #55281, #13764, #4258, #67587, #30300, #19734, #19386, #61945, #62991, #30641, #40844, #63340, #51414, #14464, #35222, #9882, #47149, #46116, #31335 ),
 .UNSPECIFIED., .F., .F.,
 ( 4, 2, 2, 2, 2, 2, 2, 2, 1, 2, 2, 2, 2, 2, 2, 2, 2, 2, 2, 2, 2, 4 ),
 ( 0.000000000000000000, 0.001466285743483476288, 0.002199428615225214323, 0.002932571486966952575, 0.004398857230450438187, 0.005865142973933924232, 0.007331428717417410278, 0.008064571589159153300, 0.008797714460900897190, 0.009530857332642639346, 0.01026400020438438324, 0.01173028594786784673, 0.01319657169135131022, 0.01466285743483477372, 0.01539600030657651587, 0.01612914317831826150, 0.01759542892180174581, 0.01906171466528523359, 0.01979485753702698095, 0.02052800040876873178, 0.02199428615225221609, 0.02346057189573570387 ),
 .UNSPECIFIED. ) ;
#35139=CARTESIAN_POINT ( 'NONE',  ( -156.9900125991010214, 72.16580261738671709, 64.47870932869700766 ) ) ;
#35140=CARTESIAN_POINT ( 'NONE',  ( -118.6157340058429668, 41.88485941274766589, 39.95035298570361704 ) ) ;
#35141=CARTESIAN_POINT ( 'NONE',  ( -59.57733000654214095, 15.94108165424593793, -48.71746015130258911 ) ) ;
#35142=ORIENTED_EDGE ( 'NONE', *, *, #23228, .F. ) ;
#35143=CARTESIAN_POINT ( 'NONE',  ( -180.5801285865472039, 97.42945596116102536, -69.85561729999363934 ) ) ;
#35145=CARTESIAN_POINT ( 'NONE',  ( 112.5721302457195634, 29.97407549554797868, 44.25599282069087081 ) ) ;
#35148=VERTEX_POINT ( 'NONE', #41166 ) ;
#35150=CARTESIAN_POINT ( 'NONE',  ( 116.1021807117071774, 31.68810634233424395, -65.55867728159829255 ) ) ;
#35151=CARTESIAN_POINT ( 'NONE',  ( 68.45098769362923008, 13.99935947269945480, 58.98388901208659263 ) ) ;
#35152=CARTESIAN_POINT ( 'NONE',  ( 136.7690435008551333, 44.39743995805025634, 3.250471752906729517 ) ) ;
#35155=EDGE_CURVE ( 'NONE', #34477, #19832, #43860, .T. ) ;
#35160=CARTESIAN_POINT ( 'NONE',  ( 127.0701306906838397, 37.47492071169578054, 87.48711923404823665 ) ) ;
#35162=CARTESIAN_POINT ( 'NONE',  ( -145.9095871962850879, 61.18682730038540285, -62.57265054608006238 ) ) ;
#35165=CARTESIAN_POINT ( 'NONE',  ( 164.9534461562627712, 63.71129898458567453, -44.20161124359641036 ) ) ;
#35172=CARTESIAN_POINT ( 'NONE',  ( 69.38831087449705137, 15.28150064080604942, 87.03339823595428015 ) ) ;
#35175=CARTESIAN_POINT ( 'NONE',  ( 46.68054346512387554, 10.48734223171576829, -95.00000000000133582 ) ) ;
#35177=CARTESIAN_POINT ( 'NONE',  ( -142.6040384731713004, 58.53810651789324737, -93.02743765931519704 ) ) ;
#35178=FACE_OUTER_BOUND ( 'NONE', #46830, .T. ) ;
#35181=CARTESIAN_POINT ( 'NONE',  ( -100.4440683050664802, 32.98184228837414622, 72.15012103992511072 ) ) ;
#35182=DIRECTION ( 'NONE',  ( 0.000000000000000000, 0.000000000000000000, 1.000000000000000000 ) ) ;
#35186=EDGE_CURVE ( 'NONE', #22496, #49023, #13606, .T. ) ;
#35187=CARTESIAN_POINT ( 'NONE',  ( -156.7435307435793845, 71.93726016406968427, -44.30516796381674283 ) ) ;
#35188=CARTESIAN_POINT ( 'NONE',  ( 211.7357196141372526, 118.3691710715567353, -14.37225973309041827 ) ) ;
#35189=CARTESIAN_POINT ( 'NONE',  ( -156.4960819023051499, 70.34114605623875605, -66.38289013128127181 ) ) ;
#35191=CARTESIAN_POINT ( 'NONE',  ( -47.55360235114366674, 12.79819361309569103, -70.07348629407573526 ) ) ;
#35192=CARTESIAN_POINT ( 'NONE',  ( -4.506365319453812468, 7.705038994660875495, -22.80363844821005515 ) ) ;
#35193=CARTESIAN_POINT ( 'NONE',  ( 179.0096185093687495, 76.53352131383243773, 2.743568850346190136 ) ) ;
#35196=CARTESIAN_POINT ( 'NONE',  ( -101.3537077702550562, 33.43904726487055967, -35.05764247501280551 ) ) ;
#35199=B_SPLINE_CURVE_WITH_KNOTS ( 'NONE', 3,
 ( #32129, #41992, #58173, #106, #38088, #15610, #53906, #15949, #42341, #48617, #32474, #21231, #64133, #58849, #37394, #37059, #53565, #5045, #10320, #10661, #5727, #47595, #16632, #36727, #31783, #27186, #31108, #458, #5398, #20883, #21563, #52876, #25832, #63456, #9989, #26507, #58498, #4702, #21912, #42677, #43006, #53216, #43360, #37744 ),
 .UNSPECIFIED., .F., .F.,
 ( 4, 2, 2, 2, 2, 2, 2, 2, 2, 2, 2, 2, 2, 2, 2, 2, 2, 2, 2, 2, 2, 4 ),
 ( 0.02895403260893130923, 0.03071603688922217718, 0.03247804116951304165, 0.03424004544980391307, 0.03600204973009477755, 0.03776405401038564202, 0.03864505615053107773, 0.03952605829067650650, 0.04040706043082194221, 0.04128806257096737098, 0.04216906471111279975, 0.04305006685125822852, 0.04393106899140365729, 0.04481207113154909299, 0.04569307327169452176, 0.04657407541183995053, 0.04745507755198538624, 0.04833607969213081501, 0.05009808397242168643, 0.05186008825271255784, 0.05362209253300343620, 0.05714610109358520679 ),
 .UNSPECIFIED. ) ;
#35200=EDGE_CURVE ( 'NONE', #34109, #31066, #39340, .T. ) ;
#35201=CARTESIAN_POINT ( 'NONE',  ( 46.65860211212413589, 10.48377752989033951, -14.31619431203790960 ) ) ;
#35205=EDGE_CURVE ( 'NONE', #58006, #59279, #7690, .T. ) ;
#35207=CARTESIAN_POINT ( 'NONE',  ( -107.0544991134679691, 36.41543129049374272, -21.45915251517910960 ) ) ;
#35209=CARTESIAN_POINT ( 'NONE',  ( -165.6393662153604396, 79.16886183052815795, 65.77194331359760326 ) ) ;
#35211=EDGE_LOOP ( 'NONE', ( #51419, #61501 ) ) ;
#35212=DIRECTION ( 'NONE',  ( 0.000000000000000000, 0.000000000000000000, 1.000000000000000000 ) ) ;
#35214=CARTESIAN_POINT ( 'NONE',  ( 173.6710158776850506, 71.42507420636734139, -18.05732277655958384 ) ) ;
#35215=CARTESIAN_POINT ( 'NONE',  ( 102.7414208686707582, 26.65627265923299305, 64.44516497733118854 ) ) ;
#35219=CARTESIAN_POINT ( 'NONE',  ( 55.51637278631173444, 12.08345311280959677, -16.88578774313057096 ) ) ;
#35222=CARTESIAN_POINT ( 'NONE',  ( 18.20314211955701111, 7.596739727129572017, -50.13654653627244784 ) ) ;
#35223=CARTESIAN_POINT ( 'NONE',  ( 15.29305096970402822, 7.491604910111008486, 71.85925826316895382 ) ) ;
#35225=FACE_BOUND ( 'NONE', #34404, .T. ) ;
#35227=VECTOR ( 'NONE', #4003, 1000.000000000000000 ) ;
#35230=EDGE_LOOP ( 'NONE', ( #63760, #51300, #10857, #31546 ) ) ;
#35236=CARTESIAN_POINT ( 'NONE',  ( 15.12874021383972334, 6.480380938026408799, 83.72563133567338411 ) ) ;
#35237=CARTESIAN_POINT ( 'NONE',  ( 83.38067517854670996, 18.33799117207140128, -76.93039019878386853 ) ) ;
#35238=VERTEX_POINT ( 'NONE', #6633 ) ;
#35240=CARTESIAN_POINT ( 'NONE',  ( 203.9228889538744909, 106.9879579748728275, -51.29625234351511409 ) ) ;
#35241=ORIENTED_EDGE ( 'NONE', *, *, #30736, .T. ) ;
#35248=ORIENTED_EDGE ( 'NONE', *, *, #36540, .F. ) ;
#35252=CARTESIAN_POINT ( 'NONE',  ( 106.6181401479172166, 28.34160787025143335, 16.83688178611173214 ) ) ;
#35257=DIRECTION ( 'NONE',  ( 0.000000000000000000, 0.000000000000000000, 1.000000000000000000 ) ) ;
#35258=CARTESIAN_POINT ( 'NONE',  ( 173.6737675136087660, 72.80308721038095143, -71.76398898605381760 ) ) ;
#35261=CARTESIAN_POINT ( 'NONE',  ( 110.7164744784864041, 29.10110206241302322, -9.077886975190001095 ) ) ;
#35262=EDGE_CURVE ( 'NONE', #10027, #29060, #29137, .T. ) ;
#35263=CARTESIAN_POINT ( 'NONE',  ( 79.54836217416617217, 18.17815803851260270, -45.80621361996720964 ) ) ;
#35269=CARTESIAN_POINT ( 'NONE',  ( 46.50207827473962396, 9.439498081273464791, 8.140350865663473101 ) ) ;
#35273=CARTESIAN_POINT ( 'NONE',  ( 128.9253503890652439, 38.52561778336672660, 4.509604327398147205 ) ) ;
#35278=CARTESIAN_POINT ( 'NONE',  ( 211.3757499519976477, 117.8130818709823444, 40.13274018705065771 ) ) ;
#35279=CARTESIAN_POINT ( 'NONE',  ( -81.23268307104839892, 24.39742801172154785, 57.71144102871279813 ) ) ;
#35280=DIRECTION ( 'NONE',  ( 0.000000000000000000, 0.000000000000000000, 1.000000000000000000 ) ) ;
#35281=ORIENTED_EDGE ( 'NONE', *, *, #66176, .T. ) ;
#35282=AXIS2_PLACEMENT_3D ( 'NONE', #28489, #39055, #1767 ) ;
#35283=CARTESIAN_POINT ( 'NONE',  ( 8.540564391411907152, 7.383006541823029067, -18.11898453561821398 ) ) ;
#35287=FACE_OUTER_BOUND ( 'NONE', #22688, .T. ) ;
#35288=CARTESIAN_POINT ( 'NONE',  ( 184.3879440808140373, 83.47316703125162007, -63.83297031623806816 ) ) ;
#35289=CIRCLE ( 'NONE', #56464, 243.4957430088094839 ) ;
#35290=CARTESIAN_POINT ( 'NONE',  ( -169.8972248494842745, 85.08697738648012887, 45.10824208028097360 ) ) ;
#35291=CARTESIAN_POINT ( 'NONE',  ( -94.88380767928869375, 29.17964217339916289, -41.24520491189826288 ) ) ;
#35293=CARTESIAN_POINT ( 'NONE',  ( -28.35957743809534648, 10.12373109553627337, 4.028907504916732663 ) ) ;
#35294=FACE_OUTER_BOUND ( 'NONE', #37627, .T. ) ;
#35295=CARTESIAN_POINT ( 'NONE',  ( 9.280894575734583540, 7.385644305345138605, -46.77988395504912944 ) ) ;
#35297=CYLINDRICAL_SURFACE ( 'NONE', #48654, 7.500000000000020428 ) ;
#35300=CARTESIAN_POINT ( 'NONE',  ( 185.5740152438940243, 84.73932458755626840, 84.48237900350213181 ) ) ;
#35307=CARTESIAN_POINT ( 'NONE',  ( -62.30163634902122283, 17.79682011226254090, -71.54896639739239106 ) ) ;
#35308=CARTESIAN_POINT ( 'NONE',  ( 176.6258282025054598, 74.21441092921637050, -76.60518865254823595 ) ) ;
#35309=CARTESIAN_POINT ( 'NONE',  ( -173.9656771507954716, 88.06879734510549440, -34.71195716474998250 ) ) ;
#35310=CARTESIAN_POINT ( 'NONE',  ( 106.4107271020440209, 27.14892220304137993, 3.815184072439286922 ) ) ;
#35313=CARTESIAN_POINT ( 'NONE',  ( -189.8133172329396814, 107.8858115918112901, 94.99999999999866418 ) ) ;
#35315=CARTESIAN_POINT ( 'NONE',  ( -3.868882431147342427, 6.665575841812235502, 58.08385180160794192 ) ) ;
#35319=CARTESIAN_POINT ( 'NONE',  ( -128.1384526288949530, 47.98891607499722056, -76.42915334089175872 ) ) ;
#35320=CARTESIAN_POINT ( 'NONE',  ( -109.7790042512818047, 37.90666514836944145, -69.65031332244757323 ) ) ;
#35321=CARTESIAN_POINT ( 'NONE',  ( -48.04019567818504299, 12.91272349839804612, -40.04495495352035306 ) ) ;
#35328=LINE ( 'NONE', #66660, #23732 ) ;
#35329=ORIENTED_EDGE ( 'NONE', *, *, #24220, .T. ) ;
#35333=CARTESIAN_POINT ( 'NONE',  ( 178.1903523079567151, 75.72906488635189248, -50.65795404092384757 ) ) ;
#35334=CARTESIAN_POINT ( 'NONE',  ( 150.2193536046551969, 53.46717047532150957, 34.97374097100669843 ) ) ;
#35340=CARTESIAN_POINT ( 'NONE',  ( -5.416136198635860488, 6.745992685878680284, 3.664297029461999422 ) ) ;
#35342=CARTESIAN_POINT ( 'NONE',  ( -84.53753601793931693, 25.73343139558518544, 33.22451195744211105 ) ) ;
#35343=CARTESIAN_POINT ( 'NONE',  ( 156.3719388878481027, 56.80180099471265720, 83.17326589912873658 ) ) ;
#35344=CARTESIAN_POINT ( 'NONE',  ( 141.2366329129481528, 46.06278879703612716, 8.803202109551088839 ) ) ;
#35350=CARTESIAN_POINT ( 'NONE',  ( 46.42281973867196854, 9.426811321855151249, -40.47057392414230037 ) ) ;
#35352=DIRECTION ( 'NONE',  ( -1.000000000000000000, 0.000000000000000000, 0.000000000000000000 ) ) ;
#35354=ORIENTED_EDGE ( 'NONE', *, *, #43789, .T. ) ;
#35355=CARTESIAN_POINT ( 'NONE',  ( 79.23200707685333555, 17.02828389812517074, -42.05917643671551787 ) ) ;
#35356=ORIENTED_EDGE ( 'NONE', *, *, #8167, .F. ) ;
#35360=CARTESIAN_POINT ( 'NONE',  ( 79.19119222799093905, 18.06817527909836230, 38.20617424704751386 ) ) ;
#35361=CARTESIAN_POINT ( 'NONE',  ( 197.6316695787931508, 97.13022718399025734, -68.13838693519056733 ) ) ;
#35364=CARTESIAN_POINT ( 'NONE',  ( -81.90760111942957167, 24.66532273091449667, -8.990629716813376859 ) ) ;
#35365=CARTESIAN_POINT ( 'NONE',  ( -175.9944734395086527, 91.92390745845763433, -8.426759268301923456 ) ) ;
#35367=CARTESIAN_POINT ( 'NONE',  ( 204.6977192012829789, 108.0580384837234931, 17.36317014830577321 ) ) ;
#35370=CARTESIAN_POINT ( 'NONE',  ( -104.5916564445180228, 35.10571011602407765, 18.32481510845080663 ) ) ;
#35371=CARTESIAN_POINT ( 'NONE',  ( 15.78827728214693416, -170.0000000000000000, -89.20804527961313113 ) ) ;
#35374=CIRCLE ( 'NONE', #21895, 242.4895526022646379 ) ;
#35376=CARTESIAN_POINT ( 'NONE',  ( 19.10216788411014122, 6.629360741291162817, 30.78208475216976225 ) ) ;
#35377=ADVANCED_FACE ( 'NONE', ( #13646 ), #52316, .F. ) ;
#35378=CARTESIAN_POINT ( 'NONE',  ( -142.4962548760750281, 59.73493706050192031, 89.22523109323365986 ) ) ;
#35380=ORIENTED_EDGE ( 'NONE', *, *, #3499, .T. ) ;
#35382=ORIENTED_EDGE ( 'NONE', *, *, #41809, .T. ) ;
#35384=CARTESIAN_POINT ( 'NONE',  ( -72.74158548548088277, 20.15252735510585325, 86.99778511234599421 ) ) ;
#35385=CARTESIAN_POINT ( 'NONE',  ( 173.9832054143776077, 71.71542822834034325, -95.00000000000133582 ) ) ;
#35386=CARTESIAN_POINT ( 'NONE',  ( 66.94779593213118574, 13.61918177102166183, -36.82943163571080447 ) ) ;
#35389=CARTESIAN_POINT ( 'NONE',  ( -37.93379515072631847, 11.77251734620209156, -73.44473663808183517 ) ) ;
#35390=CARTESIAN_POINT ( 'NONE',  ( 56.52205390515081973, 12.28646189164058100, 41.09788869876410899 ) ) ;
#35391=CARTESIAN_POINT ( 'NONE',  ( 43.73690422994441462, 9.012838840865988743, 84.97377783626691894 ) ) ;
#35392=EDGE_LOOP ( 'NONE', ( #15726, #9791, #66613, #12051 ) ) ;
#35393=CARTESIAN_POINT ( 'NONE',  ( -2.874437057892791803, 6.618922960888053098, -48.57289573616785816 ) ) ;
#35397=CARTESIAN_POINT ( 'NONE',  ( 129.6961120139403647, 38.96846414226718736, -22.92345578965780462 ) ) ;
#35398=CYLINDRICAL_SURFACE ( 'NONE', #35472, 7.500000000000027534 ) ;
#35400=ORIENTED_EDGE ( 'NONE', *, *, #47714, .T. ) ;
#35403=CARTESIAN_POINT ( 'NONE',  ( -33.12994257348896099, 10.89587983539684757, -50.12821252459180243 ) ) ;
#35405=CARTESIAN_POINT ( 'NONE',  ( 181.9411407973024950, 80.91291802046383452, -36.22505766587962484 ) ) ;
#35409=CARTESIAN_POINT ( 'NONE',  ( -29.04258984626622464, 9.210213971636679986, -23.08366245703133046 ) ) ;
#35411=CARTESIAN_POINT ( 'NONE',  ( 200.8383807319521281, 102.8517715783673623, 3.418042344880998229 ) ) ;
#35416=CARTESIAN_POINT ( 'NONE',  ( -56.97556689808916275, 16.24958672959845885, 18.22614236532972498 ) ) ;
#35417=CARTESIAN_POINT ( 'NONE',  ( 129.5193594945039308, 38.86618897895343139, 43.14722117905061083 ) ) ;
#35420=CARTESIAN_POINT ( 'NONE',  ( -157.0069571479806996, 72.18154199622279066, 37.92026323496924789 ) ) ;
#35427=CARTESIAN_POINT ( 'NONE',  ( 55.56474667084417263, 11.06706367715628758, 38.30556224444529079 ) ) ;
#35431=CARTESIAN_POINT ( 'NONE',  ( -165.6208371326873419, 80.58821715390998008, 11.17930752570401332 ) ) ;
#35434=CYLINDRICAL_SURFACE ( 'NONE', #67525, 7.500000000000020428 ) ;
#35436=CARTESIAN_POINT ( 'NONE',  ( -131.6399667378751133, 51.62465701391631256, 69.81063530948696894 ) ) ;
#35439=CARTESIAN_POINT ( 'NONE',  ( -71.57660578921959882, 20.81129687646280146, -40.11841413367452702 ) ) ;
#35441=CARTESIAN_POINT ( 'NONE',  ( 175.0086665638700083, 74.06151034403055178, -93.01110694259065781 ) ) ;
#35442=CARTESIAN_POINT ( 'NONE',  ( 136.1037846510193106, 43.98155406734453265, 44.18067958987710142 ) ) ;
#35445=CARTESIAN_POINT ( 'NONE',  ( 63.50537371531942910, 13.81987663608982331, -62.56524142263342014 ) ) ;
#35446=ORIENTED_EDGE ( 'NONE', *, *, #61796, .F. ) ;
#35450=DIRECTION ( 'NONE',  ( -0.000000000000000000, 1.000000000000000000, -0.000000000000000000 ) ) ;
#35451=CARTESIAN_POINT ( 'NONE',  ( -55.05276343752910151, 14.68156374112637330, -88.90542517938719413 ) ) ;
#35452=LINE ( 'NONE', #44351, #56754 ) ;
#35454=CARTESIAN_POINT ( 'NONE',  ( -146.5268141329886760, 61.69196909035590437, 45.10686021381179955 ) ) ;
#35455=CARTESIAN_POINT ( 'NONE',  ( -121.5928001448269100, 44.91559452735375402, 44.28205460033795049 ) ) ;
#35456=CARTESIAN_POINT ( 'NONE',  ( -172.3018509397888636, 86.22053936367348115, -61.58980725186435734 ) ) ;
#35458=CARTESIAN_POINT ( 'NONE',  ( -109.4995148930278646, 37.75156937139183100, 35.92031809713896706 ) ) ;
#35461=CARTESIAN_POINT ( 'NONE',  ( -180.4790817662267557, 95.71028656509025723, -94.42029243692577722 ) ) ;
#35465=PLANE ( 'NONE',  #61428 ) ;
#35470=CARTESIAN_POINT ( 'NONE',  ( 15.78827728214693416, -170.0000000000000000, 10.67015708224156079 ) ) ;
#35472=AXIS2_PLACEMENT_3D ( 'NONE', #8677, #68442, #25884 ) ;
#35473=AXIS2_PLACEMENT_3D ( 'NONE', #15249, #41630, #52529 ) ;
#35477=LINE ( 'NONE', #30207, #10404 ) ;
#35478=CARTESIAN_POINT ( 'NONE',  ( -62.06231780744546001, 17.72446026058427293, 67.34115632414402342 ) ) ;
#35479=CARTESIAN_POINT ( 'NONE',  ( -189.2442476610617916, 107.0963225822736007, 12.01318184954264368 ) ) ;
#35482=CARTESIAN_POINT ( 'NONE',  ( -57.15434679788744887, 15.25497255977697186, -89.20270284046692666 ) ) ;
#35483=CARTESIAN_POINT ( 'NONE',  ( -37.79601571721867970, 10.72155118426296738, 41.70395869289448143 ) ) ;
#35484=CARTESIAN_POINT ( 'NONE',  ( 135.4423125506058909, 42.39015362494584593, -50.85732353738030298 ) ) ;
#35487=ORIENTED_EDGE ( 'NONE', *, *, #65928, .T. ) ;
#35489=CARTESIAN_POINT ( 'NONE',  ( -156.7435307435793845, 71.93726016406968427, 63.07303439803798994 ) ) ;
#35492=ORIENTED_EDGE ( 'NONE', *, *, #43892, .F. ) ;
#35493=CARTESIAN_POINT ( 'NONE',  ( -175.9944734395087096, 91.92390745845763433, -62.11586044922930938 ) ) ;
#35494=CARTESIAN_POINT ( 'NONE',  ( 134.2297964129789136, 42.82763724447237053, 83.20224964760393505 ) ) ;
#35495=CARTESIAN_POINT ( 'NONE',  ( 117.7411475730015269, 32.50808475802734421, 36.56858284938125792 ) ) ;
#35497=CARTESIAN_POINT ( 'NONE',  ( -55.05276343752909440, 15.72344139423347364, -62.06087458892354647 ) ) ;
#35499=B_SPLINE_CURVE_WITH_KNOTS ( 'NONE', 3,
 ( #28785, #7330, #12254, #50927, #7681, #38994, #29128, #1700, #40026, #61486, #45296, #33717, #60778, #23158, #13306, #6622, #8016, #24208, #49874, #65728, #45654, #67133, #18921, #61815, #49514, #17517, #55147, #6973, #44607, #39335, #12602, #30509, #51283, #9751, #8375, #20635, #45992, #35093, #25928, #56905, #9059, #52307, #3098, #40708, #24557, #9405, #51962, #67462 ),
 .UNSPECIFIED., .F., .F.,
 ( 4, 2, 2, 2, 2, 2, 2, 2, 2, 2, 2, 2, 2, 2, 2, 2, 2, 2, 2, 2, 2, 2, 2, 4 ),
 ( 0.02554216173022672356, 0.02715505844859244372, 0.02796150680777527431, 0.02876795516695810837, 0.03038085188532369668, 0.03199374860368928153, 0.03360664532205487331, 0.03441309368123766227, 0.03521954204042045122, 0.03602599039960324712, 0.03683243875878603607, 0.03844533547715162092, 0.03925178383633440987, 0.04005823219551719883, 0.04086468055469999472, 0.04167112891388279061, 0.04247757727306557263, 0.04328402563224836852, 0.04489692235061398806, 0.04650981906897960760, 0.04731626742816241737, 0.04812271578734523408, 0.04973561250571080505, 0.05134850922407638296 ),
 .UNSPECIFIED. ) ;
#35503=CARTESIAN_POINT ( 'NONE',  ( 114.6890011751076344, 30.99337387307412683, -64.20757585925009892 ) ) ;
#35504=CARTESIAN_POINT ( 'NONE',  ( 67.55134213333079174, 13.77030723107741217, 58.16423836707232198 ) ) ;
#35505=CARTESIAN_POINT ( 'NONE',  ( 141.0517870458593279, 47.14452711594498169, 12.29862548867962957 ) ) ;
#35506=EDGE_CURVE ( 'NONE', #25468, #15010, #30423, .T. ) ;
#35509=CARTESIAN_POINT ( 'NONE',  ( 164.4760519199595592, 64.62478832434435105, -14.04941869432099644 ) ) ;
#35512=CYLINDRICAL_SURFACE ( 'NONE', #7567, 7.500000000000013323 ) ;
#35513=CARTESIAN_POINT ( 'NONE',  ( 135.1687848281947879, 42.22135448245729350, 83.28891585102797990 ) ) ;
#35514=EDGE_CURVE ( 'NONE', #28520, #53742, #10220, .T. ) ;
#35518=CARTESIAN_POINT ( 'NONE',  ( 164.0105905242218398, 64.23277447906895077, -47.30424189763910903 ) ) ;
#35519=CARTESIAN_POINT ( 'NONE',  ( 86.62931800182293784, 19.42108912189599934, 17.86753698201564688 ) ) ;
#35520=CARTESIAN_POINT ( 'NONE',  ( 164.3702714028688661, 63.22112480708620552, -40.67253380548667252 ) ) ;
#35523=ORIENTED_EDGE ( 'NONE', *, *, #17786, .F. ) ;
#35526=B_SPLINE_CURVE_WITH_KNOTS ( 'NONE', 3,
 ( #44958, #66444, #13311, #33722, #24213, #12967, #17884, #39341, #67140, #1355, #22807, #55153, #38640, #11901, #18231, #49880, #1706, #60784 ),
 .UNSPECIFIED., .F., .F.,
 ( 4, 2, 2, 2, 2, 2, 2, 2, 4 ),
 ( 0.000000000000000000, 0.001730692900494939504, 0.002596039350742405244, 0.003461385800989870767, 0.005192078701484792273, 0.006922771601979714647, 0.008653464502474636152, 0.01038415740296955853, 0.01384554320395945531 ),
 .UNSPECIFIED. ) ;
#35528=CARTESIAN_POINT ( 'NONE',  ( -128.1219934350341703, 47.97781708504718523, 45.29597212495090730 ) ) ;
#35531=CARTESIAN_POINT ( 'NONE',  ( 84.05289558242220949, 19.61733656419350424, -23.52466748769439064 ) ) ;
#35532=CARTESIAN_POINT ( 'NONE',  ( -172.7154982671752350, 86.67743928531949393, 30.82169460664102445 ) ) ;
#35533=CARTESIAN_POINT ( 'NONE',  ( -34.74740905761644427, 10.15745573515589051, -62.91308403526972626 ) ) ;
#35536=CARTESIAN_POINT ( 'NONE',  ( -98.67557579989346550, 32.10670856967970366, 58.26914703332497680 ) ) ;
#35539=CARTESIAN_POINT ( 'NONE',  ( 151.7783534118502189, 54.60545177578660514, -11.88952959584610447 ) ) ;
#35541=CARTESIAN_POINT ( 'NONE',  ( 104.4006536356074264, 27.36759527624478849, 32.38183756136254488 ) ) ;
#35543=CARTESIAN_POINT ( 'NONE',  ( 60.76851555108127911, 12.16255188786386121, 83.83909766377725248 ) ) ;
#35544=CARTESIAN_POINT ( 'NONE',  ( 184.3879440808139805, 83.47316703125160586, 16.70068145515297076 ) ) ;
#35545=CARTESIAN_POINT ( 'NONE',  ( 208.6132326550594485, 111.8685719053116685, -37.41518418271493829 ) ) ;
#35546=CYLINDRICAL_SURFACE ( 'NONE', #16387, 7.500000000000013323 ) ;
#35551=CARTESIAN_POINT ( 'NONE',  ( 103.9652201950894863, 26.08439499369982784, -66.15590445722637014 ) ) ;
#35555=CARTESIAN_POINT ( 'NONE',  ( -1.186912488840190738, 6.549538057797848367, 87.79949317012332699 ) ) ;
#35557=EDGE_LOOP ( 'NONE', ( #40534, #53076, #48176, #13907 ) ) ;
#35560=CARTESIAN_POINT ( 'NONE',  ( -172.3057147739576749, 86.22480007276996616, 57.69916216524889307 ) ) ;
#35561=ORIENTED_EDGE ( 'NONE', *, *, #64944, .F. ) ;
#35563=CARTESIAN_POINT ( 'NONE',  ( -154.7998111145352027, 68.80117179139328698, 32.88503397576067044 ) ) ;
#35565=CARTESIAN_POINT ( 'NONE',  ( 173.8575673535406168, 71.59843387604338716, -18.90830546057937056 ) ) ;
#35567=CARTESIAN_POINT ( 'NONE',  ( 104.7042813665017746, 27.49927371769997819, 69.03645308503956812 ) ) ;
#35570=CARTESIAN_POINT ( 'NONE',  ( 55.77012379229940819, 12.13428856597101557, -14.42319032175540450 ) ) ;
#35575=CARTESIAN_POINT ( 'NONE',  ( 210.6475357757682332, 114.8748261044495962, 5.289591715120433690 ) ) ;
#35576=CARTESIAN_POINT ( 'NONE',  ( -142.3260422482980516, 59.60034523324940636, 40.45550101730454884 ) ) ;
#35577=CARTESIAN_POINT ( 'NONE',  ( 210.6475357757682332, 114.8748261044495962, 32.13414230558411333 ) ) ;
#35578=FACE_BOUND ( 'NONE', #67494, .T. ) ;
#35585=CARTESIAN_POINT ( 'NONE',  ( -119.1595461276717742, 43.39759378353400621, 88.49148495774751666 ) ) ;
#35587=CARTESIAN_POINT ( 'NONE',  ( -179.5186635612083705, 96.12511541314938768, 15.42972251793390903 ) ) ;
#35589=CARTESIAN_POINT ( 'NONE',  ( 8.469671715138490597, 6.376661621676603886, 92.87585994188762584 ) ) ;
#35593=CARTESIAN_POINT ( 'NONE',  ( 201.9822477997853412, 104.3642793804899895, -50.82886203894460664 ) ) ;
#35597=CARTESIAN_POINT ( 'NONE',  ( -79.62258606008205675, 22.68765733708499255, -76.91402268787508945 ) ) ;
#35599=B_SPLINE_CURVE_WITH_KNOTS ( 'NONE', 3,
 ( #17144, #6957, #48797, #59708, #59367, #7316, #11179, #54077, #60061, #38262, #11881, #49497, #38978, #54428, #22091, #23145, #27354, #55485, #27708, #43875, #34046, #17863 ),
 .UNSPECIFIED., .F., .F.,
 ( 4, 2, 2, 2, 2, 2, 2, 2, 2, 2, 4 ),
 ( 0.000000000000000000, 0.001465307722066868214, 0.002197961583100300695, 0.002930615444133732525, 0.004395923166200650829, 0.005128577027234123425, 0.005861230888267594287, 0.007326538610334516928, 0.008791846332401438702, 0.01025715405446836308, 0.01172246177653528745 ),
 .UNSPECIFIED. ) ;
#35600=ADVANCED_FACE ( 'NONE', ( #60371 ), #43477, .T. ) ;
#35601=VERTEX_POINT ( 'NONE', #33650 ) ;
#35602=VERTEX_POINT ( 'NONE', #932 ) ;
#35603=CARTESIAN_POINT ( 'NONE',  ( 15.29293866748104769, 6.484959508098438796, -35.51894409868578606 ) ) ;
#35607=EDGE_CURVE ( 'NONE', #32410, #9716, #6898, .T. ) ;
#35608=CARTESIAN_POINT ( 'NONE',  ( 106.4072861358879010, 28.24787347451999153, 16.71615381848508974 ) ) ;
#35611=CARTESIAN_POINT ( 'NONE',  ( -24.05175394599741523, 8.494885318775043714, 89.95382958585727806 ) ) ;
#35613=CARTESIAN_POINT ( 'NONE',  ( 174.9161599490640526, 73.97365196673302989, -74.84476842227203974 ) ) ;
#35614=DIRECTION ( 'NONE',  ( -0.000000000000000000, 1.000000000000000000, -0.000000000000000000 ) ) ;
#35616=CARTESIAN_POINT ( 'NONE',  ( -31.43908319763709969, 9.591432048623765638, 30.21645440618916112 ) ) ;
#35618=CARTESIAN_POINT ( 'NONE',  ( -166.2471992823174958, 81.23280767746210529, -92.85267937552322337 ) ) ;
#35622=CARTESIAN_POINT ( 'NONE',  ( 43.14712943604300222, 8.926114770663675202, 17.07187046130982822 ) ) ;
#35623=CARTESIAN_POINT ( 'NONE',  ( 116.8004147899731748, 32.03558746084399189, -93.44768873162850298 ) ) ;
#35627=CARTESIAN_POINT ( 'NONE',  ( 126.5880720616305553, 37.20544379858411332, 12.03288608235020973 ) ) ;
#35629=CARTESIAN_POINT ( 'NONE',  ( 211.6571441797747468, 118.2476110685686592, 87.59423805443044841 ) ) ;
#35630=CARTESIAN_POINT ( 'NONE',  ( 207.4610690199661462, 111.9701171077052209, 43.69190904262227093 ) ) ;
#35634=AXIS2_PLACEMENT_3D ( 'NONE', #64234, #17797, #56457 ) ;
#35636=CARTESIAN_POINT ( 'NONE',  ( 14.08810621383467243, 7.458732232275137264, -23.48329793243775399 ) ) ;
#35638=CARTESIAN_POINT ( 'NONE',  ( 199.3671895066314335, 99.30947926630335587, -22.28159174662976483 ) ) ;
#35640=B_SPLINE_CURVE_WITH_KNOTS ( 'NONE', 3,
 ( #1805, #30516, #51631, #55600, #24902, #46333, #12696, #34162, #7429, #2149, #23604, #9411, #68821, #42781, #20999, #10093, #20642, #42103, #47036, #16057, #37509, #25933, #63563, #31550, #26620, #4134, #21332, #58962, #10777, #36142, #52312, #69171, #3779, #36835, #19971, #57599, #4475, #64249, #20299, #42446, #4809, #30869, #51967, #68494, #15717, #15373 ),
 .UNSPECIFIED., .F., .F.,
 ( 4, 2, 2, 2, 2, 2, 2, 2, 2, 2, 2, 2, 2, 2, 2, 2, 2, 2, 2, 2, 2, 2, 4 ),
 ( 0.02989107162308292723, 0.03170280136394034581, 0.03351453110479776093, 0.03532626084565517605, 0.03713799058651259116, 0.03894972032737000628, 0.03985558519779868608, 0.04076145006822736588, 0.04166731493865603875, 0.04257317980908471855, 0.04347904467951339835, 0.04438490954994207816, 0.04529077442037075796, 0.04619663929079943776, 0.04710250416122811756, 0.04800836903165679737, 0.04891423390208547717, 0.04982009877251415697, 0.05163182851337153045, 0.05344355825422891781, 0.05525528799508629130, 0.05706701773594367866, 0.05887874747680105214 ),
 .UNSPECIFIED. ) ;
#35643=CARTESIAN_POINT ( 'NONE',  ( -168.0003605155415016, 83.06333427281275306, 32.83646999918969556 ) ) ;
#35644=CARTESIAN_POINT ( 'NONE',  ( 33.03621582719332395, 7.666716336587119152, -47.09313870449056338 ) ) ;
#35645=CARTESIAN_POINT ( 'NONE',  ( -106.6940984894958149, 35.07986071359381697, 5.092223517931543597 ) ) ;
#35647=CARTESIAN_POINT ( 'NONE',  ( 10.15118267943872787, 7.391905976536038203, -47.97213281097538129 ) ) ;
#35655=CARTESIAN_POINT ( 'NONE',  ( -29.75049355503753645, 9.320234381800291956, -76.97328196399489286 ) ) ;
#35659=CARTESIAN_POINT ( 'NONE',  ( 173.5837434292114096, 71.34409607026154276, -70.85766065640814304 ) ) ;
#35660=CARTESIAN_POINT ( 'NONE',  ( -180.6213815675304772, 95.88446356933845038, -42.52151308631101756 ) ) ;
#35662=CARTESIAN_POINT ( 'NONE',  ( -171.0758681675585819, 84.87997360100519018, 18.70530542384813089 ) ) ;
#35666=CARTESIAN_POINT ( 'NONE',  ( -47.95193882091086834, 12.89180642785319186, 62.19750565756635297 ) ) ;
#35669=CARTESIAN_POINT ( 'NONE',  ( -98.25600799348289627, 30.78291175898263887, -89.85991034338427141 ) ) ;
#35675=CARTESIAN_POINT ( 'NONE',  ( -102.2801239173131194, 33.91021738430207932, -61.85912785543958847 ) ) ;
#35684=ORIENTED_EDGE ( 'NONE', *, *, #62022, .T. ) ;
#35685=VECTOR ( 'NONE', #68651, 1000.000000000000000 ) ;
#35687=DIRECTION ( 'NONE',  ( -0.8118923937861950435, -0.5838071093367415143, 0.000000000000000000 ) ) ;
#35688=CARTESIAN_POINT ( 'NONE',  ( -178.2427210808090194, 93.01567669683346651, -74.54080329974289043 ) ) ;
#35693=CARTESIAN_POINT ( 'NONE',  ( -5.885876544836658120, 6.772369038004114827, 3.521998547665712742 ) ) ;
#35696=CARTESIAN_POINT ( 'NONE',  ( -78.66644367742109978, 23.39876645725290061, 45.41820113967312977 ) ) ;
#35698=CARTESIAN_POINT ( 'NONE',  ( 150.9203732286581783, 52.73242726514098422, 86.92778406629997789 ) ) ;
#35699=CARTESIAN_POINT ( 'NONE',  ( -190.6985136298602015, 109.1272424661243434, 42.87371446347281534 ) ) ;
#35704=CARTESIAN_POINT ( 'NONE',  ( -71.75757423844133598, 20.87429366976958889, 88.67075130327452825 ) ) ;
#35707=FACE_OUTER_BOUND ( 'NONE', #41897, .T. ) ;
#35713=CARTESIAN_POINT ( 'NONE',  ( 197.3685896092616190, 96.80423329231987850, -72.29383356998032184 ) ) ;
#35715=CARTESIAN_POINT ( 'NONE',  ( -119.2682179969168175, 42.28333404791698769, 68.51757058174662518 ) ) ;
#35718=CARTESIAN_POINT ( 'NONE',  ( 18.66025561752211459, 6.609375019058818523, -23.11559368035124251 ) ) ;
#35719=CARTESIAN_POINT ( 'NONE',  ( -53.13788504024111603, 15.21566150156364472, 30.54986303373576462 ) ) ;
#35724=CARTESIAN_POINT ( 'NONE',  ( 107.9301116202191650, 27.82606182274594175, 56.80549743259531681 ) ) ;
#35727=VECTOR ( 'NONE', #374, 1000.000000000000000 ) ;
#35730=CARTESIAN_POINT ( 'NONE',  ( -142.0050623352988737, 59.34725908986624887, 91.61396122507353823 ) ) ;
#35735=EDGE_CURVE ( 'NONE', #36637, #58864, #12733, .T. ) ;
#35737=CARTESIAN_POINT ( 'NONE',  ( -85.75947274862032543, 25.15128705015479582, 62.27437794546533212 ) ) ;
#35738=CARTESIAN_POINT ( 'NONE',  ( 65.41496713438824884, 13.24164235279044100, -36.09838966426160312 ) ) ;
#35740=CARTESIAN_POINT ( 'NONE',  ( -56.97556689808916985, 16.24958672959845529, 45.07069295579339752 ) ) ;
#35741=CARTESIAN_POINT ( 'NONE',  ( -34.52542994698666945, 11.14027065218090762, -62.82190222610383046 ) ) ;
#35742=CARTESIAN_POINT ( 'NONE',  ( 182.7745872728867766, 81.77554423487161728, 71.01052022670802444 ) ) ;
#35743=CARTESIAN_POINT ( 'NONE',  ( 12.46704290855393005, 6.417105965824391411, -22.90343017382230428 ) ) ;
#35746=CARTESIAN_POINT ( 'NONE',  ( -3.244108878396739559, 6.635632329121487594, -36.95954016693644206 ) ) ;
#35747=CARTESIAN_POINT ( 'NONE',  ( 181.9406741394862195, 79.47484497224793643, 71.11619196314875069 ) ) ;
#35748=CARTESIAN_POINT ( 'NONE',  ( -123.4416615615272548, 44.90042688650404301, 18.36697774316868959 ) ) ;
#35752=CARTESIAN_POINT ( 'NONE',  ( 22.62427395637551086, 7.823784829753561709, -19.26947666278158877 ) ) ;
#35753=CARTESIAN_POINT ( 'NONE',  ( 197.8436586345020487, 97.39326576892285914, 60.45424050539947558 ) ) ;
#35761=CARTESIAN_POINT ( 'NONE',  ( 63.01563776193091826, 12.67277567978498531, -50.72069083216976537 ) ) ;
#35765=CARTESIAN_POINT ( 'NONE',  ( -86.05211524933166345, 25.27371147724188916, -95.00000000000133582 ) ) ;
#35768=AXIS2_PLACEMENT_3D ( 'NONE', #46039, #31262, #67181 ) ;
#35769=CARTESIAN_POINT ( 'NONE',  ( 164.8082524270398608, 64.90614020105162751, 89.03617402024222827 ) ) ;
#35771=CARTESIAN_POINT ( 'NONE',  ( 129.5225439633634323, 40.02995148249140556, -76.50699716606419543 ) ) ;
#35772=CARTESIAN_POINT ( 'NONE',  ( 126.3737790127713083, 37.08609730334948296, 37.58129485337921949 ) ) ;
#35774=CARTESIAN_POINT ( 'NONE',  ( -156.8728827992624701, 72.05711009495561825, 36.77836446409524740 ) ) ;
#35775=CARTESIAN_POINT ( 'NONE',  ( -96.78198318406111866, 30.07417864442865252, 32.89477166860936563 ) ) ;
#35777=CARTESIAN_POINT ( 'NONE',  ( 8.000000000000007105, 249.8719672152120381, 94.99999999999866418 ) ) ;
#35784=CARTESIAN_POINT ( 'NONE',  ( 173.7225111622554437, 72.84868911716897344, 38.27220697509852698 ) ) ;
#35785=CARTESIAN_POINT ( 'NONE',  ( 18.19980344696536534, 6.589834367837007711, -76.96946507082562050 ) ) ;
#35787=ORIENTED_EDGE ( 'NONE', *, *, #19720, .F. ) ;
#35788=CARTESIAN_POINT ( 'NONE',  ( -173.1211646369891355, 88.63826465341151106, -49.71195716475001092 ) ) ;
#35789=FACE_OUTER_BOUND ( 'NONE', #38297, .T. ) ;
#35791=CARTESIAN_POINT ( 'NONE',  ( -62.30463872474475551, 16.74658165105248386, -17.84944043806595815 ) ) ;
#35792=B_SPLINE_CURVE_WITH_KNOTS ( 'NONE', 3,
 ( #66736, #61092, #2016, #28737, #12918, #2699, #39981, #50878, #7974, #18530, #44566, #12557, #61440, #34719, #23113, #23811, #61771, #34373, #56156, #66043, #66394, #29428, #24161, #45603, #12210, #55820, #17836, #39635, #2358, #7641, #45252, #67088, #18877, #39293, #29091, #60737, #40325, #33677 ),
 .UNSPECIFIED., .F., .F.,
 ( 4, 2, 2, 2, 2, 2, 2, 2, 2, 2, 2, 2, 2, 2, 2, 2, 2, 2, 4 ),
 ( 0.02546424207107601811, 0.02703543426729208832, 0.02782103036540015811, 0.02860662646350822791, 0.03017781865972443342, 0.03174901085594063893, 0.03332020305215684791, 0.03489139524837305689, 0.03646258744458925893, 0.03724818354269734955, 0.03803377964080544016, 0.03881937573891353077, 0.03960497183702162138, 0.04117616403323780261, 0.04274735622945398383, 0.04431854842567016506, 0.04588974062188634628, 0.04746093281810252751, 0.05060331721053488302 ),
 .UNSPECIFIED. ) ;
#35793=CARTESIAN_POINT ( 'NONE',  ( 136.9822423813093053, 44.53121110416871176, 30.18860586589651618 ) ) ;
#35794=CARTESIAN_POINT ( 'NONE',  ( 86.62931800182293784, -170.0000000000000000, -70.16611478937539914 ) ) ;
#35795=CARTESIAN_POINT ( 'NONE',  ( -101.8191498210054675, 32.54686850610962523, 3.674523915951419362 ) ) ;
#35796=CARTESIAN_POINT ( 'NONE',  ( 67.54641595172913071, 14.80690682047550943, -64.06872420909932941 ) ) ;
#35799=CARTESIAN_POINT ( 'NONE',  ( 8.485361335568063268, 7.382900357301075189, -95.00000000000133582 ) ) ;
#35806=CARTESIAN_POINT ( 'NONE',  ( 69.48877314113907744, 15.30784187978995092, -39.42461950060443598 ) ) ;
#35808=CARTESIAN_POINT ( 'NONE',  ( 205.0999694062793424, 106.8955893716604777, 56.05227132923311473 ) ) ;
#35811=FACE_OUTER_BOUND ( 'NONE', #8760, .T. ) ;
#35813=CARTESIAN_POINT ( 'NONE',  ( -175.0671597231267924, 89.32002174371487513, -88.64685081530532784 ) ) ;
#35817=CARTESIAN_POINT ( 'NONE',  ( -81.57257563421755719, 23.44953612320489711, -89.37733141453014696 ) ) ;
#35818=CARTESIAN_POINT ( 'NONE',  ( -190.6985136298601731, 109.1272424661242582, 94.99999999999866418 ) ) ;
#35821=CARTESIAN_POINT ( 'NONE',  ( 35.65775178405254309, 7.951994368745593178, 4.066108867012141914 ) ) ;
#35822=CARTESIAN_POINT ( 'NONE',  ( -11.14668121284976721, 8.139398342256733088, -36.18907776356625305 ) ) ;
#35824=VECTOR ( 'NONE', #2231, 1000.000000000000000 ) ;
#35825=ORIENTED_EDGE ( 'NONE', *, *, #22784, .T. ) ;
#35826=CARTESIAN_POINT ( 'NONE',  ( -119.9488317262643875, 43.88555072835348625, -91.50783509519961001 ) ) ;
#35827=ORIENTED_EDGE ( 'NONE', *, *, #5572, .F. ) ;
#35829=CARTESIAN_POINT ( 'NONE',  ( -57.89360529881253825, 16.50663720601370343, 71.61556157776966813 ) ) ;
#35832=CARTESIAN_POINT ( 'NONE',  ( -60.86068608946850844, 16.31596860244180291, -91.65520414832201368 ) ) ;
#35833=CARTESIAN_POINT ( 'NONE',  ( -99.98930671699734773, 31.63190627461931470, -22.82702748219488242 ) ) ;
#35834=CARTESIAN_POINT ( 'NONE',  ( 150.4542242713869484, 53.63744268572192198, -40.96015938328587680 ) ) ;
#35839=CARTESIAN_POINT ( 'NONE',  ( -149.7268278745402199, 65.68859631971237434, 57.56537183036276417 ) ) ;
#35840=CARTESIAN_POINT ( 'NONE',  ( 174.1348882614951208, 73.23561817543357222, -14.04505384645303856 ) ) ;
#35841=CARTESIAN_POINT ( 'NONE',  ( -118.4553071845214731, 41.78724769484929880, 37.02199087950304346 ) ) ;
#35844=CARTESIAN_POINT ( 'NONE',  ( -180.2188652555596491, 96.98354576637422042, -71.49711507050399462 ) ) ;
#35845=CARTESIAN_POINT ( 'NONE',  ( 136.0649627081555195, 43.95772869497660906, 83.52517116066933056 ) ) ;
#35846=CARTESIAN_POINT ( 'NONE',  ( 204.6977192012829505, 108.0580384837234931, -24.48138044215792419 ) ) ;
#35849=EDGE_LOOP ( 'NONE', ( #15499, #60478, #9816, #26241 ) ) ;
#35851=CARTESIAN_POINT ( 'NONE',  ( 112.1012908502484748, 29.75117929736502020, -77.53697030799570200 ) ) ;
#35852=CARTESIAN_POINT ( 'NONE',  ( 188.5838389098763344, 88.03667982118679447, 37.11779938872467000 ) ) ;
#35853=CARTESIAN_POINT ( 'NONE',  ( 183.8564736226039713, 81.45095818237477658, -90.40950570902288064 ) ) ;
#35856=VERTEX_POINT ( 'NONE', #52910 ) ;
#35857=CARTESIAN_POINT ( 'NONE',  ( 164.4761273435911733, 64.62485394454741083, -19.50930807920846632 ) ) ;
#35859=CARTESIAN_POINT ( 'NONE',  ( 66.94365390260638549, 14.65531706601758977, 57.76378685776548849 ) ) ;
#35860=CARTESIAN_POINT ( 'NONE',  ( 141.2963039856138039, 46.10182040858772723, 89.73232225052716160 ) ) ;
#35864=CARTESIAN_POINT ( 'NONE',  ( 161.1112535418156710, 61.83422628788724751, -37.06319131123839128 ) ) ;
#35869=CARTESIAN_POINT ( 'NONE',  ( -94.77890319529974761, 30.24118571794803501, 10.67444691552502256 ) ) ;
#35870=CARTESIAN_POINT ( 'NONE',  ( -131.7724154034330581, 50.48821165954357326, 42.78414996048509522 ) ) ;
#35871=CARTESIAN_POINT ( 'NONE',  ( 153.9458454029195877, 56.21976558811522295, -90.68237876674034226 ) ) ;
#35872=CARTESIAN_POINT ( 'NONE',  ( 82.73618382051371611, 19.18661415186667440, -10.06194520202119591 ) ) ;
#35873=CARTESIAN_POINT ( 'NONE',  ( -166.5704851812740515, 80.12110537694670143, 34.65906088291280440 ) ) ;
#35874=CARTESIAN_POINT ( 'NONE',  ( 63.01563776193091826, 13.70579113808094895, 29.81296093922127710 ) ) ;
#35875=CARTESIAN_POINT ( 'NONE',  ( 210.6189312023034574, -170.0000000000000000, 94.99999999999866418 ) ) ;
#35877=CARTESIAN_POINT ( 'NONE',  ( 181.0840389613909736, 78.60582251573003987, 29.30859410551139277 ) ) ;
#35878=CARTESIAN_POINT ( 'NONE',  ( 150.3360255159550150, 52.31024849487489803, -95.00000000000133582 ) ) ;
#35879=EDGE_LOOP ( 'NONE', ( #1770, #16887, #27927, #59793 ) ) ;
#35883=CARTESIAN_POINT ( 'NONE',  ( 212.1976655298228991, 119.0878071902807704, -17.15924209720097693 ) ) ;
#35884=CARTESIAN_POINT ( 'NONE',  ( 106.4072861358878441, 28.24787347451998443, 43.56070440894875873 ) ) ;
#35887=CARTESIAN_POINT ( 'NONE',  ( 188.4918087359956473, 87.93403732562656216, 8.752912527378605034 ) ) ;
#35888=CARTESIAN_POINT ( 'NONE',  ( 211.7451286015361518, 116.5372661580811666, -41.24269329785643379 ) ) ;
#35890=DIRECTION ( 'NONE',  ( -0.000000000000000000, 1.000000000000000000, -0.000000000000000000 ) ) ;
#35891=ORIENTED_EDGE ( 'NONE', *, *, #64793, .F. ) ;
#35894=VERTEX_POINT ( 'NONE', #65936 ) ;
#35895=CARTESIAN_POINT ( 'NONE',  ( 106.4107271020439782, 27.14892220304137993, -76.71846769895172713 ) ) ;
#35897=CARTESIAN_POINT ( 'NONE',  ( 41.80869235728138733, 9.750404582811606602, -23.39550270451861635 ) ) ;
#35903=CARTESIAN_POINT ( 'NONE',  ( -109.7686203588201579, 37.90089348911613598, -15.17831855726085521 ) ) ;
#35905=CARTESIAN_POINT ( 'NONE',  ( -71.43874587651176000, 19.69883891272895937, 62.74430205168221875 ) ) ;
#35906=CARTESIAN_POINT ( 'NONE',  ( -167.1540252468941503, 80.72321878831101571, 60.61552501969690354 ) ) ;
#35907=ORIENTED_EDGE ( 'NONE', *, *, #13682, .T. ) ;
#35909=CARTESIAN_POINT ( 'NONE',  ( -156.1462053606562677, 70.02140399657017156, 41.72074378258265881 ) ) ;
#35911=B_SPLINE_CURVE_WITH_KNOTS ( 'NONE', 3,
 ( #47564, #59501, #5694, #63422, #26475, #42646, #11315, #15913, #69020, #10280, #52511, #4338, #27152, #5361, #31745, #21874, #16599, #53182, #75, #48583 ),
 .UNSPECIFIED., .F., .F.,
 ( 4, 2, 2, 2, 2, 2, 2, 2, 2, 4 ),
 ( 0.009941967776246129346, 0.01118871530018490136, 0.01243546282412367338, 0.01305883658609307066, 0.01368221034806246968, 0.01492895787200121047, 0.01617570539593995299, 0.01742245291987869205, 0.01866920044381743110, 0.01991594796775617363 ),
 .UNSPECIFIED. ) ;
#35912=CARTESIAN_POINT ( 'NONE',  ( 175.5493994043409316, 73.18740965572600032, -11.81303265696679183 ) ) ;
#35919=LINE ( 'NONE', #57369, #33412 ) ;
#35920=ORIENTED_EDGE ( 'NONE', *, *, #55101, .F. ) ;
#35921=CARTESIAN_POINT ( 'NONE',  ( 212.0047492081760083, 116.9348962082588343, 8.142182148364424776 ) ) ;
#35922=CARTESIAN_POINT ( 'NONE',  ( -148.6426892915312123, 64.76241938621078020, 45.72082123989908098 ) ) ;
#35923=CARTESIAN_POINT ( 'NONE',  ( 210.4897348480408539, 114.6382060222044714, 31.93660676264083165 ) ) ;
#35924=FACE_BOUND ( 'NONE', #59442, .T. ) ;
#35928=CARTESIAN_POINT ( 'NONE',  ( -118.7786458613889806, 43.16353039193077734, 89.41427216433091019 ) ) ;
#35929=CARTESIAN_POINT ( 'NONE',  ( -165.7143741370936993, 79.24519349471958662, -16.58517908087970838 ) ) ;
#35931=CARTESIAN_POINT ( 'NONE',  ( 23.17475323415827404, 6.849528528214888112, 92.54444823000328313 ) ) ;
#35933=CARTESIAN_POINT ( 'NONE',  ( 86.62931800182293784, 19.42108912189596381, -77.66611478937542756 ) ) ;
#35934=ORIENTED_EDGE ( 'NONE', *, *, #20198, .T. ) ;
#35935=CYLINDRICAL_SURFACE ( 'NONE', #20195, 7.500000000000020428 ) ;
#35936=CARTESIAN_POINT ( 'NONE',  ( -99.97541017369792371, 31.62502926470686759, 72.01622551138805761 ) ) ;
#35938=CARTESIAN_POINT ( 'NONE',  ( -85.45399718454960691, 25.02415453493131281, 14.27398530813207245 ) ) ;
#35941=ORIENTED_EDGE ( 'NONE', *, *, #8041, .T. ) ;
#35942=EDGE_LOOP ( 'NONE', ( #54693, #12245, #50580, #48959 ) ) ;
#35943=CARTESIAN_POINT ( 'NONE',  ( 43.96421756700840433, 10.06386361114659778, 58.28564946010243375 ) ) ;
#35944=VECTOR ( 'NONE', #7534, 1000.000000000000000 ) ;
#35945=CARTESIAN_POINT ( 'NONE',  ( -106.6624114166473305, 36.20432260969276683, -90.10160425761682745 ) ) ;
#35946=CARTESIAN_POINT ( 'NONE',  ( 105.7953515382196628, 27.97683113100024244, 16.32495411353482595 ) ) ;
#35949=CARTESIAN_POINT ( 'NONE',  ( -24.07560883032475729, 8.498111648314747413, 92.86635853022728782 ) ) ;
#35950=CARTESIAN_POINT ( 'NONE',  ( 173.9405361758639117, 73.05302209498820787, -68.26724894106142472 ) ) ;
#35952=CARTESIAN_POINT ( 'NONE',  ( 110.2429982417149290, 28.88204397445231209, -50.92243756565370916 ) ) ;
#35954=LINE ( 'NONE', #57406, #33269 ) ;
#35956=B_SPLINE_CURVE_WITH_KNOTS ( 'NONE', 3,
 ( #28497, #60503, #45014, #55929, #50305, #12667, #44315, #12319, #60847, #49940, #34132, #40096, #1771, #13367, #56264, #65799, #29195, #23235, #7746, #44679, #8080, #66155, #17947, #2463, #28854, #2122, #23574, #18288, #5502, #54368, #48057, #26955, #6196, #37862, #5160, #32928, #22029, #43817, #927, #54726, #10428, #16746, #38204 ),
 .UNSPECIFIED., .F., .F.,
 ( 4, 2, 2, 2, 2, 2, 2, 2, 1, 2, 2, 2, 2, 2, 2, 2, 2, 2, 2, 2, 2, 4 ),
 ( 0.000000000000000000, 0.001465684626643319350, 0.002198526939964978808, 0.002931369253286638700, 0.004397053879929970627, 0.005862738506573303421, 0.007328423133216635348, 0.008061265446538309551, 0.008794107759859986356, 0.009526950073181661427, 0.01025979238650333650, 0.01172547701314670572, 0.01319116163979007321, 0.01465684626643344417, 0.01538968857975512618, 0.01612253089307680992, 0.01758821551972015659, 0.01905390014636350327, 0.01978674245968517140, 0.02051958477300683606, 0.02198526939965016885, 0.02345095402629350512 ),
 .UNSPECIFIED. ) ;
#35958=ORIENTED_EDGE ( 'NONE', *, *, #30497, .F. ) ;
#35960=CARTESIAN_POINT ( 'NONE',  ( -85.96384504792887071, 26.32782846176032976, -67.71012703438472613 ) ) ;
#35961=CARTESIAN_POINT ( 'NONE',  ( 175.0634607207819045, 74.11351956991636314, 14.44380243719841594 ) ) ;
#35963=CARTESIAN_POINT ( 'NONE',  ( -102.2801239173131052, 32.78103895658057354, -88.70367844590326456 ) ) ;
#35964=CARTESIAN_POINT ( 'NONE',  ( 127.2397149628677369, 37.56999625068102233, 13.73394111055298339 ) ) ;
#35965=CARTESIAN_POINT ( 'NONE',  ( 32.69830313199977212, 7.632043626524796842, -93.43925476920368567 ) ) ;
#35966=CARTESIAN_POINT ( 'NONE',  ( -124.1095621208148572, 46.52671329146387080, -61.91586655676568540 ) ) ;
#35968=CARTESIAN_POINT ( 'NONE',  ( 205.5049354810107332, 109.1776577097391510, 29.20772073876942088 ) ) ;
#35969=LINE ( 'NONE', #67641, #46762 ) ;
#35970=CARTESIAN_POINT ( 'NONE',  ( -108.9452487746634120, 36.29752968355630571, 34.54237325803290304 ) ) ;
#35971=ORIENTED_EDGE ( 'NONE', *, *, #55401, .F. ) ;
#35972=CARTESIAN_POINT ( 'NONE',  ( 15.29912143387263690, 7.491799981865496783, -23.67439350822212774 ) ) ;
#35975=B_SPLINE_CURVE_WITH_KNOTS ( 'NONE', 3,
 ( #35799, #56910, #51630, #57598, #9410, #30177, #30514, #39091, #44341, #8379 ),
 .UNSPECIFIED., .F., .F.,
 ( 4, 2, 2, 2, 4 ),
 ( 0.000000000000000000, 0.002502989122560414677, 0.005005978245120829354, 0.007508967367681244030, 0.01001195649024165871 ),
 .UNSPECIFIED. ) ;
#35977=CARTESIAN_POINT ( 'NONE',  ( -149.5074843970971017, 65.50121172469319220, 3.876270649435370252 ) ) ;
#35983=CARTESIAN_POINT ( 'NONE',  ( 139.2794027252094224, 45.99190465195510313, -38.31979582468038359 ) ) ;
#35984=CARTESIAN_POINT ( 'NONE',  ( 32.67604581760323867, 7.629767527669977234, -39.79224508708363572 ) ) ;
#35985=CARTESIAN_POINT ( 'NONE',  ( 203.9150235420940476, 105.2750102756484978, 82.91810571397343210 ) ) ;
#35986=CARTESIAN_POINT ( 'NONE',  ( 13.37708032728285268, 7.441924986912761497, -50.12502757588696767 ) ) ;
#35987=CARTESIAN_POINT ( 'NONE',  ( 126.8237978310704506, 37.33705012421152958, -40.90458718104599001 ) ) ;
#35992=CARTESIAN_POINT ( 'NONE',  ( -23.93965512371324422, 8.480096402797089539, -70.16679352128214475 ) ) ;
#35993=EDGE_CURVE ( 'NONE', #57471, #988, #44087, .T. ) ;
#35997=CARTESIAN_POINT ( 'NONE',  ( 8.683531412707425901, 6.377173148747123044, 13.08527713931978198 ) ) ;
#36002=CARTESIAN_POINT ( 'NONE',  ( 179.4279766878530040, 76.94722012158230484, -77.89655909951385127 ) ) ;
#36005=CARTESIAN_POINT ( 'NONE',  ( -28.35957743809533937, 10.12373109553626804, 57.71800868584409017 ) ) ;
#36006=DIRECTION ( 'NONE',  ( 0.000000000000000000, 0.000000000000000000, 1.000000000000000000 ) ) ;
#36007=CARTESIAN_POINT ( 'NONE',  ( -47.60396279792517760, 12.80997843568595052, 63.65564769673237322 ) ) ;
#36010=CARTESIAN_POINT ( 'NONE',  ( 150.5744176759382640, 53.72473166688032364, 60.79328936379504000 ) ) ;
#36011=CARTESIAN_POINT ( 'NONE',  ( -109.6657532478350845, 37.84376708859253569, -70.68994547012663077 ) ) ;
#36013=CARTESIAN_POINT ( 'NONE',  ( -102.2801239173131194, 32.78103895658057354, -35.01457726497591239 ) ) ;
#36014=DIRECTION ( 'NONE',  ( 1.000000000000000000, 0.000000000000000000, -0.000000000000000000 ) ) ;
#36021=CARTESIAN_POINT ( 'NONE',  ( -180.2244609727084992, 95.39945930389644957, -71.48059130514354820 ) ) ;
#36030=CARTESIAN_POINT ( 'NONE',  ( -24.18270484670772902, 9.527492911955588895, -14.01251953149264473 ) ) ;
#36031=CARTESIAN_POINT ( 'NONE',  ( 141.3445468829084746, 46.13338528906588465, 10.66957849498047928 ) ) ;
#36035=ORIENTED_EDGE ( 'NONE', *, *, #58048, .T. ) ;
#36037=EDGE_CURVE ( 'NONE', #33721, #48827, #53810, .T. ) ;
#36038=CARTESIAN_POINT ( 'NONE',  ( 9.827939172326074058, 6.382931149346556587, 68.93830584714513066 ) ) ;
#36039=CARTESIAN_POINT ( 'NONE',  ( 157.4703587214989398, -170.0000000000000000, -62.96873488960130771 ) ) ;
#36040=CARTESIAN_POINT ( 'NONE',  ( 200.8383807319521281, 102.8517715783673339, 30.26259293534468497 ) ) ;
#36043=ORIENTED_EDGE ( 'NONE', *, *, #59298, .F. ) ;
#36044=CARTESIAN_POINT ( 'NONE',  ( 70.11969827741708627, 15.47408882293423993, 39.76769945686178431 ) ) ;
#36048=CARTESIAN_POINT ( 'NONE',  ( 110.7117404013330884, 30.20916032354562830, -77.76698815611739235 ) ) ;
#36052=CARTESIAN_POINT ( 'NONE',  ( -38.69449158134467126, 11.92067517118076125, 62.59844393972618803 ) ) ;
#36054=LINE ( 'NONE', #63130, #17436 ) ;
#36056=CYLINDRICAL_SURFACE ( 'NONE', #14025, 7.500000000000014211 ) ;
#36057=CARTESIAN_POINT ( 'NONE',  ( -50.14523569787233725, 14.45648954445650602, 32.12416558293933377 ) ) ;
#36063=CARTESIAN_POINT ( 'NONE',  ( 102.8816949008297712, 25.62288855336258564, 89.32272773285413336 ) ) ;
#36066=CARTESIAN_POINT ( 'NONE',  ( 183.3913492984168556, 80.96922346472079823, -50.86455848634233945 ) ) ;
#36068=CARTESIAN_POINT ( 'NONE',  ( 164.9534461562627428, 63.71129898458564611, -71.04616183406005803 ) ) ;
#36073=CARTESIAN_POINT ( 'NONE',  ( -79.62258606008208517, 22.68765733708499965, 57.30873026444331231 ) ) ;
#36077=VECTOR ( 'NONE', #20769, 1000.000000000000000 ) ;
#36078=CARTESIAN_POINT ( 'NONE',  ( -33.36965723649376514, 10.93726715887721390, -76.91312719118394625 ) ) ;
#36082=CARTESIAN_POINT ( 'NONE',  ( 187.8965227056807521, 87.27289477191499145, 66.80197625647082305 ) ) ;
#36083=CARTESIAN_POINT ( 'NONE',  ( 13.37820144534468625, 6.435512790162279728, -9.067908514598384428 ) ) ;
#36086=CARTESIAN_POINT ( 'NONE',  ( 19.10949903373832015, 7.636938177523838078, 3.941116430307622487 ) ) ;
#36087=CARTESIAN_POINT ( 'NONE',  ( 183.1910712700538681, 80.76073941711165105, 70.86391971262702327 ) ) ;
#36090=CARTESIAN_POINT ( 'NONE',  ( 132.7179291807801746, 40.74118679001691845, -24.09532512744151589 ) ) ;
#36091=CARTESIAN_POINT ( 'NONE',  ( 21.44191228441539465, 7.755009954762318358, -21.12731977189180199 ) ) ;
#36092=CARTESIAN_POINT ( 'NONE',  ( 200.4559562755961224, 100.7034888016685272, 57.34971855850135825 ) ) ;
#36096=LINE ( 'NONE', #64193, #22606 ) ;
#36100=DIRECTION ( 'NONE',  ( -0.000000000000000000, 1.000000000000000000, -0.000000000000000000 ) ) ;
#36101=CARTESIAN_POINT ( 'NONE',  ( -109.4995148930278219, 37.75156937139181679, -44.61333367425208252 ) ) ;
#36103=CARTESIAN_POINT ( 'NONE',  ( 185.5412249395995730, 84.70425786166002524, -49.76124368019702615 ) ) ;
#36109=CARTESIAN_POINT ( 'NONE',  ( 111.8699272271189358, 29.64190505307780299, 56.63057503623819144 ) ) ;
#36111=CARTESIAN_POINT ( 'NONE',  ( 126.4633682455862100, 38.28837286275648211, -69.07996067011775665 ) ) ;
#36112=CARTESIAN_POINT ( 'NONE',  ( 126.5710838895481913, 37.19597237024179748, 35.21041822320580650 ) ) ;
#36114=CARTESIAN_POINT ( 'NONE',  ( -95.05546640093039912, 29.25972325950978359, 35.93932265320741948 ) ) ;
#36121=CARTESIAN_POINT ( 'NONE',  ( -168.7329347389695613, 83.83901812802758968, 5.376343091447946421 ) ) ;
#36123=CARTESIAN_POINT ( 'NONE',  ( -145.9181947914994737, 62.49417193455357733, -35.72346211350654954 ) ) ;
#36124=CARTESIAN_POINT ( 'NONE',  ( -133.2787743207940707, 52.78950725740544669, 66.30037897548639592 ) ) ;
#36129=EDGE_LOOP ( 'NONE', ( #362, #30030, #10684, #57565 ) ) ;
#36131=CARTESIAN_POINT ( 'NONE',  ( -60.65612136648952912, 16.25551606627059442, -10.86259259823188472 ) ) ;
#36133=CARTESIAN_POINT ( 'NONE',  ( -133.3799602664182089, 52.86209125874979264, -68.72809787019492944 ) ) ;
#36136=CARTESIAN_POINT ( 'NONE',  ( 65.40383840050415643, 14.27443447873227633, -77.19146956980890195 ) ) ;
#36139=ORIENTED_EDGE ( 'NONE', *, *, #57432, .F. ) ;
#36140=CARTESIAN_POINT ( 'NONE',  ( -147.1538409485623049, 63.51600817366544049, -22.59291464346527434 ) ) ;
#36142=CARTESIAN_POINT ( 'NONE',  ( -166.2028657618940883, 79.74389853943291939, -39.30140056895983491 ) ) ;
#36143=CARTESIAN_POINT ( 'NONE',  ( -55.05276343752909440, 15.72344139423349141, -35.21632399845986328 ) ) ;
#36144=B_SPLINE_CURVE_WITH_KNOTS ( 'NONE', 3,
 ( #66384, #45940, #13586, #30122, #66724, #8318, #61430, #35047, #24151, #50869, #2348, #12548, #56147, #18868, #29083, #18176, #29420, #44557, #39626, #34008, #61082, #13929, #7276, #55447, #34710, #56489, #50529, #66036, #29763, #12909, #51225, #67406, #19197, #13250, #40658, #35391, #56850, #23801, #8667, #17828, #52593, #46627, #25194, #68102, #31492, #20240, #14621, #63501, #42388, #57195, #41013, #14958, #9697, #30807, #53268 ),
 .UNSPECIFIED., .F., .F.,
 ( 4, 2, 2, 2, 2, 2, 2, 2, 2, 2, 2, 2, 1, 2, 2, 2, 2, 2, 2, 2, 2, 2, 2, 2, 2, 2, 2, 4 ),
 ( 0.000000000000000000, 0.001981718938158233759, 0.002972578407237350638, 0.003963437876316467517, 0.004954297345395584397, 0.005945156814474701276, 0.006936016283553818156, 0.007926875752632935035, 0.009908594690791121956, 0.01089945415987021021, 0.01189031362894929673, 0.01288117309802838326, 0.01387203256710746978, 0.01486289203618655803, 0.01585375150526564456, 0.01684461097434472934, 0.01783547044342381413, 0.01981718938158197676, 0.02080804885066105808, 0.02179890831974014287, 0.02278976778881922419, 0.02378062725789830550, 0.02477148672697738682, 0.02576234619605646814, 0.02774406513421459261, 0.02972578407237271708, 0.03071664354145177758, 0.03170750301053083808 ),
 .UNSPECIFIED. ) ;
#36146=CARTESIAN_POINT ( 'NONE',  ( -72.21947956767111521, 21.03570528348186741, 34.07763384368087856 ) ) ;
#36148=CARTESIAN_POINT ( 'NONE',  ( 65.62985354949972816, 14.32996029952553485, -36.18682722834029875 ) ) ;
#36149=LINE ( 'NONE', #31226, #11503 ) ;
#36150=CARTESIAN_POINT ( 'NONE',  ( -167.9853834315979952, 81.58767916550901589, -63.57040599627210042 ) ) ;
#36151=VERTEX_POINT ( 'NONE', #34617 ) ;
#36153=ORIENTED_EDGE ( 'NONE', *, *, #18653, .T. ) ;
#36158=CARTESIAN_POINT ( 'NONE',  ( 33.77444274891858811, 8.756048688386675494, 5.605216617422771108 ) ) ;
#36160=CARTESIAN_POINT ( 'NONE',  ( 34.45817031441433897, 7.817703378455677310, 4.907621799910686811 ) ) ;
#36161=CARTESIAN_POINT ( 'NONE',  ( -12.78319349481551015, 8.274445259016799170, -37.26919679932123586 ) ) ;
#36162=CARTESIAN_POINT ( 'NONE',  ( -31.92572261726338922, 10.69135962481465363, -23.47264677473819816 ) ) ;
#36165=CARTESIAN_POINT ( 'NONE',  ( -121.3890712762008235, 44.78736737435725246, -90.10228078854700584 ) ) ;
#36168=CARTESIAN_POINT ( 'NONE',  ( 8.287863202055541834, 7.382585476140732794, -69.37525033522064177 ) ) ;
#36169=CARTESIAN_POINT ( 'NONE',  ( -31.43908319763709969, 9.591432048623765638, 3.371903815725488585 ) ) ;
#36170=ADVANCED_FACE ( 'NONE', ( #35294 ), #30017, .F. ) ;
#36172=CARTESIAN_POINT ( 'NONE',  ( -14.66033866466834823, 7.432913330382392658, -72.86005857283349485 ) ) ;
#36175=CARTESIAN_POINT ( 'NONE',  ( 153.2523375521184335, 55.69936538551847605, -49.83022819104369461 ) ) ;
#36177=AXIS2_PLACEMENT_3D ( 'NONE', #10214, #43951, #5628 ) ;
#36180=CARTESIAN_POINT ( 'NONE',  ( 179.4074606910091632, 78.34362448405030932, -9.519745835405062806 ) ) ;
#36181=CARTESIAN_POINT ( 'NONE',  ( -106.7004823116342180, 36.22460663120045865, 70.94159824621738153 ) ) ;
#36186=CARTESIAN_POINT ( 'NONE',  ( -0.5751131641471360911, 6.527254166626917709, -14.13863482346338429 ) ) ;
#36187=CARTESIAN_POINT ( 'NONE',  ( 116.8937673311172887, 32.08228998570056945, 33.63549503582235900 ) ) ;
#36189=LINE ( 'NONE', #57647, #68756 ) ;
#36190=CARTESIAN_POINT ( 'NONE',  ( -119.2682179969168601, 42.28333404791700900, -65.70518237057183342 ) ) ;
#36193=CYLINDRICAL_SURFACE ( 'NONE', #13217, 7.500000000000020428 ) ;
#36194=CARTESIAN_POINT ( 'NONE',  ( 117.3281529665582354, 32.29994712002883972, -67.75427984652691293 ) ) ;
#36196=CARTESIAN_POINT ( 'NONE',  ( 181.7896739982670908, 79.32116015393873454, -89.93903081948376155 ) ) ;
#36203=ORIENTED_EDGE ( 'NONE', *, *, #16814, .T. ) ;
#36204=CARTESIAN_POINT ( 'NONE',  ( -78.66644367742111399, 22.32174330031318021, -23.27090004125422595 ) ) ;
#36206=CARTESIAN_POINT ( 'NONE',  ( 140.4959942426281998, 45.58042999908606419, 87.19380765129805866 ) ) ;
#36209=DIRECTION ( 'NONE',  ( -0.000000000000000000, 1.000000000000000000, -0.000000000000000000 ) ) ;
#36216=ORIENTED_EDGE ( 'NONE', *, *, #15027, .T. ) ;
#36218=CARTESIAN_POINT ( 'NONE',  ( -176.1917263072137416, 92.15415277106538383, -89.04606407215415231 ) ) ;
#36219=CARTESIAN_POINT ( 'NONE',  ( 154.0293889979057269, 55.02370422818216866, 57.07356254584302491 ) ) ;
#36220=EDGE_CURVE ( 'NONE', #44581, #40831, #5938, .T. ) ;
#36225=ORIENTED_EDGE ( 'NONE', *, *, #36532, .F. ) ;
#36227=CARTESIAN_POINT ( 'NONE',  ( 150.0980941434704334, 53.37942190380060481, -18.18456334522878848 ) ) ;
#36228=CARTESIAN_POINT ( 'NONE',  ( -56.63808869004000712, 15.11210435325983070, 84.16920984612842460 ) ) ;
#36229=CARTESIAN_POINT ( 'NONE',  ( 8.000000000000007105, 249.8719672152120381, -95.00000000000133582 ) ) ;
#36231=CARTESIAN_POINT ( 'NONE',  ( -152.9121563765244218, 67.12206067149023170, -62.47090493325013227 ) ) ;
#36234=CARTESIAN_POINT ( 'NONE',  ( 210.6741002223296846, 114.9147155784838503, -39.28712141022325710 ) ) ;
#36236=CARTESIAN_POINT ( 'NONE',  ( 180.6710448012268273, 78.18844465372403363, 2.464043515047717570 ) ) ;
#36237=VERTEX_POINT ( 'NONE', #27051 ) ;
#36239=ORIENTED_EDGE ( 'NONE', *, *, #5767, .F. ) ;
#36240=CARTESIAN_POINT ( 'NONE',  ( -72.78270026377325053, 21.23376443558120741, 69.44000555021129628 ) ) ;
#36241=CARTESIAN_POINT ( 'NONE',  ( 56.53635105806416306, 11.26263375223564012, -73.85080886644499287 ) ) ;
#36244=CARTESIAN_POINT ( 'NONE',  ( 19.11382977197791178, 7.636807742668411336, 44.25505563586381896 ) ) ;
#36245=CARTESIAN_POINT ( 'NONE',  ( -108.0902552660050446, 36.97681740369922210, -20.43870904558432855 ) ) ;
#36247=CARTESIAN_POINT ( 'NONE',  ( -71.16584859396992613, 19.60484997908768179, 64.99771648647357836 ) ) ;
#36251=EDGE_LOOP ( 'NONE', ( #46132, #46123, #56314, #17769 ) ) ;
#36252=CARTESIAN_POINT ( 'NONE',  ( -151.6716822472524200, 66.03661194063731443, 31.02609834145020429 ) ) ;
#36254=CARTESIAN_POINT ( 'NONE',  ( 173.9413349464226428, 71.67637800842355489, -19.18543995565300975 ) ) ;
#36257=CARTESIAN_POINT ( 'NONE',  ( -142.0902782307734924, 58.13494170556000995, 10.22982670401919947 ) ) ;
#36261=CARTESIAN_POINT ( 'NONE',  ( 212.1983751099433562, 117.2326047784727336, 10.00450108283069639 ) ) ;
#36262=CARTESIAN_POINT ( 'NONE',  ( -144.3939084932121091, 61.25241660819418144, 43.71263044045074508 ) ) ;
#36264=CARTESIAN_POINT ( 'NONE',  ( 9.934517078398117818, 6.383749116521619804, -92.00087700128223389 ) ) ;
#36268=CARTESIAN_POINT ( 'NONE',  ( -128.7374182412640664, 49.61100189511262926, 84.84501753385171696 ) ) ;
#36270=CARTESIAN_POINT ( 'NONE',  ( 157.4703587214989398, -170.0000000000000000, 90.59856865318074881 ) ) ;
#36271=DIRECTION ( 'NONE',  ( -0.000000000000000000, 1.000000000000000000, -0.000000000000000000 ) ) ;
#36272=CARTESIAN_POINT ( 'NONE',  ( 22.42430175529976211, 6.803777996989659904, 94.71421917802801715 ) ) ;
#36273=CARTESIAN_POINT ( 'NONE',  ( 82.13067365723604496, 17.93447087949267527, -76.18668206738985305 ) ) ;
#36274=EDGE_CURVE ( 'NONE', #55797, #45282, #62174, .T. ) ;
#36280=CARTESIAN_POINT ( 'NONE',  ( 204.6977192012829789, 108.0580384837234789, -36.32593103262158252 ) ) ;
#36281=ADVANCED_FACE ( 'NONE', ( #26977 ), #6214, .F. ) ;
#36284=CARTESIAN_POINT ( 'NONE',  ( -78.66644367742111399, 22.32174330031319798, 18.57365054920947500 ) ) ;
#36291=VECTOR ( 'NONE', #67644, 1000.000000000000000 ) ;
#36293=CARTESIAN_POINT ( 'NONE',  ( 8.528421445032398296, 6.376778749352038922, -44.96446147396655846 ) ) ;
#36295=CARTESIAN_POINT ( 'NONE',  ( 129.5193594945039308, 38.86618897895345270, 69.99177176951431534 ) ) ;
#36296=VERTEX_POINT ( 'NONE', #17104 ) ;
#36297=CARTESIAN_POINT ( 'NONE',  ( -38.90396040047801307, 10.93641556689195049, 90.61005997619054142 ) ) ;
#36298=CARTESIAN_POINT ( 'NONE',  ( 181.0840389613909736, 80.03940679743418229, -63.06960825634327961 ) ) ;
#36301=CARTESIAN_POINT ( 'NONE',  ( 106.4107271020440209, 27.14892220304137282, -49.87391710848807946 ) ) ;
#36302=CARTESIAN_POINT ( 'NONE',  ( 79.63513233364427890, 18.20496177163926177, -46.04061524578445130 ) ) ;
#36307=CARTESIAN_POINT ( 'NONE',  ( -86.16504208171677703, 26.41251233979377133, -69.98968484780580468 ) ) ;
#36310=CARTESIAN_POINT ( 'NONE',  ( -190.6985136298602015, 109.1272424661243434, -10.81538671745452795 ) ) ;
#36311=CARTESIAN_POINT ( 'NONE',  ( 126.8947007444828614, 37.37669340849690514, 7.364425276940866461 ) ) ;
#36312=CARTESIAN_POINT ( 'NONE',  ( -156.8764584803561775, 70.69066846313522490, 9.952307344159024183 ) ) ;
#36314=CARTESIAN_POINT ( 'NONE',  ( 211.5034924207027700, 118.0100795718635425, 39.87353999634708401 ) ) ;
#36316=CARTESIAN_POINT ( 'NONE',  ( -103.2129897037411013, 33.25684593987700310, 45.47526677688482266 ) ) ;
#36319=CARTESIAN_POINT ( 'NONE',  ( -47.60153151963581308, 13.84303696664763095, 90.59163266529853331 ) ) ;
#36322=ORIENTED_EDGE ( 'NONE', *, *, #22874, .F. ) ;
#36323=FACE_OUTER_BOUND ( 'NONE', #11363, .T. ) ;
#36327=CARTESIAN_POINT ( 'NONE',  ( 137.6104751318277124, 44.92718313329109492, -50.02061863167904932 ) ) ;
#36328=CARTESIAN_POINT ( 'NONE',  ( -30.46002654261639009, 10.45132580906817665, 3.420144955256299468 ) ) ;
#36330=CARTESIAN_POINT ( 'NONE',  ( 11.21312910819262854, 7.403355431336990478, -48.98232984902662679 ) ) ;
#36332=CARTESIAN_POINT ( 'NONE',  ( -119.2949674747224975, 43.48097822533564738, -11.96626569522580574 ) ) ;
#36334=AXIS2_PLACEMENT_3D ( 'NONE', #46785, #58033, #30274 ) ;
#36337=CARTESIAN_POINT ( 'NONE',  ( 174.1571680927775105, 73.25653429923636395, 93.39935691738303092 ) ) ;
#36339=CARTESIAN_POINT ( 'NONE',  ( -24.94151142167917001, 8.614613465433004436, -73.43986976775646269 ) ) ;
#36341=CARTESIAN_POINT ( 'NONE',  ( 9.823983574062875590, 6.382904402091123863, 6.096740015399423562 ) ) ;
#36342=CARTESIAN_POINT ( 'NONE',  ( 43.14565945994675644, 9.942782559600564340, -76.46782334873067555 ) ) ;
#36346=CARTESIAN_POINT ( 'NONE',  ( -179.2177980985565284, 94.18084789436638005, -46.58799062249927658 ) ) ;
#36348=CARTESIAN_POINT ( 'NONE',  ( -28.13128612339710344, 10.08889185338653149, 71.30996116462026180 ) ) ;
#36350=CARTESIAN_POINT ( 'NONE',  ( -52.45215874217871743, 13.99961488531757148, 57.62305164748294573 ) ) ;
#36355=CARTESIAN_POINT ( 'NONE',  ( -109.6752351740181979, 37.84903014964773860, -68.08238526816469971 ) ) ;
#36361=LINE ( 'NONE', #42996, #29351 ) ;
#36366=CARTESIAN_POINT ( 'NONE',  ( 42.60194873408148908, 9.863670188337772871, 84.31185681664037190 ) ) ;
#36367=CARTESIAN_POINT ( 'NONE',  ( -173.1211646369891355, 87.12891641440857882, -76.55650775521370122 ) ) ;
#36374=CARTESIAN_POINT ( 'NONE',  ( 57.57684776206770749, 12.50442334002048561, -48.39072336876083824 ) ) ;
#36381=VECTOR ( 'NONE', #33157, 1000.000000000000000 ) ;
#36383=AXIS2_PLACEMENT_3D ( 'NONE', #58482, #54235, #48263 ) ;
#36384=CARTESIAN_POINT ( 'NONE',  ( 9.058156535714477542, 6.378495712187263855, 61.04019519618436362 ) ) ;
#36385=CARTESIAN_POINT ( 'NONE',  ( -26.88635117726412105, 9.904687797303049379, 43.69655592291272228 ) ) ;
#36387=CARTESIAN_POINT ( 'NONE',  ( 197.9843579228223973, 99.18296459057398806, 40.06359268299852516 ) ) ;
#36388=LINE ( 'NONE', #30768, #2798 ) ;
#36394=CARTESIAN_POINT ( 'NONE',  ( 111.1829448509513014, 30.43012797723692842, -62.81146689644553760 ) ) ;
#36396=CARTESIAN_POINT ( 'NONE',  ( 197.6145711261845292, 97.10888456119693046, -73.21698153998225678 ) ) ;
#36398=CARTESIAN_POINT ( 'NONE',  ( -125.8938041572051105, 46.49392987655495091, 72.46449846362081360 ) ) ;
#36399=CARTESIAN_POINT ( 'NONE',  ( -85.95621526752228192, 26.32462117888286102, -17.55249673712375369 ) ) ;
#36401=DIRECTION ( 'NONE',  ( -0.000000000000000000, 1.000000000000000000, -0.000000000000000000 ) ) ;
#36405=CARTESIAN_POINT ( 'NONE',  ( 64.93224207568368911, 14.16036304753835395, -9.121094072479223769 ) ) ;
#36406=CARTESIAN_POINT ( 'NONE',  ( -85.66184035008924980, 26.20110535976566979, -39.89909253867068628 ) ) ;
#36407=CARTESIAN_POINT ( 'NONE',  ( 116.3987821536696146, 31.83542673691012226, 86.50273311544268040 ) ) ;
#36408=CARTESIAN_POINT ( 'NONE',  ( -31.43908319763710679, -170.0000000000000000, 37.71645440618917888 ) ) ;
#36411=CARTESIAN_POINT ( 'NONE',  ( 164.3702714028688376, 63.22112480708619131, -67.51708439595032019 ) ) ;
#36412=ORIENTED_EDGE ( 'NONE', *, *, #62910, .F. ) ;
#36413=ORIENTED_EDGE ( 'NONE', *, *, #11597, .T. ) ;
#36417=CARTESIAN_POINT ( 'NONE',  ( -81.67992981004169906, 23.49232121719083821, 57.89061922115716641 ) ) ;
#36418=CARTESIAN_POINT ( 'NONE',  ( 103.0463737467386665, 25.69265572325593538, -95.00000000000133582 ) ) ;
#36420=CARTESIAN_POINT ( 'NONE',  ( -37.37206033059241150, 11.66494618096610836, -74.25636662139309863 ) ) ;
#36422=CARTESIAN_POINT ( 'NONE',  ( 31.91375106836930087, 7.553354707452895056, 63.77039173626905466 ) ) ;
#36423=CARTESIAN_POINT ( 'NONE',  ( 15.29293866748104413, 6.484959508098438796, -8.674393508222099314 ) ) ;
#36425=CARTESIAN_POINT ( 'NONE',  ( 23.04797191264876233, 7.849755664016357493, 8.723983137946492050 ) ) ;
#36426=CARTESIAN_POINT ( 'NONE',  ( 183.1865184929770862, 80.75677158533828504, 56.45068346174127782 ) ) ;
#36427=CARTESIAN_POINT ( 'NONE',  ( -124.1094910780272329, 45.33021696310839133, 3.987170503012005263 ) ) ;
#36430=CARTESIAN_POINT ( 'NONE',  ( 132.0440382699655117, 40.34028297386455364, -23.97074691722912121 ) ) ;
#36432=CARTESIAN_POINT ( 'NONE',  ( 15.29912143387264223, 7.491799981865497671, 3.170157082241544799 ) ) ;
#36437=CARTESIAN_POINT ( 'NONE',  ( 186.6118452967672852, 84.37814701615444335, 15.05814710111441457 ) ) ;
#36439=CARTESIAN_POINT ( 'NONE',  ( 173.6012773665503630, 71.36035397668605640, 36.22030391453991882 ) ) ;
#36442=CARTESIAN_POINT ( 'NONE',  ( 187.2296622856351291, 86.53808614709453195, -48.03209938450030592 ) ) ;
#36446=CARTESIAN_POINT ( 'NONE',  ( -142.4991775570125299, 58.45550857435407721, -12.74363189635909421 ) ) ;
#36447=CARTESIAN_POINT ( 'NONE',  ( 197.9843579228224542, 99.18296459057401648, 13.21904209253488816 ) ) ;
#36448=EDGE_CURVE ( 'NONE', #38167, #30354, #36144, .T. ) ;
#36452=CARTESIAN_POINT ( 'NONE',  ( 126.8114659053431694, 38.48351437375814044, -72.99081090039057074 ) ) ;
#36453=CARTESIAN_POINT ( 'NONE',  ( 126.5880720616305837, 37.20544379858409201, 38.87743667281387872 ) ) ;
#36455=EDGE_CURVE ( 'NONE', #22304, #67008, #32775, .T. ) ;
#36456=CARTESIAN_POINT ( 'NONE',  ( -94.88380767928866533, 29.17964217339916289, 39.28844685949278670 ) ) ;
#36460=CARTESIAN_POINT ( 'NONE',  ( -190.6985136298602015, 109.1272424661243434, 42.87371446347281534 ) ) ;
#36464=AXIS2_PLACEMENT_3D ( 'NONE', #61896, #13719, #51703 ) ;
#36465=DIRECTION ( 'NONE',  ( -0.000000000000000000, 1.000000000000000000, -0.000000000000000000 ) ) ;
#36466=ADVANCED_FACE ( 'NONE', ( #36777 ), #58220, .F. ) ;
#36467=CARTESIAN_POINT ( 'NONE',  ( -145.3233446620410803, 62.00659513626054320, -36.07151025764724750 ) ) ;
#36468=CARTESIAN_POINT ( 'NONE',  ( -127.6881387055493207, 48.89937523111244388, 57.67872152613632153 ) ) ;
#36470=CARTESIAN_POINT ( 'NONE',  ( -78.66644367742111399, -170.0000000000000000, 18.57365054920947500 ) ) ;
#36471=EDGE_CURVE ( 'NONE', #66651, #15369, #15215, .T. ) ;
#36474=EDGE_CURVE ( 'NONE', #69562, #25590, #49025, .T. ) ;
#36477=CARTESIAN_POINT ( 'NONE',  ( -62.54085973597667447, 16.81797209566547480, -16.36302326089210268 ) ) ;
#36478=CARTESIAN_POINT ( 'NONE',  ( -132.0870433264403516, 51.94057326482885628, -65.02066728891763603 ) ) ;
#36479=CARTESIAN_POINT ( 'NONE',  ( 181.0840389613909736, 78.60582251573003987, -89.91415884680696990 ) ) ;
#36483=ORIENTED_EDGE ( 'NONE', *, *, #2469, .F. ) ;
#36484=VERTEX_POINT ( 'NONE', #37442 ) ;
#36489=CARTESIAN_POINT ( 'NONE',  ( 103.5589117581614431, 27.00490790413959630, -66.82677417890924687 ) ) ;
#36490=CARTESIAN_POINT ( 'NONE',  ( -75.43271753227888610, 22.18711452892410918, 44.70239127070650653 ) ) ;
#36491=CARTESIAN_POINT ( 'NONE',  ( 79.52861599156695149, 17.11914630560288586, 34.74630206043598690 ) ) ;
#36493=CARTESIAN_POINT ( 'NONE',  ( -119.5563837756079550, 43.64229894412653721, 42.16241770139036049 ) ) ;
#36494=CARTESIAN_POINT ( 'NONE',  ( -166.9969673948021693, 80.56076768517782227, -64.71887823221233305 ) ) ;
#36496=CARTESIAN_POINT ( 'NONE',  ( -109.6660553119434951, 36.69391917620599486, -14.34154704396632418 ) ) ;
#36498=CARTESIAN_POINT ( 'NONE',  ( -177.9668641613811531, 92.68804954532606644, -90.16053173884390048 ) ) ;
#36501=CARTESIAN_POINT ( 'NONE',  ( -189.2346268516247392, 107.0830361517164846, -68.74365180755535221 ) ) ;
#36502=DIRECTION ( 'NONE',  ( -0.000000000000000000, 1.000000000000000000, -0.000000000000000000 ) ) ;
#36504=CARTESIAN_POINT ( 'NONE',  ( 37.00112095025829717, 8.109340230899352520, 17.67886562343527856 ) ) ;
#36506=CARTESIAN_POINT ( 'NONE',  ( -38.54237244144231767, 11.89088379031760034, -13.55305385010844432 ) ) ;
#36507=EDGE_LOOP ( 'NONE', ( #15363, #6378, #17648, #8008 ) ) ;
#36510=VERTEX_POINT ( 'NONE', #26897 ) ;
#36513=CARTESIAN_POINT ( 'NONE',  ( -25.50312845906833914, 8.692070753302667541, 6.281119717299506355 ) ) ;
#36515=CARTESIAN_POINT ( 'NONE',  ( -12.77647591501652791, 7.263973827022343066, -75.41787670511681085 ) ) ;
#36516=CARTESIAN_POINT ( 'NONE',  ( -94.79166046756726871, 29.13671350128075943, -15.17907392333536087 ) ) ;
#36517=CARTESIAN_POINT ( 'NONE',  ( 150.9013375937531407, 53.96275732797612790, -39.99563633385837846 ) ) ;
#36519=CIRCLE ( 'NONE', #57901, 242.4895526022646379 ) ;
#36523=CARTESIAN_POINT ( 'NONE',  ( -155.7455325080991599, 71.01834415181988902, 69.23728585488152021 ) ) ;
#36524=CARTESIAN_POINT ( 'NONE',  ( 174.4978817191264113, 73.57770570413205746, -20.47869960585826732 ) ) ;
#36529=CARTESIAN_POINT ( 'NONE',  ( -173.9526029538036198, 89.57590038685104616, -76.52212602822480392 ) ) ;
#36531=CARTESIAN_POINT ( 'NONE',  ( -1.319107422865894552, 6.554467368239822456, -19.83637397167817440 ) ) ;
#36532=EDGE_CURVE ( 'NONE', #51087, #17040, #34553, .T. ) ;
#36533=CARTESIAN_POINT ( 'NONE',  ( 110.2429982417149432, 28.88204397445228722, 44.61121420573733332 ) ) ;
#36539=CARTESIAN_POINT ( 'NONE',  ( 137.4117721579688407, 43.61242559081431125, 43.63136637536613449 ) ) ;
#36540=EDGE_CURVE ( 'NONE', #27181, #65685, #10967, .T. ) ;
#36542=CARTESIAN_POINT ( 'NONE',  ( 197.3054165770396935, 96.72615186924558373, 35.39984128414984355 ) ) ;
#36543=CARTESIAN_POINT ( 'NONE',  ( 111.1868021579656443, 29.32055685204858975, -62.81157359280074814 ) ) ;
#36544=CARTESIAN_POINT ( 'NONE',  ( 185.5457097283155008, 84.70846743303874860, 42.85523241993036692 ) ) ;
#36545=CARTESIAN_POINT ( 'NONE',  ( 164.0073343966822108, 64.23003864582456401, 13.75067327205471912 ) ) ;
#36547=VERTEX_POINT ( 'NONE', #40927 ) ;
#36549=ORIENTED_EDGE ( 'NONE', *, *, #43090, .F. ) ;
#36550=CARTESIAN_POINT ( 'NONE',  ( -74.40004226286974642, 20.74218500375954122, -21.94398046546645986 ) ) ;
#36552=CARTESIAN_POINT ( 'NONE',  ( -62.45356936877017517, 16.79156452995240301, 36.57604332370287636 ) ) ;
#36553=CARTESIAN_POINT ( 'NONE',  ( 150.4722669492348359, 53.65054032737657508, 7.353690365303933163 ) ) ;
#36555=CARTESIAN_POINT ( 'NONE',  ( 181.0840389613909736, -170.0000000000000000, 9.964043515047732669 ) ) ;
#36559=CARTESIAN_POINT ( 'NONE',  ( 111.1865443042262029, 30.43181341527239070, -50.87768516474636726 ) ) ;
#36565=VERTEX_POINT ( 'NONE', #57114 ) ;
#36566=CARTESIAN_POINT ( 'NONE',  ( 141.0804878838241052, 45.96076546397617335, 65.94046305877685654 ) ) ;
#36567=CARTESIAN_POINT ( 'NONE',  ( 157.4703587214989398, 58.92748579479259519, 71.25401806271709404 ) ) ;
#36568=CARTESIAN_POINT ( 'NONE',  ( 149.9552318559267121, 52.03645904563055780, 63.77717096610509628 ) ) ;
#36571=CARTESIAN_POINT ( 'NONE',  ( 46.65860211212412878, 10.48377752989033951, 12.52835627842576294 ) ) ;
#36572=ORIENTED_EDGE ( 'NONE', *, *, #42335, .F. ) ;
#36574=CARTESIAN_POINT ( 'NONE',  ( 156.3797504404255676, 58.07856685387021400, -24.20320859245837752 ) ) ;
#36575=CARTESIAN_POINT ( 'NONE',  ( 212.0104729185451617, 118.7959000526602722, -15.28514065634545283 ) ) ;
#36578=DIRECTION ( 'NONE',  ( -0.000000000000000000, 1.000000000000000000, -0.000000000000000000 ) ) ;
#36579=CARTESIAN_POINT ( 'NONE',  ( -151.2410113808309120, 65.66338888995504419, -76.46739901466715139 ) ) ;
#36580=DIRECTION ( 'NONE',  ( -0.000000000000000000, 1.000000000000000000, -0.000000000000000000 ) ) ;
#36582=CARTESIAN_POINT ( 'NONE',  ( 181.9295958320008424, 80.90438706151873305, 2.499716765681279096 ) ) ;
#36583=CARTESIAN_POINT ( 'NONE',  ( 211.0967808702091020, 115.5516932918876734, -47.74761114722220157 ) ) ;
#36589=CARTESIAN_POINT ( 'NONE',  ( -74.20136529587827567, 21.74007521413449595, 70.79374357570557663 ) ) ;
#36590=LINE ( 'NONE', #13828, #61031 ) ;
#36591=CARTESIAN_POINT ( 'NONE',  ( 39.40195752203892710, 9.424259417798131366, -23.77526687496409608 ) ) ;
#36594=CARTESIAN_POINT ( 'NONE',  ( -0.7888889703213518567, 6.534858899049522662, 88.68874176213427063 ) ) ;
#36595=CARTESIAN_POINT ( 'NONE',  ( -103.2164890789475322, 34.39030697009940951, -8.213902352593930090 ) ) ;
#36600=ORIENTED_EDGE ( 'NONE', *, *, #62855, .F. ) ;
#36601=CARTESIAN_POINT ( 'NONE',  ( -150.3898662070192245, 64.92828409760431896, 45.72082123989907387 ) ) ;
#36602=CARTESIAN_POINT ( 'NONE',  ( 57.07734607129818727, 11.37318329671159489, -47.82811536398262575 ) ) ;
#36603=CARTESIAN_POINT ( 'NONE',  ( 181.0840389613909736, 78.60582251573003987, -24.38050707541595230 ) ) ;
#36605=EDGE_CURVE ( 'NONE', #1104, #62158, #58800, .T. ) ;
#36608=CARTESIAN_POINT ( 'NONE',  ( -127.4644500646574556, 48.74852676951794450, 30.78273999091167568 ) ) ;
#36610=CARTESIAN_POINT ( 'NONE',  ( 210.1954643503415525, 114.1986276268023488, 14.97053208330250484 ) ) ;
#36611=CARTESIAN_POINT ( 'NONE',  ( -142.0227972901369071, 59.36121938936275200, 37.66433558148366956 ) ) ;
#36612=CARTESIAN_POINT ( 'NONE',  ( 210.1633650091869185, 114.1507944623966750, 31.56596133871580179 ) ) ;
#36619=EDGE_CURVE ( 'NONE', #5211, #32318, #4260, .T. ) ;
#36622=CARTESIAN_POINT ( 'NONE',  ( -133.3409562061681584, 52.83409703973299543, 92.75988323507705502 ) ) ;
#36624=CARTESIAN_POINT ( 'NONE',  ( 34.45158752686798209, 8.829194381142023929, -64.30894078306647543 ) ) ;
#36627=CARTESIAN_POINT ( 'NONE',  ( 8.727163641868461497, 7.383472852351860460, 88.65466339244591154 ) ) ;
#36633=AXIS2_PLACEMENT_3D ( 'NONE', #11715, #12774, #23339 ) ;
#36634=CARTESIAN_POINT ( 'NONE',  ( -97.49219489034503283, 30.41416107059312068, 59.07020065800807629 ) ) ;
#36636=CARTESIAN_POINT ( 'NONE',  ( -85.46258339457286013, 25.02772366257410042, 7.891551977632535575 ) ) ;
#36637=VERTEX_POINT ( 'NONE', #50370 ) ;
#36638=AXIS2_PLACEMENT_3D ( 'NONE', #44794, #66274, #18066 ) ;
#36641=CARTESIAN_POINT ( 'NONE',  ( -118.3918229753714968, 42.92682904595258719, 10.76576233191594234 ) ) ;
#36642=CARTESIAN_POINT ( 'NONE',  ( -177.5259994307673423, 92.16784265327248704, 59.07817098000860057 ) ) ;
#36643=CARTESIAN_POINT ( 'NONE',  ( 131.6005058089755266, 40.07838125795768747, 56.68696652403973957 ) ) ;
#36644=ORIENTED_EDGE ( 'NONE', *, *, #67276, .T. ) ;
#36646=CARTESIAN_POINT ( 'NONE',  ( -32.09835183227463773, 9.700355081940386981, 83.92768983820710105 ) ) ;
#36647=CARTESIAN_POINT ( 'NONE',  ( 152.2940756559018780, 53.73566983921581652, 31.47669956291998616 ) ) ;
#36649=CYLINDRICAL_SURFACE ( 'NONE', #11356, 7.500000000000013323 ) ;
#36650=CARTESIAN_POINT ( 'NONE',  ( -25.98312968277007329, 8.759224980175259745, 32.56453152482685454 ) ) ;
#36651=CARTESIAN_POINT ( 'NONE',  ( -143.4048679855200987, 60.45763799613827416, -64.79020762706440451 ) ) ;
#36654=CARTESIAN_POINT ( 'NONE',  ( -85.10909119100207931, 25.97025675005451717, -73.33204673147415065 ) ) ;
#36655=CARTESIAN_POINT ( 'NONE',  ( 174.2468109002383585, 73.34092405459593067, 13.05881135404167637 ) ) ;
#36659=CARTESIAN_POINT ( 'NONE',  ( -156.3790798118593557, 70.23422112803314121, 8.359172547404261522 ) ) ;
#36660=CARTESIAN_POINT ( 'NONE',  ( -118.7011544766493074, 43.11604763363182968, -67.11694934325225859 ) ) ;
#36661=CARTESIAN_POINT ( 'NONE',  ( 64.69649025047539226, 13.06878919510320891, 3.155138310929866741 ) ) ;
#36663=CARTESIAN_POINT ( 'NONE',  ( -105.4556185321791446, 34.42302275449793569, 44.83015365805241004 ) ) ;
#36667=CARTESIAN_POINT ( 'NONE',  ( -50.38034822888705833, 14.51481641465389671, 85.63106280517327207 ) ) ;
#36670=ORIENTED_EDGE ( 'NONE', *, *, #49351, .F. ) ;
#36674=CARTESIAN_POINT ( 'NONE',  ( -172.3127615181935823, 87.73358064377643473, 30.85409139483959606 ) ) ;
#36675=CARTESIAN_POINT ( 'NONE',  ( 63.01563776193091826, 12.67277567978500308, -23.87614024170608218 ) ) ;
#36682=CARTESIAN_POINT ( 'NONE',  ( 110.2429982417149432, 29.99119854320847267, 56.45576479620100940 ) ) ;
#36683=CARTESIAN_POINT ( 'NONE',  ( -120.1650841064593891, 44.02024060322521137, -10.72207681748146513 ) ) ;
#36686=ORIENTED_EDGE ( 'NONE', *, *, #59946, .T. ) ;
#36688=CARTESIAN_POINT ( 'NONE',  ( 177.5852526894774712, 76.54518907282665907, 83.85689353362545262 ) ) ;
#36699=CARTESIAN_POINT ( 'NONE',  ( 86.62931800182293784, 19.42108912189597447, -23.97701360844805407 ) ) ;
#36700=CARTESIAN_POINT ( 'NONE',  ( 205.5004956747122264, 107.4493581495448069, -24.44922967293032201 ) ) ;
#36702=CARTESIAN_POINT ( 'NONE',  ( 162.0812592823605200, 62.62783216273701470, 69.68866734599082235 ) ) ;
#36706=CARTESIAN_POINT ( 'NONE',  ( 126.6266894765173703, 38.37986986668739320, 12.22883615118388079 ) ) ;
#36708=LINE ( 'NONE', #30737, #35227 ) ;
#36709=CARTESIAN_POINT ( 'NONE',  ( -109.0291978193666438, 37.49173305805086187, -72.64004148779659431 ) ) ;
#36711=CARTESIAN_POINT ( 'NONE',  ( -6.528484601666539433, 7.817818436116853675, 83.91048964419407241 ) ) ;
#36714=CARTESIAN_POINT ( 'NONE',  ( -62.56514071794335052, 16.82532503654672240, 64.66934574899191546 ) ) ;
#36716=VECTOR ( 'NONE', #10269, 1000.000000000000000 ) ;
#36718=CARTESIAN_POINT ( 'NONE',  ( 32.28474208827732639, 8.601490596599902005, 93.49151023392415993 ) ) ;
#36719=CARTESIAN_POINT ( 'NONE',  ( -177.5259994307673992, 92.16784265327254388, -75.14458197230979408 ) ) ;
#36720=B_SPLINE_CURVE_WITH_KNOTS ( 'NONE', 3,
 ( #11297, #6384, #19365, #8125, #51391, #40474, #18685, #19023, #34868, #24318, #13068, #62276, #23617, #2165, #61919, #23275, #51038, #2506, #17991, #44722, #34531, #55614, #55972, #45054, #7784, #7082, #2851, #29237, #50348, #66199, #50682, #7443, #67564, #46095, #12711, #66540, #45407, #40822, #23956, #14094, #66890, #13405, #55262, #28539, #61594 ),
 .UNSPECIFIED., .F., .F.,
 ( 4, 2, 2, 2, 2, 2, 2, 2, 2, 2, 2, 2, 2, 1, 2, 2, 2, 2, 2, 2, 2, 2, 4 ),
 ( 0.02352719711393055566, 0.02499986300757020205, 0.02573619595439003566, 0.02647252890120986579, 0.02794519479484951566, 0.02941786068848916899, 0.03015419363530899219, 0.03089052658212881886, 0.03236319247576845137, 0.03309952542258825375, 0.03383585836940805613, 0.03530852426304766783, 0.03604485720986745634, 0.03678119015668723790, 0.03751752310350701947, 0.03825385605032680103, 0.03972652194396641273, 0.04119918783760601749, 0.04267185373124562919, 0.04340818667806543851, 0.04414451962488524783, 0.04561718551852483872, 0.04708985141216442960 ),
 .UNSPECIFIED. ) ;
#36724=CARTESIAN_POINT ( 'NONE',  ( 22.25657943806483274, 7.801867731668604478, 94.99999999999866418 ) ) ;
#36725=DIRECTION ( 'NONE',  ( -0.000000000000000000, 1.000000000000000000, -0.000000000000000000 ) ) ;
#36726=CARTESIAN_POINT ( 'NONE',  ( 33.75639351246965703, 7.742023566824293823, -21.23742916720711449 ) ) ;
#36727=CARTESIAN_POINT ( 'NONE',  ( 173.5836858989432301, 72.71885240881779566, -43.43828145153533171 ) ) ;
#36729=CARTESIAN_POINT ( 'NONE',  ( 163.5430354047457229, 62.53125887746119105, 94.99999999999866418 ) ) ;
#36730=CARTESIAN_POINT ( 'NONE',  ( 93.63037639125408873, 21.92981100938039773, 39.91368610796941852 ) ) ;
#36734=CARTESIAN_POINT ( 'NONE',  ( 14.80205238535216772, 6.470775952815776222, 56.90826214576678410 ) ) ;
#36735=CARTESIAN_POINT ( 'NONE',  ( 8.288696687633805738, 7.382586467017839382, 37.01382362586534924 ) ) ;
#36736=CARTESIAN_POINT ( 'NONE',  ( 201.5987353083855567, 103.8544727311227120, 29.86444194458761814 ) ) ;
#36737=CARTESIAN_POINT ( 'NONE',  ( 80.34841469379381351, 17.37275484083203381, 94.99999999999866418 ) ) ;
#36741=ORIENTED_EDGE ( 'NONE', *, *, #36474, .F. ) ;
#36742=CARTESIAN_POINT ( 'NONE',  ( 114.6659427952415200, 32.10199811723106222, -64.19130057980802917 ) ) ;
#36746=CARTESIAN_POINT ( 'NONE',  ( -125.4433371161043880, 46.19736518073189302, 72.46449846362084202 ) ) ;
#36747=CARTESIAN_POINT ( 'NONE',  ( 154.0401952541423043, 55.03227529428313858, -63.79514857056523169 ) ) ;
#36748=CARTESIAN_POINT ( 'NONE',  ( 22.99481266947290337, 7.846456081397400695, -94.58791541915923062 ) ) ;
#36749=CARTESIAN_POINT ( 'NONE',  ( -155.7495771807047902, 69.65980221699321362, -46.50072862889067693 ) ) ;
#36752=CARTESIAN_POINT ( 'NONE',  ( 69.35866309798979046, 15.27376159675663558, -12.36654855831349842 ) ) ;
#36754=CARTESIAN_POINT ( 'NONE',  ( 160.5141379054754225, 60.05651755415394177, 70.62330748442225570 ) ) ;
#36755=CARTESIAN_POINT ( 'NONE',  ( 116.5100763992442978, 33.01539745157282368, -12.45056777525001301 ) ) ;
#36756=EDGE_CURVE ( 'NONE', #16484, #63871, #29418, .T. ) ;
#36759=CARTESIAN_POINT ( 'NONE',  ( 18.21423326326598158, 6.590134686181414736, 44.62829782856979222 ) ) ;
#36767=EDGE_CURVE ( 'NONE', #8782, #39218, #51749, .T. ) ;
#36768=CARTESIAN_POINT ( 'NONE',  ( 36.30999198706538778, 9.040534725358947199, -36.28248531905617114 ) ) ;
#36771=EDGE_CURVE ( 'NONE', #69259, #49668, #17711, .T. ) ;
#36773=CARTESIAN_POINT ( 'NONE',  ( 197.8598785550297237, 99.02620879292952338, 60.45626783609857569 ) ) ;
#36774=ORIENTED_EDGE ( 'NONE', *, *, #27435, .T. ) ;
#36777=FACE_OUTER_BOUND ( 'NONE', #62469, .T. ) ;
#36781=CARTESIAN_POINT ( 'NONE',  ( -118.8689810167775960, 42.03922634358562505, 8.635105111016807555 ) ) ;
#36785=CARTESIAN_POINT ( 'NONE',  ( 14.08810621383467243, 7.458732232275136376, 3.361252658025919438 ) ) ;
#36789=CARTESIAN_POINT ( 'NONE',  ( 188.4904153916303642, 86.42965364612517476, 8.744626016292592396 ) ) ;
#36791=CARTESIAN_POINT ( 'NONE',  ( 180.2473887773227545, 77.76029175826236894, 44.30859410551141764 ) ) ;
#36793=CARTESIAN_POINT ( 'NONE',  ( -106.4728934171454142, 36.10295170132725673, -48.73770635309175248 ) ) ;
#36798=CARTESIAN_POINT ( 'NONE',  ( 173.5922027797725207, 71.35194229497426477, 90.90255056565294467 ) ) ;
#36799=EDGE_LOOP ( 'NONE', ( #27799, #65586, #54852, #53301 ) ) ;
#36800=CARTESIAN_POINT ( 'NONE',  ( 115.2288739107204805, 31.25773204386716486, 58.34775827273530524 ) ) ;
#36803=CARTESIAN_POINT ( 'NONE',  ( 132.0440382699655117, 40.34028297386453232, 29.71835426369820965 ) ) ;
#36805=CARTESIAN_POINT ( 'NONE',  ( -98.67723517640904163, 30.98797878696538888, 44.60132663403577169 ) ) ;
#36806=CARTESIAN_POINT ( 'NONE',  ( 93.71772995179814814, 21.96265635001559247, -40.85830305015011277 ) ) ;
#36810=CYLINDRICAL_SURFACE ( 'NONE', #15989, 7.500000000000013323 ) ;
#36814=CARTESIAN_POINT ( 'NONE',  ( -118.3927673406137160, 41.74929850983303226, -15.33123327190856600 ) ) ;
#36817=CARTESIAN_POINT ( 'NONE',  ( -180.5231752320738110, 95.76423526868921954, -14.11972369233568436 ) ) ;
#36819=CARTESIAN_POINT ( 'NONE',  ( -149.2910611247327779, 63.99625741915655652, -34.81283053149194728 ) ) ;
#36821=CARTESIAN_POINT ( 'NONE',  ( 60.40531521312254171, 13.11276739283242243, 3.433157306431154687 ) ) ;
#36825=EDGE_CURVE ( 'NONE', #52414, #27866, #52945, .T. ) ;
#36826=CARTESIAN_POINT ( 'NONE',  ( -60.13226458141418362, 16.10241298991027037, -10.34831921288341583 ) ) ;
#36828=CARTESIAN_POINT ( 'NONE',  ( -132.8257891167039304, 52.46553896898736014, -66.38325077981791367 ) ) ;
#36830=CARTESIAN_POINT ( 'NONE',  ( -94.79534239005252516, 29.13842790650044634, 10.63132434853593367 ) ) ;
#36831=CARTESIAN_POINT ( 'NONE',  ( -99.31850058233800382, 31.30166762705808381, -62.46462738374896873 ) ) ;
#36834=CARTESIAN_POINT ( 'NONE',  ( 181.0840389613909736, 78.60582251573005408, -63.06960825634327961 ) ) ;
#36835=CARTESIAN_POINT ( 'NONE',  ( -166.9969673948021409, 80.56076768517783648, -37.87432764174864985 ) ) ;
#36836=DIRECTION ( 'NONE',  ( 0.000000000000000000, 0.000000000000000000, 1.000000000000000000 ) ) ;
#36837=CARTESIAN_POINT ( 'NONE',  ( 110.2429982417149574, 29.99119854320844425, -62.76698815611734972 ) ) ;
#36838=CARTESIAN_POINT ( 'NONE',  ( -77.71801202538874520, 23.03755222122951096, 45.37301624558984514 ) ) ;
#36839=CARTESIAN_POINT ( 'NONE',  ( 86.15410276028862313, 19.25894675708892123, 29.71208757247930521 ) ) ;
#36840=CARTESIAN_POINT ( 'NONE',  ( 68.94309019697858787, 15.16533147648755175, -38.59916606691003693 ) ) ;
#36841=CARTESIAN_POINT ( 'NONE',  ( -122.8202784017355498, 45.69728649588467562, 44.96525387181218747 ) ) ;
#36847=CARTESIAN_POINT ( 'NONE',  ( -35.38560449531985341, 10.27249159032101744, 4.489560872237628786 ) ) ;
#36848=CARTESIAN_POINT ( 'NONE',  ( 79.18180043629686793, 18.06526831600450222, 63.03804907646694033 ) ) ;
#36850=CARTESIAN_POINT ( 'NONE',  ( 155.7277429502854034, 56.30804678861340307, -24.08774153568633380 ) ) ;
#36851=CARTESIAN_POINT ( 'NONE',  ( 34.83823433017390414, 8.871835168107976344, 4.597148557001253799 ) ) ;
#36853=CARTESIAN_POINT ( 'NONE',  ( 32.56927464314651388, 7.618924692399909659, -73.06680367152966937 ) ) ;
#36854=CARTESIAN_POINT ( 'NONE',  ( -102.2801239173131194, 33.91021738430207932, -61.85912785543958847 ) ) ;
#36855=EDGE_CURVE ( 'NONE', #57935, #13481, #68943, .T. ) ;
#36856=CARTESIAN_POINT ( 'NONE',  ( -38.68632430131781064, 11.91908191268691297, -14.02620273824548924 ) ) ;
#36862=CARTESIAN_POINT ( 'NONE',  ( -24.41864932425147927, 8.543938959778817122, 13.52232210049978356 ) ) ;
#36864=CARTESIAN_POINT ( 'NONE',  ( -12.39701069459754201, 7.231688578592716077, -75.72825898634536657 ) ) ;
#36865=CARTESIAN_POINT ( 'NONE',  ( -98.46684543088103680, 30.88557736720388647, -9.207280559787971441 ) ) ;
#36867=CARTESIAN_POINT ( 'NONE',  ( 151.1827182658834090, 54.16800928478852484, -47.74454161914079009 ) ) ;
#36870=ORIENTED_EDGE ( 'NONE', *, *, #60674, .T. ) ;
#36873=CARTESIAN_POINT ( 'NONE',  ( 173.6737675136087660, 72.80308721038097985, -18.07488780512645832 ) ) ;
#36876=CARTESIAN_POINT ( 'NONE',  ( -109.6657532478350561, 37.84376708859252858, 63.53280748219179941 ) ) ;
#36881=CARTESIAN_POINT ( 'NONE',  ( 91.51282003084290295, 21.14522045960332619, 69.76978587635888118 ) ) ;
#36883=CARTESIAN_POINT ( 'NONE',  ( -156.9664270383552491, 70.77351443782143292, 91.10669583694630091 ) ) ;
#36884=CARTESIAN_POINT ( 'NONE',  ( 141.0804878838241336, 45.96076546397619467, 39.09591246831315914 ) ) ;
#36885=VERTEX_POINT ( 'NONE', #34469 ) ;
#36888=CARTESIAN_POINT ( 'NONE',  ( 188.2086267457325448, 87.61890531228286250, 34.44826965832049126 ) ) ;
#36889=CARTESIAN_POINT ( 'NONE',  ( 162.7963212667073662, 63.21900188423072819, 15.35118721056019986 ) ) ;
#36890=CARTESIAN_POINT ( 'NONE',  ( -100.4440683050664518, 32.98184228837415333, 45.30557044946138490 ) ) ;
#36891=EDGE_LOOP ( 'NONE', ( #64912, #19969, #62362, #16030 ) ) ;
#36892=CARTESIAN_POINT ( 'NONE',  ( 173.6700117628886346, 72.79957362875116189, 64.82362119438116110 ) ) ;
#36894=CARTESIAN_POINT ( 'NONE',  ( -108.9452487746634120, 36.29752968355630571, -45.99127851335813943 ) ) ;
#36896=DIRECTION ( 'NONE',  ( -0.000000000000000000, 1.000000000000000000, -0.000000000000000000 ) ) ;
#36897=DIRECTION ( 'NONE',  ( 0.000000000000000000, 0.000000000000000000, 1.000000000000000000 ) ) ;
#36899=CARTESIAN_POINT ( 'NONE',  ( -178.5835577246388368, 93.42126246260829703, 33.17678452161792535 ) ) ;
#36900=CARTESIAN_POINT ( 'NONE',  ( 133.8566784816069344, -170.0000000000000000, -24.17876034193199786 ) ) ;
#36905=AXIS2_PLACEMENT_3D ( 'NONE', #26998, #618, #48428 ) ;
#36907=CARTESIAN_POINT ( 'NONE',  ( 136.9798231265810102, 43.34196232604178789, 57.02028350268891899 ) ) ;
#36908=CARTESIAN_POINT ( 'NONE',  ( -173.5372686962701039, 89.10569330281725797, 30.82169460664102800 ) ) ;
#36909=CARTESIAN_POINT ( 'NONE',  ( 152.6560521232695180, 54.00248515670892857, 57.99803634713506284 ) ) ;
#36910=CARTESIAN_POINT ( 'NONE',  ( 94.11733320392094981, 23.18939451097131865, 36.71840950062001241 ) ) ;
#36913=CARTESIAN_POINT ( 'NONE',  ( 40.38132770291768736, 9.553709436640065888, 18.02098113922875555 ) ) ;
#36915=CARTESIAN_POINT ( 'NONE',  ( 152.1381498073140790, 54.87048121475570639, -22.07591650116782844 ) ) ;
#36917=CARTESIAN_POINT ( 'NONE',  ( 206.2957331585308793, 110.2946564621822887, -24.35451595762442167 ) ) ;
#36920=CARTESIAN_POINT ( 'NONE',  ( 64.66528157600511406, 13.06122252980780019, 83.67837878186749379 ) ) ;
#36925=ADVANCED_FACE ( 'NONE', ( #39040 ), #60130, .T. ) ;
#36929=CARTESIAN_POINT ( 'NONE',  ( -75.00636493611887090, 22.03142602679958983, 71.32676556850506699 ) ) ;
#36930=CARTESIAN_POINT ( 'NONE',  ( 205.0999694062793424, 106.8955893716605061, -78.17048162308529413 ) ) ;
#36932=CARTESIAN_POINT ( 'NONE',  ( 40.38495044702529668, 9.554194848483446023, -23.72658219154430626 ) ) ;
#36935=CARTESIAN_POINT ( 'NONE',  ( 22.89270809252618832, 7.840160460323052583, 39.93075722470221933 ) ) ;
#36938=EDGE_LOOP ( 'NONE', ( #55387, #3427, #38903, #29311 ) ) ;
#36939=CARTESIAN_POINT ( 'NONE',  ( -71.59086462055189770, 19.75139532313339430, 62.26276460702656124 ) ) ;
#36940=CARTESIAN_POINT ( 'NONE',  ( 203.0745197111477580, 104.1448368405267786, -90.18520043603034253 ) ) ;
#36943=CARTESIAN_POINT ( 'NONE',  ( -156.4960819023050931, 70.34114605623871341, 40.99531223057345386 ) ) ;
#36944=CARTESIAN_POINT ( 'NONE',  ( 55.90910788310614521, 11.13585330978401267, -40.77322039613591897 ) ) ;
#36946=CARTESIAN_POINT ( 'NONE',  ( -149.5074843970971017, 64.17983161892348676, 3.876270649435373361 ) ) ;
#36951=LINE ( 'NONE', #26738, #43524 ) ;
#36954=CARTESIAN_POINT ( 'NONE',  ( 187.3988733513474756, 86.72376876819507174, -93.34304573699913021 ) ) ;
#36955=DIRECTION ( 'NONE',  ( -0.000000000000000000, 1.000000000000000000, -0.000000000000000000 ) ) ;
#36966=CARTESIAN_POINT ( 'NONE',  ( -133.1441247387262194, 52.69302668368034404, 93.75700809079965836 ) ) ;
#36967=CARTESIAN_POINT ( 'NONE',  ( 37.45439421541016145, 9.177432671831368793, -62.70490429592918957 ) ) ;
#36969=CARTESIAN_POINT ( 'NONE',  ( 69.08240197259638649, 14.16210831900842315, 32.89646892813778578 ) ) ;
#36970=CARTESIAN_POINT ( 'NONE',  ( 20.10890210143426771, 7.684797874382650384, 85.06464190967132311 ) ) ;
#36974=CARTESIAN_POINT ( 'NONE',  ( -97.85576954355161661, 30.58918648956189656, 70.93880484806753373 ) ) ;
#36976=CARTESIAN_POINT ( 'NONE',  ( -82.32931163805226049, 23.75065981441938234, 4.524469639083367412 ) ) ;
#36980=CARTESIAN_POINT ( 'NONE',  ( -118.4470345550925856, 42.96051736048242731, 10.23307076808440463 ) ) ;
#36981=CARTESIAN_POINT ( 'NONE',  ( -180.5231752320737542, 95.76423526868920533, 66.41392807905532436 ) ) ;
#36982=CARTESIAN_POINT ( 'NONE',  ( 127.2397149628677653, 37.56999625068104365, 67.42304229148038530 ) ) ;
#36984=CARTESIAN_POINT ( 'NONE',  ( -29.23666642776608526, 9.240073959287249394, 84.22891760168137409 ) ) ;
#36986=CARTESIAN_POINT ( 'NONE',  ( 151.6192474229129346, 53.24103268919209597, 32.21058103104000025 ) ) ;
#36988=CARTESIAN_POINT ( 'NONE',  ( 106.6228877857910646, 27.24245963308693064, -36.83655804471349171 ) ) ;
#36989=CARTESIAN_POINT ( 'NONE',  ( 139.6150621148398159, 46.20856238844173447, -65.53656864805886073 ) ) ;
#36995=CARTESIAN_POINT ( 'NONE',  ( -119.5404913382140251, 43.63271406506960659, -46.40773658427427506 ) ) ;
#36996=CARTESIAN_POINT ( 'NONE',  ( -85.10909119100209352, 25.97025675005451006, 7.201605039916894491 ) ) ;
#36998=CARTESIAN_POINT ( 'NONE',  ( -156.7487895666416762, 70.57327586518564999, 9.403214650218792769 ) ) ;
#36999=EDGE_CURVE ( 'NONE', #41404, #48198, #65418, .T. ) ;
#37000=CARTESIAN_POINT ( 'NONE',  ( 197.2002799314678896, 98.19982998998082735, 89.90084543270276640 ) ) ;
#37001=CARTESIAN_POINT ( 'NONE',  ( 69.50572373348799715, 14.27208627753790360, 14.25933825401109800 ) ) ;
#37003=CARTESIAN_POINT ( 'NONE',  ( -107.0584934212648704, 35.27493744466470815, 43.82066438551851917 ) ) ;
#37006=CARTESIAN_POINT ( 'NONE',  ( -62.53610861913121255, 17.86800032500430646, 90.91069339059835386 ) ) ;
#37010=VERTEX_POINT ( 'NONE', #52602 ) ;
#37011=CIRCLE ( 'NONE', #44897, 242.4895526022646379 ) ;
#37012=EDGE_CURVE ( 'NONE', #10653, #3542, #36096, .T. ) ;
#37015=CARTESIAN_POINT ( 'NONE',  ( -173.1211646369891355, 88.63826465341151106, 30.82169460664101734 ) ) ;
#37020=CARTESIAN_POINT ( 'NONE',  ( -50.14440374537738876, 14.45628984983895648, -63.86889621594647792 ) ) ;
#37022=CARTESIAN_POINT ( 'NONE',  ( -120.6739978760426197, 44.33795494230365364, -10.17821021773952594 ) ) ;
#37023=VERTEX_POINT ( 'NONE', #9357 ) ;
#37025=CARTESIAN_POINT ( 'NONE',  ( 174.6728071617951059, 73.74298290599254813, 94.40752414145283922 ) ) ;
#37028=AXIS2_PLACEMENT_3D ( 'NONE', #53322, #31213, #21670 ) ;
#37032=CARTESIAN_POINT ( 'NONE',  ( 184.5867277229704086, 83.68414666546580349, -10.24489875072611866 ) ) ;
#37033=CARTESIAN_POINT ( 'NONE',  ( 210.9631450001601252, 117.1791136960929549, 5.703577349153958309 ) ) ;
#37034=CARTESIAN_POINT ( 'NONE',  ( -178.5835577246388368, 93.42126246260829703, -47.35686724977312423 ) ) ;
#37035=CARTESIAN_POINT ( 'NONE',  ( 93.63037639125411715, 21.92981100938039063, -13.77541507295795853 ) ) ;
#37036=CARTESIAN_POINT ( 'NONE',  ( -30.95341298663139185, 10.53108683215057262, 57.06100499665286918 ) ) ;
#37039=CARTESIAN_POINT ( 'NONE',  ( 164.6561571795775194, 64.77723933022093661, 65.97358011928493227 ) ) ;
#37044=CARTESIAN_POINT ( 'NONE',  ( 133.8566784816069344, -170.0000000000000000, -43.52331093239567394 ) ) ;
#37045=CARTESIAN_POINT ( 'NONE',  ( 154.0401952541423611, 55.03227529428311726, 16.73850320082579657 ) ) ;
#37047=CARTESIAN_POINT ( 'NONE',  ( -1.036819421871533864, 7.550827156688815656, 88.09984161770725564 ) ) ;
#37051=ORIENTED_EDGE ( 'NONE', *, *, #46621, .F. ) ;
#37052=CARTESIAN_POINT ( 'NONE',  ( 36.82270405522987744, 9.100602243567198713, 84.02932348124475936 ) ) ;
#37054=CARTESIAN_POINT ( 'NONE',  ( 137.5016378680191735, 44.85812207451340328, -90.64634188293649686 ) ) ;
#37056=CARTESIAN_POINT ( 'NONE',  ( 204.6977192012829505, 108.0580384837234931, 2.363170148305746565 ) ) ;
#37058=CARTESIAN_POINT ( 'NONE',  ( 32.46582151331404020, 7.608418548522498881, -13.39088614318420412 ) ) ;
#37059=CARTESIAN_POINT ( 'NONE',  ( 174.2538192999569731, 73.34752463892030505, -46.83513099018006898 ) ) ;
#37061=CARTESIAN_POINT ( 'NONE',  ( -152.9008427825210106, 68.45483453645051952, -75.84960517240774891 ) ) ;
#37066=ADVANCED_FACE ( 'NONE', ( #25889 ), #46986, .F. ) ;
#37067=FACE_OUTER_BOUND ( 'NONE', #34322, .T. ) ;
#37068=CARTESIAN_POINT ( 'NONE',  ( -31.43908319763709969, 10.61114334766716105, 30.21645440618916112 ) ) ;
#37070=DIRECTION ( 'NONE',  ( -0.000000000000000000, 1.000000000000000000, -0.000000000000000000 ) ) ;
#37072=ORIENTED_EDGE ( 'NONE', *, *, #22449, .F. ) ;
#37073=ORIENTED_EDGE ( 'NONE', *, *, #25721, .T. ) ;
#37075=ORIENTED_EDGE ( 'NONE', *, *, #15434, .F. ) ;
#37076=CARTESIAN_POINT ( 'NONE',  ( 111.1865443042261603, 30.43181341527238359, -77.72223575521005046 ) ) ;
#37077=DIRECTION ( 'NONE',  ( 0.000000000000000000, 0.000000000000000000, 1.000000000000000000 ) ) ;
#37078=PLANE ( 'NONE',  #50120 ) ;
#37080=CARTESIAN_POINT ( 'NONE',  ( -31.43908319763709969, 10.61114334766715928, 57.06100499665286208 ) ) ;
#37081=CARTESIAN_POINT ( 'NONE',  ( -9.779603649692305112, 8.034615131607072414, -8.815743396744277760 ) ) ;
#37082=CARTESIAN_POINT ( 'NONE',  ( 152.3102623290679105, 53.74757787434985801, -65.02056816791532867 ) ) ;
#37083=CARTESIAN_POINT ( 'NONE',  ( 19.10216788411012701, 6.629360741291161041, -22.90701642875757926 ) ) ;
#37084=CARTESIAN_POINT ( 'NONE',  ( -156.6692143066620702, 70.50016761530885390, -44.55701924433694927 ) ) ;
#37089=CARTESIAN_POINT ( 'NONE',  ( 70.41705859591009187, 15.55317472777718102, -17.61350428500981025 ) ) ;
#37090=CARTESIAN_POINT ( 'NONE',  ( -31.43908319763709969, 9.591432048623758533, -23.47264677473818395 ) ) ;
#37093=CARTESIAN_POINT ( 'NONE',  ( -152.2873556200145799, 67.91256772393731467, 4.406972807603752429 ) ) ;
#37095=CARTESIAN_POINT ( 'NONE',  ( 22.30016284075437127, 6.796348835713779124, 41.26772859709231511 ) ) ;
#37096=CARTESIAN_POINT ( 'NONE',  ( -157.0087551414807194, 72.18321165533608053, 91.79709723166649837 ) ) ;
#37100=CARTESIAN_POINT ( 'NONE',  ( -150.5993571094983281, 66.43939758484178526, -22.89157138131998437 ) ) ;
#37101=CARTESIAN_POINT ( 'NONE',  ( 93.02946412630693374, 22.77895695581315039, -93.07924972775212780 ) ) ;
#37104=CARTESIAN_POINT ( 'NONE',  ( -33.36721086971962080, 9.915747831546610769, 71.81304879671020558 ) ) ;
#37105=CARTESIAN_POINT ( 'NONE',  ( -155.7495771807047333, 69.65980221699317099, -19.65617803842697242 ) ) ;
#37108=DIRECTION ( 'NONE',  ( -0.000000000000000000, 1.000000000000000000, -0.000000000000000000 ) ) ;
#37109=CARTESIAN_POINT ( 'NONE',  ( 22.72762739171800561, 7.830015800126076009, 13.54664626853137577 ) ) ;
#37110=CARTESIAN_POINT ( 'NONE',  ( 186.6118452967672567, 84.37814701615440072, 68.74724828204176674 ) ) ;
#37112=DIRECTION ( 'NONE',  ( -0.8118923937861950435, -0.5838071093367415143, 0.000000000000000000 ) ) ;
#37118=CARTESIAN_POINT ( 'NONE',  ( 187.2354698746857196, 85.05376776489252677, 5.644151847218983775 ) ) ;
#37121=CARTESIAN_POINT ( 'NONE',  ( 132.0249343950657135, 41.49728247212332377, -36.19146592362032777 ) ) ;
#37122=CARTESIAN_POINT ( 'NONE',  ( -132.4819073909166320, 50.98736898418876251, -38.79117142572575005 ) ) ;
#37123=CARTESIAN_POINT ( 'NONE',  ( -104.7956873821848802, 35.21322275870668506, -49.58398961066640709 ) ) ;
#37124=CARTESIAN_POINT ( 'NONE',  ( 60.63380853769237433, 13.16344960520420848, -77.18114081708419860 ) ) ;
#37128=CARTESIAN_POINT ( 'NONE',  ( 173.6061830963395778, 71.36490884257202083, 91.10848141826026847 ) ) ;
#37130=DIRECTION ( 'NONE',  ( -0.000000000000000000, 1.000000000000000000, -0.000000000000000000 ) ) ;
#37132=CARTESIAN_POINT ( 'NONE',  ( 132.0249343950657703, 41.49728247212335219, -63.03601651408401096 ) ) ;
#37133=CARTESIAN_POINT ( 'NONE',  ( 130.7260704202055024, 39.56565398554882051, 30.17888742523724943 ) ) ;
#37136=CARTESIAN_POINT ( 'NONE',  ( 163.1459438811106679, 62.20198481903361909, -92.39285677337488778 ) ) ;
#37138=CARTESIAN_POINT ( 'NONE',  ( 94.11746922806584337, 22.11341285603782936, -42.82955049988751739 ) ) ;
#37142=ORIENTED_EDGE ( 'NONE', *, *, #7929, .F. ) ;
#37143=ORIENTED_EDGE ( 'NONE', *, *, #28339, .T. ) ;
#37144=CARTESIAN_POINT ( 'NONE',  ( -124.1094910780272755, 45.33021696310842685, -22.85738008745166994 ) ) ;
#37147=CARTESIAN_POINT ( 'NONE',  ( -173.5394735271663365, 87.59446374803715685, -22.86740657428633838 ) ) ;
#37149=CARTESIAN_POINT ( 'NONE',  ( -143.8566410313463280, 59.53044870492033880, -37.35523672868243494 ) ) ;
#37150=ORIENTED_EDGE ( 'NONE', *, *, #58760, .F. ) ;
#37154=CARTESIAN_POINT ( 'NONE',  ( -133.2698123908828620, 51.54642138335024981, 39.50404384874914854 ) ) ;
#37156=CARTESIAN_POINT ( 'NONE',  ( 133.8566784816069344, 41.42467568809809109, -24.17876034193199786 ) ) ;
#37159=CARTESIAN_POINT ( 'NONE',  ( -96.43148989374458324, 29.90755650959363265, 15.89613036013473923 ) ) ;
#37160=CARTESIAN_POINT ( 'NONE',  ( -149.9130953879582364, 64.52387832078942154, -88.50193171241933499 ) ) ;
#37163=EDGE_LOOP ( 'NONE', ( #26737, #42892 ) ) ;
#37165=CARTESIAN_POINT ( 'NONE',  ( 187.8959968237854525, 85.77553094678181367, -73.71938198361095829 ) ) ;
#37168=CARTESIAN_POINT ( 'NONE',  ( 103.0124792097646349, 26.77148435100180990, -72.32543776868688212 ) ) ;
#37169=VECTOR ( 'NONE', #34297, 1000.000000000000000 ) ;
#37170=CARTESIAN_POINT ( 'NONE',  ( -78.66644367742111399, 23.39876645725287219, 30.41820113967310490 ) ) ;
#37171=CARTESIAN_POINT ( 'NONE',  ( 79.92465405224848496, 17.24122384219593584, 40.60998972530957474 ) ) ;
#37173=CARTESIAN_POINT ( 'NONE',  ( -125.8938041572051389, 47.69968343338778283, 30.61994787315706290 ) ) ;
#37174=CARTESIAN_POINT ( 'NONE',  ( 212.0047492081760936, 116.9348962082588628, 61.83128332929177873 ) ) ;
#37176=CARTESIAN_POINT ( 'NONE',  ( -106.6781182590523542, 35.07133425426476236, -9.576435181703248034 ) ) ;
#37181=CARTESIAN_POINT ( 'NONE',  ( -85.97225349031586461, 25.24026879827588132, -94.54786562133661221 ) ) ;
#37184=DIRECTION ( 'NONE',  ( 1.000000000000000000, 0.000000000000000000, -0.000000000000000000 ) ) ;
#37185=CARTESIAN_POINT ( 'NONE',  ( -156.9402586331177361, 70.74941713998435944, -95.00000000000133582 ) ) ;
#37186=CARTESIAN_POINT ( 'NONE',  ( -31.43908319763710679, -170.0000000000000000, -8.472646774738155528 ) ) ;
#37188=B_SPLINE_CURVE_WITH_KNOTS ( 'NONE', 3,
 ( #52145, #62710, #36316, #14511, #68334, #36663, #15552, #25773, #37003, #52489, #47202, #46169, #31721, #4311, #31385, #57772, #41932, #4641, #63744, #63045, #19437, #30693, #67642, #14850, #31045, #35970, #14170, #9238, #19791, #68660, #62357, #41254, #20470, #3962, #40898, #63398, #9585, #58114 ),
 .UNSPECIFIED., .F., .F.,
 ( 4, 2, 2, 2, 2, 2, 2, 2, 2, 2, 2, 2, 2, 2, 2, 2, 2, 2, 4 ),
 ( 1.551583845779545699E-17, 0.001559859933532273648, 0.003119719867064531683, 0.004679579800596789067, 0.006239439734129047753, 0.007799299667661305571, 0.008579229634427429710, 0.009359159601193552114, 0.01091901953472580039, 0.01169894950149191065, 0.01247887946825801918, 0.01403873940179021888, 0.01559859933532241859, 0.01715845926885461656, 0.01871831920238681626, 0.02027817913591901597, 0.02183803906945121567, 0.02339789900298341538, 0.02495775893651561508 ),
 .UNSPECIFIED. ) ;
#37189=DIRECTION ( 'NONE',  ( -0.8160245890732938934, -0.5780171883497599028, 0.000000000000000000 ) ) ;
#37190=ORIENTED_EDGE ( 'NONE', *, *, #33678, .F. ) ;
#37193=CARTESIAN_POINT ( 'NONE',  ( -190.6985136298601731, 109.1272424661242582, 94.99999999999866418 ) ) ;
#37194=CARTESIAN_POINT ( 'NONE',  ( 187.0823097343935331, 86.37667841017882608, 94.99999999999866418 ) ) ;
#37195=CARTESIAN_POINT ( 'NONE',  ( -1.088326810997878535, 6.545818265928947000, 34.28345951116151724 ) ) ;
#37198=ORIENTED_EDGE ( 'NONE', *, *, #49680, .T. ) ;
#37202=CARTESIAN_POINT ( 'NONE',  ( -109.7643866341847456, 37.89854104106755983, 64.31230601605615504 ) ) ;
#37204=CARTESIAN_POINT ( 'NONE',  ( -133.3944793432480367, 52.87251459353621641, -42.15878017665119870 ) ) ;
#37206=LINE ( 'NONE', #16453, #13169 ) ;
#37208=CARTESIAN_POINT ( 'NONE',  ( 90.31682503704260512, 20.71196693118262289, 70.60568123287703202 ) ) ;
#37210=CARTESIAN_POINT ( 'NONE',  ( -142.0064771034751061, 58.06937679312856204, 91.78148141502676083 ) ) ;
#37211=CARTESIAN_POINT ( 'NONE',  ( 137.3958226571047021, 43.60243650158411555, 30.38137377392774141 ) ) ;
#37214=CARTESIAN_POINT ( 'NONE',  ( 79.14113188808478583, 18.05280674635439553, 10.85844641349727624 ) ) ;
#37215=CARTESIAN_POINT ( 'NONE',  ( 163.1370549780983481, 63.50181104276883559, 5.126036944425179875 ) ) ;
#37218=CARTESIAN_POINT ( 'NONE',  ( 32.99392442438140449, 8.673943046035248017, 94.99999999999866418 ) ) ;
#37222=CARTESIAN_POINT ( 'NONE',  ( -107.0584934212648704, 35.27493744466470815, -36.71298738587253752 ) ) ;
#37223=CARTESIAN_POINT ( 'NONE',  ( 70.51484748609223630, 14.53801151001410652, -70.57721950703738401 ) ) ;
#37224=CARTESIAN_POINT ( 'NONE',  ( -60.65612136648952912, 16.25551606627059442, 42.82650858269547456 ) ) ;
#37225=CARTESIAN_POINT ( 'NONE',  ( 150.2805372522807374, 53.51147386362153924, 12.21657638438227167 ) ) ;
#37227=CARTESIAN_POINT ( 'NONE',  ( 158.3516718297675538, 59.61984652322051659, -51.08544735948212434 ) ) ;
#37230=CARTESIAN_POINT ( 'NONE',  ( 117.7417271423229863, 33.63613196344607559, -42.88727997055872265 ) ) ;
#37231=ORIENTED_EDGE ( 'NONE', *, *, #17569, .F. ) ;
#37232=CARTESIAN_POINT ( 'NONE',  ( 8.000000000000007105, 249.8719672152120381, -95.00000000000133582 ) ) ;
#37233=CARTESIAN_POINT ( 'NONE',  ( 134.7770330630253000, 41.98246829846534922, 71.31249374605413038 ) ) ;
#37234=CARTESIAN_POINT ( 'NONE',  ( -173.9526029538035914, 89.57590038685106038, 30.85607633362990398 ) ) ;
#37235=CARTESIAN_POINT ( 'NONE',  ( -35.38560449531986762, 10.27249159032102810, -76.04409089915343145 ) ) ;
#37238=CARTESIAN_POINT ( 'NONE',  ( 45.04020069093783007, 10.22779424730543241, 15.53914219526992468 ) ) ;
#37243=CARTESIAN_POINT ( 'NONE',  ( -62.52556685097597722, 16.81334402605504508, 90.59652277792575603 ) ) ;
#37245=CARTESIAN_POINT ( 'NONE',  ( -155.7495771807047618, 69.65980221699318520, -73.34527921935438144 ) ) ;
#37247=FACE_OUTER_BOUND ( 'NONE', #19237, .T. ) ;
#37253=CARTESIAN_POINT ( 'NONE',  ( -71.97171223898808989, 20.94894057408426491, 68.18058196594357412 ) ) ;
#37254=CARTESIAN_POINT ( 'NONE',  ( 207.8675797643809631, 110.7908513421272119, -63.86012885756652224 ) ) ;
#37256=CARTESIAN_POINT ( 'NONE',  ( -74.17694007417655655, 20.66176641130876135, 17.10122609394768389 ) ) ;
#37258=CARTESIAN_POINT ( 'NONE',  ( 19.54326199789021601, 7.657220834818549093, 31.01773977966792728 ) ) ;
#37260=CARTESIAN_POINT ( 'NONE',  ( 197.1968910587178243, 96.59211440045608299, 90.83512555983344328 ) ) ;
#37263=CARTESIAN_POINT ( 'NONE',  ( -75.00168449119591685, 20.95943092127968654, 71.31086889332340206 ) ) ;
#37265=ORIENTED_EDGE ( 'NONE', *, *, #48372, .T. ) ;
#37268=CARTESIAN_POINT ( 'NONE',  ( -31.43908319763709969, 10.61114334766716105, -23.47264677473818395 ) ) ;
#37270=PLANE ( 'NONE',  #42378 ) ;
#37277=CARTESIAN_POINT ( 'NONE',  ( -133.1566699306513613, 52.70203339370771545, 36.22971255361426302 ) ) ;
#37278=ORIENTED_EDGE ( 'NONE', *, *, #60960, .F. ) ;
#37279=CARTESIAN_POINT ( 'NONE',  ( 204.6977192012829789, 106.3443248447423315, 17.36317014830577321 ) ) ;
#37280=CARTESIAN_POINT ( 'NONE',  ( -144.7530445311634537, 61.54314312182905411, 32.41526756990536740 ) ) ;
#37281=CARTESIAN_POINT ( 'NONE',  ( 61.09275639403233527, 12.23448398202909893, 56.89203593337313691 ) ) ;
#37290=DIRECTION ( 'NONE',  ( -0.000000000000000000, 1.000000000000000000, -0.000000000000000000 ) ) ;
#37291=CARTESIAN_POINT ( 'NONE',  ( -166.7049310409072689, 80.25944422923579680, -11.47475090231446160 ) ) ;
#37293=CARTESIAN_POINT ( 'NONE',  ( -0.4996266546846081513, 7.531422798935177632, -95.00000000000133582 ) ) ;
#37294=CARTESIAN_POINT ( 'NONE',  ( 17.42558916372104250, 7.565465075731206746, 83.87742723891268781 ) ) ;
#37297=CARTESIAN_POINT ( 'NONE',  ( -95.86612279493098754, 29.64021615886204941, 68.75908302673695971 ) ) ;
#37300=CARTESIAN_POINT ( 'NONE',  ( -71.67841390531688717, 19.78168466957075466, 35.18329047664818177 ) ) ;
#37305=CARTESIAN_POINT ( 'NONE',  ( -122.1940143064357187, 45.29738883755585732, 17.80353666295016879 ) ) ;
#37307=CARTESIAN_POINT ( 'NONE',  ( -178.2427210808089058, 93.01567669683340966, 59.68194965257550422 ) ) ;
#37308=CARTESIAN_POINT ( 'NONE',  ( 126.3737790127712799, 37.08609730334949006, 64.42584544384298795 ) ) ;
#37310=EDGE_LOOP ( 'NONE', ( #32427, #36216, #38483, #31559 ) ) ;
#37311=CARTESIAN_POINT ( 'NONE',  ( -24.69950091090638722, 8.581800362251172487, 94.71242551333074289 ) ) ;
#37312=CARTESIAN_POINT ( 'NONE',  ( 155.7262569076171985, 56.30477153194512852, 44.25956702222304529 ) ) ;
#37317=CARTESIAN_POINT ( 'NONE',  ( -24.07146903340143140, 8.497560047608727629, 39.18234541147268857 ) ) ;
#37322=FACE_BOUND ( 'NONE', #13442, .T. ) ;
#37325=CARTESIAN_POINT ( 'NONE',  ( -80.31482177285911916, 24.03632224640839610, -76.78049980088347581 ) ) ;
#37327=CARTESIAN_POINT ( 'NONE',  ( -122.3994536713185255, 45.42826354555016621, -35.77335078514256850 ) ) ;
#37329=CARTESIAN_POINT ( 'NONE',  ( 132.7179291807801178, 40.74118679001691135, 2.749225463022159310 ) ) ;
#37331=DIRECTION ( 'NONE',  ( 0.000000000000000000, 0.000000000000000000, 1.000000000000000000 ) ) ;
#37334=CARTESIAN_POINT ( 'NONE',  ( 89.88147981065579017, 21.62466191578950614, -9.701577234200509992 ) ) ;
#37336=CARTESIAN_POINT ( 'NONE',  ( -38.17232309348612773, 11.81874355808868238, 14.21233894131476738 ) ) ;
#37338=CARTESIAN_POINT ( 'NONE',  ( -78.66644367742111399, -170.0000000000000000, -76.96000122218160300 ) ) ;
#37340=CARTESIAN_POINT ( 'NONE',  ( 20.36233635256088803, 7.697399815318436644, -75.82726962297421380 ) ) ;
#37343=LINE ( 'NONE', #43306, #36716 ) ;
#37344=CARTESIAN_POINT ( 'NONE',  ( 141.3036441389950824, 47.31002705502927341, -44.56327115119219684 ) ) ;
#37347=CARTESIAN_POINT ( 'NONE',  ( -31.43908319763710679, -170.0000000000000000, 91.40555558711655237 ) ) ;
#37349=EDGE_LOOP ( 'NONE', ( #282, #68241, #57694, #61140 ) ) ;
#37350=CARTESIAN_POINT ( 'NONE',  ( 66.08620257826613908, 13.40585338179127284, -36.37378492149262144 ) ) ;
#37352=CARTESIAN_POINT ( 'NONE',  ( 126.8188448246704780, 38.48775085959175613, -94.58402359101047807 ) ) ;
#37358=CARTESIAN_POINT ( 'NONE',  ( -15.22871623201694291, 7.486724405784663361, 63.23486717562329318 ) ) ;
#37359=CARTESIAN_POINT ( 'NONE',  ( -79.14678386417814693, 22.50468917936073510, -8.270900041254199309 ) ) ;
#37363=CARTESIAN_POINT ( 'NONE',  ( 46.90141780929663184, 9.503798448769773088, -16.77990280306253013 ) ) ;
#37366=CARTESIAN_POINT ( 'NONE',  ( 164.9700808964341547, 65.04346068891115351, 64.04275777180556872 ) ) ;
#37374=CARTESIAN_POINT ( 'NONE',  ( 151.6178224291901415, 54.48737267587420519, 68.45106349240374755 ) ) ;
#37376=CARTESIAN_POINT ( 'NONE',  ( 151.6192474229130198, 53.24103268919207466, 5.366030440576345484 ) ) ;
#37377=CARTESIAN_POINT ( 'NONE',  ( -9.123606769528260330, 7.986935641101333694, 83.88886893069803818 ) ) ;
#37386=CARTESIAN_POINT ( 'NONE',  ( 45.80999061969644970, 10.34829880103435507, 94.99999999999866418 ) ) ;
#37391=CARTESIAN_POINT ( 'NONE',  ( -56.02027488966933078, 14.94257193099085868, -62.10801344035115790 ) ) ;
#37392=CARTESIAN_POINT ( 'NONE',  ( -4.731197926646204088, 7.716745361328044339, 3.934633056432215614 ) ) ;
#37394=CARTESIAN_POINT ( 'NONE',  ( 174.4978817191264682, 73.57770570413205746, -47.32325019632195762 ) ) ;
#37395=CARTESIAN_POINT ( 'NONE',  ( -152.2873556200145799, 67.91256772393732888, -76.12667896378731314 ) ) ;
#37401=CARTESIAN_POINT ( 'NONE',  ( 9.050324533885207856, 7.384616180193988910, 34.18438138347604394 ) ) ;
#37403=FACE_OUTER_BOUND ( 'NONE', #40618, .T. ) ;
#37405=VERTEX_POINT ( 'NONE', #68371 ) ;
#37418=CARTESIAN_POINT ( 'NONE',  ( 150.5550643769628039, 52.46819381604268528, -73.38422485962182407 ) ) ;
#37419=CARTESIAN_POINT ( 'NONE',  ( 22.29513692215318343, 6.796052026456518291, -19.93622960288293200 ) ) ;
#37421=CYLINDRICAL_SURFACE ( 'NONE', #64343, 7.500000000000013323 ) ;
#37425=B_SPLINE_CURVE_WITH_KNOTS ( 'NONE', 3,
 ( #11583, #58393, #53452, #5284, #43243, #43599, #59769, #21128, #42899, #32025, #11240, #42572, #26742, #32708, #64361, #53107, #59428, #48511, #22155, #27420, #54493, #15838, #16530, #38325, #340, #22502, #32370, #15505, #43939, #58731, #16177, #27774, #49216, #5617, #64029, #64719, #65068, #37632, #16867, #59081, #37281, #10899, #37985, #1051 ),
 .UNSPECIFIED., .F., .F.,
 ( 4, 2, 2, 2, 2, 2, 2, 2, 2, 2, 2, 2, 2, 2, 2, 2, 2, 2, 2, 2, 2, 4 ),
 ( 1.430489624538199204E-17, 0.001482469635030033046, 0.002223704452545043064, 0.002964939270060053082, 0.004447408905090053169, 0.005929878540120054123, 0.007412348175150054209, 0.008153582992665062493, 0.008894817810180068174, 0.01037728744521007954, 0.01185975708024009263, 0.01260099189775507923, 0.01334222671527006236, 0.01482469635030007372, 0.01556593116781507594, 0.01630716598533007641, 0.01778963562036007043, 0.01927210525539006097, 0.02001334007290505798, 0.02075457489042005152, 0.02223704452545007329, 0.02371951416048009159 ),
 .UNSPECIFIED. ) ;
#37426=CARTESIAN_POINT ( 'NONE',  ( -62.33646982747445264, 17.80738194613631364, -94.56263670386991294 ) ) ;
#37428=CARTESIAN_POINT ( 'NONE',  ( -23.94843400007326295, 9.496257175156115338, 91.90182630676891051 ) ) ;
#37429=CARTESIAN_POINT ( 'NONE',  ( 116.8917656767876281, 33.20682060519246903, -13.09834932968690246 ) ) ;
#37430=CARTESIAN_POINT ( 'NONE',  ( 185.1802655733641529, 82.84606286178495793, -37.42643899651594808 ) ) ;
#37431=CARTESIAN_POINT ( 'NONE',  ( 23.03578842369135060, 6.840884649289439956, 35.56935612319515627 ) ) ;
#37435=ORIENTED_EDGE ( 'NONE', *, *, #60991, .F. ) ;
#37436=CARTESIAN_POINT ( 'NONE',  ( -156.3734885497381697, 71.59531449004288106, -18.49822134472886148 ) ) ;
#37437=CARTESIAN_POINT ( 'NONE',  ( 33.31166872005966439, 8.707041209322245123, -47.50374935772406104 ) ) ;
#37438=CARTESIAN_POINT ( 'NONE',  ( -31.92580063159127590, 9.671320706097198183, 57.06100499665285497 ) ) ;
#37439=CARTESIAN_POINT ( 'NONE',  ( 39.40195752203892710, -170.0000000000000000, 64.25838489642696061 ) ) ;
#37442=CARTESIAN_POINT ( 'NONE',  ( 157.4703587214989113, 58.92748579479258808, 2.564916881789689462 ) ) ;
#37444=CARTESIAN_POINT ( 'NONE',  ( 20.36233635256088093, 7.697399815318435756, 4.706382148416831335 ) ) ;
#37447=CARTESIAN_POINT ( 'NONE',  ( -85.91089317961402116, 25.21459833389209848, -44.62272628199698232 ) ) ;
#37448=CARTESIAN_POINT ( 'NONE',  ( 20.37135563017389117, 6.690359945346087578, 70.31641744500336699 ) ) ;
#37450=CARTESIAN_POINT ( 'NONE',  ( 13.37366753069833436, 6.435102282077987290, -76.98119335383468353 ) ) ;
#37458=CARTESIAN_POINT ( 'NONE',  ( -103.2061297292849389, 34.38496953192504435, -49.97177337113672735 ) ) ;
#37459=CARTESIAN_POINT ( 'NONE',  ( 57.41085175769455873, 12.46982565415946986, -75.05494575928295831 ) ) ;
#37464=CARTESIAN_POINT ( 'NONE',  ( -23.93965512371324422, 8.480096402797085986, -16.47769234035476771 ) ) ;
#37467=CARTESIAN_POINT ( 'NONE',  ( 201.5876148766343761, 103.8397408698165520, 16.70131438898428300 ) ) ;
#37469=VERTEX_POINT ( 'NONE', #14550 ) ;
#37472=CARTESIAN_POINT ( 'NONE',  ( 117.3281529665581928, 32.29994712002883261, 66.46847310579148882 ) ) ;
#37474=CARTESIAN_POINT ( 'NONE',  ( 113.4402889550712672, 31.50582881646777622, 70.75682576111141486 ) ) ;
#37477=CARTESIAN_POINT ( 'NONE',  ( 141.3556389957210229, 47.34429831367556574, 64.15079552814040653 ) ) ;
#37481=CARTESIAN_POINT ( 'NONE',  ( 162.8721509409114105, 61.97589144837539976, -92.09519880210693543 ) ) ;
#37482=CARTESIAN_POINT ( 'NONE',  ( 92.19920907511531993, 21.39700525884452986, -48.36761472064368661 ) ) ;
#37485=EDGE_LOOP ( 'NONE', ( #61601, #3341, #42407, #12665 ) ) ;
#37486=CARTESIAN_POINT ( 'NONE',  ( -122.3963566076408256, 44.23346594671848209, -22.22042909780819642 ) ) ;
#37488=CARTESIAN_POINT ( 'NONE',  ( -180.0175713311536185, 95.14770835574074681, -18.32925981149572081 ) ) ;
#37489=B_SPLINE_CURVE_WITH_KNOTS ( 'NONE', 3,
 ( #19026, #30627, #8833, #62639, #14781, #47132, #51731, #13749, #30975, #40478, #41179, #35207, #68595, #29930, #36245, #25361, #51396, #3209, #57702, #41522, #9166, #24664, #20400, #3889, #46099, #62282, #35903, #67568, #19368, #46796, #41869, #40826, #14448, #52073, #14097, #68265, #20068, #62975, #63325, #29575, #15133, #36595, #51041, #58041 ),
 .UNSPECIFIED., .F., .F.,
 ( 4, 2, 2, 2, 2, 2, 2, 2, 2, 2, 2, 2, 2, 2, 2, 2, 2, 2, 2, 2, 2, 4 ),
 ( 0.02477387709520258857, 0.02633314402883777869, 0.02711277749565536854, 0.02789241096247295840, 0.02945167789610817974, 0.03023131136292576959, 0.03101094482974336292, 0.03257021176337852875, 0.03334984523019610125, 0.03412947869701367376, 0.03568874563064881877, 0.03646837909746639128, 0.03724801256428395685, 0.03802764603110153629, 0.03880727949791912268, 0.04036654643155428851, 0.04192581336518945434, 0.04348508029882461323, 0.04504434723245977212, 0.04660361416609493795, 0.04816288109973010378, 0.04972214803336526268 ),
 .UNSPECIFIED. ) ;
#37490=CARTESIAN_POINT ( 'NONE',  ( -165.9154624515709884, 80.89088623112731113, -66.95487838069742281 ) ) ;
#37491=CARTESIAN_POINT ( 'NONE',  ( -145.5261806899007411, 60.87473129144527917, -48.67308456771189640 ) ) ;
#37493=CARTESIAN_POINT ( 'NONE',  ( 57.39233401791015865, 12.46575990788836918, 15.45527492068149122 ) ) ;
#37496=DIRECTION ( 'NONE',  ( -0.000000000000000000, 1.000000000000000000, -0.000000000000000000 ) ) ;
#37498=CARTESIAN_POINT ( 'NONE',  ( 86.62931800182293784, 19.42108912189597447, -23.97701360844805407 ) ) ;
#37499=CARTESIAN_POINT ( 'NONE',  ( -126.3453033442920344, 47.99870040347948930, -76.75825448869764500 ) ) ;
#37501=CARTESIAN_POINT ( 'NONE',  ( 62.60845276312630858, 12.57833377949302189, -89.40979201309711755 ) ) ;
#37503=CARTESIAN_POINT ( 'NONE',  ( -96.43148989374459745, 29.90755650959362910, -64.63752141125630146 ) ) ;
#37504=VERTEX_POINT ( 'NONE', #19476 ) ;
#37507=CARTESIAN_POINT ( 'NONE',  ( 182.5617509987553717, 80.11195108039724744, -77.92569941903248321 ) ) ;
#37509=CARTESIAN_POINT ( 'NONE',  ( -165.7143741370936709, 79.24519349471955820, -43.42972967134339513 ) ) ;
#37513=CARTESIAN_POINT ( 'NONE',  ( -71.86568654225716557, 20.91200104397925230, 34.74601522620152849 ) ) ;
#37514=CARTESIAN_POINT ( 'NONE',  ( 80.16939877002758408, 17.31693935407229290, 41.05451173327999470 ) ) ;
#37517=CARTESIAN_POINT ( 'NONE',  ( 43.14669449386823175, 9.942681284149132992, -36.60324319909982194 ) ) ;
#37519=VERTEX_POINT ( 'NONE', #40937 ) ;
#37520=CARTESIAN_POINT ( 'NONE',  ( -107.7743374187917027, 35.66028478413600311, -10.54119851968185095 ) ) ;
#37522=CARTESIAN_POINT ( 'NONE',  ( -15.26524495591509023, 7.490231452641286758, -43.89783010401615115 ) ) ;
#37526=CARTESIAN_POINT ( 'NONE',  ( 110.7117404013331026, 30.20916032354564251, 2.766663615273644350 ) ) ;
#37530=CARTESIAN_POINT ( 'NONE',  ( -102.2801239173131052, 33.91021738430207222, -8.170026674512225640 ) ) ;
#37531=VERTEX_POINT ( 'NONE', #42320 ) ;
#37532=CARTESIAN_POINT ( 'NONE',  ( 210.6189312023034574, 114.8321746285510301, 94.99999999999866418 ) ) ;
#37536=CARTESIAN_POINT ( 'NONE',  ( 13.84704553156522167, 7.452804552247572545, -77.11207471772274857 ) ) ;
#37539=CARTESIAN_POINT ( 'NONE',  ( 110.2429982417149574, -170.0000000000000000, 37.11121420573731911 ) ) ;
#37540=CARTESIAN_POINT ( 'NONE',  ( -7.825402957745083654, 6.891034867348166060, 30.11558103944718923 ) ) ;
#37543=CARTESIAN_POINT ( 'NONE',  ( 91.71454558664912327, 22.29094817986854693, 85.37844496027901187 ) ) ;
#37550=B_SPLINE_CURVE_WITH_KNOTS ( 'NONE', 3,
 ( #46772, #45387, #67547, #35181, #56286, #51019, #29552, #8456, #3868, #34510, #30260, #2828, #25335, #67218, #69163, #56990, #20988, #41157, #19345, #29909, #50663, #24297, #24643, #46076, #13388, #63896, #62256, #40456, #14071, #35536, #67897, #62617, #8808, #51709, #3515, #24986 ),
 .UNSPECIFIED., .F., .F.,
 ( 4, 2, 2, 2, 2, 2, 2, 2, 2, 2, 2, 2, 2, 2, 2, 2, 2, 4 ),
 ( 0.000000000000000000, 0.001548367318450182602, 0.003096734636900365205, 0.004645101955350548241, 0.006193469273800730410, 0.007741836592250906507, 0.008516020251475981545, 0.009290203910701058318, 0.01083857122915121186, 0.01238693854760136194, 0.01393530586605151375, 0.01548367318450166730, 0.01703204050295181737, 0.01858040782140197092, 0.02012877513985212447, 0.02167714245830228148, 0.02322550977675243503, 0.02477387709520259204 ),
 .UNSPECIFIED. ) ;
#37551=CARTESIAN_POINT ( 'NONE',  ( -102.7447593990059147, 34.14748189312169302, 57.36362509687879907 ) ) ;
#37552=CARTESIAN_POINT ( 'NONE',  ( -132.6092625803567273, 52.31125232006264270, -39.06397555526168475 ) ) ;
#37555=CARTESIAN_POINT ( 'NONE',  ( -7.825402957745083654, 6.891034867348163395, -23.57352014148015584 ) ) ;
#37556=CARTESIAN_POINT ( 'NONE',  ( 199.9103251464698872, 101.6434290204575319, -11.20346956314359943 ) ) ;
#37559=CARTESIAN_POINT ( 'NONE',  ( 134.7697261969508986, 41.97802808873667857, 29.55217423902721663 ) ) ;
#37563=CARTESIAN_POINT ( 'NONE',  ( 84.97658021689284169, 19.92447159015900837, 3.047988274556576727 ) ) ;
#37564=ADVANCED_FACE ( 'NONE', ( #12042 ), #32113, .F. ) ;
#37565=B_SPLINE_CURVE_WITH_KNOTS ( 'NONE', 3,
 ( #42379, #30798, #52245, #25532, #37100, #58541, #51564, #14275, #3373, #24827, #46268, #19543, #41006, #38132, #5769, #16337, #31826, #26552, #148, #37436, #43054, #5087, #60294, #32862, #59927, #64878, #857, #33225, #22655, #21957, #47985, #65579, #54295, #64173, #48316, #43404, #53610, #69451, #17371, #37791, #27931, #21608, #27579, #11053, #21267, #6118, #16678, #17014 ),
 .UNSPECIFIED., .F., .F.,
 ( 4, 2, 2, 2, 2, 2, 2, 2, 2, 2, 2, 2, 2, 2, 2, 2, 2, 2, 2, 2, 2, 2, 2, 4 ),
 ( 0.02698595842317762575, 0.02784423243973407555, 0.02870250645629052189, 0.03041905448940333129, 0.03127732850595971864, 0.03213560252251611293, 0.03385215055562888764, 0.03471042457218524030, 0.03556869858874159990, 0.03728524662185429828, 0.03814352063841063012, 0.03900179465496696196, 0.03986006867152329380, 0.04071834268807963259, 0.04157661670463596443, 0.04243489072119230321, 0.04415143875430497383, 0.04500971277086131261, 0.04586798678741765833, 0.04758453482053030814, 0.04930108285364295795, 0.05101763088675561469, 0.05273417891986827144, 0.05445072695298092125 ),
 .UNSPECIFIED. ) ;
#37566=CARTESIAN_POINT ( 'NONE',  ( 164.1338586910085837, 64.33646242148860495, 13.51726694518641381 ) ) ;
#37568=AXIS2_PLACEMENT_3D ( 'NONE', #45333, #34101, #2095 ) ;
#37569=EDGE_LOOP ( 'NONE', ( #7820, #45569, #34490, #35920 ) ) ;
#37574=CARTESIAN_POINT ( 'NONE',  ( -108.6909373351217596, 36.15835109565443162, -46.43893206896224513 ) ) ;
#37575=CARTESIAN_POINT ( 'NONE',  ( 63.98009977735161158, 12.89803120691696670, -77.51887576910404221 ) ) ;
#37576=VECTOR ( 'NONE', #69486, 1000.000000000000000 ) ;
#37577=CARTESIAN_POINT ( 'NONE',  ( -59.36813706141739999, 15.88103696331963377, 43.95624469312958382 ) ) ;
#37582=DIRECTION ( 'NONE',  ( 0.000000000000000000, 0.000000000000000000, 1.000000000000000000 ) ) ;
#37583=VERTEX_POINT ( 'NONE', #32801 ) ;
#37586=CARTESIAN_POINT ( 'NONE',  ( -166.2028657618940883, 79.74389853943291939, 41.23225120243120756 ) ) ;
#37587=CARTESIAN_POINT ( 'NONE',  ( 126.3554864210862121, 38.22801630372152459, 64.08286055307904405 ) ) ;
#37594=CARTESIAN_POINT ( 'NONE',  ( 70.52164504723299387, 14.53981718869930084, 90.84488468013880436 ) ) ;
#37596=CARTESIAN_POINT ( 'NONE',  ( -24.09190246691234805, 8.500289797445409690, -95.00000000000133582 ) ) ;
#37602=CARTESIAN_POINT ( 'NONE',  ( -73.09214866197369531, 21.34321757515763807, 59.72063747903552411 ) ) ;
#37603=CARTESIAN_POINT ( 'NONE',  ( 209.6525588430077960, 113.3929734759396695, -76.30558542174757974 ) ) ;
#37607=CARTESIAN_POINT ( 'NONE',  ( -37.22864127331250472, 10.61359798105728913, -91.73382525222255879 ) ) ;
#37608=CARTESIAN_POINT ( 'NONE',  ( 22.51798020284706325, 7.817376421459703018, 34.19479625308969872 ) ) ;
#37609=DIRECTION ( 'NONE',  ( -0.000000000000000000, 1.000000000000000000, -0.000000000000000000 ) ) ;
#37616=EDGE_LOOP ( 'NONE', ( #49149, #55927, #48762, #48991 ) ) ;
#37618=CARTESIAN_POINT ( 'NONE',  ( -24.60892750534350526, 9.584951112520235128, -72.76977437635076740 ) ) ;
#37620=CARTESIAN_POINT ( 'NONE',  ( 55.52750043885181697, 11.05966813607792254, -43.71057030527602905 ) ) ;
#37623=CARTESIAN_POINT ( 'NONE',  ( -147.7860806339124906, 62.73248524776227697, 4.063553114042554704 ) ) ;
#37624=EDGE_CURVE ( 'NONE', #1332, #47869, #42724, .T. ) ;
#37625=ORIENTED_EDGE ( 'NONE', *, *, #50831, .T. ) ;
#37627=EDGE_LOOP ( 'NONE', ( #6468, #60078, #59176, #13520 ) ) ;
#37631=CARTESIAN_POINT ( 'NONE',  ( -142.3187766126155225, 59.59460822661993262, 36.01124715683158684 ) ) ;
#37632=CARTESIAN_POINT ( 'NONE',  ( 59.72897338775219112, 11.93428797217974946, 57.41156910716014750 ) ) ;
#37633=CARTESIAN_POINT ( 'NONE',  ( 133.8566784816069344, -170.0000000000000000, -70.36786152285935714 ) ) ;
#37640=CARTESIAN_POINT ( 'NONE',  ( 160.4963793545269084, 60.04225845346908841, -23.65658366629068254 ) ) ;
#37644=CARTESIAN_POINT ( 'NONE',  ( 68.93219921887764201, 14.12322281954859982, 32.69723793727709449 ) ) ;
#37645=CARTESIAN_POINT ( 'NONE',  ( -190.6985136298601731, 109.1272424661242582, -73.40678087856149148 ) ) ;
#37647=CARTESIAN_POINT ( 'NONE',  ( 80.73012746365752434, 17.49169339352364716, 15.02525433145232192 ) ) ;
#37649=CARTESIAN_POINT ( 'NONE',  ( -72.78737098446268305, 20.16853011470087864, 33.23444075940503240 ) ) ;
#37653=VERTEX_POINT ( 'NONE', #40504 ) ;
#37654=CARTESIAN_POINT ( 'NONE',  ( -121.1841775822198457, 44.65790002524552449, 5.417918675821312924 ) ) ;
#37656=CARTESIAN_POINT ( 'NONE',  ( 128.3856248084844651, 38.21741401878865219, 58.70131835549462096 ) ) ;
#37663=CARTESIAN_POINT ( 'NONE',  ( -173.1211646369891071, 88.63826465341152527, -61.55650775521367279 ) ) ;
#37665=CARTESIAN_POINT ( 'NONE',  ( 70.51583798635768119, 15.57951509147424041, 37.07105218285969528 ) ) ;
#37668=LINE ( 'NONE', #5650, #67577 ) ;
#37670=CARTESIAN_POINT ( 'NONE',  ( -142.1332311300253366, 59.44822332309654200, -70.55302544014286070 ) ) ;
#37674=CARTESIAN_POINT ( 'NONE',  ( -179.8989115484067440, 96.59045402602914976, 68.38918859239640824 ) ) ;
#37676=CARTESIAN_POINT ( 'NONE',  ( -102.2801239173131052, 32.78103895658057354, -61.85912785543958847 ) ) ;
#37678=CARTESIAN_POINT ( 'NONE',  ( -85.75002235020436103, 26.23806300442549144, 13.55091505814834640 ) ) ;
#37681=CARTESIAN_POINT ( 'NONE',  ( -124.1007047332778228, 46.52282960291164926, -76.55490961030825758 ) ) ;
#37683=CARTESIAN_POINT ( 'NONE',  ( -85.75002235020438945, 26.23806300442547723, 67.24001623907572878 ) ) ;
#37684=CARTESIAN_POINT ( 'NONE',  ( 89.87840278991590992, 21.62393877508909767, -23.24105151053815632 ) ) ;
#37686=CARTESIAN_POINT ( 'NONE',  ( -37.93983213483221562, 11.77368372188051282, 14.64435496287500449 ) ) ;
#37689=ORIENTED_EDGE ( 'NONE', *, *, #52016, .F. ) ;
#37690=CARTESIAN_POINT ( 'NONE',  ( 19.10949903373832370, 7.636938177523840743, -76.59253534108344752 ) ) ;
#37691=CARTESIAN_POINT ( 'NONE',  ( 113.6770630153551167, 31.62064605900739167, 84.12484067033027202 ) ) ;
#37693=CARTESIAN_POINT ( 'NONE',  ( 67.93926590385572695, 13.86859831467923598, -10.69750007213145082 ) ) ;
#37694=CARTESIAN_POINT ( 'NONE',  ( -27.70115495247213389, 10.02455692117576369, -36.29670080177614011 ) ) ;
#37695=CARTESIAN_POINT ( 'NONE',  ( -49.43836229152577033, 14.28302414152160082, -74.55831633533836111 ) ) ;
#37696=CARTESIAN_POINT ( 'NONE',  ( -75.37792209610570637, 22.16719325496249482, -89.55030856586989785 ) ) ;
#37698=VERTEX_POINT ( 'NONE', #22946 ) ;
#37704=CARTESIAN_POINT ( 'NONE',  ( -168.1839487819771080, 83.25723186408069409, 70.81687309716325274 ) ) ;
#37713=CARTESIAN_POINT ( 'NONE',  ( 188.4365915667138438, 87.87248959723055464, -15.37144753093564908 ) ) ;
#37715=CARTESIAN_POINT ( 'NONE',  ( -79.52000911032672548, 23.72680920995770038, -88.84120912474600118 ) ) ;
#37719=CARTESIAN_POINT ( 'NONE',  ( 164.0105905242218114, 64.23277447906892235, 60.07396046421560243 ) ) ;
#37721=B_SPLINE_CURVE_WITH_KNOTS ( 'NONE', 3,
 ( #16477, #16165, #52428, #63678, #47828, #9871, #4251, #47476, #69288, #15143, #32359, #21116, #25711, #27061, #42218, #47140, #20408, #36944, #58721, #68934, #53095, #4923, #37620, #10888, #41876, #32013, #5271, #26731, #63333, #21441, #42887, #36602, #53783, #5605, #20077, #41531, #62982, #58050, #28467, #1384, #59757, #44648, #39372, #48495 ),
 .UNSPECIFIED., .F., .F.,
 ( 4, 2, 2, 2, 2, 2, 2, 2, 2, 2, 2, 2, 2, 2, 2, 2, 2, 2, 2, 2, 2, 4 ),
 ( 1.734723475976807094E-18, 0.001482469635030026541, 0.002223704452545041763, 0.002964939270060056552, 0.004447408905090094802, 0.005929878540120132185, 0.007412348175150170436, 0.008153582992665182189, 0.008894817810180194809, 0.01037728744521020791, 0.01185975708024022274, 0.01260099189775521974, 0.01334222671527021502, 0.01482469635030021077, 0.01556593116781520431, 0.01630716598533020478, 0.01778963562036018492, 0.01927210525539016506, 0.02001334007290515860, 0.02075457489042015213, 0.02223704452545011839, 0.02371951416048008465 ),
 .UNSPECIFIED. ) ;
#37727=CARTESIAN_POINT ( 'NONE',  ( 151.1700480242206481, 54.15904440870136938, 67.83133139760614938 ) ) ;
#37732=CARTESIAN_POINT ( 'NONE',  ( -11.27383957674984849, 8.149435916118470402, 84.63656658335857230 ) ) ;
#37735=CARTESIAN_POINT ( 'NONE',  ( 39.40195752203892710, -170.0000000000000000, -16.27526687496408542 ) ) ;
#37740=CARTESIAN_POINT ( 'NONE',  ( 92.20490818459941806, 22.47175429302963323, -65.12600615666283943 ) ) ;
#37743=CARTESIAN_POINT ( 'NONE',  ( -1.862553927312058821, 7.582910205528085257, 6.195710318879104506 ) ) ;
#37744=CARTESIAN_POINT ( 'NONE',  ( 181.0840389613909451, 80.03940679743416808, -36.22505766587961062 ) ) ;
#37745=CARTESIAN_POINT ( 'NONE',  ( -150.5993571094983281, 66.43939758484179947, -76.58067256224735786 ) ) ;
#37746=CARTESIAN_POINT ( 'NONE',  ( 88.98408042523109884, 20.23787745328939280, 30.08728822265231884 ) ) ;
#37749=CARTESIAN_POINT ( 'NONE',  ( -48.58011387679027848, 14.07568064779664141, -46.51327318317784432 ) ) ;
#37752=CARTESIAN_POINT ( 'NONE',  ( 9.819093282782489496, 7.389085782749409859, 42.08183418655492147 ) ) ;
#37753=CARTESIAN_POINT ( 'NONE',  ( 66.90836167404864909, 13.60846798854640127, -90.44605171876324334 ) ) ;
#37754=CARTESIAN_POINT ( 'NONE',  ( -82.50457182857807936, 24.90487912293252037, 85.15644553449918419 ) ) ;
#37762=CARTESIAN_POINT ( 'NONE',  ( -14.92903005859421306, 7.458185427130748835, -13.65509502686643195 ) ) ;
#37763=CARTESIAN_POINT ( 'NONE',  ( -167.3263409977197398, 82.35496590386728144, 87.23955561701365014 ) ) ;
#37764=CARTESIAN_POINT ( 'NONE',  ( 151.3976820382521851, 53.07948349322499837, 94.99999999999866418 ) ) ;
#37769=CARTESIAN_POINT ( 'NONE',  ( -55.54036735998995766, 15.85474597822063636, -35.21632399845986328 ) ) ;
#37770=CARTESIAN_POINT ( 'NONE',  ( -9.765753193741730342, 8.033970690975920093, -23.32232872259482548 ) ) ;
#37771=CARTESIAN_POINT ( 'NONE',  ( 154.4429418375333114, 55.33424769452792447, -77.34545030156257894 ) ) ;
#37772=CARTESIAN_POINT ( 'NONE',  ( 20.37135563017390183, 6.690359945346087578, -10.21723432638768614 ) ) ;
#37777=ORIENTED_EDGE ( 'NONE', *, *, #413, .F. ) ;
#37781=CARTESIAN_POINT ( 'NONE',  ( 117.5606268127798160, 32.41702750294250990, 92.48114496397971607 ) ) ;
#37782=CARTESIAN_POINT ( 'NONE',  ( -155.1359377029285724, 70.46175948311801562, 16.35866617282277602 ) ) ;
#37783=CARTESIAN_POINT ( 'NONE',  ( 188.2133404574782389, 86.12414067617876867, -41.37883977796289514 ) ) ;
#37784=CARTESIAN_POINT ( 'NONE',  ( 20.74093720376649586, 6.709541214524347374, 31.86137974890134572 ) ) ;
#37785=CARTESIAN_POINT ( 'NONE',  ( -156.8713506010090839, 72.05569703773764445, 93.37478388102675808 ) ) ;
#37787=ADVANCED_FACE ( 'NONE', ( #34896 ), #12392, .F. ) ;
#37791=CARTESIAN_POINT ( 'NONE',  ( -154.0833774771448645, 69.51012195447351871, -9.506901666534069761 ) ) ;
#37792=CARTESIAN_POINT ( 'NONE',  ( 35.66087318222940894, 8.964867769223234362, -49.63888608646336564 ) ) ;
#37794=CARTESIAN_POINT ( 'NONE',  ( -36.37663950036512261, 10.45389057208229033, 70.22755886848516127 ) ) ;
#37795=CARTESIAN_POINT ( 'NONE',  ( 197.9868529032975459, 99.18611233336800126, 60.19158866520284334 ) ) ;
#37797=B_SPLINE_CURVE_WITH_KNOTS ( 'NONE', 3,
 ( #11463, #7258, #66017, #12887, #49444, #60712, #28000, #23087, #6896, #33649, #54730, #22032, #38922, #55077, #60002, #38211, #12185, #17813, #28714, #18155, #17445, #28353, #6556, #43476, #49799, #1624, #11824, #59648, #33300, #43821, #44536, #50160, #1276, #22734, #65297, #66365, #44168, #65654, #39609, #32931, #39268, #12527, #54372, #33990 ),
 .UNSPECIFIED., .F., .F.,
 ( 4, 2, 2, 2, 2, 2, 2, 2, 2, 2, 2, 2, 2, 2, 2, 2, 2, 2, 2, 2, 2, 4 ),
 ( 0.000000000000000000, 0.004120577325733526357, 0.006180865988600314255, 0.008241154651467101286, 0.01030144331433388918, 0.01133158764576725278, 0.01236173197720061984, 0.01339187630863398343, 0.01442202064006734875, 0.01545216497150071581, 0.01648230930293407767, 0.01699738146865076294, 0.01751245363436744473, 0.01854259796580083608, 0.01957274229723423090, 0.02060288662866762224, 0.02266317529153437718, 0.02472346395440113212, 0.02678375261726789053, 0.02781389694870122983, 0.02884404128013456567, 0.03296461860586801657 ),
 .UNSPECIFIED. ) ;
#37799=CARTESIAN_POINT ( 'NONE',  ( -152.5046761101291963, 66.76407727525179325, 71.94415056971432421 ) ) ;
#37801=CARTESIAN_POINT ( 'NONE',  ( -0.9897066053608898351, 7.549089325901767289, -46.01382324979444860 ) ) ;
#37807=CARTESIAN_POINT ( 'NONE',  ( 15.29899606819415858, 6.485153354884283239, -77.36349468914947636 ) ) ;
#37809=ORIENTED_EDGE ( 'NONE', *, *, #51571, .F. ) ;
#37812=DIRECTION ( 'NONE',  ( 0.000000000000000000, 0.000000000000000000, 1.000000000000000000 ) ) ;
#37813=CARTESIAN_POINT ( 'NONE',  ( -131.6508182719823026, 50.40277850441007246, -47.24685355452295710 ) ) ;
#37814=EDGE_CURVE ( 'NONE', #58488, #56789, #46927, .T. ) ;
#37824=CARTESIAN_POINT ( 'NONE',  ( 197.8588046850313447, 99.02485934465610740, 12.95651097256631878 ) ) ;
#37826=CIRCLE ( 'NONE', #61441, 242.4895526022646379 ) ;
#37827=ORIENTED_EDGE ( 'NONE', *, *, #32697, .T. ) ;
#37832=CARTESIAN_POINT ( 'NONE',  ( 140.8855094313932739, 47.03549517811092784, 66.48436074708210697 ) ) ;
#37833=DIRECTION ( 'NONE',  ( -0.8160245890732938934, -0.5780171883497599028, 0.000000000000000000 ) ) ;
#37834=CARTESIAN_POINT ( 'NONE',  ( 158.9231328297667289, 58.78767772853188944, -89.91818538214990042 ) ) ;
#37841=B_SPLINE_CURVE_WITH_KNOTS ( 'NONE', 3,
 ( #18753, #38548, #61657, #59992, #17437, #45828, #22722, #34934, #56376, #24385, #19432, #33639, #33290, #55068, #8198, #8549, #67304, #30001, #3270, #46164 ),
 .UNSPECIFIED., .F., .F.,
 ( 4, 2, 2, 2, 2, 2, 2, 2, 2, 4 ),
 ( 0.000000000000000000, 0.001285001623041191797, 0.002570003246082383595, 0.003855004869123575175, 0.005140006492164767189, 0.006425008115205958770, 0.007710009738247150350, 0.008995011361288341931, 0.009637512172808941624, 0.01028001298432954305 ),
 .UNSPECIFIED. ) ;
#37842=CARTESIAN_POINT ( 'NONE',  ( -144.3939084932120807, 61.25241660819418144, -36.82102133094029739 ) ) ;
#37843=CARTESIAN_POINT ( 'NONE',  ( -166.2053056899075045, 81.18967388993337408, -71.97276839613554955 ) ) ;
#37848=CARTESIAN_POINT ( 'NONE',  ( -143.7151964745329451, 59.41799441280381444, 60.29410247371058063 ) ) ;
#37849=CYLINDRICAL_SURFACE ( 'NONE', #39046, 7.500000000000027534 ) ;
#37851=CARTESIAN_POINT ( 'NONE',  ( 81.57482918025357321, 17.75786713398421668, -10.93062121972884349 ) ) ;
#37853=CARTESIAN_POINT ( 'NONE',  ( 88.53517449242357884, 20.08005703101045469, -62.90834010636418583 ) ) ;
#37855=CARTESIAN_POINT ( 'NONE',  ( 57.27073671374542130, 11.41305252370465162, -92.07090031608234426 ) ) ;
#37857=CARTESIAN_POINT ( 'NONE',  ( -151.5114545224535902, 65.89821478636478957, -88.77172430480310084 ) ) ;
#37861=CARTESIAN_POINT ( 'NONE',  ( 188.2076037774874919, 86.11782719225438143, -72.93302748442802397 ) ) ;
#37862=CARTESIAN_POINT ( 'NONE',  ( 11.21387192505586761, 6.397095920409659797, 31.55118611238502524 ) ) ;
#37866=CARTESIAN_POINT ( 'NONE',  ( 108.3753929817421096, 29.13179266688724312, -62.98785435523912213 ) ) ;
#37867=CARTESIAN_POINT ( 'NONE',  ( 81.76092782665034520, 17.81692437267513540, 42.92251290309585698 ) ) ;
#37869=CARTESIAN_POINT ( 'NONE',  ( 63.49941241090380117, 13.81848793187417712, -50.72069083216975116 ) ) ;
#37870=CARTESIAN_POINT ( 'NONE',  ( -119.1605144823340083, 43.39823405392971267, 34.80618779126584883 ) ) ;
#37871=B_SPLINE_CURVE_WITH_KNOTS ( 'NONE', 3,
 ( #4059, #5760, #64517, #42709, #43045, #58880, #48307, #37093, #16670, #47632, #26197, #16326, #47290, #5429, #26543, #42025, #68745, #58532, #20918, #10693, #15642, #58203, #10023, #26882, #32169, #141, #48656, #32507, #31475, #53938, #69442, #64866, #53249, #20563, #53598, #42369, #59226, #37782, #63830, #27219, #21598, #15979, #11043, #25863, #21945, #10351, #69085, #31144 ),
 .UNSPECIFIED., .F., .F.,
 ( 4, 2, 2, 2, 2, 2, 2, 2, 2, 2, 2, 2, 2, 2, 2, 2, 2, 2, 2, 2, 2, 2, 2, 4 ),
 ( 0.02698595842317762922, 0.02784423243973404780, 0.02870250645629046637, 0.03041905448940321333, 0.03127732850595960068, 0.03213560252251598803, 0.03385215055562876274, 0.03471042457218512234, 0.03556869858874148888, 0.03728524662185418725, 0.03814352063841052604, 0.03900179465496686482, 0.03986006867152319666, 0.04071834268807953544, 0.04157661670463586728, 0.04243489072119220606, 0.04415143875430486975, 0.04500971277086120159, 0.04586798678741754037, 0.04758453482053021794, 0.04930108285364289550, 0.05101763088675557306, 0.05273417891986825756, 0.05445072695298092819 ),
 .UNSPECIFIED. ) ;
#37875=CARTESIAN_POINT ( 'NONE',  ( -23.93895920923072396, 9.495000752338446759, 10.62982118334621617 ) ) ;
#37876=ORIENTED_EDGE ( 'NONE', *, *, #24586, .F. ) ;
#37877=CARTESIAN_POINT ( 'NONE',  ( -15.31363169557738324, 7.494880774891998776, -43.40552099073981651 ) ) ;
#37882=CARTESIAN_POINT ( 'NONE',  ( 150.2794558856210756, 52.26944788078747450, -14.57987070555832432 ) ) ;
#37883=CARTESIAN_POINT ( 'NONE',  ( 31.90247004928963648, 8.563336936370815167, 10.06589353110114970 ) ) ;
#37888=CARTESIAN_POINT ( 'NONE',  ( 212.0383651583489097, 116.9865343143054730, 88.79641243644768167 ) ) ;
#37893=DIRECTION ( 'NONE',  ( -0.000000000000000000, 1.000000000000000000, -0.000000000000000000 ) ) ;
#37894=CARTESIAN_POINT ( 'NONE',  ( 46.84154678921881043, 10.51341196666389521, -70.94621687880534466 ) ) ;
#37895=CARTESIAN_POINT ( 'NONE',  ( -0.3747453031323927930, 6.520267647591905913, 36.62717459950940935 ) ) ;
#37897=CARTESIAN_POINT ( 'NONE',  ( 92.99472202396344755, 22.76601925259606318, 86.92061487625339566 ) ) ;
#37901=CARTESIAN_POINT ( 'NONE',  ( -132.4951995226845156, 50.99687809989499243, 7.706407028771845802 ) ) ;
#37902=CARTESIAN_POINT ( 'NONE',  ( -173.1211646369891355, 88.63826465341152527, -34.71195716474998960 ) ) ;
#37903=CARTESIAN_POINT ( 'NONE',  ( -179.9963635872885561, 95.12185477187962590, 88.99551518947737350 ) ) ;
#37908=EDGE_CURVE ( 'NONE', #25095, #22557, #37994, .T. ) ;
#37909=CARTESIAN_POINT ( 'NONE',  ( 197.8588046850312878, 99.02485934465607897, -13.88803961789735375 ) ) ;
#37910=CARTESIAN_POINT ( 'NONE',  ( -156.9749551707454316, 70.78135822687410439, 92.69151126661552098 ) ) ;
#37912=CARTESIAN_POINT ( 'NONE',  ( 138.2204650371259618, 44.12203217345472694, 43.12867697710134962 ) ) ;
#37915=CARTESIAN_POINT ( 'NONE',  ( 81.04027388895738682, 18.64386073872848826, 15.39279842491352390 ) ) ;
#37917=CARTESIAN_POINT ( 'NONE',  ( 164.9540180502650628, 65.02981548735053252, 10.63337814117685198 ) ) ;
#37918=CARTESIAN_POINT ( 'NONE',  ( -149.5074843970971301, -170.0000000000000000, 91.90992242082643315 ) ) ;
#37919=VECTOR ( 'NONE', #68058, 1000.000000000000000 ) ;
#37923=CARTESIAN_POINT ( 'NONE',  ( -75.00168449119586001, 20.95943092127970431, -9.222782878067645740 ) ) ;
#37927=CARTESIAN_POINT ( 'NONE',  ( 159.2389084450350367, 59.03884018680376755, 44.21161777826668526 ) ) ;
#37931=CARTESIAN_POINT ( 'NONE',  ( -102.2801239173131194, -170.0000000000000000, 45.51907450641513009 ) ) ;
#37932=ADVANCED_FACE ( 'NONE', ( #17222 ), #10907, .T. ) ;
#37933=CARTESIAN_POINT ( 'NONE',  ( -38.69577193929646342, 10.89562623693159971, -17.93097055276763641 ) ) ;
#37935=CARTESIAN_POINT ( 'NONE',  ( -180.5954680880247167, 97.44843622358465041, 37.68151972413897255 ) ) ;
#37936=CARTESIAN_POINT ( 'NONE',  ( -38.89042640463648581, 10.93374343663409398, -68.67378654700414131 ) ) ;
#37941=LINE ( 'NONE', #43900, #67962 ) ;
#37945=CARTESIAN_POINT ( 'NONE',  ( 68.58269726742371120, 14.03310040064105912, 85.96549742863071231 ) ) ;
#37955=CARTESIAN_POINT ( 'NONE',  ( 210.6475357757682048, 114.8748261044496104, -75.24406005627064076 ) ) ;
#37958=ADVANCED_FACE ( 'NONE', ( #32722 ), #27084, .F. ) ;
#37959=B_SPLINE_CURVE_WITH_KNOTS ( 'NONE', 3,
 ( #409, #43657, #27486, #1116, #65485, #6024, #60196, #48572, #37694, #44360, #32773, #6734, #17643, #49278, #22915, #21864, #64783, #33129, #48925, #64431, #1460, #44008, #27140, #54201, #59144, #59491, #65844, #43307, #54561, #16242, #65136, #38752, #53860, #22565, #33487, #17278, #16930, #16590, #38394, #32432, #11301, #38046, #59834, #6387 ),
 .UNSPECIFIED., .F., .F.,
 ( 4, 2, 2, 2, 2, 2, 2, 2, 2, 2, 2, 2, 2, 2, 2, 2, 2, 2, 2, 2, 2, 4 ),
 ( 6.938893903907228378E-18, 0.001473754749730493913, 0.002210632124595742713, 0.002947509499460991729, 0.004421264249191470680, 0.005895018998921949631, 0.007368773748652429449, 0.008105651123517656348, 0.008842528498382884114, 0.01031628324811332230, 0.01179003799784375875, 0.01252691537270898825, 0.01326379274757421428, 0.01473754749730467328, 0.01547442487216991146, 0.01621130224703514963, 0.01768505699676562598, 0.01915881174649610233, 0.01989568912136134224, 0.02063256649622657868, 0.02210632124595707237, 0.02358007599568756954 ),
 .UNSPECIFIED. ) ;
#37960=CARTESIAN_POINT ( 'NONE',  ( -78.66644367742111399, 22.32174330031319798, 18.57365054920947500 ) ) ;
#37964=CARTESIAN_POINT ( 'NONE',  ( 157.4703587214989113, 57.65129005721575339, -36.12418429913763163 ) ) ;
#37966=CARTESIAN_POINT ( 'NONE',  ( 162.0812592823604916, 62.62783216273700049, -64.53408560632756519 ) ) ;
#37973=CARTESIAN_POINT ( 'NONE',  ( -25.49247221749737236, 9.706368398275719400, -65.06484043158185671 ) ) ;
#37974=CARTESIAN_POINT ( 'NONE',  ( 41.34269507549201705, 9.685203600174697058, 30.15284864378948981 ) ) ;
#37975=CARTESIAN_POINT ( 'NONE',  ( -25.81763596640060499, 8.735969132042857410, 59.59007064553521360 ) ) ;
#37977=CARTESIAN_POINT ( 'NONE',  ( 132.9485794245231602, 40.87843215479635717, -9.220194473094281307 ) ) ;
#37978=B_SPLINE_CURVE_WITH_KNOTS ( 'NONE', 3,
 ( #14341, #35795, #4469, #4804, #6188, #64593, #212, #48051, #22024, #5834, #21671, #27643, #47706, #53324, #49083, #59639, #69166, #42774, #10086, #36830, #63558, #26270, #26950, #64946, #64240, #58268, #10771, #21326, #32923, #15367, #59304, #37159, #54362, #5154, #922, #16400, #11453, #48729, #48377, #573, #20992, #16739, #42441, #22371 ),
 .UNSPECIFIED., .F., .F.,
 ( 4, 2, 2, 2, 2, 2, 2, 2, 2, 2, 2, 2, 2, 2, 2, 2, 2, 2, 2, 2, 2, 4 ),
 ( 0.02495775893651561855, 0.02650251144344301785, 0.02804726395037042061, 0.02959201645729781990, 0.03113676896422521920, 0.03268152147115262196, 0.03345389772461633549, 0.03422627397808004207, 0.03577102648500748300, 0.03654340273847120346, 0.03731577899193493086, 0.03808815524539864439, 0.03886053149886237179, 0.04040528400578980578, 0.04117766025925351236, 0.04195003651271722589, 0.04349478901964463212, 0.04503954152657204529, 0.04581191778003575188, 0.04658429403349946540, 0.04812904654042689245, 0.04967379904735433338 ),
 .UNSPECIFIED. ) ;
#37980=ORIENTED_EDGE ( 'NONE', *, *, #48793, .F. ) ;
#37981=CARTESIAN_POINT ( 'NONE',  ( -128.7724923851857284, 49.63576597317771899, 45.04931761937589840 ) ) ;
#37984=CARTESIAN_POINT ( 'NONE',  ( 185.7556003757505323, 84.93464887485406223, -91.53351864259758486 ) ) ;
#37985=CARTESIAN_POINT ( 'NONE',  ( 62.53328835682432896, 12.56090025569836754, 56.65751152968496029 ) ) ;
#37987=CARTESIAN_POINT ( 'NONE',  ( -29.75554431712551917, 10.33961951730130124, -89.19458633079901233 ) ) ;
#37994=LINE ( 'NONE', #53804, #66520 ) ;
#37996=CARTESIAN_POINT ( 'NONE',  ( 138.1919700334460401, 44.10401742531043823, -76.50577590848440934 ) ) ;
#37999=CARTESIAN_POINT ( 'NONE',  ( 83.38067517854669575, 18.33799117207142260, 3.603261572607144636 ) ) ;
#38006=CARTESIAN_POINT ( 'NONE',  ( 93.61951000632933528, 21.92572933971851512, 7.638221738897885693 ) ) ;
#38010=ORIENTED_EDGE ( 'NONE', *, *, #2975, .F. ) ;
#38014=CARTESIAN_POINT ( 'NONE',  ( 152.6560521232696317, 54.00248515670892857, 31.15348575667133701 ) ) ;
#38015=CARTESIAN_POINT ( 'NONE',  ( 65.39792658623289867, 14.27332852928128126, 44.42870172783316463 ) ) ;
#38020=EDGE_LOOP ( 'NONE', ( #38459, #42285, #57750, #43237 ) ) ;
#38021=CARTESIAN_POINT ( 'NONE',  ( 136.7507824285648326, 44.38599729999913279, -63.44489443287879027 ) ) ;
#38025=FACE_BOUND ( 'NONE', #47245, .T. ) ;
#38030=CARTESIAN_POINT ( 'NONE',  ( -85.35172689181705152, 26.07142112926218758, 7.637577235932388575 ) ) ;
#38033=CARTESIAN_POINT ( 'NONE',  ( -120.4666325602655945, 44.20829586446608062, -74.44071530592697172 ) ) ;
#38035=CARTESIAN_POINT ( 'NONE',  ( 116.6734749296699505, 31.97209464358270026, 14.15860144538439336 ) ) ;
#38036=CARTESIAN_POINT ( 'NONE',  ( 94.06699947028482711, 23.17027898120149487, -17.47450249519500787 ) ) ;
#38042=CARTESIAN_POINT ( 'NONE',  ( 80.73462811483980772, 18.54763808182592300, -74.83009348606147171 ) ) ;
#38043=CARTESIAN_POINT ( 'NONE',  ( 103.2255776213605714, 26.86235640255825174, 93.47014144773791600 ) ) ;
#38044=DIRECTION ( 'NONE',  ( -0.000000000000000000, 1.000000000000000000, -0.000000000000000000 ) ) ;
#38046=CARTESIAN_POINT ( 'NONE',  ( -30.46002654261637943, 10.45132580906818021, -50.26895622567106869 ) ) ;
#38047=CARTESIAN_POINT ( 'NONE',  ( -48.58279704072702287, 14.07632445131079635, -65.75936485380451302 ) ) ;
#38048=CARTESIAN_POINT ( 'NONE',  ( -74.63254191291112249, 21.89590985985097760, -89.97802660070999536 ) ) ;
#38049=CARTESIAN_POINT ( 'NONE',  ( -120.4666325602655945, 44.20829586446606640, -20.75161412499960178 ) ) ;
#38052=CARTESIAN_POINT ( 'NONE',  ( 37.46876540261052924, 9.179568636624027889, 57.00768069096702817 ) ) ;
#38053=CARTESIAN_POINT ( 'NONE',  ( 133.8566784816069060, 42.60093787723656789, -89.71241211332301191 ) ) ;
#38057=ORIENTED_EDGE ( 'NONE', *, *, #42870, .F. ) ;
#38060=CARTESIAN_POINT ( 'NONE',  ( 186.7642514597452532, 86.02880938169742819, -11.97657000041078490 ) ) ;
#38061=CARTESIAN_POINT ( 'NONE',  ( 212.0803491126036704, 118.9047894217573003, 11.22770652852349293 ) ) ;
#38063=B_SPLINE_CURVE_WITH_KNOTS ( 'NONE', 3,
 ( #66697, #51548, #2321, #19526, #12518, #55782, #7603, #2663, #33979, #29389, #50845, #20552, #25167, #42017, #63476, #58193, #36748, #46596 ),
 .UNSPECIFIED., .F., .F.,
 ( 4, 2, 2, 2, 2, 2, 2, 2, 4 ),
 ( 0.01001195649024165871, 0.01126366347862624989, 0.01251537046701084281, 0.01376707745539543573, 0.01501878444378002692, 0.01627049143216461810, 0.01752219842054920929, 0.01877390540893380394, 0.02002561239731839512 ),
 .UNSPECIFIED. ) ;
#38065=LINE ( 'NONE', #48943, #32941 ) ;
#38066=FACE_OUTER_BOUND ( 'NONE', #49050, .T. ) ;
#38068=DIRECTION ( 'NONE',  ( -0.000000000000000000, 1.000000000000000000, -0.000000000000000000 ) ) ;
#38071=CARTESIAN_POINT ( 'NONE',  ( 86.62931800182293784, 20.48449268398423584, -35.82156419891171595 ) ) ;
#38072=CARTESIAN_POINT ( 'NONE',  ( -50.14523569787233725, 14.45648954445650780, 58.96871617340304539 ) ) ;
#38074=DIRECTION ( 'NONE',  ( 0.000000000000000000, -1.000000000000000000, 0.000000000000000000 ) ) ;
#38075=CARTESIAN_POINT ( 'NONE',  ( -14.61007982266178651, 8.438780854740821624, 88.09163706110108194 ) ) ;
#38079=CARTESIAN_POINT ( 'NONE',  ( -57.43251939610648549, 15.33203492375495003, 57.53293398456845864 ) ) ;
#38080=ORIENTED_EDGE ( 'NONE', *, *, #54919, .T. ) ;
#38082=DIRECTION ( 'NONE',  ( -0.000000000000000000, 1.000000000000000000, -0.000000000000000000 ) ) ;
#38084=CARTESIAN_POINT ( 'NONE',  ( 107.0477776024378755, 27.43148174916615645, 30.32163195193443883 ) ) ;
#38086=CARTESIAN_POINT ( 'NONE',  ( -61.75629144857964548, 16.58190704077737720, -66.18821733435061105 ) ) ;
#38087=CYLINDRICAL_SURFACE ( 'NONE', #39780, 7.500000000000013323 ) ;
#38088=CARTESIAN_POINT ( 'NONE',  ( 179.0091171455097481, 77.94933395983140656, -50.94517210893256731 ) ) ;
#38091=CARTESIAN_POINT ( 'NONE',  ( 91.13361825170458985, 21.00701373666981198, 43.22864410637488675 ) ) ;
#38092=VERTEX_POINT ( 'NONE', #29521 ) ;
#38094=CARTESIAN_POINT ( 'NONE',  ( 104.7042813665017178, 27.49927371769996753, -11.49719868635148146 ) ) ;
#38097=CARTESIAN_POINT ( 'NONE',  ( 66.18991464235057265, 13.43011255454270980, -90.06529977466986736 ) ) ;
#38103=ORIENTED_EDGE ( 'NONE', *, *, #48319, .T. ) ;
#38105=ORIENTED_EDGE ( 'NONE', *, *, #6886, .T. ) ;
#38106=CARTESIAN_POINT ( 'NONE',  ( -8.807541152391509698, 6.956521193351524524, -8.622092021015157925 ) ) ;
#38107=CARTESIAN_POINT ( 'NONE',  ( -173.7786140196550662, 89.37941604754422542, 84.53550708663692603 ) ) ;
#38110=CARTESIAN_POINT ( 'NONE',  ( -60.98168946575806615, 17.40090852531919907, -38.09669203216598987 ) ) ;
#38111=CARTESIAN_POINT ( 'NONE',  ( -7.825402957745083654, 7.899365992529244984, -8.573520141480125645 ) ) ;
#38113=CARTESIAN_POINT ( 'NONE',  ( 20.74852474914888489, 6.709938988646748648, -10.52766966389744496 ) ) ;
#38119=CARTESIAN_POINT ( 'NONE',  ( -142.3260422482980800, 59.60034523324938505, 13.61095042684088341 ) ) ;
#38121=CARTESIAN_POINT ( 'NONE',  ( -24.32220005085346770, 9.546215986458923553, 89.01704716004896056 ) ) ;
#38123=CARTESIAN_POINT ( 'NONE',  ( 112.1009898303695707, 30.86414810229296535, -9.296667012977504641 ) ) ;
#38127=CARTESIAN_POINT ( 'NONE',  ( -155.0388735873032147, 70.37329702672087706, 86.80759492728509485 ) ) ;
#38132=CARTESIAN_POINT ( 'NONE',  ( -154.6085044440278580, 69.98390342970670019, -20.97153785029703599 ) ) ;
#38133=CARTESIAN_POINT ( 'NONE',  ( 32.89501968360929851, 8.663558833820816929, -39.35812473969490810 ) ) ;
#38135=CARTESIAN_POINT ( 'NONE',  ( -32.41627406084104734, 9.753381371531505195, 72.01291641558607637 ) ) ;
#38138=ORIENTED_EDGE ( 'NONE', *, *, #17953, .T. ) ;
#38139=LINE ( 'NONE', #1211, #64926 ) ;
#38140=DIRECTION ( 'NONE',  ( 0.000000000000000000, 0.000000000000000000, 1.000000000000000000 ) ) ;
#38142=CARTESIAN_POINT ( 'NONE',  ( -5.412684891282530941, 7.753215344827982136, -50.03639412057999181 ) ) ;
#38143=CARTESIAN_POINT ( 'NONE',  ( 107.9362503323352769, 27.82881837607801856, 17.41909339002288348 ) ) ;
#38148=CARTESIAN_POINT ( 'NONE',  ( 13.83281508467570831, 7.452090093180181896, 17.92762544713185946 ) ) ;
#38149=AXIS2_PLACEMENT_3D ( 'NONE', #11017, #69059, #53225 ) ;
#38152=CARTESIAN_POINT ( 'NONE',  ( -132.4951995226845156, 50.99687809989497822, -72.82724474261920022 ) ) ;
#38154=CARTESIAN_POINT ( 'NONE',  ( 45.34143264614440483, 9.256465810451187437, -74.55058974195040378 ) ) ;
#38156=CARTESIAN_POINT ( 'NONE',  ( 58.08938767906772682, 12.61185010801509954, -64.38876158233470903 ) ) ;
#38159=ORIENTED_EDGE ( 'NONE', *, *, #38284, .F. ) ;
#38161=CARTESIAN_POINT ( 'NONE',  ( 188.4992282969374742, 86.43939134553235704, 89.35533139977708572 ) ) ;
#38162=ORIENTED_EDGE ( 'NONE', *, *, #41374, .F. ) ;
#38164=EDGE_LOOP ( 'NONE', ( #4441, #20405 ) ) ;
#38165=CARTESIAN_POINT ( 'NONE',  ( 188.0094179620990928, 87.39792407168454247, 33.91549744460515825 ) ) ;
#38167=VERTEX_POINT ( 'NONE', #23223 ) ;
#38168=CARTESIAN_POINT ( 'NONE',  ( 117.6853163455684808, 33.60747889659833731, 65.01678748886072867 ) ) ;
#38169=B_SPLINE_CURVE_WITH_KNOTS ( 'NONE', 3,
 ( #21230, #48276, #59187, #48616, #69414, #25830, #21911, #58847, #20525, #20882, #15948, #9988, #47257, #64832, #63801, #53905, #37058, #105, #5726, #15264, #68716, #10660, #16294, #11009, #27185, #9646, #58172, #32128, #32473, #5397, #16631, #5044, #31107, #36726, #31441, #53215, #457, #26506, #28225, #65177, #17692, #6070, #49326, #34220, #11350 ),
 .UNSPECIFIED., .F., .F.,
 ( 4, 2, 2, 2, 2, 2, 2, 2, 1, 2, 2, 2, 2, 2, 2, 2, 2, 2, 2, 2, 2, 2, 4 ),
 ( 0.000000000000000000, 0.001470449819620649103, 0.002205674729430984280, 0.002940899639241319891, 0.004411349458861969428, 0.005881799278482619832, 0.007352249098103270236, 0.008087474007913597607, 0.008822698917723924977, 0.009557923827534252348, 0.01029314873734457798, 0.01176359855696523446, 0.01249882346677556183, 0.01323404837658588920, 0.01470449819620655608, 0.01543972310601688866, 0.01617494801582721950, 0.01764539783544789506, 0.01911584765506857062, 0.01985107256487890146, 0.02058629747468922883, 0.02205674729430989398, 0.02352719711393055219 ),
 .UNSPECIFIED. ) ;
#38170=CARTESIAN_POINT ( 'NONE',  ( 139.6150621148398443, 46.20856238844173447, 68.68618430425954102 ) ) ;
#38172=AXIS2_PLACEMENT_3D ( 'NONE', #50671, #61234, #43991 ) ;
#38174=CARTESIAN_POINT ( 'NONE',  ( 88.28780346671264567, 19.99350429399659390, -50.63982961935722926 ) ) ;
#38175=CARTESIAN_POINT ( 'NONE',  ( -189.8071159312682425, 107.8771087123619594, 35.54271035159577252 ) ) ;
#38180=CARTESIAN_POINT ( 'NONE',  ( 110.7114632166111932, 29.09878355652111281, -50.92243756565373047 ) ) ;
#38182=CARTESIAN_POINT ( 'NONE',  ( -144.2155061717025717, 61.10843690942980544, -36.99245134645610733 ) ) ;
#38185=CARTESIAN_POINT ( 'NONE',  ( -147.3641864666714696, 62.38213854487952403, -49.51360668648376162 ) ) ;
#38190=ORIENTED_EDGE ( 'NONE', *, *, #7555, .T. ) ;
#38191=CARTESIAN_POINT ( 'NONE',  ( -131.6508182719823594, 50.40277850441008667, 33.28679821686808538 ) ) ;
#38192=DIRECTION ( 'NONE',  ( -0.000000000000000000, 1.000000000000000000, -0.000000000000000000 ) ) ;
#38194=CARTESIAN_POINT ( 'NONE',  ( 91.50468583833760761, 22.21368636549395248, 31.49154984481617703 ) ) ;
#38195=CARTESIAN_POINT ( 'NONE',  ( 84.28078136020373279, 18.63296074526051527, -9.350161758405024059 ) ) ;
#38196=CARTESIAN_POINT ( 'NONE',  ( 92.21267147730745251, 21.40196534721315658, -65.13473199430346483 ) ) ;
#38197=CARTESIAN_POINT ( 'NONE',  ( 197.3054165770396651, 96.72615186924556951, 8.555290693686146142 ) ) ;
#38200=VERTEX_POINT ( 'NONE', #61196 ) ;
#38203=CARTESIAN_POINT ( 'NONE',  ( 46.50704915687943242, 9.440294391580035693, 39.82807691976670839 ) ) ;
#38204=CARTESIAN_POINT ( 'NONE',  ( 15.78827728214693416, 6.500811158483284835, 30.01470767270522089 ) ) ;
#38205=CARTESIAN_POINT ( 'NONE',  ( 181.0840389613909736, -170.0000000000000000, -16.88050707541594164 ) ) ;
#38208=EDGE_CURVE ( 'NONE', #43433, #52438, #7389, .T. ) ;
#38211=CARTESIAN_POINT ( 'NONE',  ( 211.7357196141371674, 118.3691710715567211, -41.21681032355412100 ) ) ;
#38212=CARTESIAN_POINT ( 'NONE',  ( -72.77296415263757012, 21.23032531836537373, -74.12506392022689283 ) ) ;
#38214=CARTESIAN_POINT ( 'NONE',  ( 45.76405797021010358, 10.34101216371941767, -39.14056405445984410 ) ) ;
#38215=CARTESIAN_POINT ( 'NONE',  ( 205.1049299651096476, 106.9023875785546522, 71.05227132923316447 ) ) ;
#38217=CARTESIAN_POINT ( 'NONE',  ( -103.2169245450825201, 33.25885825286819397, -23.12591867443444471 ) ) ;
#38218=VERTEX_POINT ( 'NONE', #38696 ) ;
#38220=CARTESIAN_POINT ( 'NONE',  ( 94.14197829520114169, 23.19876121754314369, 64.06685891365469843 ) ) ;
#38221=CARTESIAN_POINT ( 'NONE',  ( 153.2282895792479280, 54.42637815496160414, -22.96929501619974445 ) ) ;
#38223=CARTESIAN_POINT ( 'NONE',  ( -101.8187363387487210, 33.67461140603126069, -76.85912785543963821 ) ) ;
#38226=CARTESIAN_POINT ( 'NONE',  ( 212.1900147491068651, 117.2197345096297312, 90.80498426450013483 ) ) ;
#38229=CARTESIAN_POINT ( 'NONE',  ( 55.51528220483957909, 12.08323518953685927, 64.39593437836721534 ) ) ;
#38231=CARTESIAN_POINT ( 'NONE',  ( -11.56945424397728139, 8.173256823723106024, 4.267794400975877700 ) ) ;
#38233=CARTESIAN_POINT ( 'NONE',  ( 46.12582897016704209, 10.39833982076225105, -66.63266472015294539 ) ) ;
#38235=CARTESIAN_POINT ( 'NONE',  ( -107.7743374187917311, 35.66028478413596048, -64.23029970060920846 ) ) ;
#38236=CARTESIAN_POINT ( 'NONE',  ( 93.88165567369813402, 23.09997474706427667, 92.84299207529174680 ) ) ;
#38241=CARTESIAN_POINT ( 'NONE',  ( -133.3765738414514885, 51.62252165471732468, 11.85205414610034680 ) ) ;
#38246=CARTESIAN_POINT ( 'NONE',  ( -5.401648928593179910, 6.744888135494083947, -8.959184697842486500 ) ) ;
#38247=CARTESIAN_POINT ( 'NONE',  ( 199.3764173596862008, 100.9540560740992277, -22.29103892941747134 ) ) ;
#38248=CARTESIAN_POINT ( 'NONE',  ( -153.2300806271756528, 67.40240937773886287, 85.39292924717106814 ) ) ;
#38254=CARTESIAN_POINT ( 'NONE',  ( -101.8187363387486926, 33.67461140603126779, 30.51907450641510167 ) ) ;
#38256=EDGE_LOOP ( 'NONE', ( #4790, #35354, #39604, #12535 ) ) ;
#38260=ORIENTED_EDGE ( 'NONE', *, *, #21740, .F. ) ;
#38262=CARTESIAN_POINT ( 'NONE',  ( -120.3886177497181507, 42.97447856924565457, -91.00427280143986764 ) ) ;
#38263=DIRECTION ( 'NONE',  ( -0.000000000000000000, 1.000000000000000000, -0.000000000000000000 ) ) ;
#38267=CARTESIAN_POINT ( 'NONE',  ( 157.4703587214989113, 57.65129005721575339, 44.40946747225338953 ) ) ;
#38272=ORIENTED_EDGE ( 'NONE', *, *, #32234, .F. ) ;
#38276=DIRECTION ( 'NONE',  ( -0.000000000000000000, 1.000000000000000000, -0.000000000000000000 ) ) ;
#38278=CARTESIAN_POINT ( 'NONE',  ( 126.3681350380370674, 38.23508791628619008, 64.34750091452772836 ) ) ;
#38284=EDGE_CURVE ( 'NONE', #57393, #34477, #8429, .T. ) ;
#38285=B_SPLINE_CURVE_WITH_KNOTS ( 'NONE', 3,
 ( #66797, #56563, #18936, #8740, #45313, #2758, #19980, #24911, #62183, #46343, #67822, #18585, #8387, #40043, #51641, #30188, #34776, #24573, #68174, #19622, #35458, #40725, #29831, #14688, #3449, #56213, #51301, #46009, #56922, #51976, #29483, #46696, #62886, #41431, #41082, #40385, #23869, #3112, #61502, #62544, #24222, #14355, #30528, #45670 ),
 .UNSPECIFIED., .F., .F.,
 ( 4, 2, 2, 2, 2, 2, 2, 2, 2, 2, 2, 2, 2, 2, 2, 2, 2, 2, 2, 2, 2, 4 ),
 ( 0.02477387709520258857, 0.02633314402883776828, 0.02711277749565535120, 0.02789241096247293758, 0.02945167789610813810, 0.03023131136292572449, 0.03101094482974331434, 0.03257021176337850099, 0.03334984523019608044, 0.03412947869701365988, 0.03568874563064881184, 0.03646837909746639128, 0.03724801256428397073, 0.03802764603110154323, 0.03880727949791912268, 0.04036654643155427463, 0.04192581336518942658, 0.04348508029882458548, 0.04504434723245973743, 0.04660361416609488938, 0.04816288109973004827, 0.04972214803336520023 ),
 .UNSPECIFIED. ) ;
#38289=CARTESIAN_POINT ( 'NONE',  ( -109.5141185504297283, 36.61008623467700573, 93.79613039457322543 ) ) ;
#38293=CARTESIAN_POINT ( 'NONE',  ( -58.13254984326171382, 16.57438752089402456, 84.66073699768521976 ) ) ;
#38294=CARTESIAN_POINT ( 'NONE',  ( 79.53408731553405175, 17.12082763744059122, 66.53775872133530811 ) ) ;
#38295=ORIENTED_EDGE ( 'NONE', *, *, #27629, .F. ) ;
#38297=EDGE_LOOP ( 'NONE', ( #11534, #18186, #61811, #42813 ) ) ;
#38299=CARTESIAN_POINT ( 'NONE',  ( 212.1983751099433562, 117.2326047784726768, -70.52915068856044911 ) ) ;
#38302=CARTESIAN_POINT ( 'NONE',  ( -37.73701155674110197, 10.71027364713581065, -92.42797313720504349 ) ) ;
#38303=CARTESIAN_POINT ( 'NONE',  ( -54.09522495088363314, 14.42642983673693102, 3.518423213031079744 ) ) ;
#38305=CARTESIAN_POINT ( 'NONE',  ( 164.9706294237034001, 65.04392654036657007, -70.74285660430801670 ) ) ;
#38312=CARTESIAN_POINT ( 'NONE',  ( -81.90020664963797969, 23.57971581008656514, 31.14685346508889907 ) ) ;
#38313=CARTESIAN_POINT ( 'NONE',  ( -28.81071653159242274, 10.19258396314334902, -62.63311570043980936 ) ) ;
#38315=CARTESIAN_POINT ( 'NONE',  ( 129.5193594945039308, 38.86618897895343139, -10.54188000187672003 ) ) ;
#38322=CARTESIAN_POINT ( 'NONE',  ( 207.4867844023103487, 110.2451255333963189, 16.83735121052653838 ) ) ;
#38323=CARTESIAN_POINT ( 'NONE',  ( -146.5230751932348596, 62.99205605665031271, 31.32563957384398279 ) ) ;
#38325=CARTESIAN_POINT ( 'NONE',  ( 55.57657751403269231, 11.06944050856661832, 63.17132437929140565 ) ) ;
#38326=CARTESIAN_POINT ( 'NONE',  ( -4.072522659361696107, 7.683023425615343349, 57.96194782726411887 ) ) ;
#38329=CARTESIAN_POINT ( 'NONE',  ( -26.37645167493199949, 9.831227391966869789, -90.95605343330562675 ) ) ;
#38333=ORIENTED_EDGE ( 'NONE', *, *, #59308, .F. ) ;
#38338=DIRECTION ( 'NONE',  ( -0.000000000000000000, 1.000000000000000000, -0.000000000000000000 ) ) ;
#38341=FACE_OUTER_BOUND ( 'NONE', #59465, .T. ) ;
#38342=AXIS2_PLACEMENT_3D ( 'NONE', #25782, #4996, #4318 ) ;
#38343=EDGE_LOOP ( 'NONE', ( #11263, #15502 ) ) ;
#38345=CARTESIAN_POINT ( 'NONE',  ( 81.04675113612957205, 17.59091904316107247, 15.40005626147305229 ) ) ;
#38347=CARTESIAN_POINT ( 'NONE',  ( -72.21652659655759976, 19.96855882996548459, 34.05819120719318249 ) ) ;
#38349=DIRECTION ( 'NONE',  ( 0.000000000000000000, 0.000000000000000000, 1.000000000000000000 ) ) ;
#38350=EDGE_CURVE ( 'NONE', #35601, #40482, #28487, .T. ) ;
#38352=ORIENTED_EDGE ( 'NONE', *, *, #45821, .F. ) ;
#38353=CARTESIAN_POINT ( 'NONE',  ( -149.0782809666403921, 63.81577337591401289, -76.65738112195566600 ) ) ;
#38356=ORIENTED_EDGE ( 'NONE', *, *, #14857, .F. ) ;
#38360=CARTESIAN_POINT ( 'NONE',  ( -173.5422248620773189, 89.11126078969418529, -34.71195716474998960 ) ) ;
#38361=CARTESIAN_POINT ( 'NONE',  ( -131.1078488676298832, 50.02394948559179255, -10.17272884446006742 ) ) ;
#38365=CARTESIAN_POINT ( 'NONE',  ( 141.3556389957210513, 47.34429831367557284, -70.07195742417799522 ) ) ;
#38367=VERTEX_POINT ( 'NONE', #64653 ) ;
#38369=FACE_BOUND ( 'NONE', #3966, .T. ) ;
#38370=CARTESIAN_POINT ( 'NONE',  ( -7.336760511143401331, 6.859209474528210393, -77.26262132240756841 ) ) ;
#38371=CARTESIAN_POINT ( 'NONE',  ( -173.1211646369891355, 88.63826465341151106, 57.66624519710472185 ) ) ;
#38375=CARTESIAN_POINT ( 'NONE',  ( -85.96384504792884229, 26.32782846176032976, 12.82352473700630924 ) ) ;
#38381=CARTESIAN_POINT ( 'NONE',  ( -8.320534640989464492, 7.931748412542457771, 45.11558103944722120 ) ) ;
#38383=CARTESIAN_POINT ( 'NONE',  ( 112.1012908502484891, 29.75117929736501310, 2.996681463395355127 ) ) ;
#38384=CARTESIAN_POINT ( 'NONE',  ( 87.11239765416380010, 20.65008247340817249, -8.977013608448023874 ) ) ;
#38385=ORIENTED_EDGE ( 'NONE', *, *, #47258, .T. ) ;
#38389=CARTESIAN_POINT ( 'NONE',  ( 141.0229350107040887, -170.0000000000000000, -95.00000000000133582 ) ) ;
#38390=CARTESIAN_POINT ( 'NONE',  ( 117.7510257530316551, 33.64085080140208817, 90.74181468113641813 ) ) ;
#38391=CARTESIAN_POINT ( 'NONE',  ( -142.0860844253783171, 59.41107357617636353, 63.94597921072897861 ) ) ;
#38394=CARTESIAN_POINT ( 'NONE',  ( -28.35957743809534648, 10.12373109553627692, -49.66019367601061418 ) ) ;
#38395=CARTESIAN_POINT ( 'NONE',  ( 210.6475351020683604, 116.6976423915685785, -92.93013880689109385 ) ) ;
#38397=FACE_OUTER_BOUND ( 'NONE', #54835, .T. ) ;
#38400=CARTESIAN_POINT ( 'NONE',  ( 32.37980458033285203, 8.611076697115697343, 66.90419927267225830 ) ) ;
#38403=CARTESIAN_POINT ( 'NONE',  ( -125.8938041572051389, 46.49392987655490828, -8.069153307770243089 ) ) ;
#38405=CARTESIAN_POINT ( 'NONE',  ( 94.06699947028484132, 23.17027898120147711, 9.370048095268675326 ) ) ;
#38406=ADVANCED_FACE ( 'NONE', ( #10141 ), #26331, .F. ) ;
#38407=CARTESIAN_POINT ( 'NONE',  ( -13.78293860383720038, 7.352367295275509029, 69.04280783764355078 ) ) ;
#38410=CARTESIAN_POINT ( 'NONE',  ( 46.13320811200731697, 9.380653113584065395, -19.61926706393606068 ) ) ;
#38413=FACE_BOUND ( 'NONE', #64640, .T. ) ;
#38414=CARTESIAN_POINT ( 'NONE',  ( -60.65612136648953623, 16.25551606627059442, -37.70714318869556791 ) ) ;
#38418=B_SPLINE_CURVE_WITH_KNOTS ( 'NONE', 3,
 ( #11644, #64423, #28171, #22556, #22908, #6016, #59134, #5343, #32424, #54902, #38745, #32765, #27475, #10604, #44000, #42952, #12006, #398, #59482, #44353, #60188, #6726, #49622, #53510, #15891, #48223, #17270, #16233, #37336, #37686, #5668, #58788, #32074, #22212, #10956, #53850, #64774, #21855, #16582, #27131, #48918, #48563, #11293 ),
 .UNSPECIFIED., .F., .F.,
 ( 4, 2, 2, 2, 2, 2, 2, 2, 2, 2, 2, 2, 1, 2, 2, 2, 2, 2, 2, 2, 2, 4 ),
 ( 0.02358007599568756260, 0.02505677178601662183, 0.02579511968118114104, 0.02653346757634566025, 0.02801016336667471601, 0.02948685915700377178, 0.03022520705216829792, 0.03096355494733282407, 0.03244025073766187983, 0.03391694652799093213, 0.03539364231831998442, 0.03613199021348451057, 0.03687033810864903671, 0.03760868600381356980, 0.03834703389897809594, 0.03982372968930714824, 0.04130042547963619359, 0.04277712126996524589, 0.04351546916512977203, 0.04425381706029428430, 0.04573051285062330884, 0.04720720864095233338 ),
 .UNSPECIFIED. ) ;
#38422=EDGE_CURVE ( 'NONE', #42704, #42164, #6684, .T. ) ;
#38424=CARTESIAN_POINT ( 'NONE',  ( -50.14440374537738876, 14.45628984983894938, 70.35385673637195225 ) ) ;
#38427=DIRECTION ( 'NONE',  ( 0.000000000000000000, 0.000000000000000000, 1.000000000000000000 ) ) ;
#38428=AXIS2_PLACEMENT_3D ( 'NONE', #49865, #16811, #59029 ) ;
#38429=ORIENTED_EDGE ( 'NONE', *, *, #68516, .F. ) ;
#38430=CARTESIAN_POINT ( 'NONE',  ( 58.48209831743720599, 11.66636741727082160, 16.46295100624673680 ) ) ;
#38432=EDGE_LOOP ( 'NONE', ( #49546, #49035, #39058, #19573 ) ) ;
#38438=CARTESIAN_POINT ( 'NONE',  ( 104.3931729003987243, 26.26823401847090977, 41.83091430256712329 ) ) ;
#38442=EDGE_CURVE ( 'NONE', #32410, #16320, #45302, .T. ) ;
#38446=CARTESIAN_POINT ( 'NONE',  ( 161.1112535418156710, 61.83422628788726172, 43.47046046015263698 ) ) ;
#38447=CARTESIAN_POINT ( 'NONE',  ( -155.2836587093738956, 70.59655508952971559, -73.94790389774894379 ) ) ;
#38448=CARTESIAN_POINT ( 'NONE',  ( 64.69738688745243849, 14.10375742873389449, 17.78141051354113245 ) ) ;
#38449=CARTESIAN_POINT ( 'NONE',  ( 90.31682503704259091, 20.71196693118261933, 43.76113064241335593 ) ) ;
#38450=CARTESIAN_POINT ( 'NONE',  ( -53.38065169970958834, 15.27943072477081543, -35.40114938969493608 ) ) ;
#38453=CARTESIAN_POINT ( 'NONE',  ( -149.5074843970971017, 65.50121172469320641, -88.50193171241930656 ) ) ;
#38459=ORIENTED_EDGE ( 'NONE', *, *, #8011, .F. ) ;
#38460=CARTESIAN_POINT ( 'NONE',  ( -14.32241591711281892, 7.401556312061829956, -12.31863017529175863 ) ) ;
#38461=CARTESIAN_POINT ( 'NONE',  ( -166.1407022362849091, 81.12296115130531859, 89.24429516090893344 ) ) ;
#38464=CARTESIAN_POINT ( 'NONE',  ( -61.77164219855451677, 17.63686644795248171, -39.34642791434716003 ) ) ;
#38465=CARTESIAN_POINT ( 'NONE',  ( -12.77550690612892481, 8.273784096785060882, -21.72907486570559854 ) ) ;
#38470=ORIENTED_EDGE ( 'NONE', *, *, #39838, .F. ) ;
#38472=CARTESIAN_POINT ( 'NONE',  ( -143.4048679855200987, 60.45763799613828837, 15.74344414432664330 ) ) ;
#38473=VECTOR ( 'NONE', #12403, 1000.000000000000000 ) ;
#38477=CARTESIAN_POINT ( 'NONE',  ( -149.5074843970971301, -170.0000000000000000, -34.81283053149196149 ) ) ;
#38479=B_SPLINE_CURVE_WITH_KNOTS ( 'NONE', 3,
 ( #42472, #30894, #31577, #67843, #47739, #69203, #20328, #9785, #30209, #26310, #68192, #3812, #35479, #52344, #10120, #41451, #19997, #62904, #3467, #21028, #51996, #68522 ),
 .UNSPECIFIED., .F., .F.,
 ( 4, 2, 2, 2, 2, 2, 2, 2, 2, 2, 4 ),
 ( 7.867692934960096083E-17, 0.001318139496345244275, 0.001977209244517810684, 0.002636278992690376660, 0.003954418489035485193, 0.005272557985380592858, 0.005931627733553143655, 0.006590697481725694452, 0.007908836978070800383, 0.009226976474415907181, 0.01054511597076101398 ),
 .UNSPECIFIED. ) ;
#38480=CARTESIAN_POINT ( 'NONE',  ( 140.5958192060901411, 46.84598876498522912, -19.98049072836446527 ) ) ;
#38483=ORIENTED_EDGE ( 'NONE', *, *, #69377, .T. ) ;
#38485=CARTESIAN_POINT ( 'NONE',  ( -11.14880195267007323, 7.129907723790828378, 17.51241905048560810 ) ) ;
#38486=CARTESIAN_POINT ( 'NONE',  ( 32.67604581760325289, 7.629767527669979010, -66.63679567754731181 ) ) ;
#38487=CARTESIAN_POINT ( 'NONE',  ( -190.6985136298601731, 109.1272424661242582, 94.99999999999866418 ) ) ;
#38489=CARTESIAN_POINT ( 'NONE',  ( -38.84150381976580491, 10.92416363971238624, 63.33002578833360730 ) ) ;
#38490=CARTESIAN_POINT ( 'NONE',  ( 199.3764470687682717, 100.9548044849099142, 68.84309499164012891 ) ) ;
#38492=CARTESIAN_POINT ( 'NONE',  ( 187.8973304652192837, 87.27378997243174297, 60.50620952073695946 ) ) ;
#38493=CARTESIAN_POINT ( 'NONE',  ( -151.2410113808308552, 65.66338888995507261, 57.75535393765130721 ) ) ;
#38497=CARTESIAN_POINT ( 'NONE',  ( -85.45399718454962112, 25.02415453493131636, -39.41511587279529749 ) ) ;
#38500=CARTESIAN_POINT ( 'NONE',  ( 8.670103207226929953, 6.377073801252345575, -72.27660206952214139 ) ) ;
#38505=CARTESIAN_POINT ( 'NONE',  ( -126.8005235842505840, 47.09307471149451629, -61.79966952219996301 ) ) ;
#38508=CARTESIAN_POINT ( 'NONE',  ( 57.39233401791015154, 12.46575990788836563, -65.07837685070954592 ) ) ;
#38512=CARTESIAN_POINT ( 'NONE',  ( 180.6638663192742342, 78.18175084954954457, 83.00395592035752657 ) ) ;
#38513=EDGE_LOOP ( 'NONE', ( #21191, #43908, #68918, #355 ) ) ;
#38516=CARTESIAN_POINT ( 'NONE',  ( 179.4207200232661421, 76.93724985992179199, -36.36109878936809281 ) ) ;
#38520=CARTESIAN_POINT ( 'NONE',  ( 115.0606351894211201, 32.29586232625067765, 58.18666269473403219 ) ) ;
#38521=CARTESIAN_POINT ( 'NONE',  ( 140.2200249818744453, 46.60103563593126808, 59.87699706130887023 ) ) ;
#38524=CARTESIAN_POINT ( 'NONE',  ( 79.40386128751609363, 17.08093333150470627, -95.00000000000133582 ) ) ;
#38525=CARTESIAN_POINT ( 'NONE',  ( 87.59061758233885087, 19.75077892934019275, -35.86783240150010954 ) ) ;
#38527=CARTESIAN_POINT ( 'NONE',  ( -189.9554299271397895, 108.0836897899587825, 41.65156110337591144 ) ) ;
#38530=DIRECTION ( 'NONE',  ( 0.000000000000000000, 0.000000000000000000, 1.000000000000000000 ) ) ;
#38532=CARTESIAN_POINT ( 'NONE',  ( -78.66644367742111399, 23.39876645725285798, 18.57365054920947500 ) ) ;
#38533=CARTESIAN_POINT ( 'NONE',  ( -142.8492950481058870, 60.01492924994602163, -45.77552445218916688 ) ) ;
#38534=DIRECTION ( 'NONE',  ( 1.000000000000000000, 0.000000000000000000, -0.000000000000000000 ) ) ;
#38537=CARTESIAN_POINT ( 'NONE',  ( 57.09527843067913722, 12.40436368789086430, 5.857540484044117868 ) ) ;
#38540=CARTESIAN_POINT ( 'NONE',  ( -144.3945994505580757, 59.96115386701887928, 59.57298621908066849 ) ) ;
#38542=CARTESIAN_POINT ( 'NONE',  ( 110.2429982417149574, -170.0000000000000000, 10.26666361527366078 ) ) ;
#38545=CARTESIAN_POINT ( 'NONE',  ( 80.16939877002758408, 17.31693935407228935, -12.63458944764736636 ) ) ;
#38548=CARTESIAN_POINT ( 'NONE',  ( -24.17914301452584169, 8.511888984123499924, -94.57447209120040554 ) ) ;
#38553=CARTESIAN_POINT ( 'NONE',  ( 181.0840389613909736, -170.0000000000000000, 63.65314469597510794 ) ) ;
#38554=DIRECTION ( 'NONE',  ( -0.000000000000000000, 1.000000000000000000, -0.000000000000000000 ) ) ;
#38560=CARTESIAN_POINT ( 'NONE',  ( 45.04020069093783007, 10.22779424730543418, -38.14995898565744170 ) ) ;
#38563=CARTESIAN_POINT ( 'NONE',  ( -104.1342612728951309, 33.73231160250195160, -22.95220324455834415 ) ) ;
#38567=CARTESIAN_POINT ( 'NONE',  ( -85.98021075183530115, 25.24360504037805342, 89.91407000372294078 ) ) ;
#38571=B_SPLINE_CURVE_WITH_KNOTS ( 'NONE', 3,
 ( #27526, #43694, #16964, #51771, #13786, #30319, #8168, #66931, #19064, #29615, #40179, #2205, #7828, #56016, #8523, #13449, #46138, #61632, #3576, #66583, #25049, #51434, #62321, #23657, #50725, #24358, #51082, #3245, #29972, #14139, #2898, #45449, #18373, #45097, #45802, #39828, #61288, #67609, #13109, #34910, #56348, #67280, #34575, #18723, #35597, #24703, #19408 ),
 .UNSPECIFIED., .F., .F.,
 ( 4, 2, 2, 2, 2, 2, 2, 2, 2, 2, 2, 2, 1, 2, 2, 2, 2, 2, 2, 2, 2, 2, 2, 4 ),
 ( 0.000000000000000000, 0.001520400357569040442, 0.002280600536353578119, 0.003040800715138115579, 0.004561201072707176188, 0.005321401251491689362, 0.006081601430276202536, 0.007602001787845172505, 0.008362201966629670066, 0.009122402145414166760, 0.01064280250298316188, 0.01140300268176763950, 0.01216320286055211537, 0.01292340303933659298, 0.01368360321812107060, 0.01520400357569003102, 0.01596420375447449302, 0.01672440393325895155, 0.01824480429082784433, 0.01976520464839674057, 0.02052540482718119563, 0.02128560500596565069, 0.02280600536353454000, 0.02432640572110343277 ),
 .UNSPECIFIED. ) ;
#38586=CARTESIAN_POINT ( 'NONE',  ( -62.21428173307536724, 16.71931747086482289, -94.13522999573226002 ) ) ;
#38590=CARTESIAN_POINT ( 'NONE',  ( 81.80567187957538522, 18.88678701137715876, 85.11920350517479505 ) ) ;
#38597=CARTESIAN_POINT ( 'NONE',  ( -166.2053056899075045, 81.18967388993343093, -45.12821780567188057 ) ) ;
#38598=CARTESIAN_POINT ( 'NONE',  ( -130.5811943660945076, 50.88295841537571818, -48.28834053933531578 ) ) ;
#38600=CARTESIAN_POINT ( 'NONE',  ( -124.3331814159187445, 45.47486189329071493, -49.75303911620572705 ) ) ;
#38601=CARTESIAN_POINT ( 'NONE',  ( 86.62931800182293784, -170.0000000000000000, -43.32156419891173016 ) ) ;
#38603=CARTESIAN_POINT ( 'NONE',  ( -3.255961059272210800, 7.643453059677442596, -63.79517828393875334 ) ) ;
#38608=CARTESIAN_POINT ( 'NONE',  ( 197.9847015768255289, 97.56951352050454318, -40.46952643750044132 ) ) ;
#38609=CARTESIAN_POINT ( 'NONE',  ( -151.6648563624118822, 67.36546864992756412, 31.02422955355707046 ) ) ;
#38616=ORIENTED_EDGE ( 'NONE', *, *, #68602, .T. ) ;
#38617=ORIENTED_EDGE ( 'NONE', *, *, #55086, .T. ) ;
#38618=CARTESIAN_POINT ( 'NONE',  ( -71.41745561414265353, 19.69148172991711832, -13.78189858334474671 ) ) ;
#38619=FACE_OUTER_BOUND ( 'NONE', #68727, .T. ) ;
#38621=CARTESIAN_POINT ( 'NONE',  ( -15.07235766390728493, 8.482541916553472561, -71.71007873016166911 ) ) ;
#38623=CARTESIAN_POINT ( 'NONE',  ( 164.8407099662995563, 63.61629583487393802, 35.49381950204995917 ) ) ;
#38625=CARTESIAN_POINT ( 'NONE',  ( -75.00636493611887090, 22.03142602679956852, -36.05143679334967999 ) ) ;
#38631=CARTESIAN_POINT ( 'NONE',  ( -34.74740905761646559, 10.15745573515589406, -9.223982854342375859 ) ) ;
#38634=CARTESIAN_POINT ( 'NONE',  ( -37.79601571721868680, 10.72155118426296738, -65.67424366896023002 ) ) ;
#38635=CARTESIAN_POINT ( 'NONE',  ( 23.23965501943001044, 7.861749956303023978, 63.37552610149469956 ) ) ;
#38640=CARTESIAN_POINT ( 'NONE',  ( 207.9985316690167565, 110.9796440870787393, -90.77140804177048494 ) ) ;
#38641=CARTESIAN_POINT ( 'NONE',  ( -48.13019811071813336, 12.93401924038758288, 94.41062383682593406 ) ) ;
#38643=CARTESIAN_POINT ( 'NONE',  ( -38.26732153931118319, 10.81230693396214093, -45.92944804569359007 ) ) ;
#38644=EDGE_CURVE ( 'NONE', #18346, #10603, #9976, .T. ) ;
#38645=CARTESIAN_POINT ( 'NONE',  ( -101.7332236082777257, 32.50383353354374805, 84.22225394076856730 ) ) ;
#38648=CARTESIAN_POINT ( 'NONE',  ( -77.71801202538870257, 23.03755222122951452, -8.316084935337491046 ) ) ;
#38649=CARTESIAN_POINT ( 'NONE',  ( 84.28078136020376121, 18.63296074526051527, 71.18349001298599887 ) ) ;
#38655=CARTESIAN_POINT ( 'NONE',  ( 204.6977192012829789, 106.3443248447423457, -63.17048162308526571 ) ) ;
#38657=CARTESIAN_POINT ( 'NONE',  ( -75.00168449119588843, 20.95943092127969720, 17.62176771239603568 ) ) ;
#38658=CARTESIAN_POINT ( 'NONE',  ( -118.3948752128398496, 42.92869324237091178, 65.26186531831542936 ) ) ;
#38659=CARTESIAN_POINT ( 'NONE',  ( -53.14475157111026249, 14.17819596930906911, 3.715487147916443522 ) ) ;
#38660=CARTESIAN_POINT ( 'NONE',  ( 152.3102623290679674, 53.74757787434987222, -38.17601757745164548 ) ) ;
#38664=FACE_OUTER_BOUND ( 'NONE', #19018, .T. ) ;
#38669=CARTESIAN_POINT ( 'NONE',  ( -84.23431294393863311, 24.52078568147202731, 32.86922510554116172 ) ) ;
#38670=CARTESIAN_POINT ( 'NONE',  ( -26.49928411671542605, 9.848831533840670005, -63.99709101584238624 ) ) ;
#38671=CARTESIAN_POINT ( 'NONE',  ( 46.51679720856117228, 10.46086439153924807, 34.99061173750302345 ) ) ;
#38672=ADVANCED_FACE ( 'NONE', ( #47333 ), #20607, .T. ) ;
#38674=CARTESIAN_POINT ( 'NONE',  ( -146.7345109736526751, 61.86270848728300109, 18.34836298419372014 ) ) ;
#38675=EDGE_CURVE ( 'NONE', #63625, #47023, #55341, .T. ) ;
#38676=ORIENTED_EDGE ( 'NONE', *, *, #18278, .T. ) ;
#38683=CARTESIAN_POINT ( 'NONE',  ( -55.05276343752910151, 15.72344139423345588, -88.90542517938717992 ) ) ;
#38684=CARTESIAN_POINT ( 'NONE',  ( 140.7150918341941122, 46.92378309712762530, 93.81823441900311877 ) ) ;
#38685=VECTOR ( 'NONE', #11655, 1000.000000000000000 ) ;
#38686=CARTESIAN_POINT ( 'NONE',  ( 198.8948370720704588, 100.3380403442581752, -92.75881832202279043 ) ) ;
#38688=SURFACE_STYLE_USAGE ( .BOTH. , #65422 ) ;
#38691=B_SPLINE_CURVE_WITH_KNOTS ( 'NONE', 3,
 ( #28401, #49491, #34040, #44930, #60052, #18204, #60416, #2375, #66415, #29109, #55479, #1324, #22779, #17856, #23834, #67106, #39658, #18549, #33349, #45277, #54780, #61113, #12937, #12234, #2721, #13283, #6605, #23490, #65707, #33699, #50214, #49846, #7303, #56177, #50558, #17497, #34398, #55126, #1675, #7663, #23139, #44585, #66065, #55842, #39316 ),
 .UNSPECIFIED., .F., .F.,
 ( 4, 2, 2, 1, 2, 2, 2, 2, 2, 2, 2, 2, 2, 2, 2, 2, 2, 2, 2, 2, 2, 2, 4 ),
 ( 0.02345095402629350512, 0.02491692321306678351, 0.02564990780645342791, 0.02638289239984007578, 0.02711587699322672018, 0.02784886158661336458, 0.02931483077338667073, 0.03004781536677332901, 0.03078079996015999076, 0.03224676914693330732, 0.03297975374031995865, 0.03371273833370660306, 0.03517870752047990573, 0.03664467670725320148, 0.03737766130063985281, 0.03811064589402650415, 0.03957661508079981377, 0.04104258426757313033, 0.04250855345434643995, 0.04324153804773309823, 0.04397452264111975651, 0.04544049182789306612, 0.04690646101466638268 ),
 .UNSPECIFIED. ) ;
#38692=CARTESIAN_POINT ( 'NONE',  ( -121.5921196778231774, 43.72569502503143468, -75.42000096489594796 ) ) ;
#38696=CARTESIAN_POINT ( 'NONE',  ( 110.2429982417149432, 28.88204397445229077, -35.92243756565368784 ) ) ;
#38706=CARTESIAN_POINT ( 'NONE',  ( -74.17694007417655655, 20.66176641130876135, 43.94577668441134222 ) ) ;
#38708=CARTESIAN_POINT ( 'NONE',  ( 133.1039262992642591, 40.97158229895780579, -89.74086916301752126 ) ) ;
#38710=CARTESIAN_POINT ( 'NONE',  ( -144.3945994505580757, 59.96115386701888639, -74.64976673323776879 ) ) ;
#38712=CYLINDRICAL_SURFACE ( 'NONE', #68746, 7.500000000000013323 ) ;
#38716=CARTESIAN_POINT ( 'NONE',  ( 32.15284246740100116, 8.588257691344876932, 39.35317935462418859 ) ) ;
#38718=CARTESIAN_POINT ( 'NONE',  ( -180.4651598106648294, 97.28730001475658185, -40.66035573052959506 ) ) ;
#38719=CARTESIAN_POINT ( 'NONE',  ( -127.6992109187852265, 47.69334801994797601, -22.86298476009724467 ) ) ;
#38722=B_SPLINE_CURVE_WITH_KNOTS ( 'NONE', 3,
 ( #7774, #24651, #23607, #24307, #8113, #34858, #7433, #2494, #51378, #3194, #14084, #39774, #55962, #39425, #12699, #2152, #29563, #40465, #66876, #13059, #35191, #23947, #51027, #55247, #66528, #49976, #45045, #60876, #56646, #45749, #61235, #61909, #34165, #8466, #2841, #67229, #13733, #29918, #18674, #61584, #46086, #7070, #44708 ),
 .UNSPECIFIED., .F., .F.,
 ( 4, 2, 2, 2, 2, 2, 2, 2, 2, 2, 2, 2, 1, 2, 2, 2, 2, 2, 2, 2, 2, 4 ),
 ( 0.02390068823634510647, 0.02538837671117073411, 0.02613222094858354966, 0.02687606518599636521, 0.02836375366082197896, 0.02985144213564758925, 0.03059528637306041521, 0.03133913061047324117, 0.03282681908529890696, 0.03431450756012456582, 0.03580219603495023162, 0.03654604027236305064, 0.03728988450977585578, 0.03803372874718866786, 0.03877757298460147994, 0.04026526145942714574, 0.04175294993425280460, 0.04324063840907846346, 0.04398448264649129635, 0.04472832688390412231, 0.04621601535872980893, 0.04770370383355549554 ),
 .UNSPECIFIED. ) ;
#38727=FACE_BOUND ( 'NONE', #17557, .T. ) ;
#38728=CARTESIAN_POINT ( 'NONE',  ( -4.070918861171934466, 6.675509947362631813, -63.26537528929446097 ) ) ;
#38730=CARTESIAN_POINT ( 'NONE',  ( -176.3763474213711220, 92.36993073950279154, 58.39546644310473766 ) ) ;
#38736=CARTESIAN_POINT ( 'NONE',  ( -151.6716822472524200, 66.03661194063732864, 4.181547750986519318 ) ) ;
#38737=CARTESIAN_POINT ( 'NONE',  ( -74.62027799914388027, 20.82126111774559618, -89.97495102220065633 ) ) ;
#38739=CARTESIAN_POINT ( 'NONE',  ( -15.13211202216340645, 8.488266782358815377, 35.90622617973726705 ) ) ;
#38740=CARTESIAN_POINT ( 'NONE',  ( 114.4640969196985765, 30.88424258798502109, 4.062649201705831103 ) ) ;
#38741=CARTESIAN_POINT ( 'NONE',  ( 93.87111289824407834, 23.09598275302506210, -14.46140212872976960 ) ) ;
#38745=CARTESIAN_POINT ( 'NONE',  ( -36.37229078872273647, 11.47648211215765279, 5.201659389993076310 ) ) ;
#38747=CARTESIAN_POINT ( 'NONE',  ( -78.66644367742111399, -170.0000000000000000, 91.60730232060049616 ) ) ;
#38748=CARTESIAN_POINT ( 'NONE',  ( 79.14113188808480004, 18.05280674635441684, -69.67520535789378755 ) ) ;
#38749=CARTESIAN_POINT ( 'NONE',  ( 107.1638638624856554, 28.58522774667099853, 83.95379775939885292 ) ) ;
#38750=CARTESIAN_POINT ( 'NONE',  ( 69.36122620657974380, -170.0000000000000000, 94.99999999999866418 ) ) ;
#38751=CARTESIAN_POINT ( 'NONE',  ( -15.30012024911653334, 7.493578574797995273, 90.60732787615089023 ) ) ;
#38752=CARTESIAN_POINT ( 'NONE',  ( -25.48750459758502629, 9.705678256319565378, -47.40729988162036079 ) ) ;
#38760=CARTESIAN_POINT ( 'NONE',  ( 32.66883187925818532, 8.640402022338117050, 60.91819067178263225 ) ) ;
#38761=CARTESIAN_POINT ( 'NONE',  ( 177.5945652320814077, 75.14951358071817822, 70.29580567297929861 ) ) ;
#38763=EDGE_CURVE ( 'NONE', #9201, #10179, #41943, .T. ) ;
#38766=EDGE_CURVE ( 'NONE', #50285, #7511, #56699, .T. ) ;
#38770=CARTESIAN_POINT ( 'NONE',  ( 92.95016907945944240, 22.74936990452175678, 6.323048487394066441 ) ) ;
#38771=CARTESIAN_POINT ( 'NONE',  ( -15.32520546926282989, 7.495995523981874520, 64.95300774305263758 ) ) ;
#38773=CARTESIAN_POINT ( 'NONE',  ( -80.35638419094748031, 24.05227397169793591, -88.98511473825129769 ) ) ;
#38774=CARTESIAN_POINT ( 'NONE',  ( 39.40195752203892710, 8.409560354027398432, -23.77526687496409608 ) ) ;
#38776=FACE_BOUND ( 'NONE', #41591, .T. ) ;
#38780=CARTESIAN_POINT ( 'NONE',  ( 133.8566784816069060, 42.60093787723655367, 17.66579024853170310 ) ) ;
#38781=CARTESIAN_POINT ( 'NONE',  ( 91.50468583833760761, 22.21368636549395248, -49.04210192657487255 ) ) ;
#38783=CARTESIAN_POINT ( 'NONE',  ( -47.65155309726505095, 13.85482731128118061, 63.42320367329789832 ) ) ;
#38784=CARTESIAN_POINT ( 'NONE',  ( -180.5234362879039622, 97.35934147644941561, 12.72465163773038377 ) ) ;
#38785=CARTESIAN_POINT ( 'NONE',  ( 211.3710169359754332, 117.8057917113659840, 60.11802606744021915 ) ) ;
#38786=CARTESIAN_POINT ( 'NONE',  ( 86.62931800182293784, 19.42108912189599579, -62.66611478937537782 ) ) ;
#38791=CARTESIAN_POINT ( 'NONE',  ( 61.09275639403234237, 12.23448398202909182, 3.202934752445754096 ) ) ;
#38793=CARTESIAN_POINT ( 'NONE',  ( -61.75956139478100226, 16.58288496614412111, 61.29573688743341364 ) ) ;
#38795=ORIENTED_EDGE ( 'NONE', *, *, #48172, .T. ) ;
#38796=VECTOR ( 'NONE', #22021, 1000.000000000000000 ) ;
#38799=CARTESIAN_POINT ( 'NONE',  ( 103.5588133492864813, 25.91050225236390858, 33.67192454186398010 ) ) ;
#38803=CARTESIAN_POINT ( 'NONE',  ( 157.4703587214989113, 58.92748579479261650, 29.40946747225336466 ) ) ;
#38804=CARTESIAN_POINT ( 'NONE',  ( 103.5849290181279088, 27.01613348792539071, 6.804909383962445268 ) ) ;
#38805=CARTESIAN_POINT ( 'NONE',  ( 70.50376765786472788, 15.57629333413342998, 9.978129533752355229 ) ) ;
#38806=CARTESIAN_POINT ( 'NONE',  ( 204.6977192012829789, 106.3443248447423315, 17.36317014830577321 ) ) ;
#38807=CARTESIAN_POINT ( 'NONE',  ( 102.7414208686707582, 26.65627265923296818, -16.08848679405983262 ) ) ;
#38808=CARTESIAN_POINT ( 'NONE',  ( -47.79955240516186876, 13.88975739862082470, 9.000507506480387221 ) ) ;
#38809=CARTESIAN_POINT ( 'NONE',  ( -133.0835080491124813, 52.64966140620841628, -17.72071528858218059 ) ) ;
#38811=CARTESIAN_POINT ( 'NONE',  ( 68.22258291815838049, 13.94003497920737011, -91.44893492023997794 ) ) ;
#38812=CARTESIAN_POINT ( 'NONE',  ( 93.99232916046767627, 22.06612048408747384, 89.43417854994513050 ) ) ;
#38816=EDGE_CURVE ( 'NONE', #65087, #14549, #39477, .T. ) ;
#38820=CARTESIAN_POINT ( 'NONE',  ( -53.38256734720887664, 14.24001356352779979, -23.18744243301667751 ) ) ;
#38821=CARTESIAN_POINT ( 'NONE',  ( 108.3906473026529653, 28.03385344351496400, -9.295257895322684760 ) ) ;
#38823=CARTESIAN_POINT ( 'NONE',  ( -57.43883374585512769, 16.37892664338858850, -35.60189161719256390 ) ) ;
#38825=CARTESIAN_POINT ( 'NONE',  ( 204.6977192012829789, -170.0000000000000000, 63.55227132923313604 ) ) ;
#38826=CARTESIAN_POINT ( 'NONE',  ( -71.21970990337018748, 19.62334883444993494, -70.48616352051527656 ) ) ;
#38827=CARTESIAN_POINT ( 'NONE',  ( 23.23895241123074840, 6.853530908437178937, -17.16259189106778749 ) ) ;
#38834=CARTESIAN_POINT ( 'NONE',  ( -142.1332311300252798, 59.44822332309657043, 9.980626331248242167 ) ) ;
#38836=CARTESIAN_POINT ( 'NONE',  ( -57.76231208694425590, 16.46985661704315618, -89.40870754664922515 ) ) ;
#38837=CARTESIAN_POINT ( 'NONE',  ( -24.01966911771076241, 9.505735805909457881, 92.54941079593402264 ) ) ;
#38838=CARTESIAN_POINT ( 'NONE',  ( -95.05546640093035649, 29.25972325950978004, -44.59432911818360168 ) ) ;
#38839=VECTOR ( 'NONE', #15163, 1000.000000000000000 ) ;
#38840=CARTESIAN_POINT ( 'NONE',  ( -106.6781182590523542, 35.07133425426477658, 17.26811540876042983 ) ) ;
#38842=CARTESIAN_POINT ( 'NONE',  ( 136.1215428813736708, 43.99260314811118633, -23.84356242264301784 ) ) ;
#38844=EDGE_LOOP ( 'NONE', ( #36239, #68645, #51551, #57807 ) ) ;
#38846=ORIENTED_EDGE ( 'NONE', *, *, #30279, .F. ) ;
#38850=CARTESIAN_POINT ( 'NONE',  ( -13.47230132170245120, 7.324574289401432736, 15.73105565795967031 ) ) ;
#38851=CARTESIAN_POINT ( 'NONE',  ( 32.28603806442398394, 7.590310383548725781, -72.38435536236562484 ) ) ;
#38852=CARTESIAN_POINT ( 'NONE',  ( 60.40277045393653310, 12.08176563382369828, -9.341763661136180730 ) ) ;
#38853=EDGE_CURVE ( 'NONE', #9471, #36296, #66581, .T. ) ;
#38859=CARTESIAN_POINT ( 'NONE',  ( 188.2950976467627697, 87.71503060978560029, 65.73591284412599123 ) ) ;
#38860=CARTESIAN_POINT ( 'NONE',  ( -154.7934364910360330, 68.79594655117534785, 70.39161810400815966 ) ) ;
#38861=CARTESIAN_POINT ( 'NONE',  ( -1.866625526081663322, 7.583073082893621475, -38.33698315850279670 ) ) ;
#38862=CARTESIAN_POINT ( 'NONE',  ( 102.8518012651273494, 25.61025413220826863, 11.56502006215868050 ) ) ;
#38863=CARTESIAN_POINT ( 'NONE',  ( -170.4515722736647092, 84.20506723175657271, -88.88108375465611743 ) ) ;
#38864=CARTESIAN_POINT ( 'NONE',  ( -79.62258606008209938, 22.68765733708495347, -50.06947209741141336 ) ) ;
#38865=FACE_BOUND ( 'NONE', #48005, .T. ) ;
#38869=CARTESIAN_POINT ( 'NONE',  ( 181.0840389613909736, 78.60582251573003987, 29.30859410551139277 ) ) ;
#38872=CARTESIAN_POINT ( 'NONE',  ( 60.61895554631706062, 13.15982272268127851, -62.94199435588256364 ) ) ;
#38877=CARTESIAN_POINT ( 'NONE',  ( 183.1997226035582003, 80.77024518673746911, 83.29662567210579027 ) ) ;
#38881=DIRECTION ( 'NONE',  ( -1.000000000000000000, 0.000000000000000000, 0.000000000000000000 ) ) ;
#38883=ORIENTED_EDGE ( 'NONE', *, *, #45649, .F. ) ;
#38886=CARTESIAN_POINT ( 'NONE',  ( -74.79002408692173276, 20.88280597089421420, -36.19028926828421078 ) ) ;
#38890=CARTESIAN_POINT ( 'NONE',  ( -29.51272929882557250, 10.30144624948894361, -8.720126078648599233 ) ) ;
#38891=CARTESIAN_POINT ( 'NONE',  ( -50.14440374537738876, 14.45628984983895471, -10.17979503501909022 ) ) ;
#38893=ORIENTED_EDGE ( 'NONE', *, *, #62660, .F. ) ;
#38894=CARTESIAN_POINT ( 'NONE',  ( 111.8699272271189216, 29.64190505307780299, -50.74762732561652712 ) ) ;
#38897=CARTESIAN_POINT ( 'NONE',  ( 41.09671232177015554, 8.635892912882335182, -50.42995035429531470 ) ) ;
#38899=CARTESIAN_POINT ( 'NONE',  ( -120.2252778751027478, 42.87312880338508592, 86.88807202166155719 ) ) ;
#38901=CARTESIAN_POINT ( 'NONE',  ( 8.000000000000007105, 249.8719672152120381, -95.00000000000133582 ) ) ;
#38903=ORIENTED_EDGE ( 'NONE', *, *, #36532, .T. ) ;
#38904=CARTESIAN_POINT ( 'NONE',  ( -129.4098618459772467, 48.85263848239745244, 31.49111774146622622 ) ) ;
#38905=FACE_OUTER_BOUND ( 'NONE', #61943, .T. ) ;
#38907=CARTESIAN_POINT ( 'NONE',  ( 93.72687053612523300, 23.04134601640627622, 34.73706976770577626 ) ) ;
#38909=CARTESIAN_POINT ( 'NONE',  ( -120.1497954511983295, 42.82624472369556656, 60.11543276227916266 ) ) ;
#38911=CARTESIAN_POINT ( 'NONE',  ( 93.92280655489130936, 22.03989931749464404, -71.93211272359918951 ) ) ;
#38917=ADVANCED_FACE ( 'NONE', ( #45095 ), #8867, .F. ) ;
#38918=CARTESIAN_POINT ( 'NONE',  ( 46.13320811200730276, 9.380653113584042302, 34.06983411699128794 ) ) ;
#38919=CARTESIAN_POINT ( 'NONE',  ( 200.4600337307565781, 100.7087439352120981, -10.77597343189907342 ) ) ;
#38921=CARTESIAN_POINT ( 'NONE',  ( -190.3074740493607351, 108.5764897054613414, 61.38473446933937794 ) ) ;
#38922=CARTESIAN_POINT ( 'NONE',  ( 211.1046732743773191, 117.3965485104337461, -39.91724935795743789 ) ) ;
#38923=CARTESIAN_POINT ( 'NONE',  ( -71.42007367207963853, 20.75704712149297393, -71.45956786119569415 ) ) ;
#38925=CARTESIAN_POINT ( 'NONE',  ( -25.48237668717800375, 8.689083390666773710, -38.23367346561963132 ) ) ;
#38926=CARTESIAN_POINT ( 'NONE',  ( 163.1265310614426767, 62.18610413911356716, -75.40005345542890325 ) ) ;
#38929=CARTESIAN_POINT ( 'NONE',  ( -28.13128612339709633, 10.08889185338652084, 17.62085998369287054 ) ) ;
#38933=CARTESIAN_POINT ( 'NONE',  ( -82.77834200299112410, 23.92990355093956012, 85.30423727294719072 ) ) ;
#38934=CARTESIAN_POINT ( 'NONE',  ( -85.75222301046098039, 25.14826148333819233, 67.27150280759872203 ) ) ;
#38935=EDGE_CURVE ( 'NONE', #56347, #58835, #8314, .T. ) ;
#38936=CARTESIAN_POINT ( 'NONE',  ( 126.4633682455861816, 38.28837286275646790, 38.29824169173695481 ) ) ;
#38940=CARTESIAN_POINT ( 'NONE',  ( -100.4440683050664802, 32.98184228837414622, -8.383530731465961949 ) ) ;
#38943=CARTESIAN_POINT ( 'NONE',  ( 211.8283568324397095, 116.6646490157212810, 92.73083172464008328 ) ) ;
#38946=CARTESIAN_POINT ( 'NONE',  ( -128.7650348665116837, 48.41336321950710442, 71.89692748193580485 ) ) ;
#38948=CARTESIAN_POINT ( 'NONE',  ( 11.20486344102687681, 7.403248964808831545, -63.90658810494937114 ) ) ;
#38949=CARTESIAN_POINT ( 'NONE',  ( -9.779603649692305112, 8.034615131607072414, 18.02880719371939833 ) ) ;
#38952=CARTESIAN_POINT ( 'NONE',  ( -94.87734348028330089, 29.17663635873013561, -95.00000000000133582 ) ) ;
#38957=CARTESIAN_POINT ( 'NONE',  ( -133.1527834403230202, 51.46311219732125153, 13.18024344451227492 ) ) ;
#38958=CARTESIAN_POINT ( 'NONE',  ( -165.6215009671260532, 80.58889799860440917, -41.89784876661412483 ) ) ;
#38960=ORIENTED_EDGE ( 'NONE', *, *, #13682, .F. ) ;
#38963=CARTESIAN_POINT ( 'NONE',  ( -144.9439644317224349, 60.40328483334189258, -21.42479971859992460 ) ) ;
#38964=CARTESIAN_POINT ( 'NONE',  ( -142.1403563221901436, 58.17414631827835336, 93.35838044322102292 ) ) ;
#38966=ORIENTED_EDGE ( 'NONE', *, *, #12159, .T. ) ;
#38967=CARTESIAN_POINT ( 'NONE',  ( -59.95412189755934662, 17.09836075175410386, 5.275069537795150865 ) ) ;
#38968=CARTESIAN_POINT ( 'NONE',  ( 200.4559562755961792, 100.7034888016685841, -50.02848380335337453 ) ) ;
#38970=CARTESIAN_POINT ( 'NONE',  ( 157.4703587214989113, 58.92748579479261650, 29.40946747225336466 ) ) ;
#38971=CARTESIAN_POINT ( 'NONE',  ( -57.43251939610648549, 15.33203492375495891, 3.843832803641082041 ) ) ;
#38978=CARTESIAN_POINT ( 'NONE',  ( -121.0374639672267989, 43.37850281258126728, -90.38315847734473607 ) ) ;
#38979=LINE ( 'NONE', #5897, #32713 ) ;
#38981=CARTESIAN_POINT ( 'NONE',  ( -15.27733754929849752, 8.502213909106947298, -68.78387266333825778 ) ) ;
#38986=AXIS2_PLACEMENT_3D ( 'NONE', #68038, #62402, #36014 ) ;
#38990=ADVANCED_FACE ( 'NONE', ( #41217 ), #25047, .F. ) ;
#38992=CARTESIAN_POINT ( 'NONE',  ( -37.92511097250854846, 10.74631978746600680, -12.19873838909606256 ) ) ;
#38994=CARTESIAN_POINT ( 'NONE',  ( -128.1282195935087316, 49.19720162550163423, 4.112327430167169062 ) ) ;
#39003=CARTESIAN_POINT ( 'NONE',  ( -33.83558513595455963, 9.996963989836508802, -35.70617816557648894 ) ) ;
#39004=CARTESIAN_POINT ( 'NONE',  ( -102.9107985116279451, 33.10231825923204241, 84.22887737053727619 ) ) ;
#39005=CARTESIAN_POINT ( 'NONE',  ( -143.8794621588508278, 59.54894433207190474, 33.25729526067438968 ) ) ;
#39006=CARTESIAN_POINT ( 'NONE',  ( -132.4951995226845156, 50.99687809989501375, 61.39550820969922285 ) ) ;
#39007=CARTESIAN_POINT ( 'NONE',  ( -72.77296415263757012, 21.23032531836539150, -20.43596273929950513 ) ) ;
#39011=CARTESIAN_POINT ( 'NONE',  ( 37.46254810722764717, 8.164772623042713562, 30.15249803224812197 ) ) ;
#39014=EDGE_CURVE ( 'NONE', #44762, #65087, #20023, .T. ) ;
#39017=CARTESIAN_POINT ( 'NONE',  ( -120.1346137380982242, 44.00127440773566434, 60.15369630792869771 ) ) ;
#39018=CARTESIAN_POINT ( 'NONE',  ( -52.68007207639879397, 14.05813534436551215, 3.853851446599284358 ) ) ;
#39020=CARTESIAN_POINT ( 'NONE',  ( 150.2794558856211040, 52.26944788078748161, -41.42442129602201106 ) ) ;
#39024=CARTESIAN_POINT ( 'NONE',  ( -109.5949300668648476, 36.65467447298198067, -94.53065599267198138 ) ) ;
#39029=ORIENTED_EDGE ( 'NONE', *, *, #24217, .T. ) ;
#39030=CARTESIAN_POINT ( 'NONE',  ( -85.75947274862033964, 25.15128705015479227, 35.42982735500162050 ) ) ;
#39032=CARTESIAN_POINT ( 'NONE',  ( 41.33434189587760699, 9.684413566891869607, 44.66476443964724297 ) ) ;
#39035=ORIENTED_EDGE ( 'NONE', *, *, #38644, .F. ) ;
#39039=DIRECTION ( 'NONE',  ( -0.000000000000000000, 1.000000000000000000, -0.000000000000000000 ) ) ;
#39040=FACE_OUTER_BOUND ( 'NONE', #23860, .T. ) ;
#39041=CARTESIAN_POINT ( 'NONE',  ( -1.866625526081660880, 7.583073082893622363, 15.35211802242455725 ) ) ;
#39042=CARTESIAN_POINT ( 'NONE',  ( 138.8350590320874574, 45.70671380708321863, 85.08020996455034890 ) ) ;
#39044=PLANE ( 'NONE',  #44808 ) ;
#39046=AXIS2_PLACEMENT_3D ( 'NONE', #48723, #54000, #915 ) ;
#39047=ORIENTED_EDGE ( 'NONE', *, *, #58052, .F. ) ;
#39051=CARTESIAN_POINT ( 'NONE',  ( 161.7209903610255424, 61.03262545641851489, -10.58304253588356936 ) ) ;
#39054=CARTESIAN_POINT ( 'NONE',  ( 138.5684226926155702, 45.53585076428270639, 16.02087130590416564 ) ) ;
#39055=DIRECTION ( 'NONE',  ( 0.000000000000000000, 0.000000000000000000, 1.000000000000000000 ) ) ;
#39058=ORIENTED_EDGE ( 'NONE', *, *, #16264, .T. ) ;
#39061=EDGE_CURVE ( 'NONE', #22304, #32549, #16198, .T. ) ;
#39064=CARTESIAN_POINT ( 'NONE',  ( -147.7860806339124906, 62.73248524776228408, -76.47009865734850109 ) ) ;
#39065=CARTESIAN_POINT ( 'NONE',  ( 88.28780346671261725, 19.99350429399657969, 3.049271561570116251 ) ) ;
#39072=CARTESIAN_POINT ( 'NONE',  ( 70.10996765587415780, 15.47155867340926960, 88.54573586507250127 ) ) ;
#39074=CARTESIAN_POINT ( 'NONE',  ( 36.30999198706540199, 9.040534725358950752, 44.25116645233489265 ) ) ;
#39075=CARTESIAN_POINT ( 'NONE',  ( -180.0154536325056540, 96.73346874014738717, -39.24493656227331684 ) ) ;
#39076=CARTESIAN_POINT ( 'NONE',  ( -132.4819073909166320, 50.98736898418876251, -11.94662083526208285 ) ) ;
#39080=ADVANCED_FACE ( 'NONE', ( #50998 ), #55570, .F. ) ;
#39089=CARTESIAN_POINT ( 'NONE',  ( -5.401648928593175469, 6.744888135494086612, -62.64828587876987598 ) ) ;
#39090=CARTESIAN_POINT ( 'NONE',  ( -34.06637338149494099, 11.05895377318623218, 30.68749078464274760 ) ) ;
#39091=CARTESIAN_POINT ( 'NONE',  ( 14.11945145860287809, 7.458327016560931000, -89.34736952536303534 ) ) ;
#39092=DIRECTION ( 'NONE',  ( 0.000000000000000000, 0.000000000000000000, 1.000000000000000000 ) ) ;
#39098=CARTESIAN_POINT ( 'NONE',  ( 164.9709596662455908, 63.72607097915132357, 10.32857681705704067 ) ) ;
#39099=CARTESIAN_POINT ( 'NONE',  ( -49.66729301550846998, 14.33905798229759121, -91.16771365468441957 ) ) ;
#39106=CARTESIAN_POINT ( 'NONE',  ( 83.59652366361575559, 19.46709838196858655, -63.30246192554085383 ) ) ;
#39107=CARTESIAN_POINT ( 'NONE',  ( 115.2886225100560438, 32.40839894504812690, 85.24140403135865540 ) ) ;
#39109=CARTESIAN_POINT ( 'NONE',  ( -14.35185884954381308, 7.404296649871966451, 94.99999999999866418 ) ) ;
#39111=EDGE_CURVE ( 'NONE', #31650, #67324, #35956, .T. ) ;
#39115=CARTESIAN_POINT ( 'NONE',  ( -118.8392474096542344, 43.20060570451234838, -18.16838627151736674 ) ) ;
#39118=CARTESIAN_POINT ( 'NONE',  ( 35.65622260226242446, 8.964590916200315007, 70.76066538983499754 ) ) ;
#39125=CARTESIAN_POINT ( 'NONE',  ( 94.02861641584117081, 23.15570573563316259, 9.116654949391469032 ) ) ;
#39129=CARTESIAN_POINT ( 'NONE',  ( 211.5066273949819617, 116.1727691518061789, -20.17497244266030165 ) ) ;
#39130=FACE_BOUND ( 'NONE', #3761, .T. ) ;
#39131=CARTESIAN_POINT ( 'NONE',  ( -56.96214175905166854, 15.20165595797839941, -35.45940458566272468 ) ) ;
#39139=CARTESIAN_POINT ( 'NONE',  ( 208.9583973663598329, 114.1615900753670729, 57.36381220210540022 ) ) ;
#39141=AXIS2_PLACEMENT_3D ( 'NONE', #16729, #7238, #59632 ) ;
#39142=VERTEX_POINT ( 'NONE', #26619 ) ;
#39143=CARTESIAN_POINT ( 'NONE',  ( 60.62939143133406361, 12.13148391928980629, 3.341460604810993384 ) ) ;
#39145=VERTEX_POINT ( 'NONE', #21677 ) ;
#39150=CARTESIAN_POINT ( 'NONE',  ( -55.05276343752909440, 15.72344139423348430, -23.37177340799619785 ) ) ;
#39151=CARTESIAN_POINT ( 'NONE',  ( 106.6192711434718632, 27.24117154335862523, 30.54033420133337628 ) ) ;
#39153=ORIENTED_EDGE ( 'NONE', *, *, #51305, .F. ) ;
#39155=CARTESIAN_POINT ( 'NONE',  ( 162.0862735437576134, 62.63196145447164298, 30.97879343093337212 ) ) ;
#39158=DIRECTION ( 'NONE',  ( 1.000000000000000000, 0.000000000000000000, -0.000000000000000000 ) ) ;
#39159=ADVANCED_FACE ( 'NONE', ( #11122 ), #65291, .F. ) ;
#39161=CARTESIAN_POINT ( 'NONE',  ( -50.14523569787235147, 14.45648954445650602, 5.279614992475671897 ) ) ;
#39162=CARTESIAN_POINT ( 'NONE',  ( -132.6092625803567273, 52.31125232006262138, -12.21942496479799800 ) ) ;
#39163=ADVANCED_FACE ( 'NONE', ( #17442 ), #17085, .F. ) ;
#39173=CARTESIAN_POINT ( 'NONE',  ( -48.56549579811112238, 13.03742088415615896, 41.61317450176976251 ) ) ;
#39176=CARTESIAN_POINT ( 'NONE',  ( -60.64199216239839529, 17.30050036439945060, -47.72342124229984250 ) ) ;
#39179=CARTESIAN_POINT ( 'NONE',  ( -10.46803069297986788, 7.077485182625209426, 44.63888823349410018 ) ) ;
#39180=ORIENTED_EDGE ( 'NONE', *, *, #4436, .F. ) ;
#39185=CARTESIAN_POINT ( 'NONE',  ( -144.3939084932120807, 61.25241660819418144, 16.86807984998707255 ) ) ;
#39186=CARTESIAN_POINT ( 'NONE',  ( -166.3205068063721512, 81.30869308872871670, 35.14705211311118660 ) ) ;
#39190=CARTESIAN_POINT ( 'NONE',  ( -102.7502407665687372, 33.01985383847076605, 18.67452391595144690 ) ) ;
#39194=EDGE_LOOP ( 'NONE', ( #6390, #66279, #27964, #32857 ) ) ;
#39196=VERTEX_POINT ( 'NONE', #22728 ) ;
#39198=CARTESIAN_POINT ( 'NONE',  ( -15.13254930056756642, 7.477527548005403091, 12.47888104443209123 ) ) ;
#39199=CARTESIAN_POINT ( 'NONE',  ( 36.08729376665095145, 8.001156100723207487, -63.21872957073706800 ) ) ;
#39200=CARTESIAN_POINT ( 'NONE',  ( 59.29615173875419032, 11.84060224810187911, -22.89344993205446244 ) ) ;
#39201=CARTESIAN_POINT ( 'NONE',  ( -47.68743014591520080, 12.82957810971108081, 39.29583277014084786 ) ) ;
#39204=CARTESIAN_POINT ( 'NONE',  ( 204.6977192012829789, -170.0000000000000000, 17.36317014830577321 ) ) ;
#39208=CARTESIAN_POINT ( 'NONE',  ( -165.9986675144415358, 79.53506019208352029, 13.84447030584273364 ) ) ;
#39210=FACE_BOUND ( 'NONE', #51078, .T. ) ;
#39211=CARTESIAN_POINT ( 'NONE',  ( -189.4814416122051455, 107.4245629773156594, 90.19736142070722451 ) ) ;
#39214=CARTESIAN_POINT ( 'NONE',  ( -130.5740389938243311, 49.65308610043482673, -63.37811513693232257 ) ) ;
#39216=CARTESIAN_POINT ( 'NONE',  ( 42.71504753277074684, 8.863481902720376837, -63.23136117686474478 ) ) ;
#39218=VERTEX_POINT ( 'NONE', #59310 ) ;
#39221=FACE_OUTER_BOUND ( 'NONE', #48055, .T. ) ;
#39223=CARTESIAN_POINT ( 'NONE',  ( 186.9579425186612696, 84.75281520165634674, 85.82254035461609476 ) ) ;
#39228=CARTESIAN_POINT ( 'NONE',  ( 152.1153500913667642, 54.85403770686899350, 42.16645570227397855 ) ) ;
#39229=CARTESIAN_POINT ( 'NONE',  ( 204.6977192012829789, 106.3443248447423315, -36.32593103262158252 ) ) ;
#39231=CARTESIAN_POINT ( 'NONE',  ( 117.6924004117966263, 33.61107268965019301, 62.94190954259333637 ) ) ;
#39233=CARTESIAN_POINT ( 'NONE',  ( -179.0654441437003186, 93.99779465816536117, 6.897009515522955603 ) ) ;
#39234=CARTESIAN_POINT ( 'NONE',  ( -72.21652659655764239, 19.96855882996549170, -46.47546056419784577 ) ) ;
#39235=CARTESIAN_POINT ( 'NONE',  ( 80.22637088046110421, 17.33468451430266200, -93.08378292954130018 ) ) ;
#39237=CARTESIAN_POINT ( 'NONE',  ( 23.09119322872580682, 6.844329382916375160, -95.00000000000133582 ) ) ;
#39238=CARTESIAN_POINT ( 'NONE',  ( -48.71337292867759317, 14.10768470390588902, -11.85640319484388705 ) ) ;
#39244=CARTESIAN_POINT ( 'NONE',  ( -142.5042386072304623, 59.74110826975217492, -45.04988858504612637 ) ) ;
#39247=CARTESIAN_POINT ( 'NONE',  ( -132.6811329440527061, 51.12842468617797920, 94.99999999999866418 ) ) ;
#39249=CARTESIAN_POINT ( 'NONE',  ( 84.28078136020374700, 18.63296074526051882, -36.19471234886871969 ) ) ;
#39251=VERTEX_POINT ( 'NONE', #46521 ) ;
#39252=CARTESIAN_POINT ( 'NONE',  ( -125.8938041572051389, 46.49392987655492249, 30.61994787315706290 ) ) ;
#39253=CARTESIAN_POINT ( 'NONE',  ( 81.57915404881516963, 18.81499384983930767, 31.66182794264046763 ) ) ;
#39255=CARTESIAN_POINT ( 'NONE',  ( 187.5272808203428099, 85.37192123373904451, -20.75736303806692007 ) ) ;
#39257=CARTESIAN_POINT ( 'NONE',  ( -125.8938041572051105, 46.49392987655492959, 57.46449846362076386 ) ) ;
#39258=CARTESIAN_POINT ( 'NONE',  ( 42.71247067544613429, 9.879726907348448606, 3.834988087375502008 ) ) ;
#39259=CARTESIAN_POINT ( 'NONE',  ( 93.32502112557681073, 21.81526022999038261, -73.58157134791495935 ) ) ;
#39261=ORIENTED_EDGE ( 'NONE', *, *, #41915, .T. ) ;
#39263=CARTESIAN_POINT ( 'NONE',  ( 43.35980717318837208, 8.957244490220908517, 43.78924419203700324 ) ) ;
#39264=CARTESIAN_POINT ( 'NONE',  ( 204.6977192012829789, 106.3443248447423173, -9.481380442157895772 ) ) ;
#39265=CYLINDRICAL_SURFACE ( 'NONE', #45868, 7.500000000000013323 ) ;
#39268=CARTESIAN_POINT ( 'NONE',  ( 207.2640160519426331, 111.6867652229576464, -50.87616464366998770 ) ) ;
#39269=CARTESIAN_POINT ( 'NONE',  ( -77.71490760329790248, 23.03637365463982078, -76.91457645186844161 ) ) ;
#39270=CARTESIAN_POINT ( 'NONE',  ( -149.5074843970971301, -170.0000000000000000, -88.50193171241930656 ) ) ;
#39271=CARTESIAN_POINT ( 'NONE',  ( -28.13852122803040601, 9.072484007196647937, -49.56943753559436061 ) ) ;
#39276=B_SPLINE_CURVE_WITH_KNOTS ( 'NONE', 3,
 ( #10761, #5486, #58259, #48038, #38185, #53309, #63889, #37491, #15699, #69497, #11105, #11438, #21315, #69157, #32568, #31881, #58942, #20979, #53995, #42763, #53663, #48717, #64226, #198, #32910, #559, #26940, #42431, #10411, #48367, #22013, #15359, #16040, #37149, #21660, #43110, #31537, #64579, #58594, #16391, #43453, #52969, #4460, #64932, #47348, #25919, #36819, #26261 ),
 .UNSPECIFIED., .F., .F.,
 ( 4, 2, 2, 2, 2, 2, 2, 2, 2, 2, 2, 2, 2, 2, 2, 2, 2, 2, 2, 2, 2, 2, 2, 4 ),
 ( 0.02746511744866864460, 0.02914922134997091976, 0.03083332525127319146, 0.03251742915257545274, 0.03335948110322661808, 0.03420153305387777648, 0.03504358500452893488, 0.03588563695518009328, 0.03756974085648236844, 0.03841179280713351296, 0.03925384475778465748, 0.04009589670843580200, 0.04093794865908693958, 0.04262205256038922863, 0.04430615646169151767, 0.04514820841234267607, 0.04599026036299384140, 0.04767436426429616514, 0.04935846816559849581, 0.05020052011624965421, 0.05104257206690081261, 0.05272667596820312941, 0.05356872791885426699, 0.05441077986950541151 ),
 .UNSPECIFIED. ) ;
#39281=CARTESIAN_POINT ( 'NONE',  ( -7.825402957745085430, -170.0000000000000000, 56.96013162991089018 ) ) ;
#39283=DIRECTION ( 'NONE',  ( 0.000000000000000000, -1.000000000000000000, 0.000000000000000000 ) ) ;
#39284=CARTESIAN_POINT ( 'NONE',  ( -97.48179118242302366, 31.52606332398821110, -21.45542205896860466 ) ) ;
#39285=CARTESIAN_POINT ( 'NONE',  ( 62.53356220515464514, 13.59349015304564112, 29.81296093922127000 ) ) ;
#39288=ORIENTED_EDGE ( 'NONE', *, *, #29169, .F. ) ;
#39290=CARTESIAN_POINT ( 'NONE',  ( -10.92576759990585700, 8.121994053275065184, 17.60457009605725887 ) ) ;
#39293=CARTESIAN_POINT ( 'NONE',  ( 130.3035708464390154, 40.48418876551455980, -10.05640674831288806 ) ) ;
#39296=VECTOR ( 'NONE', #33384, 1000.000000000000000 ) ;
#39298=CARTESIAN_POINT ( 'NONE',  ( -34.74563762132952149, 11.17960945723135602, -36.08099439004806186 ) ) ;
#39299=LINE ( 'NONE', #33335, #48036 ) ;
#39302=VERTEX_POINT ( 'NONE', #40904 ) ;
#39304=CARTESIAN_POINT ( 'NONE',  ( -7.825402957745085430, 6.891034867348157178, -8.573520141480125645 ) ) ;
#39306=EDGE_CURVE ( 'NONE', #35856, #56740, #64480, .T. ) ;
#39307=CARTESIAN_POINT ( 'NONE',  ( -7.825402957745087207, 7.899365992529248537, -62.26262132240749736 ) ) ;
#39309=CARTESIAN_POINT ( 'NONE',  ( 63.01563776193091826, -170.0000000000000000, -70.06524142263343435 ) ) ;
#39310=VERTEX_POINT ( 'NONE', #44533 ) ;
#39311=CARTESIAN_POINT ( 'NONE',  ( 160.3272647999154401, 61.19822819988351625, -90.36850820003876095 ) ) ;
#39312=CARTESIAN_POINT ( 'NONE',  ( 198.2545923567585362, 97.90679023593578734, -47.67529484694221509 ) ) ;
#39314=CARTESIAN_POINT ( 'NONE',  ( -95.60805465865863084, 30.63099276904602775, 34.55587408256688775 ) ) ;
#39316=CARTESIAN_POINT ( 'NONE',  ( 15.78827728214693416, 6.500811158483327468, -35.51894409868578606 ) ) ;
#39319=CARTESIAN_POINT ( 'NONE',  ( 59.08638499266955080, 11.79550614876701609, 30.91997476302164927 ) ) ;
#39321=ORIENTED_EDGE ( 'NONE', *, *, #41912, .F. ) ;
#39322=CARTESIAN_POINT ( 'NONE',  ( -71.16770070143911653, 19.60548673929831054, -16.29567994807987219 ) ) ;
#39323=ADVANCED_FACE ( 'NONE', ( #62004 ), #33987, .F. ) ;
#39325=CARTESIAN_POINT ( 'NONE',  ( -7.825402957745081878, 7.899365992529270741, -77.26262132240753999 ) ) ;
#39327=CARTESIAN_POINT ( 'NONE',  ( -94.81218273889635384, 30.25676132809585894, 92.47620566321978686 ) ) ;
#39332=CARTESIAN_POINT ( 'NONE',  ( 211.4997502125519304, 118.0043045815490643, -73.84422742146547591 ) ) ;
#39333=CARTESIAN_POINT ( 'NONE',  ( -38.15923928782688535, 10.79140400702259406, -12.63341888148066694 ) ) ;
#39334=CARTESIAN_POINT ( 'NONE',  ( -179.5186635612083705, 96.12511541314941610, 42.27427310839760111 ) ) ;
#39335=CARTESIAN_POINT ( 'NONE',  ( -132.9227230387960503, 52.53474289881227577, 13.90519458082851756 ) ) ;
#39336=CARTESIAN_POINT ( 'NONE',  ( 18.20314211955701467, 7.596739727129570241, 57.24165582558227783 ) ) ;
#39340=CIRCLE ( 'NONE', #47162, 242.4895526022646379 ) ;
#39341=CARTESIAN_POINT ( 'NONE',  ( 210.1083934089977276, 114.0683883068361979, -92.30473204684062694 ) ) ;
#39342=CARTESIAN_POINT ( 'NONE',  ( -108.6944271866238694, 37.30738480893075604, 15.09322670349537887 ) ) ;
#39343=FACE_OUTER_BOUND ( 'NONE', #11657, .T. ) ;
#39344=CARTESIAN_POINT ( 'NONE',  ( -38.69408084385329261, 10.89529537250242797, -40.85159504354631821 ) ) ;
#39345=CARTESIAN_POINT ( 'NONE',  ( -94.82654088125009650, 29.15296007446479365, 90.81183754180923984 ) ) ;
#39348=CARTESIAN_POINT ( 'NONE',  ( -71.42007367207961011, 20.75704712149298103, -17.77046668026834553 ) ) ;
#39350=CARTESIAN_POINT ( 'NONE',  ( 80.17205177205137545, 17.31791394718355193, 60.23348464139676395 ) ) ;
#39351=ORIENTED_EDGE ( 'NONE', *, *, #2469, .T. ) ;
#39352=CARTESIAN_POINT ( 'NONE',  ( 31.91375106836931508, 7.553354707452896832, 36.92584114580535726 ) ) ;
#39354=CARTESIAN_POINT ( 'NONE',  ( 184.0013086981203116, 81.60415045669144263, 43.73133913719384225 ) ) ;
#39357=CARTESIAN_POINT ( 'NONE',  ( -118.4106078162223241, 42.93830006159887347, 65.53424955688741704 ) ) ;
#39358=CARTESIAN_POINT ( 'NONE',  ( -47.56463531432803649, 12.80077789972091118, 11.46294120578592413 ) ) ;
#39360=CARTESIAN_POINT ( 'NONE',  ( 157.9121974517528599, 59.27335488206247049, -77.96873488960137877 ) ) ;
#39361=EDGE_LOOP ( 'NONE', ( #31989, #15933 ) ) ;
#39363=CARTESIAN_POINT ( 'NONE',  ( -109.6445876100719801, 36.68207583875867073, -94.76434699328210343 ) ) ;
#39371=CARTESIAN_POINT ( 'NONE',  ( 157.0316110297313514, 58.58403635656377872, -62.96873488960130771 ) ) ;
#39372=CARTESIAN_POINT ( 'NONE',  ( 62.53328835682435738, 12.56090025569837287, -50.72069083216976537 ) ) ;
#39373=CARTESIAN_POINT ( 'NONE',  ( 136.3292018078238925, 42.93753790426541883, -50.60784358443687125 ) ) ;
#39374=ORIENTED_EDGE ( 'NONE', *, *, #40268, .F. ) ;
#39379=FACE_OUTER_BOUND ( 'NONE', #32914, .T. ) ;
#39381=CARTESIAN_POINT ( 'NONE',  ( -1.455067768715152310, 7.566780179921177130, 14.73709619961304540 ) ) ;
#39382=CARTESIAN_POINT ( 'NONE',  ( -2.172839205444464739, 7.595638683704374117, 59.50596416994952875 ) ) ;
#39386=ORIENTED_EDGE ( 'NONE', *, *, #64362, .F. ) ;
#39389=CARTESIAN_POINT ( 'NONE',  ( 162.6190874793280159, 61.76782592053312726, -22.23833498129200237 ) ) ;
#39392=CARTESIAN_POINT ( 'NONE',  ( 141.2894128405439460, 46.09731134920845363, -69.33034730996990902 ) ) ;
#39396=ORIENTED_EDGE ( 'NONE', *, *, #38816, .T. ) ;
#39400=CARTESIAN_POINT ( 'NONE',  ( -60.97727891098332975, 16.35024395194892222, -74.18606411768185183 ) ) ;
#39401=LINE ( 'NONE', #60850, #24093 ) ;
#39402=EDGE_CURVE ( 'NONE', #14285, #53742, #64081, .T. ) ;
#39404=CARTESIAN_POINT ( 'NONE',  ( -142.5211356634642073, 58.47296527616903461, -71.89897564660120111 ) ) ;
#39409=CARTESIAN_POINT ( 'NONE',  ( 56.65085722429434156, 12.31291088688619872, 87.02077204420697853 ) ) ;
#39411=CARTESIAN_POINT ( 'NONE',  ( -180.5200658187031308, 97.35517482626556784, -43.47889771769175127 ) ) ;
#39412=CARTESIAN_POINT ( 'NONE',  ( -129.6001310305488801, 48.98284622040321068, -9.044787352631615818 ) ) ;
#39414=CARTESIAN_POINT ( 'NONE',  ( 127.6144785300460143, 37.78099129859913319, -74.53306838336926887 ) ) ;
#39416=CARTESIAN_POINT ( 'NONE',  ( 140.8855094313932739, 47.03549517811092784, -67.73839220523630900 ) ) ;
#39417=CARTESIAN_POINT ( 'NONE',  ( 86.62931800182293784, -170.0000000000000000, -23.97701360844805407 ) ) ;
#39419=CARTESIAN_POINT ( 'NONE',  ( -155.7457403566965866, 71.01814553754117298, -46.50655860890988436 ) ) ;
#39421=CARTESIAN_POINT ( 'NONE',  ( -32.41898580403139363, 10.77423026598440003, 45.16838497460151558 ) ) ;
#39423=CARTESIAN_POINT ( 'NONE',  ( -7.825402957745085430, 7.899365992529246761, 45.11558103944722120 ) ) ;
#39425=CARTESIAN_POINT ( 'NONE',  ( -49.14234466229832776, 13.17605306081208383, -74.18447387590266828 ) ) ;
#39426=CARTESIAN_POINT ( 'NONE',  ( -2.869721780807579226, 7.625909776230887616, -10.42278629837480075 ) ) ;
#39427=CARTESIAN_POINT ( 'NONE',  ( -11.14668121284976543, 8.139398342256731311, 44.34457400782481074 ) ) ;
#39429=CARTESIAN_POINT ( 'NONE',  ( -51.75505017849845757, 14.85991436727098680, -89.65576684818640274 ) ) ;
#39431=CARTESIAN_POINT ( 'NONE',  ( -98.67557579989349392, 32.10670856967969655, -49.10905532852981281 ) ) ;
#39434=B_SPLINE_CURVE_WITH_KNOTS ( 'NONE', 3,
 ( #32900, #43443, #42071, #32218, #31525, #15689, #58930, #37136, #37481, #16714, #11092, #58248, #21645, #10064, #69138, #37834, #20611, #5125 ),
 .UNSPECIFIED., .F., .F.,
 ( 4, 2, 2, 2, 2, 2, 2, 2, 4 ),
 ( 0.000000000000000000, 0.001383361344168719618, 0.002075042016253087016, 0.002766722688337454415, 0.004150084032506189645, 0.005533445376674925309, 0.006916806720843658371, 0.008300168065012393168, 0.01106689075334992868 ),
 .UNSPECIFIED. ) ;
#39435=CARTESIAN_POINT ( 'NONE',  ( 85.68197636629476222, 20.16141071296262055, -77.62144078439391137 ) ) ;
#39443=CYLINDRICAL_SURFACE ( 'NONE', #30813, 7.500000000000013323 ) ;
#39444=CARTESIAN_POINT ( 'NONE',  ( -120.1346137380982526, 44.00127440773566434, -20.37995546346237674 ) ) ;
#39448=CARTESIAN_POINT ( 'NONE',  ( 173.6020601204682237, 71.36108012062135231, 64.25024514119610330 ) ) ;
#39453=CARTESIAN_POINT ( 'NONE',  ( 103.0124792097646775, 26.77148435100180635, 61.89731518363151253 ) ) ;
#39454=CARTESIAN_POINT ( 'NONE',  ( -165.6215009671260816, 80.58889799860442338, -15.05329817615042742 ) ) ;
#39455=LINE ( 'NONE', #60209, #17295 ) ;
#39457=CARTESIAN_POINT ( 'NONE',  ( 90.30840373526895348, 21.77864858272153725, 3.827423155247575703 ) ) ;
#39458=CARTESIAN_POINT ( 'NONE',  ( -8.811275908848678284, 6.956777180392053062, 57.00910973746761812 ) ) ;
#39459=CARTESIAN_POINT ( 'NONE',  ( 14.08810621383466710, 7.458732232275135487, 57.05035383895328494 ) ) ;
#39462=FACE_BOUND ( 'NONE', #28558, .T. ) ;
#39468=CARTESIAN_POINT ( 'NONE',  ( 31.90170717962885405, 8.563261373066634263, -69.72421537717313811 ) ) ;
#39471=CARTESIAN_POINT ( 'NONE',  ( 211.7318474105134101, 118.3631723164074430, 60.93285753849514919 ) ) ;
#39474=CARTESIAN_POINT ( 'NONE',  ( 55.57657751403270652, 11.06944050856661654, 9.482223198364021499 ) ) ;
#39477=LINE ( 'NONE', #18721, #4779 ) ;
#39481=CARTESIAN_POINT ( 'NONE',  ( 93.87111289824406413, 23.09598275302505854, -68.15050330965711112 ) ) ;
#39487=CARTESIAN_POINT ( 'NONE',  ( -78.66644367742109978, 23.39876645725289706, 57.26275173013680586 ) ) ;
#39488=EDGE_CURVE ( 'NONE', #58835, #48695, #5345, .T. ) ;
#39489=CARTESIAN_POINT ( 'NONE',  ( 160.9097745014957752, 61.67033591969550343, 43.57822560071761586 ) ) ;
#39492=CARTESIAN_POINT ( 'NONE',  ( -149.5074843970970733, 65.50121172469317798, -61.65738112195564469 ) ) ;
#39493=CARTESIAN_POINT ( 'NONE',  ( 70.45451534980409747, 15.56315969138428734, 9.480703485068785241 ) ) ;
#39499=AXIS2_PLACEMENT_3D ( 'NONE', #50437, #41271, #14533 ) ;
#39500=CARTESIAN_POINT ( 'NONE',  ( -188.8754233303960746, 108.3048424661242137, 94.99999999999866418 ) ) ;
#39502=CARTESIAN_POINT ( 'NONE',  ( -11.12071801323846820, 8.136093035169569276, -89.81606957978225125 ) ) ;
#39503=CARTESIAN_POINT ( 'NONE',  ( 15.78827728214693416, 7.507518794609575608, 45.01470767270524931 ) ) ;
#39504=CARTESIAN_POINT ( 'NONE',  ( 117.0065308422768453, 32.13872219870571456, -19.82875574738446289 ) ) ;
#39505=CARTESIAN_POINT ( 'NONE',  ( 92.40591237198245267, 21.47348772973007769, 86.10604474285490539 ) ) ;
#39510=CARTESIAN_POINT ( 'NONE',  ( 43.96465529479667822, 9.046527005589322101, 4.596442995059748071 ) ) ;
#39511=CARTESIAN_POINT ( 'NONE',  ( -179.5301766695108086, 96.13943360322242881, 88.10265356730171504 ) ) ;
#39513=CARTESIAN_POINT ( 'NONE',  ( 104.3931729003987243, 26.26823401847090977, -11.85818687836022889 ) ) ;
#39514=CARTESIAN_POINT ( 'NONE',  ( 140.3489479654237186, 45.48511634645607415, -93.43377705359233687 ) ) ;
#39515=CARTESIAN_POINT ( 'NONE',  ( 197.4179691534359904, 98.47175324380101813, 88.57974532536528045 ) ) ;
#39517=CARTESIAN_POINT ( 'NONE',  ( -78.66644367742111399, 22.32174330031318377, -76.96000122218160300 ) ) ;
#39518=CARTESIAN_POINT ( 'NONE',  ( -9.525868120571905351, 7.007646177566256185, 44.92434374916574313 ) ) ;
#39522=ORIENTED_EDGE ( 'NONE', *, *, #35015, .F. ) ;
#39524=CARTESIAN_POINT ( 'NONE',  ( 181.9411407973024666, 80.91291802046382031, -63.06960825634326540 ) ) ;
#39525=CARTESIAN_POINT ( 'NONE',  ( -166.5742238910466142, 81.57147158222490191, 34.65224386300440074 ) ) ;
#39526=CARTESIAN_POINT ( 'NONE',  ( 117.4396227366912626, 32.35611529020199129, -95.00000000000133582 ) ) ;
#39527=CARTESIAN_POINT ( 'NONE',  ( -107.0584934212648420, 35.27493744466471526, 16.97611379505483953 ) ) ;
#39528=CARTESIAN_POINT ( 'NONE',  ( 63.01563776193091826, 13.70579113808095251, 56.65751152968497451 ) ) ;
#39529=CARTESIAN_POINT ( 'NONE',  ( 133.8566784816069060, 42.60093787723653236, -24.17876034193199786 ) ) ;
#39535=CARTESIAN_POINT ( 'NONE',  ( -15.07200981767290848, 7.471751903425209562, 12.71961635690741765 ) ) ;
#39537=CARTESIAN_POINT ( 'NONE',  ( 57.08336938683662964, 11.37442068895388836, -11.76070366654272981 ) ) ;
#39540=CARTESIAN_POINT ( 'NONE',  ( -49.14234466229832776, 13.17605306081208028, 33.19372848595200054 ) ) ;
#39548=DIRECTION ( 'NONE',  ( 0.000000000000000000, -1.000000000000000000, 0.000000000000000000 ) ) ;
#39550=FACE_BOUND ( 'NONE', #12474, .T. ) ;
#39556=CARTESIAN_POINT ( 'NONE',  ( -4.070918861171935355, 6.675509947362632701, 70.95737766302396210 ) ) ;
#39561=CARTESIAN_POINT ( 'NONE',  ( 178.1903523079567435, 75.72906488635187827, 29.87569773046720201 ) ) ;
#39564=CARTESIAN_POINT ( 'NONE',  ( 133.8566784816069344, -170.0000000000000000, 71.35489142945907304 ) ) ;
#39566=CARTESIAN_POINT ( 'NONE',  ( -130.9137245142390498, 49.88865066924345371, -90.51337433235501351 ) ) ;
#39567=CARTESIAN_POINT ( 'NONE',  ( 188.3360522968598616, 86.25934009027517391, 88.57512505238727840 ) ) ;
#39570=CARTESIAN_POINT ( 'NONE',  ( 173.9413349464227281, 71.67637800842359752, -46.02999054611672847 ) ) ;
#39571=CARTESIAN_POINT ( 'NONE',  ( -179.8996803435689174, 95.00451760716444483, -65.83508346284071422 ) ) ;
#39575=CARTESIAN_POINT ( 'NONE',  ( -179.9014775667593540, 95.00669833041662571, 8.259492724175739653 ) ) ;
#39576=CARTESIAN_POINT ( 'NONE',  ( -6.126800896373024052, 6.786243985899683473, 3.461768403377602610 ) ) ;
#39578=DIRECTION ( 'NONE',  ( -0.000000000000000000, 1.000000000000000000, -0.000000000000000000 ) ) ;
#39581=CARTESIAN_POINT ( 'NONE',  ( -47.80251179448167420, 13.89045662648309509, -13.88776572326466230 ) ) ;
#39585=CARTESIAN_POINT ( 'NONE',  ( -71.97658551692140350, 20.95070248419153103, 7.673782731213468544 ) ) ;
#39587=CARTESIAN_POINT ( 'NONE',  ( -166.5742238910465858, 81.57147158222490191, -72.72595849885027519 ) ) ;
#39590=CARTESIAN_POINT ( 'NONE',  ( 84.05098130332767425, 18.55728792516086401, -36.27452980240430946 ) ) ;
#39595=CARTESIAN_POINT ( 'NONE',  ( 84.05289558242219528, 19.61733656419350069, 30.16443369323296864 ) ) ;
#39597=CARTESIAN_POINT ( 'NONE',  ( 183.3913492984167988, 80.96922346472078402, -24.02000789587866691 ) ) ;
#39598=AXIS2_PLACEMENT_3D ( 'NONE', #18159, #28717, #13236 ) ;
#39599=CARTESIAN_POINT ( 'NONE',  ( 141.2811136745703209, 46.09188267874203149, -17.77400908926494694 ) ) ;
#39600=FACE_OUTER_BOUND ( 'NONE', #56873, .T. ) ;
#39601=CARTESIAN_POINT ( 'NONE',  ( -177.1514380519393512, 93.28180884530866024, -9.027143560223994001 ) ) ;
#39604=ORIENTED_EDGE ( 'NONE', *, *, #19720, .T. ) ;
#39609=CARTESIAN_POINT ( 'NONE',  ( 207.8398359204633152, 112.5208221429021478, -50.63919247862472162 ) ) ;
#39610=CARTESIAN_POINT ( 'NONE',  ( -74.79539698934958381, 21.95498232236882785, -75.88833620473140229 ) ) ;
#39611=CARTESIAN_POINT ( 'NONE',  ( -107.7743374187917169, 35.66028478413597469, 69.99245325170923593 ) ) ;
#39612=CARTESIAN_POINT ( 'NONE',  ( 39.40195752203892710, 9.424259417798134919, -50.61981746542779348 ) ) ;
#39613=CARTESIAN_POINT ( 'NONE',  ( 159.2319614735956463, 59.03334608081211599, -77.77237424278591504 ) ) ;
#39617=CARTESIAN_POINT ( 'NONE',  ( -8.811275908848687166, 6.956777180392055726, -50.36909262438710755 ) ) ;
#39618=ADVANCED_FACE ( 'NONE', ( #32767 ), #17636, .F. ) ;
#39620=CARTESIAN_POINT ( 'NONE',  ( -78.66644367742109978, 22.32174330031321574, 72.26275173013684139 ) ) ;
#39621=CARTESIAN_POINT ( 'NONE',  ( 127.2358066117907072, 38.72257733469226082, 33.44959100710425304 ) ) ;
#39624=CARTESIAN_POINT ( 'NONE',  ( -101.3502439362134737, 33.43728945125136676, -23.12672091462772883 ) ) ;
#39625=CARTESIAN_POINT ( 'NONE',  ( 59.73312635112156244, 12.96464920523511033, 30.55208854348506975 ) ) ;
#39626=CARTESIAN_POINT ( 'NONE',  ( 34.55331630735146575, 7.828237636019207635, 85.37150955030359967 ) ) ;
#39631=CARTESIAN_POINT ( 'NONE',  ( -189.5329886872042948, 107.4958891766010964, -44.24249695867173671 ) ) ;
#39633=CARTESIAN_POINT ( 'NONE',  ( -94.87734348028330089, -170.0000000000000000, -95.00000000000133582 ) ) ;
#39634=CARTESIAN_POINT ( 'NONE',  ( 197.8572563162090887, 97.41072138832258531, 66.64235681249728316 ) ) ;
#39635=CARTESIAN_POINT ( 'NONE',  ( 127.2107679985236217, 38.70844091144998345, -13.16384531823007897 ) ) ;
#39641=CARTESIAN_POINT ( 'NONE',  ( -126.7989199172159260, 47.09198523267863834, 3.816158964292980738 ) ) ;
#39646=CARTESIAN_POINT ( 'NONE',  ( -123.6699087229881968, 45.04696784753414818, -49.58003572520509294 ) ) ;
#39650=CARTESIAN_POINT ( 'NONE',  ( -0.3740447803642789060, 7.527031846085010081, -70.74654756650022591 ) ) ;
#39654=CARTESIAN_POINT ( 'NONE',  ( -55.53456145826333312, 15.85318253404851774, 3.472777182467473356 ) ) ;
#39656=CARTESIAN_POINT ( 'NONE',  ( -97.86516199987805464, 31.71158167298307617, 31.93729686093309184 ) ) ;
#39658=CARTESIAN_POINT ( 'NONE',  ( 22.29513692215317988, 6.796052026456506745, -46.78078019334662940 ) ) ;
#39659=CARTESIAN_POINT ( 'NONE',  ( 116.0963032583228483, 32.80867113471310148, 5.551094412785531063 ) ) ;
#39664=ORIENTED_EDGE ( 'NONE', *, *, #13251, .T. ) ;
#39665=CARTESIAN_POINT ( 'NONE',  ( 178.1888264190354505, 77.13727704498028004, 43.74063381377031590 ) ) ;
#39666=CARTESIAN_POINT ( 'NONE',  ( 23.23895241123075550, 6.853530908437178049, -70.85169307199515742 ) ) ;
#39667=PLANE ( 'NONE',  #48889 ) ;
#39669=CARTESIAN_POINT ( 'NONE',  ( -95.54114085644955878, 30.59949910443587839, 94.99999999999866418 ) ) ;
#39671=CARTESIAN_POINT ( 'NONE',  ( -72.21947956767114363, 21.03570528348187452, -46.45601792771012839 ) ) ;
#39673=CARTESIAN_POINT ( 'NONE',  ( 208.5884523568772693, 113.6152425727545250, -64.24464719657447631 ) ) ;
#39674=CARTESIAN_POINT ( 'NONE',  ( 139.3041645503688244, 46.00819478311335331, 31.84931363288263384 ) ) ;
#39676=CARTESIAN_POINT ( 'NONE',  ( -175.9944734395086527, 91.92390745845763433, 45.26234191262543050 ) ) ;
#39677=FACE_OUTER_BOUND ( 'NONE', #176, .T. ) ;
#39687=CARTESIAN_POINT ( 'NONE',  ( -38.16002576456689610, 10.79155573432543314, -46.15488383467597089 ) ) ;
#39689=CARTESIAN_POINT ( 'NONE',  ( -142.0685766576042397, 58.11789490499574384, 39.33001764120334087 ) ) ;
#39694=EDGE_CURVE ( 'NONE', #40482, #35601, #30119, .T. ) ;
#39697=CARTESIAN_POINT ( 'NONE',  ( 84.74140601443113496, 18.78541996275572856, 71.31910537301371278 ) ) ;
#39699=CARTESIAN_POINT ( 'NONE',  ( -95.15214927927195276, 30.41622044381585255, -93.85950614209359344 ) ) ;
#39703=DIRECTION ( 'NONE',  ( -0.000000000000000000, 1.000000000000000000, -0.000000000000000000 ) ) ;
#39706=CARTESIAN_POINT ( 'NONE',  ( 163.5430354047457229, 63.84092878795252801, 94.99999999999866418 ) ) ;
#39712=CARTESIAN_POINT ( 'NONE',  ( -156.9406434201984553, 70.74968524571475825, -14.31838670552433257 ) ) ;
#39715=CARTESIAN_POINT ( 'NONE',  ( -62.30163634902125125, 17.79682011226253380, 62.67378655492601780 ) ) ;
#39717=VERTEX_POINT ( 'NONE', #24658 ) ;
#39720=CARTESIAN_POINT ( 'NONE',  ( -38.69577193929646342, 10.89562623693160326, 35.75813062815972643 ) ) ;
#39727=EDGE_LOOP ( 'NONE', ( #68161, #64170, #36644, #55034 ) ) ;
#39730=CARTESIAN_POINT ( 'NONE',  ( 141.3476419847744694, 47.33903275097040364, 90.28850992081258653 ) ) ;
#39731=CARTESIAN_POINT ( 'NONE',  ( -25.51439092786625906, 9.709553105505657200, -91.90258131718498191 ) ) ;
#39745=CARTESIAN_POINT ( 'NONE',  ( 158.3636111008086687, 59.62671916656141491, -9.279633708673955539 ) ) ;
#39747=DIRECTION ( 'NONE',  ( 0.000000000000000000, 0.000000000000000000, 1.000000000000000000 ) ) ;
#39749=CARTESIAN_POINT ( 'NONE',  ( -61.86845765289633192, 16.61548683002700599, -72.70064571127269915 ) ) ;
#39754=CARTESIAN_POINT ( 'NONE',  ( -146.7345109736526183, 61.86270848728296556, -62.18528878719732944 ) ) ;
#39757=EDGE_LOOP ( 'NONE', ( #40573, #42331, #67465, #41830 ) ) ;
#39758=CARTESIAN_POINT ( 'NONE',  ( -96.76336539645313906, 31.18045094643428428, 6.069607441441186246 ) ) ;
#39760=CARTESIAN_POINT ( 'NONE',  ( 32.15613847490629240, 8.588587416860168133, 35.46206655629798377 ) ) ;
#39761=CARTESIAN_POINT ( 'NONE',  ( -179.8926034784145713, 96.58272071140105197, -45.44813079124821797 ) ) ;
#39762=CARTESIAN_POINT ( 'NONE',  ( -132.9109786433856186, 51.29129389542017492, -12.90849194883207041 ) ) ;
#39763=CARTESIAN_POINT ( 'NONE',  ( 32.65658189266903122, 8.638786419050411780, -93.42454832150183108 ) ) ;
#39766=FACE_OUTER_BOUND ( 'NONE', #7028, .T. ) ;
#39767=CARTESIAN_POINT ( 'NONE',  ( -12.77550690612892481, 8.273784096785073316, 58.80457690568544393 ) ) ;
#39769=CARTESIAN_POINT ( 'NONE',  ( -152.5101325120253080, 68.10842280990927122, -35.42590201308884446 ) ) ;
#39771=CARTESIAN_POINT ( 'NONE',  ( -31.43908319763709969, 10.61114334766716105, 45.21645440618919309 ) ) ;
#39772=FACE_OUTER_BOUND ( 'NONE', #62147, .T. ) ;
#39773=CARTESIAN_POINT ( 'NONE',  ( -85.35521056349260505, -170.0000000000000000, 94.99999999999866418 ) ) ;
#39774=CARTESIAN_POINT ( 'NONE',  ( -49.62489392740899063, 13.29305723289024499, -74.74236697503437199 ) ) ;
#39775=CARTESIAN_POINT ( 'NONE',  ( -4.071369321747700276, 7.682719369516286534, -9.562191003685860835 ) ) ;
#39777=CARTESIAN_POINT ( 'NONE',  ( -13.45956523846225039, 8.333781915634245863, 32.65906174219168889 ) ) ;
#39778=CARTESIAN_POINT ( 'NONE',  ( -61.39252081892701796, 16.47343302442960677, 6.958049073610734325 ) ) ;
#39780=AXIS2_PLACEMENT_3D ( 'NONE', #32820, #6438, #43699 ) ;
#39784=CARTESIAN_POINT ( 'NONE',  ( 107.2672065034543039, 27.52931006625853172, -77.15546443931920351 ) ) ;
#39785=CARTESIAN_POINT ( 'NONE',  ( 46.51377856795993893, 10.46037936279324576, -13.84377530420647240 ) ) ;
#39794=LINE ( 'NONE', #19370, #11707 ) ;
#39795=CARTESIAN_POINT ( 'NONE',  ( -165.7699288023689519, 79.30174988963860017, 63.65066555552893846 ) ) ;
#39797=AXIS2_PLACEMENT_3D ( 'NONE', #59749, #53778, #59066 ) ;
#39798=ORIENTED_EDGE ( 'NONE', *, *, #51245, .T. ) ;
#39799=AXIS2_PLACEMENT_3D ( 'NONE', #15431, #48696, #14729 ) ;
#39802=CARTESIAN_POINT ( 'NONE',  ( 46.14647339926992231, 9.382387518671809090, -93.42281443246146466 ) ) ;
#39803=CARTESIAN_POINT ( 'NONE',  ( -173.1211646369891355, 88.63826465341151106, 57.66624519710472185 ) ) ;
#39805=CARTESIAN_POINT ( 'NONE',  ( -165.9154624515710168, 80.89088623112733956, -13.26577719977006531 ) ) ;
#39807=DIRECTION ( 'NONE',  ( 0.000000000000000000, 0.000000000000000000, 1.000000000000000000 ) ) ;
#39809=CARTESIAN_POINT ( 'NONE',  ( 107.0447263249841541, 28.53200276018956671, -36.63432886298605240 ) ) ;
#39810=CARTESIAN_POINT ( 'NONE',  ( 20.74561700410410836, 7.717362891868937425, -37.36968443880168422 ) ) ;
#39811=CARTESIAN_POINT ( 'NONE',  ( -83.14462298835724141, 24.07775853418029044, -21.80647150814679947 ) ) ;
#39812=DIRECTION ( 'NONE',  ( -0.000000000000000000, 1.000000000000000000, -0.000000000000000000 ) ) ;
#39814=FACE_BOUND ( 'NONE', #64227, .T. ) ;
#39818=CARTESIAN_POINT ( 'NONE',  ( 32.29578462738147238, 8.602609172809795979, -67.55334439686617998 ) ) ;
#39819=CARTESIAN_POINT ( 'NONE',  ( -179.8926034784146282, 96.58272071140106618, 8.240970389679118213 ) ) ;
#39820=CARTESIAN_POINT ( 'NONE',  ( 212.1976655298228707, 119.0878071902807562, 63.37440967419005489 ) ) ;
#39828=CARTESIAN_POINT ( 'NONE',  ( -84.23431294393864732, 24.52078568147204862, -74.50897725631355684 ) ) ;
#39829=CARTESIAN_POINT ( 'NONE',  ( -62.30163634902124414, 17.79682011226252669, -17.85986521646501757 ) ) ;
#39833=CARTESIAN_POINT ( 'NONE',  ( 8.288451200428832877, 6.376395059685425082, -42.52704783185547655 ) ) ;
#39835=CARTESIAN_POINT ( 'NONE',  ( 109.3047140914111424, 29.55674059952507093, 17.72275918544008277 ) ) ;
#39838=EDGE_CURVE ( 'NONE', #15039, #42011, #22495, .T. ) ;
#39842=CARTESIAN_POINT ( 'NONE',  ( -52.68206656346372796, 15.09776187114412949, 18.09236373069973780 ) ) ;
#39846=CARTESIAN_POINT ( 'NONE',  ( 79.93911349260510235, 17.24571896967717777, 87.49448148412906789 ) ) ;
#39847=CARTESIAN_POINT ( 'NONE',  ( -167.0144425875893432, 82.02896103816512152, -91.51796402915401529 ) ) ;
#39851=CARTESIAN_POINT ( 'NONE',  ( 44.86216938219160966, 9.182565662897500758, 5.421885990403858990 ) ) ;
#39852=CARTESIAN_POINT ( 'NONE',  ( -178.4080989094417475, 94.78067157791448949, 86.68361982195993676 ) ) ;
#39854=CARTESIAN_POINT ( 'NONE',  ( 102.7435092758397843, 25.56449004647816992, -16.30709162799740142 ) ) ;
#39855=CARTESIAN_POINT ( 'NONE',  ( 197.5334904971815888, 97.00846725096930356, 12.10439990847099345 ) ) ;
#39857=CARTESIAN_POINT ( 'NONE',  ( 199.0264175060451066, 100.5059091267551707, 85.47604204415401341 ) ) ;
#39859=CARTESIAN_POINT ( 'NONE',  ( -38.02163356681019479, -170.0000000000000000, 94.99999999999866418 ) ) ;
#39860=CARTESIAN_POINT ( 'NONE',  ( -77.02372450489328060, 21.70271995013165167, -76.78175660144862036 ) ) ;
#39861=CARTESIAN_POINT ( 'NONE',  ( -15.22871623201694291, 7.486724405784661585, 36.39031658515959577 ) ) ;
#39863=CARTESIAN_POINT ( 'NONE',  ( 14.81290967676422277, 7.477658233646008235, -23.62699843601409455 ) ) ;
#39866=CARTESIAN_POINT ( 'NONE',  ( -147.7925265216585444, 64.04960911618972830, 4.071655134873576110 ) ) ;
#39867=CARTESIAN_POINT ( 'NONE',  ( 186.5979919519638202, 85.84756789133379584, -65.47989607005200696 ) ) ;
#39868=CARTESIAN_POINT ( 'NONE',  ( -35.68184644965160857, 11.34911992846755524, 85.21252114010754042 ) ) ;
#39869=ADVANCED_FACE ( 'NONE', ( #22470 ), #64692, .F. ) ;
#39870=FACE_OUTER_BOUND ( 'NONE', #67740, .T. ) ;
#39874=ORIENTED_EDGE ( 'NONE', *, *, #50598, .F. ) ;
#39877=CARTESIAN_POINT ( 'NONE',  ( 188.2493301599116933, 87.66407108637575618, 92.74603266058126394 ) ) ;
#39880=CARTESIAN_POINT ( 'NONE',  ( 60.63507185982727066, 12.13307030573223777, -9.259813910333594578 ) ) ;
#39882=CARTESIAN_POINT ( 'NONE',  ( -55.05276343752909440, 14.68156374112638751, 30.31732777293113301 ) ) ;
#39884=CARTESIAN_POINT ( 'NONE',  ( 203.1414537950835779, 105.9225671689748367, 70.89961707943172087 ) ) ;
#39886=ORIENTED_EDGE ( 'NONE', *, *, #35993, .T. ) ;
#39890=CARTESIAN_POINT ( 'NONE',  ( -61.53550548562874667, 17.56596194025585334, -65.75729484215656839 ) ) ;
#39891=CARTESIAN_POINT ( 'NONE',  ( 197.2199569260504006, 98.22436319491369261, -70.00670125119623322 ) ) ;
#39893=CARTESIAN_POINT ( 'NONE',  ( -165.7143741370937562, 79.24519349471960084, 10.25937150958397659 ) ) ;
#39896=FACE_BOUND ( 'NONE', #40594, .T. ) ;
#39900=CARTESIAN_POINT ( 'NONE',  ( -2.355184675731021748, 6.596450510445358795, 59.32335353079142237 ) ) ;
#39908=ORIENTED_EDGE ( 'NONE', *, *, #16853, .T. ) ;
#39912=CARTESIAN_POINT ( 'NONE',  ( -7.825402957745087207, -170.0000000000000000, -16.07352014148014163 ) ) ;
#39913=CARTESIAN_POINT ( 'NONE',  ( 153.8224167330181729, 56.12711234192239829, 43.46668491457897687 ) ) ;
#39916=CARTESIAN_POINT ( 'NONE',  ( 110.7117404013331026, 30.20916032354562120, 56.45576479620101651 ) ) ;
#39917=CARTESIAN_POINT ( 'NONE',  ( -179.6470915626256897, 94.69856161161347075, 7.770636087711473294 ) ) ;
#39918=CARTESIAN_POINT ( 'NONE',  ( -0.5158933718595621887, 6.525180340836104875, 12.46832194864746413 ) ) ;
#39919=CARTESIAN_POINT ( 'NONE',  ( -81.00768240531206743, 24.30850321514431656, 30.78898729842287807 ) ) ;
#39920=CARTESIAN_POINT ( 'NONE',  ( 91.13361825170457564, 21.00701373666980842, -37.30500766501614862 ) ) ;
#39923=ORIENTED_EDGE ( 'NONE', *, *, #1597, .T. ) ;
#39927=CARTESIAN_POINT ( 'NONE',  ( -72.78270026377323632, 21.23376443558118964, 15.75090436928392990 ) ) ;
#39928=CARTESIAN_POINT ( 'NONE',  ( 46.85206196242846488, 9.495795933269471689, -44.11339331410427178 ) ) ;
#39929=CARTESIAN_POINT ( 'NONE',  ( -168.0003605155415300, 83.06333427281272463, -74.54173236266500169 ) ) ;
#39930=CARTESIAN_POINT ( 'NONE',  ( -133.3755351667540481, 51.62178393940525467, 92.43199189059410514 ) ) ;
#39931=EDGE_LOOP ( 'NONE', ( #11144, #24312 ) ) ;
#39932=CARTESIAN_POINT ( 'NONE',  ( 79.14129363775931836, 17.00055658855363205, -43.81460635687067651 ) ) ;
#39937=CARTESIAN_POINT ( 'NONE',  ( 79.39764314491567632, 18.13166883367086868, 35.20801747820795669 ) ) ;
#39939=ADVANCED_FACE ( 'NONE', ( #5590 ), #11916, .F. ) ;
#39943=CARTESIAN_POINT ( 'NONE',  ( 141.2470358420065963, 46.06959063280893218, -15.37362590030078202 ) ) ;
#39945=CARTESIAN_POINT ( 'NONE',  ( -175.9864315813574080, 91.91454246454361510, -22.31134190825564190 ) ) ;
#39947=CARTESIAN_POINT ( 'NONE',  ( -47.94536219817737788, 13.92422159065987763, 35.37158188387844149 ) ) ;
#39951=CARTESIAN_POINT ( 'NONE',  ( 107.0477776024378471, 27.43148174916615645, 57.16618254239813268 ) ) ;
#39952=CARTESIAN_POINT ( 'NONE',  ( 162.0835148203877054, 61.32844276806160622, 57.82138791843907910 ) ) ;
#39955=CARTESIAN_POINT ( 'NONE',  ( 185.1647878987786555, 82.82967084668432278, -50.03327312915156000 ) ) ;
#39956=CARTESIAN_POINT ( 'NONE',  ( -106.6940984894957865, 35.07986071359381697, 58.78132469885891709 ) ) ;
#39957=CARTESIAN_POINT ( 'NONE',  ( -26.49516976694650694, 8.831756547364872034, -37.15611514740469090 ) ) ;
#39961=EDGE_LOOP ( 'NONE', ( #21409, #16363, #1319, #26688 ) ) ;
#39962=DIRECTION ( 'NONE',  ( 0.000000000000000000, 0.000000000000000000, 1.000000000000000000 ) ) ;
#39963=DIRECTION ( 'NONE',  ( 0.000000000000000000, 0.000000000000000000, 1.000000000000000000 ) ) ;
#39964=DIRECTION ( 'NONE',  ( -0.000000000000000000, 1.000000000000000000, -0.000000000000000000 ) ) ;
#39965=CARTESIAN_POINT ( 'NONE',  ( 127.4669243510812890, 38.85312661085428232, 40.96951064535277709 ) ) ;
#39967=CARTESIAN_POINT ( 'NONE',  ( -62.30163634902122993, 17.79682011226253380, 35.82923596446230619 ) ) ;
#39969=ADVANCED_FACE ( 'NONE', ( #54104 ), #1022, .F. ) ;
#39971=CARTESIAN_POINT ( 'NONE',  ( 37.47081272996200596, 8.166145978397523209, 71.50965036819673060 ) ) ;
#39976=CARTESIAN_POINT ( 'NONE',  ( -189.5325095384513645, 107.4952257375067433, -39.98148027700779750 ) ) ;
#39980=CARTESIAN_POINT ( 'NONE',  ( 200.8410151090926661, 101.2014854111317419, 69.99904410503900465 ) ) ;
#39981=CARTESIAN_POINT ( 'NONE',  ( 131.3924949472282719, 41.12442122814100998, -23.76614924233935611 ) ) ;
#39983=ORIENTED_EDGE ( 'NONE', *, *, #18316, .F. ) ;
#39985=CARTESIAN_POINT ( 'NONE',  ( 129.4887940973039235, 40.01039828304090662, -37.40761579681454663 ) ) ;
#39986=CARTESIAN_POINT ( 'NONE',  ( -128.7810612886106583, 48.42424427998342651, 4.349626167892300721 ) ) ;
#39989=CARTESIAN_POINT ( 'NONE',  ( -190.6985136298601731, 109.1272424661242582, -46.56223028809779407 ) ) ;
#39990=EDGE_LOOP ( 'NONE', ( #52110, #39180 ) ) ;
#39991=CARTESIAN_POINT ( 'NONE',  ( -122.3745688183166180, 44.21964839958062043, -35.77374999016983281 ) ) ;
#39997=CARTESIAN_POINT ( 'NONE',  ( 163.6822386031149961, 63.95725419756645636, 86.38138517414357409 ) ) ;
#40001=CARTESIAN_POINT ( 'NONE',  ( -153.1031717208032035, 68.63449618039560107, 31.63498310044917616 ) ) ;
#40003=CARTESIAN_POINT ( 'NONE',  ( 84.05098130332766004, 18.55728792516086401, 17.41457137852304982 ) ) ;
#40004=CARTESIAN_POINT ( 'NONE',  ( -58.10608953386396536, 15.52134062643865242, 4.118145803309525732 ) ) ;
#40006=CARTESIAN_POINT ( 'NONE',  ( 55.61382797299287972, 11.07686102552914953, 36.07810415337662846 ) ) ;
#40007=ORIENTED_EDGE ( 'NONE', *, *, #11514, .T. ) ;
#40008=ORIENTED_EDGE ( 'NONE', *, *, #42505, .T. ) ;
#40009=CARTESIAN_POINT ( 'NONE',  ( 175.8874477961784351, 74.89984466412603581, 42.23741952950327061 ) ) ;
#40011=CARTESIAN_POINT ( 'NONE',  ( -31.86813133847536506, 10.68216487685447724, -89.01555078892404538 ) ) ;
#40014=FACE_OUTER_BOUND ( 'NONE', #36507, .T. ) ;
#40016=CARTESIAN_POINT ( 'NONE',  ( -24.60892750534350171, 9.584951112520229799, 34.60842798550392274 ) ) ;
#40020=CARTESIAN_POINT ( 'NONE',  ( 205.5130322755755969, 109.1888880665735684, -63.17048162308527992 ) ) ;
#40024=CARTESIAN_POINT ( 'NONE',  ( 136.9654665832768217, 44.52067472585215313, 43.83972285872444274 ) ) ;
#40026=CARTESIAN_POINT ( 'NONE',  ( -129.3970594949619795, 50.06339481638098476, 4.627477422553299746 ) ) ;
#40028=CARTESIAN_POINT ( 'NONE',  ( 22.72762739171800561, 7.830015800126070680, 67.23574744945879900 ) ) ;
#40033=DIRECTION ( 'NONE',  ( -0.000000000000000000, 1.000000000000000000, -0.000000000000000000 ) ) ;
#40037=CARTESIAN_POINT ( 'NONE',  ( -96.88650755818751747, 30.12426815936638391, 86.48723326776581644 ) ) ;
#40041=CARTESIAN_POINT ( 'NONE',  ( -77.02112161466368434, 22.77583432622785864, -8.449775604031531273 ) ) ;
#40043=CARTESIAN_POINT ( 'NONE',  ( -107.7677210873465867, 36.80113675102408877, 32.88384746470102016 ) ) ;
#40045=CARTESIAN_POINT ( 'NONE',  ( 31.90184941268615759, 7.552181687745346927, 37.17179062719809224 ) ) ;
#40051=EDGE_CURVE ( 'NONE', #63684, #51410, #19885, .T. ) ;
#40054=CARTESIAN_POINT ( 'NONE',  ( -47.55235941796723154, 12.79790236059687558, 11.21044603464288869 ) ) ;
#40055=CARTESIAN_POINT ( 'NONE',  ( 152.2940756559017927, 53.73566983921581652, -49.05695220847099591 ) ) ;
#40059=CARTESIAN_POINT ( 'NONE',  ( -151.2497169612548760, 65.66843968092747730, -8.119136368407126270 ) ) ;
#40064=ADVANCED_FACE ( 'NONE', ( #26294 ), #69527, .F. ) ;
#40067=CARTESIAN_POINT ( 'NONE',  ( 153.8224167330181729, 56.12711234192239829, -63.91151744727573458 ) ) ;
#40068=CARTESIAN_POINT ( 'NONE',  ( -37.07602570886409410, 10.58457435034603300, 32.74454515178810965 ) ) ;
#40069=CARTESIAN_POINT ( 'NONE',  ( 140.8984307802396643, 45.84194788389000763, -46.15581894915797534 ) ) ;
#40072=LINE ( 'NONE', #64451, #49766 ) ;
#40073=CARTESIAN_POINT ( 'NONE',  ( -119.2982054035570911, 42.30181775808006250, 34.54033407936248068 ) ) ;
#40075=CARTESIAN_POINT ( 'NONE',  ( 32.30062460741315533, 8.603096374765343057, -18.70062496153113685 ) ) ;
#40076=CARTESIAN_POINT ( 'NONE',  ( 183.1865184929770862, 80.75677158533827082, 2.761582280813896340 ) ) ;
#40077=CARTESIAN_POINT ( 'NONE',  ( 89.87518614971251907, 20.55373388674512469, 57.27852128848381597 ) ) ;
#40079=DIRECTION ( 'NONE',  ( -0.000000000000000000, 0.000000000000000000, -1.000000000000000000 ) ) ;
#40080=( NAMED_UNIT ( * ) PLANE_ANGLE_UNIT ( ) SI_UNIT ( $, .RADIAN. ) );
#40082=B_SPLINE_CURVE_WITH_KNOTS ( 'NONE', 3,
 ( #60707, #66012, #59644, #60365, #28348, #27995, #577, #43816, #23083, #27296, #49792, #11458, #22028, #12523, #50156, #49440, #38918, #48736, #22727, #43470, #64950, #17441, #55424, #33296, #16745, #44164, #11820, #23442, #38203, #1619, #27647, #44881, #65290, #18152, #6892, #1984, #39263, #12181, #17809, #33644, #44532, #32927, #49088, #7250, #66362 ),
 .UNSPECIFIED., .F., .F.,
 ( 4, 2, 2, 2, 2, 2, 2, 2, 2, 2, 2, 2, 2, 1, 2, 2, 2, 2, 2, 2, 2, 2, 4 ),
 ( 0.02352719711393055912, 0.02499986300757017083, 0.02573619595438998708, 0.02647252890120980334, 0.02794519479484943586, 0.02941786068848907185, 0.03015419363530889157, 0.03089052658212870783, 0.03236319247576834035, 0.03309952542258814273, 0.03383585836940794511, 0.03530852426304757763, 0.03604485720986738695, 0.03678119015668719627, 0.03751752310350699865, 0.03825385605032680103, 0.03972652194396641273, 0.04119918783760602443, 0.04267185373124562919, 0.04340818667806543851, 0.04414451962488524783, 0.04561718551852484566, 0.04708985141216444348 ),
 .UNSPECIFIED. ) ;
#40084=EDGE_LOOP ( 'NONE', ( #63627, #31085, #53722, #31103 ) ) ;
#40085=CARTESIAN_POINT ( 'NONE',  ( 162.7921669283191193, 61.91024532638674316, -22.07005389488237057 ) ) ;
#40087=VECTOR ( 'NONE', #58304, 1000.000000000000000 ) ;
#40088=CARTESIAN_POINT ( 'NONE',  ( 68.95451040317567504, 14.12887482153123386, 68.76426114867949480 ) ) ;
#40089=CARTESIAN_POINT ( 'NONE',  ( 141.2801018238827169, 47.29457739955284978, 11.26812789576816876 ) ) ;
#40093=AXIS2_PLACEMENT_3D ( 'NONE', #17005, #6472, #140 ) ;
#40096=CARTESIAN_POINT ( 'NONE',  ( 10.13846145460683701, 6.385368868491634764, 42.47142630253362228 ) ) ;
#40099=CARTESIAN_POINT ( 'NONE',  ( 63.49941241090381538, 13.81848793187418600, 56.65751152968498161 ) ) ;
#40101=CARTESIAN_POINT ( 'NONE',  ( 130.2154003102709225, 39.26869728108905377, -90.64406281561510070 ) ) ;
#40103=CARTESIAN_POINT ( 'NONE',  ( 162.8034185388970627, 63.22443559329413176, -48.91927988040787056 ) ) ;
#40108=CARTESIAN_POINT ( 'NONE',  ( -99.98584758882478241, 32.75338129098886952, 4.018470313552430895 ) ) ;
#40109=CARTESIAN_POINT ( 'NONE',  ( 66.50978889550178508, 14.54692747110987483, 84.35750253269495147 ) ) ;
#40110=CARTESIAN_POINT ( 'NONE',  ( 151.2878525843655666, 54.24529526600250051, -93.06221793583787871 ) ) ;
#40111=CARTESIAN_POINT ( 'NONE',  ( 86.62931800182292363, 20.48449268398422163, -8.977013608448025650 ) ) ;
#40112=CARTESIAN_POINT ( 'NONE',  ( -165.7689197919845014, 79.30072199592278537, 39.83247271659003985 ) ) ;
#40113=CARTESIAN_POINT ( 'NONE',  ( 33.57125916965274115, 8.734028988681728833, -92.01757106967839661 ) ) ;
#40115=CYLINDRICAL_SURFACE ( 'NONE', #51847, 7.500000000000020428 ) ;
#40120=ORIENTED_EDGE ( 'NONE', *, *, #43245, .T. ) ;
#40121=CYLINDRICAL_SURFACE ( 'NONE', #11500, 7.500000000000013323 ) ;
#40122=CARTESIAN_POINT ( 'NONE',  ( 210.9608386442062624, 117.1762372255315654, -12.84724971893104062 ) ) ;
#40126=CARTESIAN_POINT ( 'NONE',  ( -9.914178172705819136, 7.035763242673981566, -89.39128270836016554 ) ) ;
#40130=CARTESIAN_POINT ( 'NONE',  ( -56.02027488966933788, 14.94257193099085868, 18.42563833103987392 ) ) ;
#40133=CARTESIAN_POINT ( 'NONE',  ( -100.4347360276019145, 32.97716872911834685, -49.79891040578767303 ) ) ;
#40137=AXIS2_PLACEMENT_3D ( 'NONE', #46191, #40925, #29678 ) ;
#40141=CARTESIAN_POINT ( 'NONE',  ( -15.32732096506169661, 7.496199110535271437, 91.58149418733879088 ) ) ;
#40151=B_SPLINE_CURVE_WITH_KNOTS ( 'NONE', 3,
 ( #68147, #51613, #9393, #56896, #36468, #18912, #9740, #46319, #30852, #19594, #19955, #31203, #52298, #25234, #62154, #3423, #3764, #47022, #35083, #41057, #40696, #20285, #52635, #14662, #24198, #45984, #36124, #46672, #19242, #45641, #40358, #61806, #4117, #56535, #13974, #35436, #63205, #8363, #8712, #68478, #29811, #41744, #51273, #62517, #14329, #57235, #9050, #59289 ),
 .UNSPECIFIED., .F., .F.,
 ( 4, 2, 2, 2, 2, 2, 2, 2, 2, 2, 2, 2, 2, 2, 2, 2, 2, 2, 2, 2, 2, 2, 2, 4 ),
 ( 0.02554216173022670275, 0.02715505844859215229, 0.02796150680777490655, 0.02876795516695766428, 0.03038085188532323178, 0.03199374860368880275, 0.03360664532205437371, 0.03441309368123716267, 0.03521954204041995162, 0.03602599039960274058, 0.03683243875878554341, 0.03844533547715116295, 0.03925178383633396578, 0.04005823219551677555, 0.04086468055469958532, 0.04167112891388238816, 0.04247757727306519793, 0.04328402563224800770, 0.04489692235061367581, 0.04650981906897934393, 0.04731626742816219533, 0.04812271578734504673, 0.04973561250571066628, 0.05134850922407628582 ),
 .UNSPECIFIED. ) ;
#40152=CARTESIAN_POINT ( 'NONE',  ( 106.6181401479172308, 28.34160787025144046, 70.52598296703905589 ) ) ;
#40155=CARTESIAN_POINT ( 'NONE',  ( 58.46823952472684027, 12.69204591816732730, -10.39183658609108996 ) ) ;
#40157=CARTESIAN_POINT ( 'NONE',  ( 109.3047140914111850, 29.55674059952507093, -35.96634199548729072 ) ) ;
#40158=CARTESIAN_POINT ( 'NONE',  ( -31.43908319763710679, 10.61114334766716283, -8.472646774738153752 ) ) ;
#40161=FACE_BOUND ( 'NONE', #33463, .T. ) ;
#40165=CARTESIAN_POINT ( 'NONE',  ( 34.83823433017388993, 8.871835168107978120, -75.93650321438980200 ) ) ;
#40166=CARTESIAN_POINT ( 'NONE',  ( -180.5801285865471186, 97.42945596116098272, 10.67803447139740491 ) ) ;
#40167=CARTESIAN_POINT ( 'NONE',  ( 211.5034924207027700, 118.0100795718634856, 66.71809058681080273 ) ) ;
#40168=CARTESIAN_POINT ( 'NONE',  ( 86.15410276028859471, 19.25894675708890347, -77.66611478937541335 ) ) ;
#40172=DIRECTION ( 'NONE',  ( 0.000000000000000000, 0.000000000000000000, 1.000000000000000000 ) ) ;
#40173=CARTESIAN_POINT ( 'NONE',  ( 197.8598785550297521, 99.02620879292953759, -46.92193452575618551 ) ) ;
#40177=DIRECTION ( 'NONE',  ( -0.000000000000000000, 1.000000000000000000, -0.000000000000000000 ) ) ;
#40178=ORIENTED_EDGE ( 'NONE', *, *, #7256, .F. ) ;
#40179=CARTESIAN_POINT ( 'NONE',  ( -83.12901536265223967, 24.07178615860086168, -63.42720624446700128 ) ) ;
#40180=CARTESIAN_POINT ( 'NONE',  ( -62.41727141396690826, 17.83188754031768752, -14.38874286553851611 ) ) ;
#40181=ADVANCED_FACE ( 'NONE', ( #48754 ), #59660, .F. ) ;
#40182=B_SPLINE_CURVE_WITH_KNOTS ( 'NONE', 3,
 ( #65092, #17602, #6349, #39065, #60510, #59795, #34140, #23242, #43267, #33446, #54162, #27802, #11975, #49240, #6697, #17955, #12326, #38006, #33785, #11266, #48883, #1075, #66163, #16551, #22525, #28143, #729, #55224, #17239, #60853, #50311, #64747, #55577, #5986, #1779, #7042, #49588, #43967, #65446, #28505, #7406, #28861, #22179, #59453, #13036, #35519 ),
 .UNSPECIFIED., .F., .F.,
 ( 4, 2, 2, 2, 2, 2, 2, 2, 2, 2, 2, 2, 2, 2, 2, 2, 2, 2, 2, 2, 2, 2, 4 ),
 ( 0.02404638330965502141, 0.02555608299537558831, 0.02631093283823587523, 0.02706578268109615867, 0.02857548236681672904, 0.02933033220967700902, 0.03008518205253728900, 0.03159488173825784896, 0.03310458142397840892, 0.03385943126683869236, 0.03461428110969896887, 0.03612398079541952189, 0.03687883063827980534, 0.03763368048114007491, 0.03838853032400035142, 0.03914338016686062793, 0.04065307985258118095, 0.04216277953830172703, 0.04367247922402228699, 0.04518217890974284001, 0.04593702875260310958, 0.04669187859546338609, 0.04820157828118393911 ),
 .UNSPECIFIED. ) ;
#40183=CARTESIAN_POINT ( 'NONE',  ( 92.53033045403536505, 22.59263332688196257, -74.82145947628868043 ) ) ;
#40184=ORIENTED_EDGE ( 'NONE', *, *, #413, .T. ) ;
#40187=EDGE_LOOP ( 'NONE', ( #30168, #46137, #10530, #64349 ) ) ;
#40189=CARTESIAN_POINT ( 'NONE',  ( -109.4874964445488104, 37.74487348321786584, -94.07812955749422201 ) ) ;
#40192=ORIENTED_EDGE ( 'NONE', *, *, #17513, .T. ) ;
#40195=CARTESIAN_POINT ( 'NONE',  ( -48.71337292867760027, 14.10768470390589435, 14.98814739561979437 ) ) ;
#40196=CARTESIAN_POINT ( 'NONE',  ( -132.2286325684322037, 52.04087929935079870, -11.54593800350672872 ) ) ;
#40199=CARTESIAN_POINT ( 'NONE',  ( 79.13041963748372609, 18.04952109592810672, -43.84177388801760600 ) ) ;
#40200=CARTESIAN_POINT ( 'NONE',  ( -173.1211646369891355, -170.0000000000000000, 65.16624519710472896 ) ) ;
#40201=ORIENTED_EDGE ( 'NONE', *, *, #33376, .T. ) ;
#40206=CARTESIAN_POINT ( 'NONE',  ( 117.4396227366912626, 33.48307633470226818, -95.00000000000133582 ) ) ;
#40208=CARTESIAN_POINT ( 'NONE',  ( 197.2200752504830632, 96.62072041958359137, 10.52740617786156463 ) ) ;
#40210=CARTESIAN_POINT ( 'NONE',  ( 212.0690325386321433, 118.8871691880494836, 88.99556113406791269 ) ) ;
#40212=CARTESIAN_POINT ( 'NONE',  ( -82.93126516400698733, 25.07709093823495650, 58.58861024883177038 ) ) ;
#40216=ORIENTED_EDGE ( 'NONE', *, *, #27399, .T. ) ;
#40218=LINE ( 'NONE', #13485, #46656 ) ;
#40220=CARTESIAN_POINT ( 'NONE',  ( -31.13302211571334155, 10.56067280572192146, 83.90492538947324874 ) ) ;
#40221=CARTESIAN_POINT ( 'NONE',  ( -101.3492134984965389, 32.31003911421601771, -35.05777063899205359 ) ) ;
#40225=CARTESIAN_POINT ( 'NONE',  ( 8.763528846667099970, 7.383598436776582119, -40.38010197442696381 ) ) ;
#40226=CARTESIAN_POINT ( 'NONE',  ( 126.5710838895481629, 37.19597237024176906, -45.32323354818519334 ) ) ;
#40230=CARTESIAN_POINT ( 'NONE',  ( 188.3911424972466193, 87.82183351239343949, 88.76307796285202301 ) ) ;
#40233=CARTESIAN_POINT ( 'NONE',  ( -24.33435124463267130, 8.532637995283112176, -67.24644030340769518 ) ) ;
#40236=CARTESIAN_POINT ( 'NONE',  ( 11.21387192505586405, 6.397095920409661574, 4.706635521921354481 ) ) ;
#40239=CARTESIAN_POINT ( 'NONE',  ( 41.34269507549201705, 9.685203600174695282, -77.22535371806525006 ) ) ;
#40240=CARTESIAN_POINT ( 'NONE',  ( -60.95805269991218722, 17.39401718769329719, -74.19099977899746534 ) ) ;
#40241=CARTESIAN_POINT ( 'NONE',  ( 197.3064269725219049, 98.33232022113060111, -69.35658200132850482 ) ) ;
#40243=ADVANCED_FACE ( 'NONE', ( #54028 ), #28011, .T. ) ;
#40245=CARTESIAN_POINT ( 'NONE',  ( -173.1211646369891071, 87.12891641440859303, 3.977144016177345254 ) ) ;
#40247=CARTESIAN_POINT ( 'NONE',  ( -55.05276343752909440, 14.68156374112638929, 57.16187836339483397 ) ) ;
#40249=CARTESIAN_POINT ( 'NONE',  ( -0.5183605925911988210, 6.525266619725955231, 62.75222543575570455 ) ) ;
#40252=CARTESIAN_POINT ( 'NONE',  ( 150.0516754638056227, 53.34587188591231666, 62.61862363090603623 ) ) ;
#40262=CARTESIAN_POINT ( 'NONE',  ( 152.8672128926848757, 55.41186463791521533, 30.98344588502664365 ) ) ;
#40266=CARTESIAN_POINT ( 'NONE',  ( -178.0658882571759989, 92.80593104957416983, 5.833208099788561363 ) ) ;
#40267=DIRECTION ( 'NONE',  ( 0.000000000000000000, 0.000000000000000000, 1.000000000000000000 ) ) ;
#40268=EDGE_CURVE ( 'NONE', #52035, #9829, #11510, .T. ) ;
#40269=CARTESIAN_POINT ( 'NONE',  ( 55.77012379229939398, 12.13428856597101202, -41.26774091221908236 ) ) ;
#40270=CARTESIAN_POINT ( 'NONE',  ( -85.10909119100207931, 25.97025675005452428, 34.04615563038053949 ) ) ;
#40271=CARTESIAN_POINT ( 'NONE',  ( -27.70185240367226953, 10.02491413133431308, -22.47982293096844941 ) ) ;
#40272=CARTESIAN_POINT ( 'NONE',  ( 134.3159642998340360, 41.70198410084977780, 2.665790248531664908 ) ) ;
#40275=B_SPLINE_CURVE_WITH_KNOTS ( 'NONE', 3,
 ( #67322, #62724, #9253, #7873, #34953, #19814, #57097, #66978, #29323, #61333, #18771, #52160, #51479, #68348, #35987, #40916, #24052, #3290, #51128, #24405, #8914, #45491, #61675, #40226, #29667, #57442, #13494, #56397, #67656, #24748, #30711, #19453, #8219, #3623, #8572, #30019, #3978, #2943, #45846, #19108, #62374, #25449, #40562, #62014, #13155, #56057 ),
 .UNSPECIFIED., .F., .F.,
 ( 4, 2, 2, 2, 2, 2, 2, 2, 2, 2, 2, 2, 2, 2, 2, 2, 2, 2, 2, 2, 2, 2, 4 ),
 ( 3.179800655392250756E-17, 0.001572224531395693828, 0.003144449062791355564, 0.004716673594187017517, 0.006288898125582679903, 0.007861122656978341422, 0.009433347188374002074, 0.01021945945407182026, 0.01100557171976963497, 0.01179168398546745315, 0.01257779625116526960, 0.01415002078256088341, 0.01493613304825867037, 0.01572224531395645733, 0.01650835757965424949, 0.01729446984535203818, 0.01886669437674766067, 0.01965280664244547365, 0.02043891890814329010, 0.02201114343953891606, 0.02358336797093454548, 0.02436948023663238969, 0.02515559250233023042 ),
 .UNSPECIFIED. ) ;
#40279=ADVANCED_FACE ( 'NONE', ( #34703 ), #18513, .F. ) ;
#40280=CARTESIAN_POINT ( 'NONE',  ( 46.50704915687941821, 9.440294391580033917, -40.70557485162431988 ) ) ;
#40283=CARTESIAN_POINT ( 'NONE',  ( 204.6977192012829789, -170.0000000000000000, -97.51503221354896311 ) ) ;
#40284=VERTEX_POINT ( 'NONE', #3033 ) ;
#40285=CARTESIAN_POINT ( 'NONE',  ( 79.38459371357853911, 17.07499996355401706, -41.31674572369035303 ) ) ;
#40288=CARTESIAN_POINT ( 'NONE',  ( -142.0685766576042113, 58.11789490499571542, 66.17456823166700985 ) ) ;
#40291=CARTESIAN_POINT ( 'NONE',  ( 187.9007786055418023, 85.78077355327275200, -13.74105984729973251 ) ) ;
#40292=CARTESIAN_POINT ( 'NONE',  ( 140.8984307802396927, 45.84194788389002184, -19.31126835869425662 ) ) ;
#40293=CARTESIAN_POINT ( 'NONE',  ( -84.21836162213168109, 25.60181819557223548, -20.83666508763759140 ) ) ;
#40294=CARTESIAN_POINT ( 'NONE',  ( -177.5100621450480389, 93.70693725195823731, -21.46705021681216863 ) ) ;
#40295=CARTESIAN_POINT ( 'NONE',  ( -49.43836229152577033, 14.28302414152159727, 32.81988602651634324 ) ) ;
#40296=ORIENTED_EDGE ( 'NONE', *, *, #18646, .T. ) ;
#40298=CARTESIAN_POINT ( 'NONE',  ( 103.1567541746301373, 25.73937982110321343, 61.44734176770268874 ) ) ;
#40303=CARTESIAN_POINT ( 'NONE',  ( -24.70354720400822757, 8.582324684301863016, -39.48142304760889942 ) ) ;
#40309=CARTESIAN_POINT ( 'NONE',  ( -71.35455658117328426, 19.66980550601473254, 89.90639409444233365 ) ) ;
#40310=CARTESIAN_POINT ( 'NONE',  ( -82.32750425780473336, 23.74963782027935721, 71.32606545563898237 ) ) ;
#40311=CARTESIAN_POINT ( 'NONE',  ( 63.98009977735164000, 12.89803120691695959, -50.67432517864035901 ) ) ;
#40312=DIRECTION ( 'NONE',  ( -0.000000000000000000, 1.000000000000000000, -0.000000000000000000 ) ) ;
#40313=CARTESIAN_POINT ( 'NONE',  ( -61.52761555060400411, 17.56359742150279146, 34.00003020467226378 ) ) ;
#40315=CARTESIAN_POINT ( 'NONE',  ( 55.91494169499918598, 12.16343363043255899, 39.74022306742683952 ) ) ;
#40317=ADVANCED_FACE ( 'NONE', ( #60720 ), #30113, .F. ) ;
#40318=ORIENTED_EDGE ( 'NONE', *, *, #51620, .T. ) ;
#40319=CARTESIAN_POINT ( 'NONE',  ( -7.336760511143403107, 6.859209474528211281, -50.41807073194384969 ) ) ;
#40321=CARTESIAN_POINT ( 'NONE',  ( -190.3074740493607067, 108.5764897054613414, -45.99346789251534773 ) ) ;
#40322=FACE_OUTER_BOUND ( 'NONE', #49663, .T. ) ;
#40324=CARTESIAN_POINT ( 'NONE',  ( -109.3553681454883844, 36.52260784104394986, -71.89925778247966548 ) ) ;
#40325=CARTESIAN_POINT ( 'NONE',  ( 132.9453095272139649, 42.04754713161464963, -9.178760341931969435 ) ) ;
#40326=ADVANCED_FACE ( 'NONE', ( #50171 ), #55800, .F. ) ;
#40329=CARTESIAN_POINT ( 'NONE',  ( 126.4633682455862100, 38.28837286275646790, -42.23541007965406635 ) ) ;
#40330=CARTESIAN_POINT ( 'NONE',  ( -38.54712373114178092, 11.89174538567467643, -45.26023169000558255 ) ) ;
#40333=CARTESIAN_POINT ( 'NONE',  ( -170.7765859439901419, 84.55522338090253243, 84.86709083567915002 ) ) ;
#40335=CARTESIAN_POINT ( 'NONE',  ( 132.2818448028687897, 41.65267246304668447, 2.829438630737001859 ) ) ;
#40339=ADVANCED_FACE ( 'NONE', ( #7624 ), #33999, .F. ) ;
#40341=CARTESIAN_POINT ( 'NONE',  ( 164.6219598329275868, 64.74833093291276498, 88.30847154703400292 ) ) ;
#40345=CARTESIAN_POINT ( 'NONE',  ( 126.8015497489690091, 37.32461426945042859, 34.45213346083535555 ) ) ;
#40351=ORIENTED_EDGE ( 'NONE', *, *, #58265, .T. ) ;
#40352=CARTESIAN_POINT ( 'NONE',  ( -6.972379992530896686, 7.843576898687570242, -89.10717191287119476 ) ) ;
#40355=CARTESIAN_POINT ( 'NONE',  ( -166.9992034932275544, 82.01285191063136892, 15.83985853835711488 ) ) ;
#40357=CARTESIAN_POINT ( 'NONE',  ( 20.74852474914887068, 6.709938988646750424, -64.21677084482480780 ) ) ;
#40358=CARTESIAN_POINT ( 'NONE',  ( -132.8257891167039588, 52.46553896898736724, 67.83950217250055914 ) ) ;
#40360=CARTESIAN_POINT ( 'NONE',  ( -94.77353847196663139, 30.23867427826260013, 91.81396056268231121 ) ) ;
#40364=CARTESIAN_POINT ( 'NONE',  ( -71.23176719684943237, 20.69188312694500453, -41.59565793431328729 ) ) ;
#40368=B_SPLINE_CURVE_WITH_KNOTS ( 'NONE', 3,
 ( #63577, #3454, #15391, #10108, #30533, #35817, #24915, #46349, #14360, #57269, #51982, #3799, #30884, #25267, #52328, #58977, #10791, #15731, #49103, #48071, #37181, #942 ),
 .UNSPECIFIED., .F., .F.,
 ( 4, 2, 2, 2, 2, 2, 2, 2, 2, 2, 4 ),
 ( 0.01079565252593830092, 0.01215565516365934261, 0.01351565780138038603, 0.01487566043910142771, 0.01555566175796195202, 0.01623566307682247287, 0.01759566571454351802, 0.01827566703340402846, 0.01895566835226453889, 0.02031567098998559445, 0.02167567362770664655 ),
 .UNSPECIFIED. ) ;
#40369=DIRECTION ( 'NONE',  ( 0.000000000000000000, 0.000000000000000000, 1.000000000000000000 ) ) ;
#40370=CARTESIAN_POINT ( 'NONE',  ( 113.8626313173125766, 31.71036178495293001, 43.69715942616913651 ) ) ;
#40371=DIRECTION ( 'NONE',  ( 0.000000000000000000, 0.000000000000000000, 1.000000000000000000 ) ) ;
#40376=CARTESIAN_POINT ( 'NONE',  ( -142.8492950481059154, 60.01492924994602873, -18.93097386172547303 ) ) ;
#40379=CYLINDRICAL_SURFACE ( 'NONE', #59133, 7.500000000000020428 ) ;
#40381=CARTESIAN_POINT ( 'NONE',  ( -142.5211356634642073, 58.47296527616907014, 35.47922671525356009 ) ) ;
#40382=CARTESIAN_POINT ( 'NONE',  ( -132.9409505933031426, 51.31241517713429801, 62.34483324402277304 ) ) ;
#40383=CARTESIAN_POINT ( 'NONE',  ( -171.4814970982679654, 85.32124710276286805, -61.72613384226752942 ) ) ;
#40385=CARTESIAN_POINT ( 'NONE',  ( -107.0809603157386647, 36.42942792191063717, 43.80174314235760846 ) ) ;
#40387=CARTESIAN_POINT ( 'NONE',  ( 36.09137906183516264, 8.001963043161765654, 30.67956151840819246 ) ) ;
#40393=CARTESIAN_POINT ( 'NONE',  ( -8.320534640989466268, 7.931748412542452442, -35.41807073194379996 ) ) ;
#40395=CARTESIAN_POINT ( 'NONE',  ( 153.2282895792479280, 54.42637815496157572, -49.81384560666342054 ) ) ;
#40396=EDGE_LOOP ( 'NONE', ( #64094, #24258 ) ) ;
#40398=ORIENTED_EDGE ( 'NONE', *, *, #65765, .T. ) ;
#40400=CARTESIAN_POINT ( 'NONE',  ( -58.97243502469714826, 16.81420332340175605, 71.06078827025896771 ) ) ;
#40404=CARTESIAN_POINT ( 'NONE',  ( -8.807541152391513251, 6.956521193351525412, -62.31119320194252964 ) ) ;
#40405=CARTESIAN_POINT ( 'NONE',  ( -95.63568360745013308, 29.53168204475775482, -19.15801658276413377 ) ) ;
#40406=CARTESIAN_POINT ( 'NONE',  ( 136.1310312718401860, 42.81430973242786564, -36.36153061589796920 ) ) ;
#40411=CARTESIAN_POINT ( 'NONE',  ( -152.2873556200144378, 67.91256772393730046, 58.09607398853111704 ) ) ;
#40412=CARTESIAN_POINT ( 'NONE',  ( -118.9468627709229054, 42.08677365399181269, 40.95864189269519784 ) ) ;
#40413=CARTESIAN_POINT ( 'NONE',  ( -61.75956139478098805, 16.58288496614411756, -46.08246547442131202 ) ) ;
#40415=CARTESIAN_POINT ( 'NONE',  ( -177.5100621450479537, 93.70693725195826573, -75.15615139773954922 ) ) ;
#40416=CARTESIAN_POINT ( 'NONE',  ( 129.7308524360012427, 40.15101741188608742, 84.42769425744016587 ) ) ;
#40420=DIRECTION ( 'NONE',  ( -0.000000000000000000, 1.000000000000000000, -0.000000000000000000 ) ) ;
#40424=EDGE_CURVE ( 'NONE', #33190, #44118, #37565, .T. ) ;
#40425=ORIENTED_EDGE ( 'NONE', *, *, #17860, .F. ) ;
#40426=CARTESIAN_POINT ( 'NONE',  ( 162.8142581494936394, 61.92799983924231810, -11.49565247231627119 ) ) ;
#40427=CARTESIAN_POINT ( 'NONE',  ( 115.7561705820729117, 31.51689401996055651, -75.37479631241809841 ) ) ;
#40429=CARTESIAN_POINT ( 'NONE',  ( 138.5943620234099001, 45.55242290395132443, 4.331259207765530306 ) ) ;
#40434=LINE ( 'NONE', #3162, #32819 ) ;
#40437=CARTESIAN_POINT ( 'NONE',  ( 141.3651931500070305, 46.14690144103921199, 90.63982096354233420 ) ) ;
#40438=B_SPLINE_CURVE_WITH_KNOTS ( 'NONE', 3,
 ( #44212, #55119, #28391, #17128, #23127, #17849, #60044, #6596, #65696, #38963, #55471, #50549, #7651, #60407, #44577, #66405, #28754, #28043, #66055, #50202, #23483, #18195, #61106, #12928, #34388, #55832, #63183, #62841, #36446, #8690, #19930, #61785, #3065, #29437, #20264, #2711, #67098, #30144, #8340, #51594, #62493, #4099, #46648, #24173, #9031, #18887, #35063, #25216 ),
 .UNSPECIFIED., .F., .F.,
 ( 4, 2, 2, 2, 2, 2, 2, 2, 2, 2, 2, 2, 2, 2, 2, 2, 2, 2, 2, 2, 2, 2, 2, 4 ),
 ( 0.02746511744866863072, 0.02914922134997089548, 0.03083332525127316023, 0.03251742915257541111, 0.03335948110322656951, 0.03420153305387772097, 0.03504358500452887937, 0.03588563695518003083, 0.03756974085648229905, 0.03841179280713343663, 0.03925384475778457422, 0.04009589670843571874, 0.04093794865908685632, 0.04262205256038914536, 0.04430615646169143440, 0.04514820841234259974, 0.04599026036299375814, 0.04767436426429607493, 0.04935846816559839867, 0.05020052011624956401, 0.05104257206690072934, 0.05272667596820305308, 0.05356872791885422536, 0.05441077986950540457 ),
 .UNSPECIFIED. ) ;
#40440=CARTESIAN_POINT ( 'NONE',  ( -147.7845268487069177, 62.73119438705056439, -61.84506813724533458 ) ) ;
#40442=DIRECTION ( 'NONE',  ( 0.000000000000000000, 0.000000000000000000, 1.000000000000000000 ) ) ;
#40445=CARTESIAN_POINT ( 'NONE',  ( 163.2886151008987667, 62.32020850087170771, -48.36354064594853952 ) ) ;
#40449=CARTESIAN_POINT ( 'NONE',  ( 70.43355351840769174, 15.55757160495454983, 89.84466342665578509 ) ) ;
#40450=CARTESIAN_POINT ( 'NONE',  ( 153.6141452268275884, 55.97027600123225000, -90.86889088305335349 ) ) ;
#40451=CARTESIAN_POINT ( 'NONE',  ( 84.74089592029042706, 19.84571403269345424, -23.73936403045067678 ) ) ;
#40453=CARTESIAN_POINT ( 'NONE',  ( 38.57561400113527839, 9.317436507016033431, -89.34323513843901310 ) ) ;
#40454=CARTESIAN_POINT ( 'NONE',  ( 126.4083787442700242, 37.10531539900951969, -71.39317657368648895 ) ) ;
#40456=CARTESIAN_POINT ( 'NONE',  ( -97.48179118242298102, 31.52606332398822531, 59.07822971242244137 ) ) ;
#40457=CARTESIAN_POINT ( 'NONE',  ( -15.32495246574475267, 8.506829480038508251, 63.95817259830450752 ) ) ;
#40460=CARTESIAN_POINT ( 'NONE',  ( -157.0069571479806996, 72.18154199622277645, -42.61338853642176616 ) ) ;
#40461=CARTESIAN_POINT ( 'NONE',  ( 210.0122310839192323, 115.7355030290288198, -11.66628312975793413 ) ) ;
#40462=CARTESIAN_POINT ( 'NONE',  ( -37.07436112751819479, 11.60822760208521842, 42.68967068761850214 ) ) ;
#40463=CARTESIAN_POINT ( 'NONE',  ( -155.2912910578197057, 69.24479901948498650, -64.37611446947235549 ) ) ;
#40464=CARTESIAN_POINT ( 'NONE',  ( 57.23318867907233454, 11.40538244752438857, 86.21413257773676264 ) ) ;
#40465=CARTESIAN_POINT ( 'NONE',  ( -47.95193882091085413, 12.89180642785319364, -72.02524729475207721 ) ) ;
#40466=CARTESIAN_POINT ( 'NONE',  ( -3.255961059272217462, 7.643453059677442596, -10.10607710301138518 ) ) ;
#40467=CARTESIAN_POINT ( 'NONE',  ( 174.2469308602414912, 71.96142024047681218, 6.869062816487226719 ) ) ;
#40468=CARTESIAN_POINT ( 'NONE',  ( -61.38706483483512244, 16.47181058798475917, 14.99613853738705771 ) ) ;
#40470=CARTESIAN_POINT ( 'NONE',  ( -97.48179118242302366, 31.52606332398818267, -48.29997264943230562 ) ) ;
#40471=ORIENTED_EDGE ( 'NONE', *, *, #24858, .F. ) ;
#40472=CARTESIAN_POINT ( 'NONE',  ( 108.3819860115547300, 28.02992728837240577, -77.54759093648532087 ) ) ;
#40474=CARTESIAN_POINT ( 'NONE',  ( 41.80536115778105710, 8.734184316430663841, 57.14969185523772666 ) ) ;
#40476=CARTESIAN_POINT ( 'NONE',  ( -3.023885888100138697, 6.625757189166515460, 85.53385992682667904 ) ) ;
#40478=CARTESIAN_POINT ( 'NONE',  ( -106.4728934171453858, 36.10295170132724962, -21.89315576262807639 ) ) ;
#40480=CARTESIAN_POINT ( 'NONE',  ( -165.6398193834831716, 79.16932278174803628, 64.55551728305448478 ) ) ;
#40481=ORIENTED_EDGE ( 'NONE', *, *, #25098, .T. ) ;
#40482=VERTEX_POINT ( 'NONE', #22310 ) ;
#40483=EDGE_CURVE ( 'NONE', #9471, #61817, #49256, .T. ) ;
#40487=CARTESIAN_POINT ( 'NONE',  ( 104.4006536356073980, 27.36759527624477073, 59.22638815182622807 ) ) ;
#40491=CARTESIAN_POINT ( 'NONE',  ( 55.56634333706183781, 12.09342294753930069, -17.37762842755674342 ) ) ;
#40492=ORIENTED_EDGE ( 'NONE', *, *, #10875, .F. ) ;
#40494=CARTESIAN_POINT ( 'NONE',  ( 15.78827728214693416, 7.507518794609576496, -35.51894409868578606 ) ) ;
#40495=CARTESIAN_POINT ( 'NONE',  ( 8.679939806240504652, 7.383357464882123189, 66.76383109117342940 ) ) ;
#40497=CARTESIAN_POINT ( 'NONE',  ( 12.92334181113699465, 6.425676190254471010, -89.76395520566100572 ) ) ;
#40499=ADVANCED_FACE ( 'NONE', ( #61679 ), #28635, .F. ) ;
#40504=CARTESIAN_POINT ( 'NONE',  ( 39.40195752203892710, 8.409560354027384221, 71.75838489642698903 ) ) ;
#40506=CARTESIAN_POINT ( 'NONE',  ( 133.8566784816069344, -170.0000000000000000, 63.85489142945905172 ) ) ;
#40507=CARTESIAN_POINT ( 'NONE',  ( 8.286608610395276742, 6.376392877433615602, 90.91779146060531502 ) ) ;
#40508=VECTOR ( 'NONE', #15738, 1000.000000000000000 ) ;
#40509=CARTESIAN_POINT ( 'NONE',  ( 79.23200707685334976, 17.02828389812517784, -68.90372702717917264 ) ) ;
#40511=B_SPLINE_CURVE_WITH_KNOTS ( 'NONE', 3,
 ( #1699, #11531, #33008, #60777, #28784, #55866, #23509, #7680, #22104, #6621, #43544, #54440, #28069, #49161, #1000, #44245, #22452, #12253 ),
 .UNSPECIFIED., .F., .F.,
 ( 4, 2, 2, 2, 2, 2, 2, 2, 4 ),
 ( 0.01106689075334992868, 0.01242473758491097549, 0.01378258441647202230, 0.01514043124803306911, 0.01649827807959411766, 0.01785612491115516273, 0.01921397174271621128, 0.02057181857427725635, 0.02192966540583830490 ),
 .UNSPECIFIED. ) ;
#40514=CARTESIAN_POINT ( 'NONE',  ( 197.6341357773624452, 98.74251867088339907, -41.28717180241687146 ) ) ;
#40515=ORIENTED_EDGE ( 'NONE', *, *, #17860, .T. ) ;
#40519=CARTESIAN_POINT ( 'NONE',  ( -58.97243502469712695, 16.81420332340174895, -9.472863501132078312 ) ) ;
#40523=CARTESIAN_POINT ( 'NONE',  ( 46.85361596800671435, 10.51535167202354693, 65.24308912524901416 ) ) ;
#40524=CARTESIAN_POINT ( 'NONE',  ( -102.4897449030618333, 34.01725961887433414, -88.70367844590327877 ) ) ;
#40525=CARTESIAN_POINT ( 'NONE',  ( 103.1695711638930675, 26.83837309506526481, 7.722913913205804448 ) ) ;
#40530=CARTESIAN_POINT ( 'NONE',  ( 8.485361335568063268, 7.382900357301075189, -95.00000000000133582 ) ) ;
#40531=CARTESIAN_POINT ( 'NONE',  ( 113.8748103246145575, 30.59837980920002565, -9.998117947202244338 ) ) ;
#40532=CARTESIAN_POINT ( 'NONE',  ( 82.73618382051374454, 19.18661415186669217, -36.90649579248486845 ) ) ;
#40534=ORIENTED_EDGE ( 'NONE', *, *, #27524, .F. ) ;
#40537=CARTESIAN_POINT ( 'NONE',  ( 181.0840389613909736, 80.03940679743416808, 2.464043515047717570 ) ) ;
#40538=VECTOR ( 'NONE', #40420, 1000.000000000000000 ) ;
#40542=CARTESIAN_POINT ( 'NONE',  ( 127.1040286383415037, 37.49395136275128237, 6.891878244443025103 ) ) ;
#40544=CARTESIAN_POINT ( 'NONE',  ( 208.5412688739946248, 113.5467507967246945, 83.95023641488762678 ) ) ;
#40548=CARTESIAN_POINT ( 'NONE',  ( -13.78293860383719327, 7.352367295275509029, 42.19825724717986759 ) ) ;
#40550=CARTESIAN_POINT ( 'NONE',  ( 9.689943677145720358, 7.388265075009365468, -20.54709311085173695 ) ) ;
#40554=CARTESIAN_POINT ( 'NONE',  ( -142.3187766126154941, 59.59460822661997526, 9.166696566367921406 ) ) ;
#40555=CARTESIAN_POINT ( 'NONE',  ( 184.9757174666827382, 84.09845285279331506, -76.98475161410866008 ) ) ;
#40556=CARTESIAN_POINT ( 'NONE',  ( -166.7050147108375029, 81.70694330787517856, 42.24510784831770138 ) ) ;
#40559=CARTESIAN_POINT ( 'NONE',  ( 31.96227686234409049, 7.558148489540042370, -44.10090099851916534 ) ) ;
#40561=CARTESIAN_POINT ( 'NONE',  ( 13.83281508467570475, 7.452090093180183672, -35.76147573379551403 ) ) ;
#40562=CARTESIAN_POINT ( 'NONE',  ( 132.9440032680862771, 40.87616997986733480, -50.97107703778330290 ) ) ;
#40567=CARTESIAN_POINT ( 'NONE',  ( -15.31363169557738679, 7.494880774892000552, 10.28358019018753389 ) ) ;
#40570=CARTESIAN_POINT ( 'NONE',  ( -25.48237668717799309, 8.689083390666786144, -65.07822405608331451 ) ) ;
#40572=CARTESIAN_POINT ( 'NONE',  ( 12.46277766093406569, 6.416700641561361884, 17.41053802626028357 ) ) ;
#40573=ORIENTED_EDGE ( 'NONE', *, *, #30519, .F. ) ;
#40575=CARTESIAN_POINT ( 'NONE',  ( -62.54086041493280135, 17.86944394914986844, -69.06975546854211245 ) ) ;
#40576=CARTESIAN_POINT ( 'NONE',  ( 199.3764470687683286, 100.9548044849099568, -65.37965796067832969 ) ) ;
#40577=CARTESIAN_POINT ( 'NONE',  ( -180.3153482337535252, 95.51031295027644319, -40.07067488068217642 ) ) ;
#40578=CARTESIAN_POINT ( 'NONE',  ( 108.3819860115547584, 28.02992728837241287, 2.986060834905694961 ) ) ;
#40581=CARTESIAN_POINT ( 'NONE',  ( -51.99406906667272921, 13.88268392809765750, 71.51408645859281421 ) ) ;
#40583=CARTESIAN_POINT ( 'NONE',  ( -98.82269223037674521, 31.05895700771357326, -89.54463258280026139 ) ) ;
#40588=CARTESIAN_POINT ( 'NONE',  ( -131.3154845336012500, 50.16828105866952825, -74.46309887825546525 ) ) ;
#40589=CARTESIAN_POINT ( 'NONE',  ( -108.5248383251030475, 37.21456094989610364, -73.52032136529315665 ) ) ;
#40590=CARTESIAN_POINT ( 'NONE',  ( -48.99162761293257518, 13.13973062091724131, -47.14059449902415366 ) ) ;
#40594=EDGE_LOOP ( 'NONE', ( #3695, #52630 ) ) ;
#40600=DIRECTION ( 'NONE',  ( 0.000000000000000000, 0.000000000000000000, 1.000000000000000000 ) ) ;
#40601=CARTESIAN_POINT ( 'NONE',  ( 150.0278556977734468, 53.32860603304213498, 37.98783775011875719 ) ) ;
#40605=CARTESIAN_POINT ( 'NONE',  ( -174.7800083645697100, 88.99302808536937448, 4.150939364941768517 ) ) ;
#40609=CARTESIAN_POINT ( 'NONE',  ( -85.96384504792885650, 26.32782846176032621, 39.66807532746997822 ) ) ;
#40610=CARTESIAN_POINT ( 'NONE',  ( 150.4558794230171657, 52.39657120201827922, 87.91895567814847823 ) ) ;
#40611=CARTESIAN_POINT ( 'NONE',  ( 139.2921620648436942, 44.80435067172502528, 4.974970203711714944 ) ) ;
#40614=CARTESIAN_POINT ( 'NONE',  ( 9.823983574062873814, 6.382904402091122975, 59.78584119632682103 ) ) ;
#40615=CARTESIAN_POINT ( 'NONE',  ( 45.34143264614440483, 9.256465810451187437, -47.70603915148674190 ) ) ;
#40618=EDGE_LOOP ( 'NONE', ( #29294, #56897, #29217, #48871 ) ) ;
#40619=CARTESIAN_POINT ( 'NONE',  ( 86.62931800182292363, 19.42108912189597092, -35.82156419891171595 ) ) ;
#40620=VERTEX_POINT ( 'NONE', #63419 ) ;
#40622=CARTESIAN_POINT ( 'NONE',  ( 79.92842440418704086, 18.29578799637231512, 33.80686922133299532 ) ) ;
#40625=DIRECTION ( 'NONE',  ( -0.000000000000000000, 1.000000000000000000, -0.000000000000000000 ) ) ;
#40626=CARTESIAN_POINT ( 'NONE',  ( -81.23268307104842734, 24.39742801172156561, -22.82221074267823724 ) ) ;
#40627=CARTESIAN_POINT ( 'NONE',  ( -180.2243452982809515, 96.99029284948635166, -12.94268875518402240 ) ) ;
#40628=CARTESIAN_POINT ( 'NONE',  ( -52.68206656346373506, 15.09776187114413659, 44.93691432116340678 ) ) ;
#40629=ORIENTED_EDGE ( 'NONE', *, *, #4846, .T. ) ;
#40633=CARTESIAN_POINT ( 'NONE',  ( 102.7571040248401175, 25.57023079238896557, 64.48323540187037395 ) ) ;
#40637=CARTESIAN_POINT ( 'NONE',  ( 188.5837490358996149, 86.53279111916958755, -44.03581940269903328 ) ) ;
#40638=CARTESIAN_POINT ( 'NONE',  ( 17.72992212664810552, 6.570588738776105053, 30.26623964099782427 ) ) ;
#40639=CARTESIAN_POINT ( 'NONE',  ( -142.1933357692790878, 59.49560539235535117, 90.21512086776893113 ) ) ;
#40642=ORIENTED_EDGE ( 'NONE', *, *, #37012, .F. ) ;
#40647=DIRECTION ( 'NONE',  ( -0.000000000000000000, 1.000000000000000000, -0.000000000000000000 ) ) ;
#40649=CARTESIAN_POINT ( 'NONE',  ( -86.15441609607631790, 25.31657638323078530, 64.26769477816569065 ) ) ;
#40650=CARTESIAN_POINT ( 'NONE',  ( 70.38121440378670002, 14.50253793787158862, -41.74354549825704908 ) ) ;
#40653=CARTESIAN_POINT ( 'NONE',  ( -62.14837099232447315, 17.75045801599141271, 40.25957659325134586 ) ) ;
#40656=CARTESIAN_POINT ( 'NONE',  ( -38.88884187334147668, 11.95889603743728102, -70.65858916182976657 ) ) ;
#40657=CARTESIAN_POINT ( 'NONE',  ( 33.44983424733139543, 7.709709042132401713, 68.84813754810760145 ) ) ;
#40658=CARTESIAN_POINT ( 'NONE',  ( 43.46000298353792601, 8.971888098965388636, 84.78699099868985911 ) ) ;
#40663=CARTESIAN_POINT ( 'NONE',  ( 66.73594759725088466, 13.56641407806658073, -63.54845448085986703 ) ) ;
#40664=CARTESIAN_POINT ( 'NONE',  ( 129.4987365823222660, 38.85470922756779544, -22.78752412490684165 ) ) ;
#40666=CARTESIAN_POINT ( 'NONE',  ( -107.7893514267588557, 35.66840175773126020, -74.47184679149792430 ) ) ;
#40670=CARTESIAN_POINT ( 'NONE',  ( 126.4757069339777189, 38.29528077539266206, -44.88019376975797314 ) ) ;
#40675=VERTEX_POINT ( 'NONE', #62730 ) ;
#40681=CARTESIAN_POINT ( 'NONE',  ( 130.3281282802763315, 40.49854652972194202, -77.00284772816436885 ) ) ;
#40683=CARTESIAN_POINT ( 'NONE',  ( -153.6946616617039183, 69.16142959008686830, 31.98171298067408586 ) ) ;
#40689=B_SPLINE_CURVE_WITH_KNOTS ( 'NONE', 3,
 ( #56985, #50657, #8096, #8803, #40451, #7761, #35531, #24637, #46412, #3510, #57327, #13045, #61568, #62250, #14420, #46071, #68235, #8451, #61217, #20043, #34844, #2477, #67542, #18659, #52048, #19339, #2823, #29210, #45733, #9140, #34505, #29545, #51014, #40795, #19687, #35872, #23932, #13383, #45382, #67212, #66861, #18999, #14065, #40111 ),
 .UNSPECIFIED., .F., .F.,
 ( 4, 2, 2, 2, 2, 2, 2, 2, 2, 2, 2, 2, 2, 2, 2, 2, 2, 2, 2, 2, 2, 4 ),
 ( 0.02416815208377490892, 0.02567033257376878305, 0.02642142281876571838, 0.02717251306376265718, 0.02867469355375653131, 0.02942578379875344929, 0.03017687404375036728, 0.03167905453374421365, 0.03318123502373805656, 0.03393232526873497801, 0.03468341551373190640, 0.03618559600372574930, 0.03693668624872267076, 0.03768777649371959221, 0.03918995698371342817, 0.04069213747370725720, 0.04219431796370109317, 0.04369649845369492913, 0.04444758869869186446, 0.04519867894368879979, 0.04670085943368265657, 0.04820303992367652723 ),
 .UNSPECIFIED. ) ;
#40690=CARTESIAN_POINT ( 'NONE',  ( -4.529991408371923711, 7.705014754505700836, -89.81607011104952676 ) ) ;
#40691=VERTEX_POINT ( 'NONE', #25454 ) ;
#40692=VECTOR ( 'NONE', #4482, 1000.000000000000000 ) ;
#40694=CARTESIAN_POINT ( 'NONE',  ( 175.0634607207818760, 74.11351956991630630, 41.28835302766208315 ) ) ;
#40695=CARTESIAN_POINT ( 'NONE',  ( 19.53470118933705635, 6.649487981843462236, -76.36537058919049059 ) ) ;
#40696=CARTESIAN_POINT ( 'NONE',  ( -133.1566699306513044, 52.70203339370771545, 63.07426314407797463 ) ) ;
#40698=CARTESIAN_POINT ( 'NONE',  ( -94.87248710667839191, 30.28499078005656742, 90.48868467975900387 ) ) ;
#40704=CARTESIAN_POINT ( 'NONE',  ( 208.5936709733498446, 113.6229123546138311, -77.09327358427836430 ) ) ;
#40707=CARTESIAN_POINT ( 'NONE',  ( 112.5612011511790058, 31.08353758940340938, 29.96277884949118331 ) ) ;
#40708=CARTESIAN_POINT ( 'NONE',  ( -128.1267916618075446, 49.19573276651589566, 18.45006178907944161 ) ) ;
#40711=ORIENTED_EDGE ( 'NONE', *, *, #2462, .F. ) ;
#40712=B_SPLINE_CURVE_WITH_KNOTS ( 'NONE', 3,
 ( #25414, #10240, #14152, #3594, #51785, #4623, #36988, #3946, #57069, #52126, #47185, #46494, #8882, #25064, #68642, #42266, #31706, #63727, #30333, #15189, #63025, #62695, #67977, #47518, #53138, #14495, #41571, #26438, #20806, #15536, #63379, #19775, #14832, #58426, #26087, #36301, #46849, #68978, #41234, #9571, #68317, #20120, #31030, #35952 ),
 .UNSPECIFIED., .F., .F.,
 ( 4, 2, 2, 2, 2, 2, 2, 2, 2, 2, 2, 2, 2, 2, 2, 2, 2, 2, 2, 2, 2, 4 ),
 ( 0.000000000000000000, 0.001533942663855634905, 0.003067885327711269809, 0.004601827991566905147, 0.005368799323494720215, 0.006135770655422535282, 0.007669713319278181896, 0.008436684651206005636, 0.009203655983133829377, 0.01073759864698946125, 0.01150456997891726590, 0.01227154131084507056, 0.01303851264277287522, 0.01380548397470067988, 0.01533942663855628746, 0.01687336930241190025, 0.01840731196626750957, 0.01994125463012312235, 0.02070822596205092528, 0.02147519729397872820, 0.02300913995783436181, 0.02454308262168999541 ),
 .UNSPECIFIED. ) ;
#40713=CARTESIAN_POINT ( 'NONE',  ( -142.8556048422594529, 60.01994222009838609, -11.99344991105233937 ) ) ;
#40714=CARTESIAN_POINT ( 'NONE',  ( -124.9970785861867739, 47.10847819093958577, -49.86331799269337495 ) ) ;
#40716=CARTESIAN_POINT ( 'NONE',  ( -52.95121991886625068, 14.12782764494541432, -89.19314900505109733 ) ) ;
#40719=CARTESIAN_POINT ( 'NONE',  ( 70.51583798635768119, 15.57951509147423508, -43.46259958853134719 ) ) ;
#40721=CARTESIAN_POINT ( 'NONE',  ( -142.0747101610765242, -170.0000000000000000, -95.00000000000133582 ) ) ;
#40722=CARTESIAN_POINT ( 'NONE',  ( -165.9992860119574516, 79.53569239468048124, -71.42556836936645936 ) ) ;
#40725=CARTESIAN_POINT ( 'NONE',  ( -109.6657532478350419, 37.84376708859253569, 36.68825689172810200 ) ) ;
#40728=CARTESIAN_POINT ( 'NONE',  ( -31.93184248720559637, 9.672312402099827011, 18.37190381572552056 ) ) ;
#40733=CYLINDRICAL_SURFACE ( 'NONE', #65859, 7.500000000000013323 ) ;
#40736=CARTESIAN_POINT ( 'NONE',  ( -55.05276343752910151, -170.0000000000000000, 64.66187836339484818 ) ) ;
#40741=AXIS2_PLACEMENT_3D ( 'NONE', #52652, #25252, #14677 ) ;
#40744=CARTESIAN_POINT ( 'NONE',  ( -59.57733000654212674, 15.94108165424592727, 31.81619162008844626 ) ) ;
#40745=CARTESIAN_POINT ( 'NONE',  ( -61.10880364359508121, 17.43879918625642134, 60.23065452846851997 ) ) ;
#40749=CARTESIAN_POINT ( 'NONE',  ( -15.32520546926283522, 7.495995523981878073, -69.26974520926577839 ) ) ;
#40750=CARTESIAN_POINT ( 'NONE',  ( -37.92511097250854846, 10.74631978746601213, 41.49036279183128073 ) ) ;
#40752=CARTESIAN_POINT ( 'NONE',  ( -27.48703802937315288, 8.975952825337621732, 70.94001361132677630 ) ) ;
#40757=DIRECTION ( 'NONE',  ( 0.000000000000000000, 0.000000000000000000, 1.000000000000000000 ) ) ;
#40759=EDGE_CURVE ( 'NONE', #61817, #8726, #2094, .T. ) ;
#40760=EDGE_CURVE ( 'NONE', #35601, #5954, #17559, .T. ) ;
#40761=CARTESIAN_POINT ( 'NONE',  ( -118.8689810167776244, 42.03922634358561794, 35.47965570148047476 ) ) ;
#40762=CARTESIAN_POINT ( 'NONE',  ( -56.72814287166056602, 15.13700122306437201, -35.40189249770946134 ) ) ;
#40764=CARTESIAN_POINT ( 'NONE',  ( -179.8989115484066303, 96.59045402602906449, -65.83356435992200772 ) ) ;
#40765=CARTESIAN_POINT ( 'NONE',  ( 91.67571176799444288, 21.20498955963028820, 58.50299178729044769 ) ) ;
#40766=CARTESIAN_POINT ( 'NONE',  ( 111.8699272271189074, 29.64190505307781009, 29.78602444577448338 ) ) ;
#40767=CARTESIAN_POINT ( 'NONE',  ( 133.8566784816069344, -170.0000000000000000, 44.51034083899536142 ) ) ;
#40768=CARTESIAN_POINT ( 'NONE',  ( -118.6849742182705540, 41.92701402439730884, -67.17183305668943660 ) ) ;
#40769=EDGE_LOOP ( 'NONE', ( #41211, #35958 ) ) ;
#40770=CARTESIAN_POINT ( 'NONE',  ( 198.8687991397275709, 98.67887821384412916, 31.98142328829086622 ) ) ;
#40771=CARTESIAN_POINT ( 'NONE',  ( 115.7746371641014775, 31.52600568297706829, -65.17888831513212722 ) ) ;
#40773=CARTESIAN_POINT ( 'NONE',  ( 141.2361973397653117, 47.26569015399787332, 11.53046231077025752 ) ) ;
#40776=CARTESIAN_POINT ( 'NONE',  ( 164.8433205901839074, 64.93586312665797777, -15.37696764588941178 ) ) ;
#40777=VERTEX_POINT ( 'NONE', #28820 ) ;
#40778=CARTESIAN_POINT ( 'NONE',  ( -173.1211646369891355, 88.63826465341152527, -7.867406574286299303 ) ) ;
#40784=CARTESIAN_POINT ( 'NONE',  ( 164.1338586910085553, 64.33646242148854810, -40.17183423574092416 ) ) ;
#40786=CARTESIAN_POINT ( 'NONE',  ( 162.6190874793280159, 61.76782592053310594, -49.08288557175567490 ) ) ;
#40790=CARTESIAN_POINT ( 'NONE',  ( -97.49665543375860466, 31.53324358035374075, 16.97217977605912154 ) ) ;
#40792=CARTESIAN_POINT ( 'NONE',  ( -127.6861178856153458, 47.68458428355325651, 45.41653894850171724 ) ) ;
#40794=CARTESIAN_POINT ( 'NONE',  ( 156.7505278390357262, 58.36400587947789376, -89.81328548006503354 ) ) ;
#40795=CARTESIAN_POINT ( 'NONE',  ( 81.74250361646204510, 18.86685472882136239, -10.76652222608316301 ) ) ;
#40798=CARTESIAN_POINT ( 'NONE',  ( 150.0973882686024865, 52.13852366454154463, 65.15538058431675950 ) ) ;
#40799=CARTESIAN_POINT ( 'NONE',  ( 90.91356992076215704, 21.99794663086830937, 43.37270543508057585 ) ) ;
#40802=CARTESIAN_POINT ( 'NONE',  ( -12.40598104375064281, 8.242193636955557068, 70.41920131499857405 ) ) ;
#40803=ORIENTED_EDGE ( 'NONE', *, *, #55726, .F. ) ;
#40807=CARTESIAN_POINT ( 'NONE',  ( 103.4725384926517080, 26.96797537091730135, 33.87479904705897837 ) ) ;
#40809=CARTESIAN_POINT ( 'NONE',  ( 63.36339561252631114, 12.75346589351348392, 83.50301528697106335 ) ) ;
#40812=CARTESIAN_POINT ( 'NONE',  ( -1.095583923122881442, 7.553030873957006897, -12.75389933006059806 ) ) ;
#40813=CARTESIAN_POINT ( 'NONE',  ( 173.6012773665503914, 71.36035397668605640, 9.375753324076253392 ) ) ;
#40814=CARTESIAN_POINT ( 'NONE',  ( -59.36813706141742131, 15.88103696331963732, 17.11169410266594682 ) ) ;
#40816=VERTEX_POINT ( 'NONE', #50269 ) ;
#40817=CARTESIAN_POINT ( 'NONE',  ( 133.8566784816069344, 42.60093787723652525, 29.51034083899533300 ) ) ;
#40819=CARTESIAN_POINT ( 'NONE',  ( 104.7147873368645037, 26.40702926859710686, -65.17463016867208125 ) ) ;
#40822=CARTESIAN_POINT ( 'NONE',  ( 43.14712943604300932, 8.926114770663669873, 70.76097164223719460 ) ) ;
#40823=CARTESIAN_POINT ( 'NONE',  ( -32.29068479830811356, 9.732388393132145765, -89.04274443136878858 ) ) ;
#40825=DIRECTION ( 'NONE',  ( 0.000000000000000000, -1.000000000000000000, 0.000000000000000000 ) ) ;
#40826=CARTESIAN_POINT ( 'NONE',  ( -108.9444157621018405, 37.44493815491210853, -12.19092097621495974 ) ) ;
#40828=DIRECTION ( 'NONE',  ( 0.000000000000000000, -1.000000000000000000, 0.000000000000000000 ) ) ;
#40829=CARTESIAN_POINT ( 'NONE',  ( -165.9986675144415926, 79.53506019208352029, 67.53357148677014266 ) ) ;
#40831=VERTEX_POINT ( 'NONE', #60472 ) ;
#40832=CARTESIAN_POINT ( 'NONE',  ( -156.4841188516943191, 70.33041971808555104, 35.45435599281108807 ) ) ;
#40835=CARTESIAN_POINT ( 'NONE',  ( 107.0447263249840830, 28.53200276018955961, 70.74387349886869458 ) ) ;
#40838=CARTESIAN_POINT ( 'NONE',  ( 59.30258796551119360, 12.87111270082601600, -22.91115838005825722 ) ) ;
#40839=ORIENTED_EDGE ( 'NONE', *, *, #1755, .T. ) ;
#40844=CARTESIAN_POINT ( 'NONE',  ( 19.75315861330097533, 7.667327050329333815, -49.38992306506955998 ) ) ;
#40845=CARTESIAN_POINT ( 'NONE',  ( -144.9412191745148561, 61.69548892475973645, 44.19022063994489713 ) ) ;
#40847=FACE_BOUND ( 'NONE', #15962, .T. ) ;
#40850=VECTOR ( 'NONE', #42240, 1000.000000000000000 ) ;
#40855=CARTESIAN_POINT ( 'NONE',  ( -133.3902399421379812, 52.86946745625289168, 91.39822547968469735 ) ) ;
#40857=CARTESIAN_POINT ( 'NONE',  ( 36.99999522780156980, 9.122638774496635961, -77.07355369017872704 ) ) ;
#40859=CARTESIAN_POINT ( 'NONE',  ( 13.21458769038542336, 6.431875961233155081, 84.15148632264042305 ) ) ;
#40860=CARTESIAN_POINT ( 'NONE',  ( 22.60595478824430415, 7.822665100698110940, 88.06109399808075011 ) ) ;
#40865=CARTESIAN_POINT ( 'NONE',  ( -83.12901536265223967, 24.07178615860086879, 17.10644552692404119 ) ) ;
#40866=ORIENTED_EDGE ( 'NONE', *, *, #50598, .T. ) ;
#40873=CARTESIAN_POINT ( 'NONE',  ( 102.7446498997619955, 26.65764321315727159, 9.730055971096106759 ) ) ;
#40875=CARTESIAN_POINT ( 'NONE',  ( -30.81072340916226793, 9.488257828543728678, 83.90441008401572276 ) ) ;
#40876=EDGE_CURVE ( 'NONE', #40902, #44954, #69326, .T. ) ;
#40877=CARTESIAN_POINT ( 'NONE',  ( 174.2538192999569731, 73.34752463892029084, -73.67968158064373085 ) ) ;
#40881=CARTESIAN_POINT ( 'NONE',  ( 82.94816950786172072, 19.25538918181908343, -36.78261693489493211 ) ) ;
#40884=AXIS2_PLACEMENT_3D ( 'NONE', #6565, #33658, #43830 ) ;
#40887=CARTESIAN_POINT ( 'NONE',  ( 44.34263167748004264, 9.103379693481585377, 4.905521142611629415 ) ) ;
#40888=CARTESIAN_POINT ( 'NONE',  ( -180.6072146854561993, 97.46297145775103843, 91.41803955879689170 ) ) ;
#40891=CARTESIAN_POINT ( 'NONE',  ( 128.4224537826253822, 38.23837035195744249, 15.35765953459713451 ) ) ;
#40893=CARTESIAN_POINT ( 'NONE',  ( 38.98661671391530348, 8.355545674958261060, -89.30891864635513855 ) ) ;
#40895=CARTESIAN_POINT ( 'NONE',  ( 203.6529352990553150, 106.6193458023785183, 82.96504318203567152 ) ) ;
#40896=CARTESIAN_POINT ( 'NONE',  ( 208.5884523568772693, 113.6152425727545534, 43.13355516528025646 ) ) ;
#40897=CARTESIAN_POINT ( 'NONE',  ( -78.66644367742109978, 22.32174330031320508, -61.96000122218157458 ) ) ;
#40898=CARTESIAN_POINT ( 'NONE',  ( -104.1342612728951593, 33.73231160250194449, 30.73689793636901157 ) ) ;
#40901=LINE ( 'NONE', #45482, #36291 ) ;
#40902=VERTEX_POINT ( 'NONE', #18608 ) ;
#40904=CARTESIAN_POINT ( 'NONE',  ( -149.5074843970971017, 65.50121172469319220, -76.65738112195568021 ) ) ;
#40908=CARTESIAN_POINT ( 'NONE',  ( 187.8965227056806953, 87.27289477191497724, -67.42077669584755029 ) ) ;
#40910=DIRECTION ( 'NONE',  ( -0.8160245890732938934, -0.5780171883497599028, 0.000000000000000000 ) ) ;
#40911=CARTESIAN_POINT ( 'NONE',  ( 206.2980740120524388, 108.5619562183279925, -78.00887972345341836 ) ) ;
#40912=B_SPLINE_CURVE_WITH_KNOTS ( 'NONE', 3,
 ( #14393, #18967, #36529, #3827, #14721, #30221, #30913, #51333, #40415, #57984, #56954, #20342, #67506, #13687, #9452, #35844, #19303, #30560, #51673, #35143, #15071, #57296, #25298, #41117, #9801, #52012, #46380, #19654, #56595, #8417, #40764, #62215, #3149, #25644, #46732, #24606, #20011, #52361, #35493, #4175, #67859, #14032, #41467, #62921 ),
 .UNSPECIFIED., .F., .F.,
 ( 4, 2, 2, 2, 2, 2, 2, 2, 2, 2, 2, 2, 2, 2, 2, 2, 2, 2, 2, 2, 2, 4 ),
 ( 0.02908143158676657763, 0.03095422299093864363, 0.03282701439511070962, 0.03469980579928277215, 0.03657259720345483467, 0.03844538860762689719, 0.04031818001179896666, 0.04125457571388498057, 0.04219097141597099448, 0.04312736711805700840, 0.04359556496910003964, 0.04406376282014306395, 0.04500015852222907786, 0.04593655422431509872, 0.04687294992640111263, 0.04780934562848712654, 0.04968213703265918907, 0.05155492843683125159, 0.05342771984100331412, 0.05530051124517537664, 0.05717330264934743222, 0.05904609405351949475 ),
 .UNSPECIFIED. ) ;
#40913=CARTESIAN_POINT ( 'NONE',  ( 32.15641333221389431, 7.577415570152252755, -41.16723562843993989 ) ) ;
#40916=CARTESIAN_POINT ( 'NONE',  ( 126.6576865394846152, 37.24426596493990615, -41.40349033908344012 ) ) ;
#40917=ORIENTED_EDGE ( 'NONE', *, *, #29845, .T. ) ;
#40920=CARTESIAN_POINT ( 'NONE',  ( -24.18258876560172155, 8.512344710720679331, -71.62007224143587791 ) ) ;
#40923=CARTESIAN_POINT ( 'NONE',  ( 9.057575839850581900, 6.378493414438676012, 13.98797822051807849 ) ) ;
#40924=B_SPLINE_CURVE_WITH_KNOTS ( 'NONE', 3,
 ( #37156, #58603, #53671, #48374, #16397, #59300, #5831, #27287, #569, #59636, #1610, #2319, #55780, #29734, #23075, #45563, #61049, #40292, #60701, #12516, #39599, #7600, #23434, #67046, #49784, #39943, #66695, #18836, #34684, #55065, #44525, #33636, #61397, #12876, #28340, #6883, #44873, #7242, #18488, #66001, #33977, #17433, #13221 ),
 .UNSPECIFIED., .F., .F.,
 ( 4, 2, 2, 2, 2, 2, 2, 2, 2, 2, 2, 1, 2, 2, 2, 2, 2, 2, 2, 2, 2, 4 ),
 ( 0.02515559250233026858, 0.02674001423437959851, 0.02753222510040426521, 0.02832443596642893191, 0.02990885769847832429, 0.03149327943052772361, 0.03307770116257711251, 0.03386991202860181044, 0.03466212289462650142, 0.03624654462667584870, 0.03703875549270052581, 0.03783096635872520985, 0.03862317722474989390, 0.03941538809077457101, 0.04099980982282393216, 0.04258423155487330025, 0.04337644242089798430, 0.04416865328692266141, 0.04575307501897196705, 0.04733749675102127963, 0.04892191848307057833, 0.05050634021511988397 ),
 .UNSPECIFIED. ) ;
#40925=DIRECTION ( 'NONE',  ( 0.000000000000000000, 0.000000000000000000, 1.000000000000000000 ) ) ;
#40927=CARTESIAN_POINT ( 'NONE',  ( 133.8566784816069344, 41.42467568809808398, 71.35489142945907304 ) ) ;
#40928=CARTESIAN_POINT ( 'NONE',  ( -180.0179082103088035, 95.14811732286295864, -39.25080714274592708 ) ) ;
#40929=CARTESIAN_POINT ( 'NONE',  ( 94.11746922806585758, 22.11341285603784002, -15.98499990942385907 ) ) ;
#40930=CARTESIAN_POINT ( 'NONE',  ( -171.4814970982680222, 85.32124710276291069, 18.80751792912352727 ) ) ;
#40933=CARTESIAN_POINT ( 'NONE',  ( -51.78153763344963778, 13.82841714689605439, 57.89563959941560967 ) ) ;
#40934=CARTESIAN_POINT ( 'NONE',  ( -1.857619870843137733, 6.575690665396234813, 69.02910518084183877 ) ) ;
#40937=CARTESIAN_POINT ( 'NONE',  ( -190.6985136298601731, 109.1272424661242582, 33.97142148329322708 ) ) ;
#40939=CARTESIAN_POINT ( 'NONE',  ( 153.4509883044095773, 55.84811350575043321, 57.41771316415564286 ) ) ;
#40940=CARTESIAN_POINT ( 'NONE',  ( -104.1393288135077597, 34.86912007524089319, -62.07806153423428697 ) ) ;
#40941=CARTESIAN_POINT ( 'NONE',  ( -54.09522495088364735, 14.42642983673692925, -50.17067796789629597 ) ) ;
#40943=FACE_OUTER_BOUND ( 'NONE', #62529, .T. ) ;
#40950=VERTEX_POINT ( 'NONE', #62903 ) ;
#40957=CARTESIAN_POINT ( 'NONE',  ( -55.05276343752909440, 14.68156374112637863, -62.06087458892354647 ) ) ;
#40960=CARTESIAN_POINT ( 'NONE',  ( -81.24432217070641116, 24.40203426192925207, 44.96528098049749644 ) ) ;
#40961=CARTESIAN_POINT ( 'NONE',  ( -27.49195330402089255, 9.993776132065303131, -22.35462794406847920 ) ) ;
#40962=CARTESIAN_POINT ( 'NONE',  ( 140.5781926063689298, 45.63383190293699698, 6.828449788819809463 ) ) ;
#40963=EDGE_CURVE ( 'NONE', #36565, #51770, #9792, .T. ) ;
#40970=CARTESIAN_POINT ( 'NONE',  ( -79.92415359841270117, 23.88316156050048988, 84.18770871290736579 ) ) ;
#40975=ORIENTED_EDGE ( 'NONE', *, *, #64567, .F. ) ;
#40980=CARTESIAN_POINT ( 'NONE',  ( -121.5677746760273692, 43.71038933438990881, 71.10937227840975083 ) ) ;
#40982=CARTESIAN_POINT ( 'NONE',  ( -180.6209674222602644, 97.47999311542515954, -15.53406542695830161 ) ) ;
#40984=CARTESIAN_POINT ( 'NONE',  ( -51.77779688167512973, 14.86590802019196822, 31.06571622856426274 ) ) ;
#40985=ORIENTED_EDGE ( 'NONE', *, *, #52303, .T. ) ;
#40992=CARTESIAN_POINT ( 'NONE',  ( 103.5588133492864813, 25.91050225236391213, 60.51647513232768461 ) ) ;
#40993=CARTESIAN_POINT ( 'NONE',  ( 164.8942204024298235, 63.66138186734711724, 64.85643587009047906 ) ) ;
#40998=CARTESIAN_POINT ( 'NONE',  ( 16.27765348919936983, 6.516472002017811072, 30.01470767270521733 ) ) ;
#40999=AXIS2_PLACEMENT_3D ( 'NONE', #14370, #30891, #67839 ) ;
#41001=ORIENTED_EDGE ( 'NONE', *, *, #47179, .T. ) ;
#41004=VERTEX_POINT ( 'NONE', #6576 ) ;
#41006=CARTESIAN_POINT ( 'NONE',  ( -154.0716379918897303, 69.49957566103795159, -21.43849890716462170 ) ) ;
#41007=CARTESIAN_POINT ( 'NONE',  ( 176.4195038744034605, 74.01628939311422073, -91.52755031942164976 ) ) ;
#41008=CARTESIAN_POINT ( 'NONE',  ( 63.50528314073025626, 12.78634332146812547, -35.72069083216974406 ) ) ;
#41010=DIRECTION ( 'NONE',  ( -0.8118923937861950435, -0.5838071093367415143, 0.000000000000000000 ) ) ;
#41011=CARTESIAN_POINT ( 'NONE',  ( -38.68632430131781774, 11.91908191268692008, -67.71530391917285385 ) ) ;
#41012=CARTESIAN_POINT ( 'NONE',  ( 32.67604596315972287, 7.629767358313825021, 60.93075647368799252 ) ) ;
#41013=CARTESIAN_POINT ( 'NONE',  ( 46.51849888769739039, 9.442121512056541377, 93.49346967249300633 ) ) ;
#41015=CARTESIAN_POINT ( 'NONE',  ( -0.7174461528505763352, 6.532311451815526304, -40.51236224071276126 ) ) ;
#41017=CARTESIAN_POINT ( 'NONE',  ( -120.4586945679390766, 43.01762219615313398, 16.46653791979410641 ) ) ;
#41020=CARTESIAN_POINT ( 'NONE',  ( 16.28382582968307446, 7.523443033994206885, -8.674393508222102867 ) ) ;
#41021=CARTESIAN_POINT ( 'NONE',  ( 11.21312910819263031, 7.403355431337016235, 4.706771331900731603 ) ) ;
#41024=CARTESIAN_POINT ( 'NONE',  ( 131.3924949472283004, 41.12442122814099577, -50.61069983280304285 ) ) ;
#41026=CYLINDRICAL_SURFACE ( 'NONE', #20003, 7.500000000000013323 ) ;
#41028=CARTESIAN_POINT ( 'NONE',  ( 187.8965227056806953, 87.27289477191493461, -40.57622610538386709 ) ) ;
#41030=VERTEX_POINT ( 'NONE', #59672 ) ;
#41032=CARTESIAN_POINT ( 'NONE',  ( 197.9868529032975744, 99.18611233336801547, 6.502487484275444096 ) ) ;
#41033=EDGE_LOOP ( 'NONE', ( #18772, #50069, #55433, #54774 ) ) ;
#41034=VECTOR ( 'NONE', #46514, 1000.000000000000000 ) ;
#41035=CARTESIAN_POINT ( 'NONE',  ( 153.7637790416463872, 56.08283792975861815, 84.07092255572784723 ) ) ;
#41037=CARTESIAN_POINT ( 'NONE',  ( -56.02289203441038268, 15.98631679403369965, 18.42565426861631650 ) ) ;
#41038=CARTESIAN_POINT ( 'NONE',  ( 126.4324872316703363, 37.11876756822025669, 38.10631402826915348 ) ) ;
#41040=CARTESIAN_POINT ( 'NONE',  ( -154.0833774771448361, 69.51012195447349029, 44.18219951439326820 ) ) ;
#41041=CARTESIAN_POINT ( 'NONE',  ( -98.69283175933883001, 30.99524616306737812, 31.41528330781012102 ) ) ;
#41046=DIRECTION ( 'NONE',  ( -0.000000000000000000, 1.000000000000000000, -0.000000000000000000 ) ) ;
#41048=CARTESIAN_POINT ( 'NONE',  ( 204.6977192012829789, -170.0000000000000000, -16.98138044215791354 ) ) ;
#41049=AXIS2_PLACEMENT_3D ( 'NONE', #30498, #41407, #51951 ) ;
#41053=CARTESIAN_POINT ( 'NONE',  ( 173.8576514579035575, 72.97529922124006418, 38.83678981078923442 ) ) ;
#41054=AXIS2_PLACEMENT_3D ( 'NONE', #12339, #22890, #44333 ) ;
#41056=CARTESIAN_POINT ( 'NONE',  ( 19.54475376904848360, 6.649964688461121654, -63.36740267540860572 ) ) ;
#41057=CARTESIAN_POINT ( 'NONE',  ( -133.0835080491125098, 52.64966140620840918, 62.81293648280888675 ) ) ;
#41065=CARTESIAN_POINT ( 'NONE',  ( 141.0517870458594132, 47.14452711594498879, 39.14317607914329500 ) ) ;
#41066=CARTESIAN_POINT ( 'NONE',  ( 115.0606351894211485, 32.29586232625066344, 31.34211210427034899 ) ) ;
#41068=CARTESIAN_POINT ( 'NONE',  ( -101.3602137809054540, 32.31558061113913283, -76.81699020212612083 ) ) ;
#41071=ORIENTED_EDGE ( 'NONE', *, *, #20805, .F. ) ;
#41072=CARTESIAN_POINT ( 'NONE',  ( -147.3669217311067712, 63.69361261596466761, -22.65969703386014800 ) ) ;
#41076=CARTESIAN_POINT ( 'NONE',  ( -47.76881570271230970, 13.88249791001275391, -94.56390181705104681 ) ) ;
#41079=CARTESIAN_POINT ( 'NONE',  ( -120.5002574492098688, 44.22930148497319891, 43.33742215016130217 ) ) ;
#41080=CARTESIAN_POINT ( 'NONE',  ( 208.5889601154908632, 111.8333159387241693, 57.12700094515400906 ) ) ;
#41082=CARTESIAN_POINT ( 'NONE',  ( -107.7886332494339854, 36.81249801143972178, 43.13215690507624345 ) ) ;
#41083=ORIENTED_EDGE ( 'NONE', *, *, #22534, .T. ) ;
#41085=CARTESIAN_POINT ( 'NONE',  ( 83.52009074181535198, 19.44074360878495966, -90.13814207189352601 ) ) ;
#41088=CARTESIAN_POINT ( 'NONE',  ( 204.6977192012829789, 106.3443248447423599, 2.363170148305747009 ) ) ;
#41090=CARTESIAN_POINT ( 'NONE',  ( 8.000000000000007105, 249.8719672152120381, -95.00000000000133582 ) ) ;
#41093=CARTESIAN_POINT ( 'NONE',  ( 33.03722315490662709, 7.666819786578629170, 14.54433801149057537 ) ) ;
#41094=CARTESIAN_POINT ( 'NONE',  ( -11.79249160485393766, 8.191429102467035150, -36.54839574459859364 ) ) ;
#41100=VERTEX_POINT ( 'NONE', #3384 ) ;
#41102=CARTESIAN_POINT ( 'NONE',  ( -62.29496909743952671, 17.79481128341708285, 66.62724933386981263 ) ) ;
#41103=CARTESIAN_POINT ( 'NONE',  ( -30.95355748062275936, 9.511738996772322707, 3.371903815725488140 ) ) ;
#41108=CARTESIAN_POINT ( 'NONE',  ( -38.92726670956012924, 10.94099576009806718, 37.22770458825116435 ) ) ;
#41113=CARTESIAN_POINT ( 'NONE',  ( 180.6713229637342693, 79.61878926895393249, -24.38050707541595941 ) ) ;
#41117=CARTESIAN_POINT ( 'NONE',  ( -180.6215424137752166, 97.48070480470860844, -68.75056467222114520 ) ) ;
#41119=CARTESIAN_POINT ( 'NONE',  ( 134.5432377632815815, 43.01906612978911681, 83.22447129036004299 ) ) ;
#41120=CARTESIAN_POINT ( 'NONE',  ( 117.0065308422768453, 32.13872219870568614, 33.86034543354286086 ) ) ;
#41123=LINE ( 'NONE', #8783, #54712 ) ;
#41125=CARTESIAN_POINT ( 'NONE',  ( 188.4365915667139006, 87.87248959723054043, 38.31765364999172618 ) ) ;
#41126=CARTESIAN_POINT ( 'NONE',  ( 139.3041645503688528, 46.00819478311335331, 5.004763042418960417 ) ) ;
#41128=EDGE_LOOP ( 'NONE', ( #26468, #49960, #60513, #9688 ) ) ;
#41129=CARTESIAN_POINT ( 'NONE',  ( 159.6614743841975042, 60.66237087206236822, -23.96642233299556324 ) ) ;
#41134=CARTESIAN_POINT ( 'NONE',  ( 140.6546466870198628, 45.68345804077596739, 87.51171208969724091 ) ) ;
#41136=CARTESIAN_POINT ( 'NONE',  ( 155.2992895652388086, 57.24699634758579236, 2.872173225997780133 ) ) ;
#41138=CARTESIAN_POINT ( 'NONE',  ( 161.7006237583813970, 62.31514460450499371, -49.83437428245752443 ) ) ;
#41141=CARTESIAN_POINT ( 'NONE',  ( 162.7921669283191477, 61.91024532638673605, -48.91460448534603955 ) ) ;
#41153=CARTESIAN_POINT ( 'NONE',  ( 149.9872551245001091, 52.05943539582077761, 64.32859008368343723 ) ) ;
#41157=CARTESIAN_POINT ( 'NONE',  ( -94.83794676023106263, 30.26879337035743944, 65.92642283735828812 ) ) ;
#41158=CARTESIAN_POINT ( 'NONE',  ( -13.47517652744367034, 8.334971000693553123, 69.41689693878558387 ) ) ;
#41160=EDGE_CURVE ( 'NONE', #41997, #64948, #12913, .T. ) ;
#41163=CARTESIAN_POINT ( 'NONE',  ( 204.6977192012829505, 108.0580384837234931, -24.48138044215792419 ) ) ;
#41164=CARTESIAN_POINT ( 'NONE',  ( 103.5849290181278803, 27.01613348792541913, 33.64945997442609382 ) ) ;
#41166=CARTESIAN_POINT ( 'NONE',  ( -55.05276343752909440, 15.72344139423348430, -23.37177340799619785 ) ) ;
#41167=CARTESIAN_POINT ( 'NONE',  ( 188.4920037102894241, 87.93425473911916868, 11.17357535198952867 ) ) ;
#41168=CARTESIAN_POINT ( 'NONE',  ( 211.3917124729450734, 115.9987099435923597, -40.43198958513412578 ) ) ;
#41169=CARTESIAN_POINT ( 'NONE',  ( 178.1999009735081358, 75.73911533785327777, 16.89086260446840981 ) ) ;
#41170=CARTESIAN_POINT ( 'NONE',  ( -58.32860549785896609, 15.58423118879329472, 4.221608677645580343 ) ) ;
#41171=VERTEX_POINT ( 'NONE', #35051 ) ;
#41174=CARTESIAN_POINT ( 'NONE',  ( 102.7425154123292828, 25.56407025871219219, -70.50869499390829276 ) ) ;
#41175=CARTESIAN_POINT ( 'NONE',  ( 41.80372346091802882, 9.750024116765237281, -9.166004075864405465 ) ) ;
#41178=CARTESIAN_POINT ( 'NONE',  ( -0.7270333525066480229, 6.532611081232851724, 93.81168647148426487 ) ) ;
#41179=CARTESIAN_POINT ( 'NONE',  ( -106.6711220790663077, 36.20923238211246797, -21.75507159268790147 ) ) ;
#41181=CARTESIAN_POINT ( 'NONE',  ( -72.76696720809546548, 20.16136115364205494, 69.42024918034346115 ) ) ;
#41182=CARTESIAN_POINT ( 'NONE',  ( -166.2028657618940599, 79.74389853943287676, 68.07680179289491207 ) ) ;
#41185=CARTESIAN_POINT ( 'NONE',  ( -152.5046761101291963, 66.76407727525177904, 45.09959997925059838 ) ) ;
#41187=CARTESIAN_POINT ( 'NONE',  ( 176.0745160362857860, 73.68684431790052258, -11.29378876841035684 ) ) ;
#41195=CARTESIAN_POINT ( 'NONE',  ( 207.8484262634767674, 110.7633525054914401, 3.044159929133792186 ) ) ;
#41196=CARTESIAN_POINT ( 'NONE',  ( 8.336237313193162635, 7.382629160459399209, 65.33688261179428025 ) ) ;
#41197=CARTESIAN_POINT ( 'NONE',  ( 211.5175447467296408, 116.1901475271413915, 39.84285645812254018 ) ) ;
#41199=FACE_BOUND ( 'NONE', #30457, .T. ) ;
#41200=CARTESIAN_POINT ( 'NONE',  ( 68.11829950231073383, 13.91429225309574313, 85.49552249958776429 ) ) ;
#41203=ORIENTED_EDGE ( 'NONE', *, *, #23784, .T. ) ;
#41204=VERTEX_POINT ( 'NONE', #56493 ) ;
#41206=CARTESIAN_POINT ( 'NONE',  ( -119.4731043141009792, 43.59103079130043312, 87.91918064160569202 ) ) ;
#41207=CARTESIAN_POINT ( 'NONE',  ( -165.6398193834832284, 79.16932278174802207, -15.97813448833655592 ) ) ;
#41208=DIRECTION ( 'NONE',  ( -0.000000000000000000, 1.000000000000000000, -0.000000000000000000 ) ) ;
#41209=CARTESIAN_POINT ( 'NONE',  ( 22.13124724433581392, 6.786568030646046523, 87.18837163059359341 ) ) ;
#41210=CARTESIAN_POINT ( 'NONE',  ( 23.12438659259228046, 7.854523583799140063, 89.61051317704388453 ) ) ;
#41211=ORIENTED_EDGE ( 'NONE', *, *, #52767, .F. ) ;
#41214=CARTESIAN_POINT ( 'NONE',  ( 199.9103251464698303, 101.6434290204574893, -38.04802015360730394 ) ) ;
#41215=ORIENTED_EDGE ( 'NONE', *, *, #7929, .T. ) ;
#41217=FACE_OUTER_BOUND ( 'NONE', #24542, .T. ) ;
#41219=CARTESIAN_POINT ( 'NONE',  ( -59.58556642339446796, 16.99097764963620705, -9.876509403717985691 ) ) ;
#41220=B_SPLINE_CURVE_WITH_KNOTS ( 'NONE', 3,
 ( #31555, #68826, #4141, #20649, #63568, #56918, #36148, #8734, #20304, #68500, #67815, #25607, #36840, #15381, #35806, #41769, #52993, #4814, #46005, #67471, #19266, #40719, #30183, #19618, #62539, #57258, #9071, #30524, #3786, #25256, #63909, #10434, #26629, #43479, #47718, #11129, #15723, #31904, #48389, #65300, #64254, #27302, #37869, #53335 ),
 .UNSPECIFIED., .F., .F.,
 ( 4, 2, 2, 2, 2, 2, 2, 2, 2, 2, 2, 2, 2, 2, 2, 2, 2, 2, 2, 2, 2, 4 ),
 ( 0.000000000000000000, 0.001487235713946800280, 0.002230853570920181446, 0.002974471427893562395, 0.004461707141840288299, 0.005948942855787013768, 0.007436178569733738371, 0.008179796426707101539, 0.008923414283680465575, 0.01041064999762722661, 0.01189788571157398590, 0.01264150356854737769, 0.01338512142552076949, 0.01487235713946754440, 0.01561597499644093792, 0.01635959285341433492, 0.01784682856736112197, 0.01933406428130791249, 0.02007768213828130602, 0.02082129999525470301, 0.02230853570920150047, 0.02379577142314829794 ),
 .UNSPECIFIED. ) ;
#41224=CARTESIAN_POINT ( 'NONE',  ( 8.480442907658520824, 6.376693431076494889, -41.31410600788661469 ) ) ;
#41227=CARTESIAN_POINT ( 'NONE',  ( 108.3753929817421238, 29.13179266688724312, 17.54579741615193100 ) ) ;
#41228=EDGE_LOOP ( 'NONE', ( #6870, #57262, #54007, #1059 ) ) ;
#41230=CARTESIAN_POINT ( 'NONE',  ( -24.01932733213275739, 8.490648912832073236, 92.54723777928531092 ) ) ;
#41232=CARTESIAN_POINT ( 'NONE',  ( 180.2565361171340896, 79.19912802278403774, -78.03579697056984799 ) ) ;
#41234=CARTESIAN_POINT ( 'NONE',  ( 107.2672065034543465, 27.52931006625853172, -50.31091384885557716 ) ) ;
#41239=EDGE_LOOP ( 'NONE', ( #38883, #50238 ) ) ;
#41243=EDGE_LOOP ( 'NONE', ( #10568, #60782, #52572, #11880 ) ) ;
#41244=CARTESIAN_POINT ( 'NONE',  ( -85.89078989036967471, 26.29712602777652819, -71.49050017303922289 ) ) ;
#41245=CARTESIAN_POINT ( 'NONE',  ( -2.460717450366728620, 6.600113625476148549, -91.29677748862752651 ) ) ;
#41249=CARTESIAN_POINT ( 'NONE',  ( 127.2202105166096402, 37.55913282978157497, 6.662491736991211333 ) ) ;
#41250=CARTESIAN_POINT ( 'NONE',  ( 36.01249374622354082, 7.992843789158042611, -90.11533793215521371 ) ) ;
#41252=CARTESIAN_POINT ( 'NONE',  ( 204.6977192012829789, -170.0000000000000000, 56.05227132923312183 ) ) ;
#41254=CARTESIAN_POINT ( 'NONE',  ( -105.8879439778144445, 34.65133284149107595, 31.42656481232496901 ) ) ;
#41257=CARTESIAN_POINT ( 'NONE',  ( 8.288696687633807514, 7.382586467017839382, -16.67527755506199938 ) ) ;
#41258=ORIENTED_EDGE ( 'NONE', *, *, #21752, .T. ) ;
#41261=CARTESIAN_POINT ( 'NONE',  ( -149.0764453401867229, 65.13297611514535390, 3.876270649435373805 ) ) ;
#41263=DIRECTION ( 'NONE',  ( 0.000000000000000000, 0.000000000000000000, 1.000000000000000000 ) ) ;
#41265=CARTESIAN_POINT ( 'NONE',  ( 33.44527180510249309, 7.709232309484704615, -47.70323226738239697 ) ) ;
#41267=CARTESIAN_POINT ( 'NONE',  ( 8.540564391411910705, 7.383006541823031732, -44.96353512608188652 ) ) ;
#41268=DIRECTION ( 'NONE',  ( 0.000000000000000000, 0.000000000000000000, 1.000000000000000000 ) ) ;
#41269=ORIENTED_EDGE ( 'NONE', *, *, #24502, .F. ) ;
#41271=DIRECTION ( 'NONE',  ( -0.000000000000000000, 1.000000000000000000, -0.000000000000000000 ) ) ;
#41273=CARTESIAN_POINT ( 'NONE',  ( -25.98312968277007684, 8.759224980175259745, -74.81367083702784271 ) ) ;
#41274=CARTESIAN_POINT ( 'NONE',  ( 8.528421445032394743, 6.376778749352033593, 8.724639706960820362 ) ) ;
#41275=CARTESIAN_POINT ( 'NONE',  ( 42.71247067544614140, 9.879726907348448606, -76.69866368401555690 ) ) ;
#41276=DIRECTION ( 'NONE',  ( 0.000000000000000000, 0.000000000000000000, 1.000000000000000000 ) ) ;
#41277=CARTESIAN_POINT ( 'NONE',  ( 176.0745160362857860, 73.68684431790050837, -64.98288994933773211 ) ) ;
#41280=CARTESIAN_POINT ( 'NONE',  ( -176.3896317155480062, 90.84057090619019448, -48.97646663013337331 ) ) ;
#41281=CARTESIAN_POINT ( 'NONE',  ( 91.13361825170460406, 21.00701373666981198, -10.46045707455249563 ) ) ;
#41282=CARTESIAN_POINT ( 'NONE',  ( -26.49928411671542605, 9.848831533840664676, 70.22566193647604393 ) ) ;
#41286=EDGE_CURVE ( 'NONE', #7422, #52011, #58352, .T. ) ;
#41287=ORIENTED_EDGE ( 'NONE', *, *, #4434, .T. ) ;
#41291=CARTESIAN_POINT ( 'NONE',  ( -127.6992109187851980, 47.69334801994793338, -76.55208594102460040 ) ) ;
#41293=CARTESIAN_POINT ( 'NONE',  ( -47.68742944762956881, 12.82957801017945343, -41.23781885043871398 ) ) ;
#41297=ORIENTED_EDGE ( 'NONE', *, *, #65529, .F. ) ;
#41300=DIRECTION ( 'NONE',  ( -0.000000000000000000, 1.000000000000000000, -0.000000000000000000 ) ) ;
#41305=CARTESIAN_POINT ( 'NONE',  ( -180.5230320745700965, 95.76406004447554210, -70.30535114727260293 ) ) ;
#41306=CARTESIAN_POINT ( 'NONE',  ( 136.2687650510572155, 44.08481419469791263, -90.10835114847000682 ) ) ;
#41308=LINE ( 'NONE', #62415, #27805 ) ;
#41311=DIRECTION ( 'NONE',  ( -0.000000000000000000, 1.000000000000000000, -0.000000000000000000 ) ) ;
#41313=CARTESIAN_POINT ( 'NONE',  ( -55.05276343752910151, -170.0000000000000000, 57.16187836339483397 ) ) ;
#41314=CARTESIAN_POINT ( 'NONE',  ( -25.79929641484368830, 9.749255553662438345, -20.94138654446484438 ) ) ;
#41315=LINE ( 'NONE', #62770, #26431 ) ;
#41317=CARTESIAN_POINT ( 'NONE',  ( 107.0555969502564437, 28.53646637607230829, -23.38328407531912490 ) ) ;
#41318=CARTESIAN_POINT ( 'NONE',  ( 11.21387192505587294, 6.397095920409659797, 58.39573670284872975 ) ) ;
#41319=B_SPLINE_CURVE_WITH_KNOTS ( 'NONE', 3,
 ( #33422, #28837, #17212, #1397, #34115, #6673, #38686, #12302, #61189, #34473, #55203, #46734, #8778, #68205, #20013, #19307, #57986, #68541 ),
 .UNSPECIFIED., .F., .F.,
 ( 4, 2, 2, 2, 2, 2, 2, 2, 4 ),
 ( 0.000000000000000000, 0.001652083204940604571, 0.002478124807410915422, 0.003304166409881226056, 0.004956249614821870743, 0.006608332819762517164, 0.009912499229643743220, 0.01156458243458435668, 0.01321666563952497188 ),
 .UNSPECIFIED. ) ;
#41320=CARTESIAN_POINT ( 'NONE',  ( -24.32471770265757982, 9.546495606312143778, 35.29174336063405804 ) ) ;
#41321=CARTESIAN_POINT ( 'NONE',  ( 204.6977192012829505, 108.0580384837234931, 29.20772073876942088 ) ) ;
#41326=VERTEX_POINT ( 'NONE', #17025 ) ;
#41329=CARTESIAN_POINT ( 'NONE',  ( 110.7167338301703694, 30.21148223254618159, -62.76698815611733551 ) ) ;
#41330=AXIS2_PLACEMENT_3D ( 'NONE', #7217, #66331, #23051 ) ;
#41332=CARTESIAN_POINT ( 'NONE',  ( 197.8436586345020487, 97.39326576892288756, -73.76851244691899012 ) ) ;
#41334=FACE_OUTER_BOUND ( 'NONE', #23219, .T. ) ;
#41335=CARTESIAN_POINT ( 'NONE',  ( -118.4063383664799858, 41.75753822095644097, 65.47488579310427781 ) ) ;
#41338=CARTESIAN_POINT ( 'NONE',  ( -49.12372073857199695, 14.20664392157176437, 33.19790897520485373 ) ) ;
#41344=CARTESIAN_POINT ( 'NONE',  ( 103.5839822277950049, 25.92130892112108853, 67.41571189329286540 ) ) ;
#41345=CARTESIAN_POINT ( 'NONE',  ( 113.3994433585436923, 30.36970469616434087, 83.98924600679271180 ) ) ;
#41346=DIRECTION ( 'NONE',  ( -0.000000000000000000, 1.000000000000000000, -0.000000000000000000 ) ) ;
#41348=CARTESIAN_POINT ( 'NONE',  ( 182.7720841008444097, 80.32850885226592652, -51.03576020520832657 ) ) ;
#41350=CARTESIAN_POINT ( 'NONE',  ( -146.1773277338104720, 62.70721456556563567, 85.18395948454488575 ) ) ;
#41351=ORIENTED_EDGE ( 'NONE', *, *, #33020, .F. ) ;
#41356=CARTESIAN_POINT ( 'NONE',  ( -85.35127931077731489, 24.98147633333000428, 61.35301968501214276 ) ) ;
#41359=CARTESIAN_POINT ( 'NONE',  ( -58.75378739419586793, 16.75118858561005553, 31.27567419135673177 ) ) ;
#41360=CARTESIAN_POINT ( 'NONE',  ( -33.85171821065139852, 11.02091558840052521, -62.54379208760393993 ) ) ;
#41361=CARTESIAN_POINT ( 'NONE',  ( -156.4960819023051215, 70.34114605623871341, -12.69378895035390009 ) ) ;
#41363=CARTESIAN_POINT ( 'NONE',  ( 181.9411407973026087, 80.91291802046383452, 71.15314469597515767 ) ) ;
#41364=CARTESIAN_POINT ( 'NONE',  ( 8.683531412707427677, 6.377173148747124820, -13.75927345114389233 ) ) ;
#41366=CARTESIAN_POINT ( 'NONE',  ( -4.513903087372270306, 6.697902023160578366, -49.65186798646897870 ) ) ;
#41367=CARTESIAN_POINT ( 'NONE',  ( 181.9295719569814480, 79.46350097013163349, 56.18870136843697338 ) ) ;
#41368=CARTESIAN_POINT ( 'NONE',  ( -121.2008155373973466, 43.48033530165982796, 5.404909548456530821 ) ) ;
#41370=CARTESIAN_POINT ( 'NONE',  ( 126.5880720616305553, 37.20544379858408490, -14.81166450811346458 ) ) ;
#41371=CARTESIAN_POINT ( 'NONE',  ( 22.72762739171800206, 7.830015800126074232, -13.29790432193229321 ) ) ;
#41373=CARTESIAN_POINT ( 'NONE',  ( 12.47451846520756646, 7.423604437114562415, 3.937467224307672264 ) ) ;
#41374=EDGE_CURVE ( 'NONE', #32365, #49097, #34962, .T. ) ;
#41375=EDGE_LOOP ( 'NONE', ( #40711, #56738, #25010, #25480 ) ) ;
#41376=CARTESIAN_POINT ( 'NONE',  ( 186.6054783416232397, 84.37128553200979297, 4.863526534070675034 ) ) ;
#41378=CARTESIAN_POINT ( 'NONE',  ( 126.4318266066171930, 38.27072266789464550, -44.61505896352816336 ) ) ;
#41379=CARTESIAN_POINT ( 'NONE',  ( -128.7650348665116837, 48.41336321950710442, -35.48127487991890661 ) ) ;
#41381=CARTESIAN_POINT ( 'NONE',  ( 187.0788993276711665, 86.37277723143233743, -48.23884571524198606 ) ) ;
#41390=CARTESIAN_POINT ( 'NONE',  ( 156.3795552199950976, 58.07715209813575541, 83.15336215789184848 ) ) ;
#41392=CARTESIAN_POINT ( 'NONE',  ( 127.4992165631961285, 38.87141012667721895, -74.37822084336917783 ) ) ;
#41403=VERTEX_POINT ( 'NONE', #44474 ) ;
#41404=VERTEX_POINT ( 'NONE', #8588 ) ;
#41406=CARTESIAN_POINT ( 'NONE',  ( -178.0658882571760557, 92.80593104957422668, -21.01134249067511917 ) ) ;
#41407=DIRECTION ( 'NONE',  ( -0.000000000000000000, 1.000000000000000000, -0.000000000000000000 ) ) ;
#41413=CARTESIAN_POINT ( 'NONE',  ( -61.52143283897134296, 16.51181063611435462, -19.67550361010446380 ) ) ;
#41415=CARTESIAN_POINT ( 'NONE',  ( -133.3923804760465543, 52.87100816290223548, -69.82553800854516624 ) ) ;
#41416=CARTESIAN_POINT ( 'NONE',  ( 116.9197133427646804, 33.22079464767577406, 33.65725764894440886 ) ) ;
#41418=CARTESIAN_POINT ( 'NONE',  ( 70.45451534980406905, 15.56315969138428201, -71.05294828632224835 ) ) ;
#41421=CARTESIAN_POINT ( 'NONE',  ( -149.0764453401866945, 65.13297611514533969, -22.96827994102829251 ) ) ;
#41424=DIRECTION ( 'NONE',  ( -0.000000000000000000, 1.000000000000000000, -0.000000000000000000 ) ) ;
#41425=CARTESIAN_POINT ( 'NONE',  ( -54.20542732064039626, 15.49651042269896806, -88.94138983813944321 ) ) ;
#41427=CARTESIAN_POINT ( 'NONE',  ( -143.8566410313463564, 59.53044870492033169, 43.17841504270860753 ) ) ;
#41429=CARTESIAN_POINT ( 'NONE',  ( -165.6398193834832284, 79.16932278174806470, -69.66723566926393119 ) ) ;
#41431=CARTESIAN_POINT ( 'NONE',  ( -108.1180879163843116, 36.99199941971028238, 42.75380726691431477 ) ) ;
#41432=EDGE_LOOP ( 'NONE', ( #5218, #36686, #37073, #8853 ) ) ;
#41434=CARTESIAN_POINT ( 'NONE',  ( 79.39764314491567632, 18.13166883367086868, 62.05256806867162567 ) ) ;
#41439=CARTESIAN_POINT ( 'NONE',  ( 218.0000000000000000, 126.6235316737731296, -95.00000000000133582 ) ) ;
#41440=CARTESIAN_POINT ( 'NONE',  ( 31.90184941268615759, 7.552181687745348704, 10.32724003673442148 ) ) ;
#41442=CARTESIAN_POINT ( 'NONE',  ( -38.88884187334145537, 11.95889603743730056, -16.96948798090240373 ) ) ;
#41446=B_SPLINE_CURVE_WITH_KNOTS ( 'NONE', 3,
 ( #49434, #21669, #48726, #1265, #11451, #48375, #6547, #65283, #17435, #65642, #28342, #53673, #32579, #33289, #55067, #17078, #39259, #49082, #32239, #60703, #38911, #17802, #6185, #60355, #32921, #12176, #11812, #59990, #59637, #209, #43810, #33638, #16737, #64590, #38196, #570, #6885, #16398, #22022, #49786, #921, #37853, #1612, #23077, #66004, #5495 ),
 .UNSPECIFIED., .F., .F.,
 ( 4, 2, 2, 2, 2, 2, 2, 2, 2, 2, 2, 2, 2, 2, 2, 2, 2, 2, 2, 2, 2, 2, 4 ),
 ( 0.02404638330965504917, 0.02555608299537562300, 0.02631093283823590992, 0.02706578268109620031, 0.02857548236681679496, 0.02933033220967708882, 0.03008518205253738614, 0.03159488173825795304, 0.03310458142397851300, 0.03385943126683879645, 0.03461428110969907990, 0.03612398079541960516, 0.03687883063827988861, 0.03763368048114017206, 0.03838853032400045551, 0.03914338016686073896, 0.04065307985258127810, 0.04216277953830183112, 0.04367247922402237026, 0.04518217890974292328, 0.04593702875260319285, 0.04669187859546346242, 0.04820157828118400850 ),
 .UNSPECIFIED. ) ;
#41449=CARTESIAN_POINT ( 'NONE',  ( -60.66241560458684035, 16.25736033771450550, 32.81469839604517347 ) ) ;
#41451=CARTESIAN_POINT ( 'NONE',  ( -189.4223925288096098, 107.3427006758676612, 13.29886559940774049 ) ) ;
#41453=CARTESIAN_POINT ( 'NONE',  ( -14.92903005859420951, 7.458185427130747946, -67.34419620779377169 ) ) ;
#41455=CARTESIAN_POINT ( 'NONE',  ( -96.76159256735195413, 30.06445763698410190, -10.56742495184200159 ) ) ;
#41458=B_SPLINE_CURVE_WITH_KNOTS ( 'NONE', 3,
 ( #36204, #58673, #15092, #9821, #5220, #31279, #64308, #10838, #16115, #36550, #59022, #47426, #32309, #53737, #27015, #43185, #68880, #21733, #63629, #15443, #33705, #44228, #39322, #23497, #22438, #66074, #11521, #38618, #65009, #5896, #28407, #28058, #60765, #2045, #12590, #49855, #37923, #639, #54788, #16468, #64660, #990, #16802, #28771 ),
 .UNSPECIFIED., .F., .F.,
 ( 4, 2, 2, 2, 2, 2, 2, 2, 2, 2, 2, 2, 2, 2, 2, 2, 2, 2, 2, 2, 2, 4 ),
 ( 0.02432640572110343624, 0.02583721026359370523, 0.02659261253483881718, 0.02734801480608393259, 0.02885881934857419465, 0.02961422161981931006, 0.03036962389106442894, 0.03188042843355462508, 0.03339123297604482121, 0.03414663524728990540, 0.03490203751853499653, 0.03641284206102517185, 0.03716824433227024910, 0.03792364660351533329, 0.03943445114600548779, 0.04094525568849564923, 0.04245606023098580373, 0.04396686477347595823, 0.04472226704472104242, 0.04547766931596611967, 0.04698847385845632274, 0.04849927840094651887 ),
 .UNSPECIFIED. ) ;
#41463=CARTESIAN_POINT ( 'NONE',  ( 174.6307688320643194, 73.70327352127000609, -20.71130733032186200 ) ) ;
#41464=CARTESIAN_POINT ( 'NONE',  ( -188.6739852773920632, 108.2139733222100375, 63.56149477935467473 ) ) ;
#41467=CARTESIAN_POINT ( 'NONE',  ( -173.5422248620772621, 89.11126078969415687, -61.55650775521368701 ) ) ;
#41468=CARTESIAN_POINT ( 'NONE',  ( -0.7215816834507519095, 6.532459459468095808, -18.49149345562722146 ) ) ;
#41470=LINE ( 'NONE', #30566, #52879 ) ;
#41472=CARTESIAN_POINT ( 'NONE',  ( -120.1259246007803654, 42.81147313035992141, -64.43732786190635409 ) ) ;
#41474=CARTESIAN_POINT ( 'NONE',  ( 197.3059626281005592, 96.72682679064186573, 38.01856143111450592 ) ) ;
#41476=EDGE_CURVE ( 'NONE', #22455, #50199, #49123, .T. ) ;
#41477=CARTESIAN_POINT ( 'NONE',  ( 185.1710994180822354, 84.30654632312743502, 43.11307207121964780 ) ) ;
#41478=CARTESIAN_POINT ( 'NONE',  ( 141.3556389957210229, 47.34429831367555863, 10.46169434721303482 ) ) ;
#41481=CARTESIAN_POINT ( 'NONE',  ( 173.5836858989432301, 72.71885240881780987, 63.93992091031944369 ) ) ;
#41483=CARTESIAN_POINT ( 'NONE',  ( 67.93154431625913503, 14.90489441944787430, 58.47168318147574695 ) ) ;
#41484=CARTESIAN_POINT ( 'NONE',  ( 141.2060940825452064, 46.04283574924851052, 89.19312868080487533 ) ) ;
#41486=CARTESIAN_POINT ( 'NONE',  ( 154.0515132159916902, 56.29926936869306076, 3.373288628613766882 ) ) ;
#41488=CARTESIAN_POINT ( 'NONE',  ( -178.2427210808090479, 93.01567669683340966, 32.83739906211183524 ) ) ;
#41491=CARTESIAN_POINT ( 'NONE',  ( 116.6681538161788438, 33.09439081574000596, -47.32309755658299366 ) ) ;
#41494=CARTESIAN_POINT ( 'NONE',  ( 38.90907126433567242, 9.359889524363186553, 44.91383430596329163 ) ) ;
#41496=CARTESIAN_POINT ( 'NONE',  ( 136.1081004736419402, 42.80058051492066085, 56.69709667588018931 ) ) ;
#41497=CARTESIAN_POINT ( 'NONE',  ( -165.7699288023689803, 79.30174988963855753, 36.80611496506521263 ) ) ;
#41499=CARTESIAN_POINT ( 'NONE',  ( 133.6288034103009750, 41.28708886999546479, -77.86786152285937135 ) ) ;
#41501=DIRECTION ( 'NONE',  ( -0.000000000000000000, 1.000000000000000000, -0.000000000000000000 ) ) ;
#41504=CARTESIAN_POINT ( 'NONE',  ( 154.0281735872261493, 56.28213428456459866, -10.11222482322573413 ) ) ;
#41505=CARTESIAN_POINT ( 'NONE',  ( -50.37626225203914032, 13.47725392609373429, 85.63415519923331942 ) ) ;
#41506=CARTESIAN_POINT ( 'NONE',  ( 106.6181401479172308, 28.34160787025143691, 43.68143237657537981 ) ) ;
#41507=CARTESIAN_POINT ( 'NONE',  ( -150.3898662070192529, 64.92828409760431896, -61.65738112195564469 ) ) ;
#41508=CARTESIAN_POINT ( 'NONE',  ( 58.16156486118065772, 11.59853826451868564, 85.24551411657452604 ) ) ;
#41509=CARTESIAN_POINT ( 'NONE',  ( 181.0840389613909736, 80.03940679743416808, 2.464043515047717570 ) ) ;
#41510=CARTESIAN_POINT ( 'NONE',  ( 209.9944361927104239, 113.8994774711241291, -49.14096817356703895 ) ) ;
#41511=CARTESIAN_POINT ( 'NONE',  ( 174.1364721914477229, 71.85829564941442982, 7.124632976745406410 ) ) ;
#41512=( BOUNDED_CURVE ( )  B_SPLINE_CURVE ( 3, ( #50444, #2263, #23711, #18431 ),
 .UNSPECIFIED., .F., .F. ) 
 B_SPLINE_CURVE_WITH_KNOTS ( ( 4, 4 ),
 ( 2.506209174768084580, 3.776976132411494103 ),
 .UNSPECIFIED. ) 
 CURVE ( )  GEOMETRIC_REPRESENTATION_ITEM ( )  RATIONAL_B_SPLINE_CURVE ( ( 1.000000000000000000, 0.8698961108463049152, 0.8698961108463049152, 1.000000000000000000 ) ) 
 REPRESENTATION_ITEM ( '' )  );
#41513=ORIENTED_EDGE ( 'NONE', *, *, #35015, .T. ) ;
#41517=CARTESIAN_POINT ( 'NONE',  ( 55.57657751403269231, 11.06944050856661832, -71.05142857302701032 ) ) ;
#41518=CARTESIAN_POINT ( 'NONE',  ( -74.40004226286974642, 20.74218500375952701, 4.900570124997223331 ) ) ;
#41520=CARTESIAN_POINT ( 'NONE',  ( -0.3230440667461953463, 6.518512734653291396, 91.57163373586021748 ) ) ;
#41521=AXIS2_PLACEMENT_3D ( 'NONE', #11542, #28082, #26709 ) ;
#41522=CARTESIAN_POINT ( 'NONE',  ( -109.3386876948163433, 37.66246927061206407, -18.25541805540258622 ) ) ;
#41524=B_SPLINE_CURVE_WITH_KNOTS ( 'NONE', 3,
 ( #55947, #66862, #65455, #17963, #23591, #22886, #18304, #34506, #39412, #49957, #7762, #38361, #6356, #60860, #66512, #44329, #39076, #27811, #39762, #45383, #17249, #55231, #49598, #29211, #59806, #12683, #34150, #54530, #49249, #28870, #45029, #50658, #61219, #2478, #23933, #65816, #11620, #33094, #17610, #22535, #1082, #43973, #38719, #60518, #55585, #33792 ),
 .UNSPECIFIED., .F., .F.,
 ( 4, 2, 2, 2, 2, 2, 2, 2, 2, 2, 2, 2, 2, 2, 2, 2, 2, 2, 2, 2, 2, 2, 4 ),
 ( 0.000000000000000000, 0.001615199098318994761, 0.003230398196637989522, 0.004037997745797492107, 0.004845597294956995559, 0.006460796393276001595, 0.007268395942435538007, 0.008075995491595072684, 0.009691194589914093466, 0.01049879413907361947, 0.01130639368823314374, 0.01211399323739267148, 0.01292159278655219921, 0.01453679188487125643, 0.01615199098319031190, 0.01695959053234982056, 0.01776719008150933268, 0.01938238917982830489, 0.02099758827814728057, 0.02180518782730674412, 0.02261278737646620421, 0.02422798647478506540, 0.02584318557310392658 ),
 .UNSPECIFIED. ) ;
#41526=CARTESIAN_POINT ( 'NONE',  ( 203.3978200800095237, 104.5785882372513242, -90.12130148826626908 ) ) ;
#41529=CARTESIAN_POINT ( 'NONE',  ( -156.9910258076866114, 70.79617246506499839, 37.64717199668289282 ) ) ;
#41531=CARTESIAN_POINT ( 'NONE',  ( 59.08638499266955790, 11.79550614876701431, -49.61367700836938610 ) ) ;
#41534=VECTOR ( 'NONE', #35614, 1000.000000000000000 ) ;
#41535=EDGE_CURVE ( 'NONE', #16864, #6290, #38065, .T. ) ;
#41536=EDGE_LOOP ( 'NONE', ( #24296, #23041 ) ) ;
#41539=CARTESIAN_POINT ( 'NONE',  ( 211.3917124729449881, 115.9987099435922886, 13.25711159579326548 ) ) ;
#41540=CARTESIAN_POINT ( 'NONE',  ( 13.36262230781616012, 7.441298897118794997, 71.47295967330329347 ) ) ;
#41542=CARTESIAN_POINT ( 'NONE',  ( 14.12575540446280264, 6.452943588436218292, -89.38275910569522864 ) ) ;
#41544=EDGE_LOOP ( 'NONE', ( #18995, #36483 ) ) ;
#41547=CARTESIAN_POINT ( 'NONE',  ( -130.2612055759786074, 50.66074200725057608, 85.70470224599091580 ) ) ;
#41548=B_SPLINE_CURVE_WITH_KNOTS ( 'NONE', 3,
 ( #12411, #33868, #50396, #60941, #55310, #59882, #7129, #44770, #28590, #12760, #50043, #66246, #18038, #2211, #23662, #46837, #7833, #24710, #56021, #40523, #18378, #2903, #14144, #61972, #8873, #13792, #29622, #24008, #24363, #9211, #13116, #2554, #50731, #3583, #35943, #45808, #34583, #51088, #46144, #45454, #29282, #67287, #67614, #14488 ),
 .UNSPECIFIED., .F., .F.,
 ( 4, 2, 2, 2, 2, 2, 2, 2, 2, 2, 2, 2, 2, 2, 2, 2, 2, 2, 2, 2, 2, 4 ),
 ( 0.000000000000000000, 0.001472974678681641860, 0.002209462018022466910, 0.002945949357363291526, 0.004418924036044906932, 0.005891898714726521470, 0.007364873393408136008, 0.008101360732748960625, 0.008837848072089786108, 0.01031082275077139544, 0.01178379742945300651, 0.01252028476879383373, 0.01325677210813466095, 0.01472974678681628936, 0.01546623412615710617, 0.01620272146549792125, 0.01767569614417955487, 0.01914867082286118502, 0.01988515816220200877, 0.02062164550154282558, 0.02209462018022446961, 0.02356759485890611364 ),
 .UNSPECIFIED. ) ;
#41549=CARTESIAN_POINT ( 'NONE',  ( -168.7150276173048269, 82.35404041280330034, -9.279753688084731778 ) ) ;
#41551=CARTESIAN_POINT ( 'NONE',  ( 18.97610100625297491, 6.623071417957627993, 84.38338133953382680 ) ) ;
#41553=CARTESIAN_POINT ( 'NONE',  ( 79.82127737190242556, 17.20935440217363066, -73.32255258993723146 ) ) ;
#41556=CARTESIAN_POINT ( 'NONE',  ( -94.77925136849377452, 29.13093715379787696, 65.09547375720568141 ) ) ;
#41558=CARTESIAN_POINT ( 'NONE',  ( -85.09761763353358788, 24.87634954265997322, 14.94058973873350382 ) ) ;
#41560=CARTESIAN_POINT ( 'NONE',  ( -57.43883374585514900, 16.37892664338859916, -8.757341026728871825 ) ) ;
#41562=ORIENTED_EDGE ( 'NONE', *, *, #36471, .T. ) ;
#41563=CARTESIAN_POINT ( 'NONE',  ( -121.2119672714299412, 44.67540322905998806, 17.15459649910451745 ) ) ;
#41566=DIRECTION ( 'NONE',  ( 0.000000000000000000, 0.000000000000000000, 1.000000000000000000 ) ) ;
#41568=CARTESIAN_POINT ( 'NONE',  ( -24.56126296900623274, 8.563129532889934836, 94.41426630670055431 ) ) ;
#41569=CARTESIAN_POINT ( 'NONE',  ( 179.4227152810057930, 78.36166152262363482, -77.89550332129535093 ) ) ;
#41570=CARTESIAN_POINT ( 'NONE',  ( -126.3495878770406762, 48.00153794568859666, -8.069153307770246641 ) ) ;
#41571=CARTESIAN_POINT ( 'NONE',  ( 102.8458551240039611, 25.60773946375957166, -44.68694561986643521 ) ) ;
#41572=CARTESIAN_POINT ( 'NONE',  ( 84.27937148876358719, 19.69225537006224513, -50.44796742885471730 ) ) ;
#41577=CARTESIAN_POINT ( 'NONE',  ( -85.73740570227380431, 26.23277384689415115, -71.97308702196428953 ) ) ;
#41578=CARTESIAN_POINT ( 'NONE',  ( 174.2538192999570015, 73.34752463892027663, 6.853970190747312508 ) ) ;
#41580=EDGE_CURVE ( 'NONE', #20568, #6663, #59222, .T. ) ;
#41582=CARTESIAN_POINT ( 'NONE',  ( 131.6189313563687620, 40.08924984825279125, 17.33914888436516222 ) ) ;
#41583=CARTESIAN_POINT ( 'NONE',  ( -156.4960819023051499, 70.34114605623869920, 14.15076164010977600 ) ) ;
#41586=CARTESIAN_POINT ( 'NONE',  ( -81.00768240531211006, 24.30850321514432366, 57.63353788888659324 ) ) ;
#41590=CARTESIAN_POINT ( 'NONE',  ( -47.61678346849998178, 13.84663486211544026, 92.53719257853346392 ) ) ;
#41591=EDGE_LOOP ( 'NONE', ( #41351, #52244 ) ) ;
#41593=VERTEX_POINT ( 'NONE', #82 ) ;
#41594=CARTESIAN_POINT ( 'NONE',  ( 23.09590709048885060, 7.852755081912508928, -68.15776028566385492 ) ) ;
#41595=DIRECTION ( 'NONE',  ( -0.000000000000000000, 1.000000000000000000, -0.000000000000000000 ) ) ;
#41599=CARTESIAN_POINT ( 'NONE',  ( 134.7720294983483313, 43.15885542353190374, -36.06555109292058603 ) ) ;
#41600=CARTESIAN_POINT ( 'NONE',  ( 31.99894129856762603, 7.561773404408281607, -44.34697420425325021 ) ) ;
#41601=CARTESIAN_POINT ( 'NONE',  ( 11.81843724556920883, 7.412394300769733491, -36.65097937619014346 ) ) ;
#41603=CARTESIAN_POINT ( 'NONE',  ( -120.0051930351106648, 43.92079660368833771, -10.91750049354815388 ) ) ;
#41607=EDGE_LOOP ( 'NONE', ( #30969, #62151 ) ) ;
#41611=CARTESIAN_POINT ( 'NONE',  ( -26.88245755577922935, 8.887394979218514734, -75.63929455523587819 ) ) ;
#41615=CARTESIAN_POINT ( 'NONE',  ( 9.416603677636263825, 6.380307115728825806, 6.706382208024352920 ) ) ;
#41618=CARTESIAN_POINT ( 'NONE',  ( 206.3053863259449372, 110.3084416756849464, 17.23374409832117138 ) ) ;
#41621=CARTESIAN_POINT ( 'NONE',  ( 92.51858280840788495, 21.51505926344913533, -21.14771471057316177 ) ) ;
#41625=ADVANCED_FACE ( 'NONE', ( #18010 ), #44380, .F. ) ;
#41630=DIRECTION ( 'NONE',  ( -0.000000000000000000, 1.000000000000000000, -0.000000000000000000 ) ) ;
#41631=CARTESIAN_POINT ( 'NONE',  ( -47.56463531432803649, 12.80077789972090230, -42.22615997514142805 ) ) ;
#41633=FACE_OUTER_BOUND ( 'NONE', #40084, .T. ) ;
#41635=CARTESIAN_POINT ( 'NONE',  ( -0.4850857408069293442, 7.530899315854036935, 92.87821500056037394 ) ) ;
#41636=ADVANCED_FACE ( 'NONE', ( #23299 ), #50371, .F. ) ;
#41639=CARTESIAN_POINT ( 'NONE',  ( -61.51762070241279190, 16.51067482779403761, 68.47209165092128558 ) ) ;
#41642=CARTESIAN_POINT ( 'NONE',  ( 46.89562634055204882, 10.52219511967644650, 91.55471069079136726 ) ) ;
#41643=CARTESIAN_POINT ( 'NONE',  ( -179.0654441437004039, 93.99779465816536117, -73.63664225586808243 ) ) ;
#41644=CARTESIAN_POINT ( 'NONE',  ( 134.6156496652957628, 43.06323651754149040, -89.74142866289044207 ) ) ;
#41645=ORIENTED_EDGE ( 'NONE', *, *, #4786, .F. ) ;
#41646=CARTESIAN_POINT ( 'NONE',  ( -47.68562151781910785, 13.86286849776707797, -95.00000000000133582 ) ) ;
#41649=CARTESIAN_POINT ( 'NONE',  ( 55.91133443650746671, 12.16263767238153726, -45.67481826356996777 ) ) ;
#41650=CARTESIAN_POINT ( 'NONE',  ( -82.32006615997345023, 24.83050031643764655, 31.35040515247533577 ) ) ;
#41652=CARTESIAN_POINT ( 'NONE',  ( 91.67571176799445709, 21.20498955963030596, 31.65844119682673963 ) ) ;
#41655=AXIS2_PLACEMENT_3D ( 'NONE', #34047, #43877, #49498 ) ;
#41656=CARTESIAN_POINT ( 'NONE',  ( 106.0228389049370321, 28.07756796303168301, -22.78257232089758944 ) ) ;
#41657=CARTESIAN_POINT ( 'NONE',  ( 8.480442907658519047, 6.376693431076494889, 66.06409635396809676 ) ) ;
#41658=CARTESIAN_POINT ( 'NONE',  ( -24.71645982722742119, 9.599558729461499240, 41.05070016659301047 ) ) ;
#41659=CARTESIAN_POINT ( 'NONE',  ( 201.9822477997853412, 104.3642793804899895, 29.70478973244642873 ) ) ;
#41660=CARTESIAN_POINT ( 'NONE',  ( -72.03776141304246039, 20.97207231437463548, 88.08361387805356912 ) ) ;
#41663=CARTESIAN_POINT ( 'NONE',  ( 70.51522979775974420, 15.57935281015687323, 37.81516837416805998 ) ) ;
#41664=ORIENTED_EDGE ( 'NONE', *, *, #34077, .F. ) ;
#41667=CARTESIAN_POINT ( 'NONE',  ( 117.3246714514015707, 33.42485879931865611, -72.78854422093228038 ) ) ;
#41669=CARTESIAN_POINT ( 'NONE',  ( 203.1420903260746229, 104.2307086582027864, -63.28900608065381306 ) ) ;
#41670=CARTESIAN_POINT ( 'NONE',  ( -37.37206033059241861, 11.66494618096612967, 59.96638633092528892 ) ) ;
#41671=CARTESIAN_POINT ( 'NONE',  ( -120.4586945679390482, 43.01762219615316241, 70.15563910072147280 ) ) ;
#41672=CARTESIAN_POINT ( 'NONE',  ( -83.69370847062539553, 25.38703975185374517, -21.34185604462549790 ) ) ;
#41675=CARTESIAN_POINT ( 'NONE',  ( -157.0069704378501854, 70.81086990254192415, -41.73065021801657082 ) ) ;
#41677=ORIENTED_EDGE ( 'NONE', *, *, #15797, .F. ) ;
#41678=VECTOR ( 'NONE', #44268, 1000.000000000000000 ) ;
#41680=CARTESIAN_POINT ( 'NONE',  ( -78.66644367742111399, 23.39876645725287219, -50.11545063171791270 ) ) ;
#41681=CARTESIAN_POINT ( 'NONE',  ( 102.9219037530332486, 25.63991434460579200, 92.46589979971660966 ) ) ;
#41693=CARTESIAN_POINT ( 'NONE',  ( -84.97622048504844372, 24.82614411847755420, 60.70097479970424104 ) ) ;
#41697=CARTESIAN_POINT ( 'NONE',  ( -32.40928421737412890, 10.77259363352673915, -77.11483472157956953 ) ) ;
#41699=CARTESIAN_POINT ( 'NONE',  ( 32.46582168790594380, 7.608418697099895489, 67.14276555145990244 ) ) ;
#41700=CARTESIAN_POINT ( 'NONE',  ( 9.827939172326077610, 6.382931149346554811, -11.59534592424589228 ) ) ;
#41703=CARTESIAN_POINT ( 'NONE',  ( 21.75198946226450047, 7.772524967554915953, 6.095983826864362243 ) ) ;
#41704=CARTESIAN_POINT ( 'NONE',  ( 184.0013086981203401, 81.60415045669145684, 70.57588972765756807 ) ) ;
#41708=CARTESIAN_POINT ( 'NONE',  ( 16.77480716385436921, 7.540753720029936602, -23.62535031654175199 ) ) ;
#41709=CARTESIAN_POINT ( 'NONE',  ( 203.9276061909314990, 105.2889220654479061, 56.05227132923313604 ) ) ;
#41711=CIRCLE ( 'NONE', #49570, 243.4957430088094839 ) ;
#41712=ORIENTED_EDGE ( 'NONE', *, *, #15088, .T. ) ;
#41713=DIRECTION ( 'NONE',  ( -0.000000000000000000, 1.000000000000000000, -0.000000000000000000 ) ) ;
#41716=CARTESIAN_POINT ( 'NONE',  ( 176.6214367443247397, 74.20967084876662057, 42.85525822452583355 ) ) ;
#41719=CARTESIAN_POINT ( 'NONE',  ( -109.7686203588201295, 37.90089348911612888, -42.02286914772454907 ) ) ;
#41723=ORIENTED_EDGE ( 'NONE', *, *, #49743, .T. ) ;
#41726=CARTESIAN_POINT ( 'NONE',  ( 197.3700262219431067, 98.41176242030789467, 11.49295832791582050 ) ) ;
#41727=EDGE_LOOP ( 'NONE', ( #8446, #67443, #1704, #47014 ) ) ;
#41728=CARTESIAN_POINT ( 'NONE',  ( 151.3976820382521851, 54.32583990172415156, 94.99999999999866418 ) ) ;
#41730=CARTESIAN_POINT ( 'NONE',  ( 128.0882145863933772, 39.20607399008167704, -75.18710712909908978 ) ) ;
#41731=CARTESIAN_POINT ( 'NONE',  ( 130.7531879853686405, 39.58149302537893988, 43.85379998291934101 ) ) ;
#41733=CARTESIAN_POINT ( 'NONE',  ( -97.88309373898361798, 30.60238467438961862, 31.92441710568320801 ) ) ;
#41738=VERTEX_POINT ( 'NONE', #7103 ) ;
#41739=ORIENTED_EDGE ( 'NONE', *, *, #62280, .T. ) ;
#41740=CARTESIAN_POINT ( 'NONE',  ( -166.2053056899075045, 81.18967388993343093, 8.560883375255476935 ) ) ;
#41743=CARTESIAN_POINT ( 'NONE',  ( -175.9852529046322616, 90.37283472601129120, -8.422923135414874807 ) ) ;
#41744=CARTESIAN_POINT ( 'NONE',  ( -128.9863978264385480, 49.78205252558957739, 71.80115395911820997 ) ) ;
#41746=CARTESIAN_POINT ( 'NONE',  ( -106.7873000096882947, 36.27154431140346702, 85.70575407879229601 ) ) ;
#41750=ORIENTED_EDGE ( 'NONE', *, *, #9966, .F. ) ;
#41752=CARTESIAN_POINT ( 'NONE',  ( -62.15324028806259093, 16.70091357159900980, -13.40636474727677552 ) ) ;
#41755=CARTESIAN_POINT ( 'NONE',  ( -128.7724923851857000, 49.63576597317770478, -62.32888474247882016 ) ) ;
#41757=CARTESIAN_POINT ( 'NONE',  ( 57.83361077722076971, 11.53004742544596795, -91.47238847476954504 ) ) ;
#41759=CARTESIAN_POINT ( 'NONE',  ( 69.48877314113909165, 15.30784187978995448, -66.26917009106811918 ) ) ;
#41762=CARTESIAN_POINT ( 'NONE',  ( 182.7720841008444381, 80.32850885226592652, -77.88031079567201687 ) ) ;
#41767=CARTESIAN_POINT ( 'NONE',  ( -74.39861643904070831, 21.81123504700007487, 44.09021573614353429 ) ) ;
#41768=CARTESIAN_POINT ( 'NONE',  ( 81.04675113612958626, 17.59091904316107247, 42.24460685193674436 ) ) ;
#41769=CARTESIAN_POINT ( 'NONE',  ( 69.72564955710444679, 15.37006465677308853, -39.86102107153551088 ) ) ;
#41770=CARTESIAN_POINT ( 'NONE',  ( -122.1940143064357187, 45.29738883755587153, 44.64808725341385554 ) ) ;
#41771=CARTESIAN_POINT ( 'NONE',  ( -165.7699288023690087, 79.30174988963861438, -70.57208739678948461 ) ) ;
#41774=CARTESIAN_POINT ( 'NONE',  ( -102.2801239173131194, 32.78103895658057354, -8.170026674512225640 ) ) ;
#41775=ORIENTED_EDGE ( 'NONE', *, *, #42622, .F. ) ;
#41776=CARTESIAN_POINT ( 'NONE',  ( -38.16002576456688899, 10.79155573432543314, 7.534217346251379510 ) ) ;
#41778=EDGE_CURVE ( 'NONE', #5626, #56227, #27331, .T. ) ;
#41780=CARTESIAN_POINT ( 'NONE',  ( -189.9554299271397895, 108.0836897899587825, -65.72664125847879291 ) ) ;
#41783=LINE ( 'NONE', #41439, #669 ) ;
#41784=CARTESIAN_POINT ( 'NONE',  ( 34.45500533947588906, 7.817363290423890554, 16.22768104404066491 ) ) ;
#41787=EDGE_CURVE ( 'NONE', #55692, #22488, #37425, .T. ) ;
#41789=CARTESIAN_POINT ( 'NONE',  ( -124.4645780562616153, 46.76022866786750143, -88.73732779037004548 ) ) ;
#41792=CARTESIAN_POINT ( 'NONE',  ( 8.478575283864735468, 7.382882227715641399, -68.16705165657022292 ) ) ;
#41796=CARTESIAN_POINT ( 'NONE',  ( -94.88380767928869375, 29.17964217339916999, -14.40065432143456370 ) ) ;
#41797=CARTESIAN_POINT ( 'NONE',  ( 155.2992895652387801, 57.24699634758579947, -50.81692795492956805 ) ) ;
#41801=CARTESIAN_POINT ( 'NONE',  ( -150.5993571094983849, 66.43939758484181368, 57.64208039007107232 ) ) ;
#41803=CARTESIAN_POINT ( 'NONE',  ( -106.6711220790662935, 36.20923238211247508, 58.77858017870315877 ) ) ;
#41808=CARTESIAN_POINT ( 'NONE',  ( 87.59061758233883666, 19.75077892934020340, 71.51036996035465165 ) ) ;
#41809=EDGE_CURVE ( 'NONE', #52011, #59523, #21795, .T. ) ;
#41810=CARTESIAN_POINT ( 'NONE',  ( 116.6734749296699079, 31.97209464358272157, 41.00315203584806056 ) ) ;
#41814=CARTESIAN_POINT ( 'NONE',  ( 134.7770330630253284, 41.98246829846536343, 44.46794315559043298 ) ) ;
#41817=CARTESIAN_POINT ( 'NONE',  ( 204.6977192012829789, 106.3443248447423599, 29.20772073876942088 ) ) ;
#41818=CARTESIAN_POINT ( 'NONE',  ( 117.0065308422768595, 32.13872219870569324, -73.51785692831180086 ) ) ;
#41819=CARTESIAN_POINT ( 'NONE',  ( 188.5842358232186484, 88.03712271786936583, 36.50917097965209024 ) ) ;
#41820=CARTESIAN_POINT ( 'NONE',  ( 157.2533363798599737, 58.75760182111574892, 29.40946747225335756 ) ) ;
#41821=CARTESIAN_POINT ( 'NONE',  ( 140.0012045870120687, 45.26048451937214878, 94.99999999999866418 ) ) ;
#41823=EDGE_LOOP ( 'NONE', ( #5542, #14801, #45822, #59812 ) ) ;
#41826=CARTESIAN_POINT ( 'NONE',  ( -104.1342612728951593, 33.73231160250194449, -49.79675383502204511 ) ) ;
#41827=CARTESIAN_POINT ( 'NONE',  ( 139.5488375718656755, 44.96856655640365830, 85.77057805547978830 ) ) ;
#41828=CARTESIAN_POINT ( 'NONE',  ( -62.56514071794335052, 16.82532503654671885, 37.82479515852823937 ) ) ;
#41829=CARTESIAN_POINT ( 'NONE',  ( 150.9128604434957310, 53.97103482421775311, 6.386753527089024551 ) ) ;
#41830=ORIENTED_EDGE ( 'NONE', *, *, #24253, .F. ) ;
#41833=CARTESIAN_POINT ( 'NONE',  ( 114.6797682035589219, 32.10876583290006892, -49.48826977818937678 ) ) ;
#41834=ORIENTED_EDGE ( 'NONE', *, *, #26459, .T. ) ;
#41840=CARTESIAN_POINT ( 'NONE',  ( 133.8566784816069060, 41.42467568809810530, 56.35489142945903751 ) ) ;
#41842=CARTESIAN_POINT ( 'NONE',  ( -173.1211646369891071, 87.12891641440859303, 45.82169460664104577 ) ) ;
#41843=CARTESIAN_POINT ( 'NONE',  ( 150.7926588734435427, 52.63999027731880886, 67.17871942891498804 ) ) ;
#41844=CARTESIAN_POINT ( 'NONE',  ( 91.11019107624156277, 22.06959540317787827, 43.23133666582459966 ) ) ;
#41846=CARTESIAN_POINT ( 'NONE',  ( 46.12582897016703498, 10.39833982076227592, 13.90098705123808109 ) ) ;
#41847=VERTEX_POINT ( 'NONE', #38683 ) ;
#41848=CARTESIAN_POINT ( 'NONE',  ( 149.9683128897950155, 53.28564708287390062, -16.24937733141493368 ) ) ;
#41849=CARTESIAN_POINT ( 'NONE',  ( -61.59945957978030151, 16.53503624374673109, 87.83294754670791349 ) ) ;
#41850=CARTESIAN_POINT ( 'NONE',  ( 107.9213359589208920, 28.92595015506874390, 44.25850654564636244 ) ) ;
#41852=CARTESIAN_POINT ( 'NONE',  ( -156.1462053606562677, 70.02140399657012892, -65.65745857927204554 ) ) ;
#41853=CARTESIAN_POINT ( 'NONE',  ( 55.52619835477052135, 11.05941016560235823, 91.52244839951424638 ) ) ;
#41855=CARTESIAN_POINT ( 'NONE',  ( 184.9757174666827382, 84.09845285279331506, 3.548900157282363299 ) ) ;
#41863=CARTESIAN_POINT ( 'NONE',  ( 39.88975917505627677, 9.487965272711658571, -23.77526687496410673 ) ) ;
#41864=EDGE_CURVE ( 'NONE', #46944, #24801, #28833, .T. ) ;
#41868=CARTESIAN_POINT ( 'NONE',  ( -0.6810348268179097220, 6.531004596334747170, 88.99908247484378876 ) ) ;
#41869=CARTESIAN_POINT ( 'NONE',  ( -109.3585523124447576, 37.67345343047318806, -13.13767328143380375 ) ) ;
#41870=ORIENTED_EDGE ( 'NONE', *, *, #24458, .F. ) ;
#41875=CARTESIAN_POINT ( 'NONE',  ( -153.1121305730336815, 67.29834700374526335, 44.80172431058477400 ) ) ;
#41876=CARTESIAN_POINT ( 'NONE',  ( 55.61382797299286551, 11.07686102552912111, -44.45554761801439270 ) ) ;
#41879=CARTESIAN_POINT ( 'NONE',  ( -142.9728934044261734, 58.82891228489262403, 7.656646529977067850 ) ) ;
#41881=CARTESIAN_POINT ( 'NONE',  ( -133.3316503378477478, 52.82738260200862612, 37.01664400818041400 ) ) ;
#41883=CARTESIAN_POINT ( 'NONE',  ( 212.0850679406003678, 117.0583048437722056, 11.20260716300226633 ) ) ;
#41884=CARTESIAN_POINT ( 'NONE',  ( -142.0729208125266609, 59.40063722436772053, 39.35843688284292341 ) ) ;
#41885=CARTESIAN_POINT ( 'NONE',  ( 211.0967808702091020, 115.5516932918876734, 32.78604062416883380 ) ) ;
#41887=VERTEX_POINT ( 'NONE', #23213 ) ;
#41890=CARTESIAN_POINT ( 'NONE',  ( -120.0222670449324767, 43.93136592529501172, 87.13176881600898582 ) ) ;
#41892=CARTESIAN_POINT ( 'NONE',  ( -172.3057147739576749, 86.22480007276992353, -22.83448960614214585 ) ) ;
#41894=CARTESIAN_POINT ( 'NONE',  ( 23.28688665153870474, 6.856560375048495359, 91.56380556558386274 ) ) ;
#41895=CARTESIAN_POINT ( 'NONE',  ( 10.03051694092593316, 7.390832984323265187, 86.38638643135473671 ) ) ;
#41897=EDGE_LOOP ( 'NONE', ( #57060, #41215, #48208, #48039 ) ) ;
#41899=CARTESIAN_POINT ( 'NONE',  ( -98.69283175933881580, 30.99524616306737101, 58.25983389827380421 ) ) ;
#41900=ORIENTED_EDGE ( 'NONE', *, *, #68025, .F. ) ;
#41902=CARTESIAN_POINT ( 'NONE',  ( -82.53770812813169755, 23.83403279300011590, 4.645480920856400076 ) ) ;
#41903=ORIENTED_EDGE ( 'NONE', *, *, #62489, .F. ) ;
#41907=CARTESIAN_POINT ( 'NONE',  ( 11.82322073186612954, 6.406156243758795554, -49.38981688001822334 ) ) ;
#41908=CARTESIAN_POINT ( 'NONE',  ( -174.7800083645697100, 88.99302808536937448, 57.84004054586915800 ) ) ;
#41909=CARTESIAN_POINT ( 'NONE',  ( 133.8566784816069060, 41.42467568809810530, 56.35489142945903751 ) ) ;
#41910=B_SPLINE_CURVE_WITH_KNOTS ( 'NONE', 3,
 ( #7706, #34091, #66807, #28812, #44975, #66458, #50602, #2422, #23877, #18598, #14699, #62555, #46709, #63239, #24921, #3124, #8397, #57620, #15051, #24584, #51651, #35117, #67485, #56933, #56575, #29491, #30538, #67834, #29843, #30888, #18947, #3459, #2767, #47056, #36161, #30200, #41094, #45681, #35822, #51987, #13664, #46018, #46354, #40393, #19281 ),
 .UNSPECIFIED., .F., .F.,
 ( 4, 2, 2, 1, 2, 2, 2, 2, 2, 2, 2, 2, 2, 2, 2, 2, 2, 2, 2, 2, 2, 2, 4 ),
 ( 0.02346464386237015476, 0.02493212228186622928, 0.02566586149161426827, 0.02639960070136230380, 0.02713333991111034280, 0.02786707912085838179, 0.02933455754035447019, 0.03006829675010251959, 0.03080203595985056900, 0.03226951437934669209, 0.03300325358909474843, 0.03373699279884281171, 0.03520447121833893134, 0.03667194963783505096, 0.03740568884758310730, 0.03813942805733116365, 0.03960690647682728327, 0.04107438489632340983, 0.04254186331581952946, 0.04327560252556759968, 0.04400934173531566990, 0.04547682015481181034, 0.04694429857430795078 ),
 .UNSPECIFIED. ) ;
#41911=ORIENTED_EDGE ( 'NONE', *, *, #13989, .F. ) ;
#41912=EDGE_CURVE ( 'NONE', #36296, #8726, #25619, .T. ) ;
#41913=CARTESIAN_POINT ( 'NONE',  ( 110.2429982417149574, -170.0000000000000000, -24.07788697519002596 ) ) ;
#41915=EDGE_CURVE ( 'NONE', #6663, #20568, #38169, .T. ) ;
#41918=CARTESIAN_POINT ( 'NONE',  ( -26.87327614295025313, 8.886070347947290671, 43.68680226973125258 ) ) ;
#41923=CARTESIAN_POINT ( 'NONE',  ( -86.16710354151693707, 26.41338104675949694, -69.22550752038515043 ) ) ;
#41924=CARTESIAN_POINT ( 'NONE',  ( 173.7263186949344060, 72.85225335320951956, 8.481618603203305184 ) ) ;
#41927=CARTESIAN_POINT ( 'NONE',  ( 131.6005058089755266, 40.07838125795770878, 2.997865343112388725 ) ) ;
#41928=CARTESIAN_POINT ( 'NONE',  ( 33.00361537314734051, 7.663360536940698964, -92.89042083272292416 ) ) ;
#41929=CARTESIAN_POINT ( 'NONE',  ( 197.9644510826045689, 99.15771744523051723, 93.72331163113166497 ) ) ;
#41932=CARTESIAN_POINT ( 'NONE',  ( -109.5025362253418564, 36.60371748273998094, 40.10572810313013292 ) ) ;
#41935=CARTESIAN_POINT ( 'NONE',  ( -47.66938934256014448, 13.85902735690713250, 92.86349970662286069 ) ) ;
#41940=CARTESIAN_POINT ( 'NONE',  ( 204.6977192012829789, -170.0000000000000000, -97.51503221354896311 ) ) ;
#41943=B_SPLINE_CURVE_WITH_KNOTS ( 'NONE', 3,
 ( #43095, #64563, #53982, #5808, #27262, #48700, #543, #21994, #23317, #60586, #19406, #34212, #3243, #67607 ),
 .UNSPECIFIED., .F., .F.,
 ( 4, 2, 2, 2, 2, 2, 4 ),
 ( 0.000000000000000000, 0.001269157135653070081, 0.002538314271306140162, 0.003807471406959210027, 0.005076628542612280325, 0.007614942813918446941, 0.01015325708522461443 ),
 .UNSPECIFIED. ) ;
#41944=CARTESIAN_POINT ( 'NONE',  ( -169.1122507277983118, 84.24359299875010265, 31.96755716570773131 ) ) ;
#41946=CARTESIAN_POINT ( 'NONE',  ( 140.4769819293527178, 46.76840769395176522, -47.05706312325354901 ) ) ;
#41947=CARTESIAN_POINT ( 'NONE',  ( 32.90953848114694580, 7.653665824624195757, -46.88272753811734361 ) ) ;
#41948=VECTOR ( 'NONE', #27567, 1000.000000000000000 ) ;
#41949=CARTESIAN_POINT ( 'NONE',  ( 155.7262569076171417, 56.30477153194511430, -36.27408474916799008 ) ) ;
#41951=CARTESIAN_POINT ( 'NONE',  ( -124.1095621208148430, 46.52671329146387791, -8.226765375838317240 ) ) ;
#41952=ORIENTED_EDGE ( 'NONE', *, *, #29937, .T. ) ;
#41954=ORIENTED_EDGE ( 'NONE', *, *, #28347, .F. ) ;
#41955=AXIS2_PLACEMENT_3D ( 'NONE', #6045, #54582, #5700 ) ;
#41956=CARTESIAN_POINT ( 'NONE',  ( 182.6575447192646209, 81.65756500564891951, 83.15904816998347826 ) ) ;
#41959=CARTESIAN_POINT ( 'NONE',  ( -168.1839487819771080, 83.25723186408069409, -9.716778674227802171 ) ) ;
#41962=CARTESIAN_POINT ( 'NONE',  ( 86.62931800182293784, 20.48449268398423584, 17.86753698201564688 ) ) ;
#41964=CARTESIAN_POINT ( 'NONE',  ( 180.6710448012267989, 78.18844465372403363, -78.06960825634332934 ) ) ;
#41966=CARTESIAN_POINT ( 'NONE',  ( 94.06703982324145841, 22.09435144471463630, -15.47962683577384446 ) ) ;
#41967=LINE ( 'NONE', #57456, #5029 ) ;
#41970=ORIENTED_EDGE ( 'NONE', *, *, #67294, .T. ) ;
#41971=CARTESIAN_POINT ( 'NONE',  ( 129.5225439633633755, 40.02995148249138424, 4.026654605326871028 ) ) ;
#41973=CARTESIAN_POINT ( 'NONE',  ( -53.14657859411973106, 15.21831473227210552, 71.91964493646879930 ) ) ;
#41974=CARTESIAN_POINT ( 'NONE',  ( -106.7004823116342749, 36.22460663120047997, -63.28115470610104154 ) ) ;
#41978=ORIENTED_EDGE ( 'NONE', *, *, #63766, .F. ) ;
#41980=CARTESIAN_POINT ( 'NONE',  ( -62.30100056228380367, 16.74548393487070896, 66.65337513678986170 ) ) ;
#41981=ORIENTED_EDGE ( 'NONE', *, *, #49368, .T. ) ;
#41982=ORIENTED_EDGE ( 'NONE', *, *, #6157, .F. ) ;
#41984=CARTESIAN_POINT ( 'NONE',  ( 45.60406750853972824, 10.31565594232976402, 86.83412138438860950 ) ) ;
#41985=CARTESIAN_POINT ( 'NONE',  ( -180.6009936245623351, 95.85948119829086522, -68.42513485405468998 ) ) ;
#41987=ORIENTED_EDGE ( 'NONE', *, *, #46368, .F. ) ;
#41989=CARTESIAN_POINT ( 'NONE',  ( -7.330690860789849772, 6.858814156830896458, 18.27103044898354867 ) ) ;
#41991=CARTESIAN_POINT ( 'NONE',  ( -1.454841858088668394, 7.566772088227304849, 6.805462143089243909 ) ) ;
#41992=CARTESIAN_POINT ( 'NONE',  ( 180.6713229637342408, 79.61878926895391828, -51.22505766587962484 ) ) ;
#41993=CARTESIAN_POINT ( 'NONE',  ( 164.6594616662011106, 63.46377020933756086, 92.76704941086832434 ) ) ;
#41995=CARTESIAN_POINT ( 'NONE',  ( 94.07616572255075482, 22.09777530676769430, 36.18770730423079129 ) ) ;
#41997=VERTEX_POINT ( 'NONE', #65534 ) ;
#42000=CARTESIAN_POINT ( 'NONE',  ( 105.8229724512851249, 27.98935528750253354, -22.64196685832511591 ) ) ;
#42002=CARTESIAN_POINT ( 'NONE',  ( 13.84937401517046318, 6.446378549072247388, 71.60848226474631417 ) ) ;
#42003=CARTESIAN_POINT ( 'NONE',  ( -28.81071653159243695, 10.19258396314335258, 44.74508666141489499 ) ) ;
#42004=CARTESIAN_POINT ( 'NONE',  ( 201.5876148766342908, 103.8397408698165378, 43.54586497944792711 ) ) ;
#42005=CARTESIAN_POINT ( 'NONE',  ( -75.42286590136558289, 22.18381414075804869, 84.83773244433049854 ) ) ;
#42007=EDGE_LOOP ( 'NONE', ( #53593, #6328, #16676, #2944 ) ) ;
#42008=EDGE_LOOP ( 'NONE', ( #50517, #54479 ) ) ;
#42010=ADVANCED_FACE ( 'NONE', ( #22266 ), #38087, .F. ) ;
#42011=VERTEX_POINT ( 'NONE', #39487 ) ;
#42013=CARTESIAN_POINT ( 'NONE',  ( 203.9276061909314421, 105.2889220654478777, -78.17048162308530834 ) ) ;
#42016=CARTESIAN_POINT ( 'NONE',  ( 157.4703587214989113, 57.65129005721576050, -62.96873488960130771 ) ) ;
#42017=CARTESIAN_POINT ( 'NONE',  ( 22.34696839782165867, 7.807102111783818188, -93.04585276060377907 ) ) ;
#42018=CARTESIAN_POINT ( 'NONE',  ( -149.9449619562961686, 64.55090813009799433, -49.81283053149199702 ) ) ;
#42022=CARTESIAN_POINT ( 'NONE',  ( 67.93317348534930034, 14.90531593353392026, -10.69219403348423292 ) ) ;
#42023=CARTESIAN_POINT ( 'NONE',  ( -85.89078989036968892, 26.29712602777651043, -44.64594958257553969 ) ) ;
#42024=CARTESIAN_POINT ( 'NONE',  ( 106.8765028100539496, 27.35519873236687260, 84.09029707093864658 ) ) ;
#42025=CARTESIAN_POINT ( 'NONE',  ( -155.1204242627070471, 70.44799358128194910, 6.395789732132856287 ) ) ;
#42026=EDGE_CURVE ( 'NONE', #68287, #42704, #59532, .T. ) ;
#42030=CARTESIAN_POINT ( 'NONE',  ( -189.9051212200399448, 108.7693414241253720, -92.42498137349568310 ) ) ;
#42031=ORIENTED_EDGE ( 'NONE', *, *, #31141, .T. ) ;
#42036=CARTESIAN_POINT ( 'NONE',  ( 89.35694261521391013, 21.43730924572641072, -90.01283748679323082 ) ) ;
#42039=CARTESIAN_POINT ( 'NONE',  ( 200.4590013143046860, 102.3556155835303088, 57.34765393025211466 ) ) ;
#42041=CARTESIAN_POINT ( 'NONE',  ( 31.95008798096002423, 7.556925044648909129, 65.24089643825568885 ) ) ;
#42042=CARTESIAN_POINT ( 'NONE',  ( 13.37366753069833258, 6.435102282077983737, -23.29209217290729939 ) ) ;
#42043=CARTESIAN_POINT ( 'NONE',  ( 18.20314211955701822, 7.596739727129570241, 3.552554644654912330 ) ) ;
#42044=CARTESIAN_POINT ( 'NONE',  ( 188.4359598230020651, 86.36951380984524462, 62.14128191421917791 ) ) ;
#42045=CARTESIAN_POINT ( 'NONE',  ( -123.4531143159639015, 44.90777521523904880, 4.179957208476558606 ) ) ;
#42046=CARTESIAN_POINT ( 'NONE',  ( 66.94779593213115731, 13.61918177102164762, -63.67398222617447345 ) ) ;
#42050=CARTESIAN_POINT ( 'NONE',  ( 201.5903370237274146, 102.1785392640257726, 56.71277855772954979 ) ) ;
#42051=B_SPLINE_CURVE_WITH_KNOTS ( 'NONE', 3,
 ( #65070, #27076, #22158, #342, #37987, #48860, #59430, #11243, #5963, #27423, #703, #43601, #16869, #38329, #17930, #2112, #39731, #7024, #22850, #45351, #28122, #28477 ),
 .UNSPECIFIED., .F., .F.,
 ( 4, 2, 2, 2, 2, 2, 2, 2, 2, 2, 4 ),
 ( 0.01030631445004988149, 0.01159271714570041245, 0.01223591849352568227, 0.01287911984135095382, 0.01416552253700148478, 0.01480872388482676327, 0.01545192523265203829, 0.01673832792830262650, 0.01738152927612790846, 0.01802473062395318695, 0.02059753601525430092 ),
 .UNSPECIFIED. ) ;
#42053=CARTESIAN_POINT ( 'NONE',  ( 185.1802655733641245, 82.84606286178495793, 16.26266218441142541 ) ) ;
#42057=CARTESIAN_POINT ( 'NONE',  ( -107.7677210873465867, 36.80113675102408166, -47.64980430669002232 ) ) ;
#42058=CARTESIAN_POINT ( 'NONE',  ( 188.5653887627527752, 88.01608521313127653, -44.33439866442006405 ) ) ;
#42060=EDGE_CURVE ( 'NONE', #57348, #21955, #12062, .T. ) ;
#42063=CARTESIAN_POINT ( 'NONE',  ( 173.6802822489493963, 71.43367662455597156, 91.71180641136416511 ) ) ;
#42066=CARTESIAN_POINT ( 'NONE',  ( 116.5096233816162083, 31.89062767870469983, 59.82761199116307438 ) ) ;
#42067=ORIENTED_EDGE ( 'NONE', *, *, #18828, .T. ) ;
#42068=CARTESIAN_POINT ( 'NONE',  ( 126.7877523219523255, 38.47018873135925077, -67.80797154038901908 ) ) ;
#42070=LINE ( 'NONE', #58580, #37576 ) ;
#42071=CARTESIAN_POINT ( 'NONE',  ( 164.2909821920446234, 63.15460073159351140, -94.16473412953207855 ) ) ;
#42072=CARTESIAN_POINT ( 'NONE',  ( 88.52345267551655184, 20.07594890262053866, -50.58241302559184049 ) ) ;
#42076=DIRECTION ( 'NONE',  ( -0.000000000000000000, 1.000000000000000000, -0.000000000000000000 ) ) ;
#42077=VERTEX_POINT ( 'NONE', #22966 ) ;
#42078=EDGE_CURVE ( 'NONE', #8034, #29948, #41548, .T. ) ;
#42080=CARTESIAN_POINT ( 'NONE',  ( -170.2856292770789821, 85.50720222068223109, 4.520652531662902263 ) ) ;
#42083=CARTESIAN_POINT ( 'NONE',  ( -173.9656771507955000, 88.06879734510550861, -7.867406574286302856 ) ) ;
#42087=FACE_OUTER_BOUND ( 'NONE', #33027, .T. ) ;
#42090=VECTOR ( 'NONE', #28563, 1000.000000000000000 ) ;
#42094=CARTESIAN_POINT ( 'NONE',  ( 134.3135005523732559, 42.87884033955815966, 29.52074435543002906 ) ) ;
#42096=CARTESIAN_POINT ( 'NONE',  ( 56.55557087522677762, 11.26645937438482115, -93.07732634674349015 ) ) ;
#42099=CARTESIAN_POINT ( 'NONE',  ( -102.2801239173131052, 32.78103895658057354, -61.85912785543958847 ) ) ;
#42102=CARTESIAN_POINT ( 'NONE',  ( 183.1910712700538681, 80.76073941711163684, -63.35883323969136427 ) ) ;
#42103=CARTESIAN_POINT ( 'NONE',  ( -165.9992860119575084, 79.53569239468049545, -44.58101777890279038 ) ) ;
#42107=CARTESIAN_POINT ( 'NONE',  ( 103.8325688302027459, 27.12251147381402561, -74.16827293220038086 ) ) ;
#42108=CARTESIAN_POINT ( 'NONE',  ( -75.00452312211128003, 22.03104735285380755, 31.36846399027299626 ) ) ;
#42109=CARTESIAN_POINT ( 'NONE',  ( 86.62931800182292363, 19.42108912189597092, 44.71208757247933363 ) ) ;
#42110=EDGE_CURVE ( 'NONE', #45314, #19626, #34833, .T. ) ;
#42111=CARTESIAN_POINT ( 'NONE',  ( -142.9730935922299295, 58.82921737386681116, 41.91139747252092462 ) ) ;
#42113=CARTESIAN_POINT ( 'NONE',  ( 212.1707951106656651, 117.1901534358505899, 64.21020998533151669 ) ) ;
#42115=CARTESIAN_POINT ( 'NONE',  ( -105.4589068214114462, 34.42476264325677704, -22.47934715272176476 ) ) ;
#42117=CARTESIAN_POINT ( 'NONE',  ( -38.15923928782689245, 10.79140400702259228, 14.21113170898300915 ) ) ;
#42118=CARTESIAN_POINT ( 'NONE',  ( 79.33384730094456927, 18.11203072455034047, 62.29897845281649182 ) ) ;
#42120=CARTESIAN_POINT ( 'NONE',  ( 86.62931800182293784, 19.42108912189599934, 17.86753698201564688 ) ) ;
#42123=CARTESIAN_POINT ( 'NONE',  ( 39.40195752203892710, 8.409560354027393103, -62.46436805589144114 ) ) ;
#42125=CARTESIAN_POINT ( 'NONE',  ( -38.93847286785603501, 11.96870349976818027, -16.47936910502927077 ) ) ;
#42130=CARTESIAN_POINT ( 'NONE',  ( 9.275903038161093406, 7.385619229189523516, -66.11132412825449478 ) ) ;
#42131=CARTESIAN_POINT ( 'NONE',  ( -24.19091603582231542, 8.513464105188681685, 12.81483973167518187 ) ) ;
#42132=LINE ( 'NONE', #31248, #28895 ) ;
#42133=CARTESIAN_POINT ( 'NONE',  ( -13.47230132170245653, 7.324574289401438065, -64.80259611343139170 ) ) ;
#42135=CARTESIAN_POINT ( 'NONE',  ( 154.4617654203035784, 56.60942201271841867, -50.50876627099340510 ) ) ;
#42137=ORIENTED_EDGE ( 'NONE', *, *, #57402, .T. ) ;
#42140=CARTESIAN_POINT ( 'NONE',  ( -150.3850953947693085, 66.25368649589884740, 72.52681933769164857 ) ) ;
#42142=CARTESIAN_POINT ( 'NONE',  ( -109.7156874346698174, 37.87149323084330632, 65.87937654599812731 ) ) ;
#42148=CARTESIAN_POINT ( 'NONE',  ( -4.513903087372272083, 6.697902023160598795, -22.80731739600529906 ) ) ;
#42149=CARTESIAN_POINT ( 'NONE',  ( 197.3064269725218765, 98.33232022113057269, -15.66748082040111534 ) ) ;
#42151=CARTESIAN_POINT ( 'NONE',  ( -143.2562389366337925, 59.05327470469417506, 87.75316541060529119 ) ) ;
#42154=CARTESIAN_POINT ( 'NONE',  ( 141.2366329129480675, 46.06278879703613427, 35.64775270001474183 ) ) ;
#42156=CARTESIAN_POINT ( 'NONE',  ( 198.7084915431530021, 98.47675983942193056, 32.18548563730031020 ) ) ;
#42157=CARTESIAN_POINT ( 'NONE',  ( 83.38619203015946368, 19.39783821526631513, 3.588035180901903765 ) ) ;
#42158=CARTESIAN_POINT ( 'NONE',  ( 183.1873354889582117, 82.20882912211247628, 29.59664944175426271 ) ) ;
#42159=CARTESIAN_POINT ( 'NONE',  ( 163.7379901688713062, 64.00402364591248272, 14.19210081108414201 ) ) ;
#42162=EDGE_CURVE ( 'NONE', #50858, #2381, #28980, .T. ) ;
#42163=CARTESIAN_POINT ( 'NONE',  ( 174.1422537179814469, 73.24254491731254291, 60.79958808295376116 ) ) ;
#42164=VERTEX_POINT ( 'NONE', #44684 ) ;
#42165=CARTESIAN_POINT ( 'NONE',  ( -102.7456062648101778, 33.01749955571778372, -50.01457726497594791 ) ) ;
#42168=CARTESIAN_POINT ( 'NONE',  ( -61.52143283897135717, 16.51181063611435818, 34.01359757082287416 ) ) ;
#42170=CARTESIAN_POINT ( 'NONE',  ( 154.4617654203035499, 56.60942201271836893, 3.180334909933947074 ) ) ;
#42172=CARTESIAN_POINT ( 'NONE',  ( 157.9121974517528315, 59.27335488206246339, -51.12418429913765294 ) ) ;
#42179=CARTESIAN_POINT ( 'NONE',  ( 135.6842057900327347, 42.53841116629839547, 71.14344607389850239 ) ) ;
#42180=CARTESIAN_POINT ( 'NONE',  ( -172.3018509397888067, 86.22053936367352378, 45.78839510999039675 ) ) ;
#42181=CARTESIAN_POINT ( 'NONE',  ( 152.1190604254710195, 53.60705199010334354, 58.49325996993837151 ) ) ;
#42182=DIRECTION ( 'NONE',  ( -0.000000000000000000, 1.000000000000000000, -0.000000000000000000 ) ) ;
#42183=VERTEX_POINT ( 'NONE', #43620 ) ;
#42184=CARTESIAN_POINT ( 'NONE',  ( 46.65974587859241041, 10.48396258569370509, 8.615397572259070103 ) ) ;
#42187=CARTESIAN_POINT ( 'NONE',  ( 150.5744176759382924, 53.72473166688033785, -19.74036240759600958 ) ) ;
#42189=CARTESIAN_POINT ( 'NONE',  ( -53.82256742816888817, 14.35433967245538511, 84.08070474350741108 ) ) ;
#42193=CARTESIAN_POINT ( 'NONE',  ( -153.5002794404625490, 67.64160439471093866, -75.51027764244948060 ) ) ;
#42197=CARTESIAN_POINT ( 'NONE',  ( 188.5842358232186200, 88.03712271786933741, 9.664620389188403493 ) ) ;
#42205=CARTESIAN_POINT ( 'NONE',  ( -71.22896441287284119, 20.69091426169410397, 63.76365484910760983 ) ) ;
#42206=CARTESIAN_POINT ( 'NONE',  ( -95.19652294162978023, 29.32558722310179178, -39.99725502653443954 ) ) ;
#42207=CARTESIAN_POINT ( 'NONE',  ( 59.95259601283822093, 11.98300577492410923, -76.91558238451790430 ) ) ;
#42210=DIRECTION ( 'NONE',  ( -0.8160245890732938934, -0.5780171883497599028, 0.000000000000000000 ) ) ;
#42217=CARTESIAN_POINT ( 'NONE',  ( -156.0171627975467743, 69.90368824761763733, 41.95465397809884678 ) ) ;
#42218=CARTESIAN_POINT ( 'NONE',  ( 56.53776994993147298, 11.26292242501182805, -39.43272109873624487 ) ) ;
#42222=ORIENTED_EDGE ( 'NONE', *, *, #18655, .T. ) ;
#42223=CARTESIAN_POINT ( 'NONE',  ( -132.0870433264402948, 51.94057326482882786, 42.35753507293710385 ) ) ;
#42225=ORIENTED_EDGE ( 'NONE', *, *, #18406, .F. ) ;
#42227=CARTESIAN_POINT ( 'NONE',  ( -142.5042386072304623, 59.74110826975219624, 35.48376318634494453 ) ) ;
#42228=CARTESIAN_POINT ( 'NONE',  ( 209.5118425285948831, 113.1852661712287471, 42.46319131594169960 ) ) ;
#42229=DIRECTION ( 'NONE',  ( -0.000000000000000000, 1.000000000000000000, -0.000000000000000000 ) ) ;
#42238=CARTESIAN_POINT ( 'NONE',  ( -120.8834178727915400, 44.46913122494650139, 86.21984674650981617 ) ) ;
#42240=DIRECTION ( 'NONE',  ( -0.000000000000000000, 1.000000000000000000, -0.000000000000000000 ) ) ;
#42243=CARTESIAN_POINT ( 'NONE',  ( 11.75170693505526032, 7.411272167608774275, 84.87420514505134861 ) ) ;
#42245=AXIS2_PLACEMENT_3D ( 'NONE', #17686, #34576, #19065 ) ;
#42249=ADVANCED_FACE ( 'NONE', ( #17238 ), #65090, .F. ) ;
#42251=CARTESIAN_POINT ( 'NONE',  ( -94.84390436305041305, 29.16104988397309938, 65.87395087744090461 ) ) ;
#42253=CARTESIAN_POINT ( 'NONE',  ( -85.10774223992955001, 24.88053943842881921, 7.223589135002512762 ) ) ;
#42258=EDGE_CURVE ( 'NONE', #24352, #34130, #64210, .T. ) ;
#42260=CARTESIAN_POINT ( 'NONE',  ( 10.83418588031599583, 6.392467435475928994, -48.67156742485343557 ) ) ;
#42261=CARTESIAN_POINT ( 'NONE',  ( -55.05276343752910151, -170.0000000000000000, 72.16187836339486239 ) ) ;
#42262=CARTESIAN_POINT ( 'NONE',  ( 8.000000000000007105, 249.8719672152120381, 94.99999999999866418 ) ) ;
#42263=ORIENTED_EDGE ( 'NONE', *, *, #2529, .F. ) ;
#42265=CARTESIAN_POINT ( 'NONE',  ( 154.0401952541422474, 55.03227529428313147, 43.58305379128945134 ) ) ;
#42266=CARTESIAN_POINT ( 'NONE',  ( 103.5839822277949764, 25.92130892112108498, -39.96249046856183895 ) ) ;
#42267=CARTESIAN_POINT ( 'NONE',  ( 139.2794027252093940, 45.99190465195506050, -65.16434641514403836 ) ) ;
#42269=ORIENTED_EDGE ( 'NONE', *, *, #15732, .T. ) ;
#42271=CARTESIAN_POINT ( 'NONE',  ( -85.12122836439579032, 25.97531040437156946, -65.60879660851998096 ) ) ;
#42273=CARTESIAN_POINT ( 'NONE',  ( -121.5928001448268958, 44.91559452735374691, -36.25159717105308488 ) ) ;
#42274=CARTESIAN_POINT ( 'NONE',  ( -79.14638003838379632, 23.58242782405879012, 18.57365054920947856 ) ) ;
#42276=CARTESIAN_POINT ( 'NONE',  ( -155.5978531700837095, 69.52241200678679434, 15.76037129834827510 ) ) ;
#42278=CARTESIAN_POINT ( 'NONE',  ( 70.11438327604405174, 14.43198353181102256, 12.90143265241210280 ) ) ;
#42279=CARTESIAN_POINT ( 'NONE',  ( 164.8886903222557407, 63.65672212134880681, 8.925453984754252446 ) ) ;
#42282=VECTOR ( 'NONE', #52653, 1000.000000000000000 ) ;
#42284=DIRECTION ( 'NONE',  ( -0.8160245890732938934, -0.5780171883497599028, 0.000000000000000000 ) ) ;
#42285=ORIENTED_EDGE ( 'NONE', *, *, #1603, .T. ) ;
#42288=CARTESIAN_POINT ( 'NONE',  ( 23.28809538736928886, 7.864824219997537114, -69.37130277028362002 ) ) ;
#42293=CARTESIAN_POINT ( 'NONE',  ( 137.5911612413395630, 44.91497189902067078, -37.01495899583318305 ) ) ;
#42296=CARTESIAN_POINT ( 'NONE',  ( 152.1327777395850376, 53.61712543276775733, -38.34954180087900966 ) ) ;
#42307=EDGE_CURVE ( 'NONE', #37010, #25774, #55775, .T. ) ;
#42308=CARTESIAN_POINT ( 'NONE',  ( 87.58754341703159696, 20.81465688423119786, 17.82130253370978323 ) ) ;
#42310=CARTESIAN_POINT ( 'NONE',  ( 173.9413349464226997, 71.67637800842362594, -72.87454113658040455 ) ) ;
#42316=ADVANCED_FACE ( 'NONE', ( #4878 ), #47099, .F. ) ;
#42320=CARTESIAN_POINT ( 'NONE',  ( 110.2429982417149432, 28.88204397445231564, -9.077886975189997543 ) ) ;
#42321=EDGE_CURVE ( 'NONE', #28307, #61600, #50788, .T. ) ;
#42322=CARTESIAN_POINT ( 'NONE',  ( 151.7783534118502189, 54.60545177578661225, 68.64412217554496465 ) ) ;
#42325=CARTESIAN_POINT ( 'NONE',  ( -2.773325569976919702, 7.621740129702524236, 85.75189649308317996 ) ) ;
#42330=VECTOR ( 'NONE', #62638, 1000.000000000000000 ) ;
#42331=ORIENTED_EDGE ( 'NONE', *, *, #3444, .T. ) ;
#42332=CARTESIAN_POINT ( 'NONE',  ( 43.75276484590834514, 10.03191092760626724, 84.95856299007903090 ) ) ;
#42334=CARTESIAN_POINT ( 'NONE',  ( 139.3536337508564031, 46.03986978183306888, -92.09433734929739046 ) ) ;
#42335=EDGE_CURVE ( 'NONE', #49747, #61334, #66759, .T. ) ;
#42340=CARTESIAN_POINT ( 'NONE',  ( -0.3252226420479325530, 7.525368746738511305, 10.28429167359196583 ) ) ;
#42341=CARTESIAN_POINT ( 'NONE',  ( 176.6238742729555327, 75.60943990211370647, -49.77349832926806528 ) ) ;
#42342=VECTOR ( 'NONE', #23731, 1000.000000000000000 ) ;
#42347=CARTESIAN_POINT ( 'NONE',  ( 103.4725384926516938, 26.96797537091726582, -19.81430213386833472 ) ) ;
#42348=CYLINDRICAL_SURFACE ( 'NONE', #29185, 7.500000000000013323 ) ;
#42349=CARTESIAN_POINT ( 'NONE',  ( 13.36262230781615301, 7.441298897118795885, 44.62840908283959607 ) ) ;
#42350=CARTESIAN_POINT ( 'NONE',  ( 199.9103251464698872, 101.6434290204574751, 42.48563161778374564 ) ) ;
#42351=CARTESIAN_POINT ( 'NONE',  ( -84.79548387674154242, 25.84023516422310252, 87.27273205877571627 ) ) ;
#42356=CARTESIAN_POINT ( 'NONE',  ( 113.4418023215250457, 31.50656691678299026, -77.06712383350409823 ) ) ;
#42358=CARTESIAN_POINT ( 'NONE',  ( 198.7029050523552769, 98.46895521196213963, -66.13463292241958413 ) ) ;
#42360=CARTESIAN_POINT ( 'NONE',  ( -12.39770133248888939, 8.241491894828989473, -22.03905660758730889 ) ) ;
#42361=CARTESIAN_POINT ( 'NONE',  ( 152.8558173410470147, 54.14978343559394602, -64.53641076882379934 ) ) ;
#42363=DIRECTION ( 'NONE',  ( 0.000000000000000000, 0.000000000000000000, 1.000000000000000000 ) ) ;
#42366=CARTESIAN_POINT ( 'NONE',  ( 70.50376765786472788, 15.57629333413343353, -16.86642105671132086 ) ) ;
#42367=CARTESIAN_POINT ( 'NONE',  ( -81.89510452344295288, 24.66033552777455995, -49.40161435469455853 ) ) ;
#42368=CARTESIAN_POINT ( 'NONE',  ( 108.0836640549675991, 27.89549093408031766, 83.61057402085626222 ) ) ;
#42369=CARTESIAN_POINT ( 'NONE',  ( -155.7455325080991031, 71.01834415181987481, 15.54818467395414316 ) ) ;
#42370=EDGE_CURVE ( 'NONE', #32880, #36565, #21739, .T. ) ;
#42374=CARTESIAN_POINT ( 'NONE',  ( -156.5979701648280695, 71.80257276515639830, 94.37845108976992492 ) ) ;
#42378=AXIS2_PLACEMENT_3D ( 'NONE', #1641, #20761, #63679 ) ;
#42379=CARTESIAN_POINT ( 'NONE',  ( -149.5074843970971017, 65.50121172469319220, -22.96827994102830317 ) ) ;
#42380=CARTESIAN_POINT ( 'NONE',  ( 63.01563776193091826, 12.67277567978498176, 56.65751152968497451 ) ) ;
#42381=CARTESIAN_POINT ( 'NONE',  ( 104.3787150408505653, 26.26206731247476256, -92.41814093530493324 ) ) ;
#42384=CARTESIAN_POINT ( 'NONE',  ( 200.8383807319520997, 102.8517715783673339, 57.10714352580840369 ) ) ;
#42387=CARTESIAN_POINT ( 'NONE',  ( 181.0840389613909736, 80.03940679743415387, 71.15314469597512925 ) ) ;
#42388=CARTESIAN_POINT ( 'NONE',  ( 46.89128214611609735, 9.502158095527986958, 91.88262892997218501 ) ) ;
#42391=CARTESIAN_POINT ( 'NONE',  ( 188.2988323915788271, 86.21831227955483712, 65.72281026858398434 ) ) ;
#42393=CARTESIAN_POINT ( 'NONE',  ( -85.90441187606238316, 25.21188850826090899, -40.58563879895491766 ) ) ;
#42394=CARTESIAN_POINT ( 'NONE',  ( 21.42484406671928099, 6.746536496442160136, 59.40547109256082337 ) ) ;
#42396=CARTESIAN_POINT ( 'NONE',  ( 8.683910719548894264, 7.383368463746304400, 8.253806082366962116 ) ) ;
#42400=CARTESIAN_POINT ( 'NONE',  ( 186.2651679807462415, 84.00458780104318635, 4.520801913443380116 ) ) ;
#42404=CARTESIAN_POINT ( 'NONE',  ( -156.9402586331177361, 72.11962769956262775, -95.00000000000133582 ) ) ;
#42406=CARTESIAN_POINT ( 'NONE',  ( 181.0840389613909736, 80.03940679743416808, -51.22505766587963905 ) ) ;
#42407=ORIENTED_EDGE ( 'NONE', *, *, #3318, .T. ) ;
#42410=CARTESIAN_POINT ( 'NONE',  ( 203.9203998321607116, 106.9845510704142413, 17.33319198133153805 ) ) ;
#42416=DIRECTION ( 'NONE',  ( -0.8118923937861950435, -0.5838071093367415143, 0.000000000000000000 ) ) ;
#42419=CARTESIAN_POINT ( 'NONE',  ( -96.76159256735192571, 30.06445763698411255, 43.12167622908535236 ) ) ;
#42420=CARTESIAN_POINT ( 'NONE',  ( 93.85846834761630930, 22.01563781856521018, -45.33479466209353603 ) ) ;
#42422=EDGE_LOOP ( 'NONE', ( #12249, #58786, #21896, #14851 ) ) ;
#42423=VECTOR ( 'NONE', #67103, 1000.000000000000000 ) ;
#42426=CARTESIAN_POINT ( 'NONE',  ( -167.6524579626395166, 82.69702609844094354, 6.338703478976664307 ) ) ;
#42428=CARTESIAN_POINT ( 'NONE',  ( -179.0654441437004323, 93.99779465816534696, -19.94754107494070183 ) ) ;
#42431=CARTESIAN_POINT ( 'NONE',  ( -142.3178993725748853, 58.31327888234797285, -40.10431696157230874 ) ) ;
#42433=CARTESIAN_POINT ( 'NONE',  ( -109.5517607553961739, 37.78054172120042153, 89.84167037464601435 ) ) ;
#42436=CARTESIAN_POINT ( 'NONE',  ( -133.0808647576834005, 51.41195281028756625, 40.28004429727871383 ) ) ;
#42441=CARTESIAN_POINT ( 'NONE',  ( -101.8145602049406051, 32.54453702486151201, 18.67452391595144334 ) ) ;
#42442=CARTESIAN_POINT ( 'NONE',  ( -94.89192151156326815, 29.18342430963125977, -70.67526850584850706 ) ) ;
#42445=CARTESIAN_POINT ( 'NONE',  ( 185.5415406465189676, 83.23025870924408309, -76.61970377424405854 ) ) ;
#42446=CARTESIAN_POINT ( 'NONE',  ( -169.8791831685529985, 83.59058982490282119, -35.43423335292201415 ) ) ;
#42448=CARTESIAN_POINT ( 'NONE',  ( 105.4376736768159191, 27.81988511842611800, -76.03054162972082963 ) ) ;
#42449=CARTESIAN_POINT ( 'NONE',  ( -72.21889834709583056, 21.03534256744171316, 41.78139917607329323 ) ) ;
#42451=CARTESIAN_POINT ( 'NONE',  ( 82.94943325692331371, 18.19803534719805782, 30.67239719205550941 ) ) ;
#42453=CARTESIAN_POINT ( 'NONE',  ( 41.09759788073308329, 9.651672055033845510, -35.80995810388947120 ) ) ;
#42454=CARTESIAN_POINT ( 'NONE',  ( 207.4867844023104624, 110.2451255333963331, 70.52645239145388700 ) ) ;
#42457=ORIENTED_EDGE ( 'NONE', *, *, #47179, .F. ) ;
#42459=CARTESIAN_POINT ( 'NONE',  ( -37.07602570886410831, 10.58457435034603478, 5.899994561324445108 ) ) ;
#42461=CARTESIAN_POINT ( 'NONE',  ( 89.65730223173024172, 21.54473673261223254, 57.19084295439972720 ) ) ;
#42462=CARTESIAN_POINT ( 'NONE',  ( 133.8566784816069344, 42.60093787723652525, 29.51034083899533300 ) ) ;
#42464=CARTESIAN_POINT ( 'NONE',  ( 33.75639351246965703, 7.742023566824297376, -74.92653034813449153 ) ) ;
#42466=CARTESIAN_POINT ( 'NONE',  ( -35.17296606710972640, 11.25626711331309515, -22.49574526638046024 ) ) ;
#42467=ORIENTED_EDGE ( 'NONE', *, *, #62022, .F. ) ;
#42470=CARTESIAN_POINT ( 'NONE',  ( -7.825402957745087207, -170.0000000000000000, -42.91807073194382838 ) ) ;
#42471=CARTESIAN_POINT ( 'NONE',  ( 12.04188192036245653, 7.416006018508749520, -76.36538918330802517 ) ) ;
#42472=CARTESIAN_POINT ( 'NONE',  ( -190.6985136298601731, 109.1272424661242582, 7.126870892829554549 ) ) ;
#42474=CARTESIAN_POINT ( 'NONE',  ( 8.000000000000007105, 249.8719672152120381, -95.00000000000133582 ) ) ;
#42475=CARTESIAN_POINT ( 'NONE',  ( -2.866724795119724778, 6.618578306599219196, 43.26370662482394636 ) ) ;
#42476=CARTESIAN_POINT ( 'NONE',  ( -95.05546640093037070, 29.25972325950975517, -17.74977852771992204 ) ) ;
#42479=CARTESIAN_POINT ( 'NONE',  ( 157.0357419681844249, 58.58786672900117765, -51.11478325206026341 ) ) ;
#42484=ADVANCED_FACE ( 'NONE', ( #67122 ), #2388, .F. ) ;
#42486=CARTESIAN_POINT ( 'NONE',  ( 177.0027897064244939, 75.97676392242547649, -10.57201763481611856 ) ) ;
#42488=CARTESIAN_POINT ( 'NONE',  ( -109.4995148930278361, 37.75156937139181679, 62.76486868760267157 ) ) ;
#42493=CARTESIAN_POINT ( 'NONE',  ( -4.955782654901483397, 6.720825733572408645, -23.01568829693101392 ) ) ;
#42494=CARTESIAN_POINT ( 'NONE',  ( 197.3700262219431067, 98.41176242030789467, -15.35159226254784315 ) ) ;
#42495=CARTESIAN_POINT ( 'NONE',  ( -142.3798905661107028, 58.36196886944601658, 89.55050332779295275 ) ) ;
#42496=AXIS2_PLACEMENT_3D ( 'NONE', #29238, #33485, #44723 ) ;
#42499=ORIENTED_EDGE ( 'NONE', *, *, #31873, .T. ) ;
#42501=CARTESIAN_POINT ( 'NONE',  ( 79.39764314491569053, 18.13166883367087223, 8.363466887744241518 ) ) ;
#42502=CARTESIAN_POINT ( 'NONE',  ( 163.7403496014744633, 64.00600007368875310, 5.941244934767215824 ) ) ;
#42503=CARTESIAN_POINT ( 'NONE',  ( -98.68609963468200874, 32.11186931716880366, 44.61905611811087624 ) ) ;
#42504=ADVANCED_FACE ( 'NONE', ( #40014 ), #61477, .F. ) ;
#42505=EDGE_CURVE ( 'NONE', #5910, #66136, #30609, .T. ) ;
#42507=VERTEX_POINT ( 'NONE', #35788 ) ;
#42512=CARTESIAN_POINT ( 'NONE',  ( 70.11766033381769603, 14.43277633974327046, -72.52602136616579287 ) ) ;
#42514=CARTESIAN_POINT ( 'NONE',  ( 152.8373718734504791, 55.38925997611394081, 15.98291334453402079 ) ) ;
#42515=ORIENTED_EDGE ( 'NONE', *, *, #22416, .T. ) ;
#42516=CARTESIAN_POINT ( 'NONE',  ( -179.5082312244189495, 94.53075638132058600, 34.38164526738366789 ) ) ;
#42518=CARTESIAN_POINT ( 'NONE',  ( -71.28077210551055032, -170.0000000000000000, -95.00000000000133582 ) ) ;
#42519=ORIENTED_EDGE ( 'NONE', *, *, #39014, .T. ) ;
#42521=CARTESIAN_POINT ( 'NONE',  ( 141.3445468829084746, 46.13338528906590597, 64.35867967590782257 ) ) ;
#42523=CARTESIAN_POINT ( 'NONE',  ( -32.41982179707238032, 9.753975577087194537, -77.11329407010529735 ) ) ;
#42524=CARTESIAN_POINT ( 'NONE',  ( 93.87650740736113164, 23.09802612281734113, 35.21570653740766943 ) ) ;
#42527=CARTESIAN_POINT ( 'NONE',  ( 45.04506994399700659, 10.22854084020123722, 5.604377804579494082 ) ) ;
#42532=CARTESIAN_POINT ( 'NONE',  ( 211.3710169359753763, 117.8057917113659556, -20.41562570395084109 ) ) ;
#42534=CARTESIAN_POINT ( 'NONE',  ( -156.0300823189602113, 69.91528270335479078, -72.89804073699036735 ) ) ;
#42535=CARTESIAN_POINT ( 'NONE',  ( -109.1218018794893538, 36.39436146239677328, 88.61840892032539330 ) ) ;
#42536=CARTESIAN_POINT ( 'NONE',  ( 186.2575601542430377, 85.47765906955507376, 15.39943919417170370 ) ) ;
#42543=CARTESIAN_POINT ( 'NONE',  ( -78.66644367742111399, 23.39876645725286863, 72.26275173013684139 ) ) ;
#42544=CARTESIAN_POINT ( 'NONE',  ( 205.5105258529712557, 107.4632495673648265, -63.20359001240491637 ) ) ;
#42545=CARTESIAN_POINT ( 'NONE',  ( 62.04664474957771603, 12.44961624115901877, -62.61246026202184112 ) ) ;
#42547=CARTESIAN_POINT ( 'NONE',  ( -36.80780718687457664, 10.53430034069837440, -91.25189668311308822 ) ) ;
#42548=CARTESIAN_POINT ( 'NONE',  ( 22.72762730455395896, 7.830015919864530716, 40.39119682621441854 ) ) ;
#42549=CARTESIAN_POINT ( 'NONE',  ( 197.8107221832102312, 97.35272301387820448, 87.39809707970657371 ) ) ;
#42550=CARTESIAN_POINT ( 'NONE',  ( 157.4703587214989113, 58.92748579479259519, -62.96873488960130771 ) ) ;
#42552=CARTESIAN_POINT ( 'NONE',  ( -71.56718866013697777, 19.74312628447963647, 67.23400750481188481 ) ) ;
#42557=ADVANCED_FACE ( 'NONE', ( #42087 ), #10413, .F. ) ;
#42565=EDGE_CURVE ( 'NONE', #56347, #22683, #68480, .T. ) ;
#42567=ORIENTED_EDGE ( 'NONE', *, *, #44221, .F. ) ;
#42568=CARTESIAN_POINT ( 'NONE',  ( -128.3448054685827913, 49.34430406923179646, 31.02807967144357804 ) ) ;
#42569=EDGE_LOOP ( 'NONE', ( #52218, #47774 ) ) ;
#42572=CARTESIAN_POINT ( 'NONE',  ( 57.39674746172462960, 11.43903079040059190, 69.14934571406377017 ) ) ;
#42577=AXIS2_PLACEMENT_3D ( 'NONE', #63203, #36465, #40442 ) ;
#42581=CARTESIAN_POINT ( 'NONE',  ( -165.6393662153604396, 79.16886183052815795, -14.76170845779348539 ) ) ;
#42582=CARTESIAN_POINT ( 'NONE',  ( 136.1081004736419402, 42.80058051492065374, -77.52565627643819823 ) ) ;
#42583=CARTESIAN_POINT ( 'NONE',  ( 66.72974708835177182, 13.56459745268607087, 30.77864159763544549 ) ) ;
#42584=EDGE_CURVE ( 'NONE', #34225, #63173, #54116, .T. ) ;
#42585=CARTESIAN_POINT ( 'NONE',  ( -189.5329886872043517, 107.4958891766011106, -71.08704754913541990 ) ) ;
#42590=EDGE_CURVE ( 'NONE', #48880, #39196, #33280, .T. ) ;
#42591=CARTESIAN_POINT ( 'NONE',  ( 202.7506655727289058, 105.3943386412348673, -36.57149851176358624 ) ) ;
#42596=CARTESIAN_POINT ( 'NONE',  ( -119.9771613955297198, 43.90337778233482879, 6.659436444873731098 ) ) ;
#42597=CARTESIAN_POINT ( 'NONE',  ( -180.0175713311536470, 95.14770835574077523, 62.20439195989532521 ) ) ;
#42598=CARTESIAN_POINT ( 'NONE',  ( 126.8015497489690091, 37.32461426945040728, 61.29668405129906716 ) ) ;
#42601=CARTESIAN_POINT ( 'NONE',  ( 150.0501577908836168, 52.10460126680126791, 38.03534073332230747 ) ) ;
#42605=CARTESIAN_POINT ( 'NONE',  ( -24.18258876560172865, 8.512344710720677554, 35.75813012041879091 ) ) ;
#42607=EDGE_LOOP ( 'NONE', ( #46202, #9602, #20787, #40642 ) ) ;
#42608=VECTOR ( 'NONE', #31214, 1000.000000000000000 ) ;
#42609=FACE_BOUND ( 'NONE', #61488, .T. ) ;
#42613=CARTESIAN_POINT ( 'NONE',  ( -119.6801029354224823, 43.71909921132880328, -46.62127720739779591 ) ) ;
#42614=CARTESIAN_POINT ( 'NONE',  ( -86.11230725916327344, 26.39026888680166749, 10.03994749107184070 ) ) ;
#42617=CARTESIAN_POINT ( 'NONE',  ( 197.7943621856794891, 98.94371996881450571, 93.35786775789816261 ) ) ;
#42618=CARTESIAN_POINT ( 'NONE',  ( 65.41496713438827726, 13.24164235279043922, 17.59071151666574195 ) ) ;
#42620=CARTESIAN_POINT ( 'NONE',  ( 87.10672734544985474, 20.64813880796637235, -23.97701360844805762 ) ) ;
#42622=EDGE_CURVE ( 'NONE', #5387, #59334, #33049, .T. ) ;
#42627=CARTESIAN_POINT ( 'NONE',  ( 22.28556289340100349, 7.803548444155008035, -73.61795775605594372 ) ) ;
#42629=CARTESIAN_POINT ( 'NONE',  ( -143.8634661037140745, 60.82480701605700091, 60.09994342671955536 ) ) ;
#42630=CARTESIAN_POINT ( 'NONE',  ( 69.50572373348801136, 14.27208627753790537, -12.58521233645258874 ) ) ;
#42632=CARTESIAN_POINT ( 'NONE',  ( 139.6150621148398727, 46.20856238844175579, -38.69201805759518464 ) ) ;
#42633=CARTESIAN_POINT ( 'NONE',  ( 211.3689821960821291, 117.8027529136708296, -94.07932131241392426 ) ) ;
#42635=CARTESIAN_POINT ( 'NONE',  ( -121.2119672714299838, 44.67540322905997385, -9.689954091359160415 ) ) ;
#42637=ORIENTED_EDGE ( 'NONE', *, *, #4822, .T. ) ;
#42638=EDGE_CURVE ( 'NONE', #61969, #45785, #44148, .T. ) ;
#42639=CARTESIAN_POINT ( 'NONE',  ( 69.73342236697681074, 14.33173522011653134, -46.59197138149946937 ) ) ;
#42640=DIRECTION ( 'NONE',  ( 0.000000000000000000, 0.000000000000000000, 1.000000000000000000 ) ) ;
#42646=CARTESIAN_POINT ( 'NONE',  ( 65.60421405224433045, 14.32371900106614149, -89.86771203546919651 ) ) ;
#42647=ADVANCED_FACE ( 'NONE', ( #11107 ), #32570, .F. ) ;
#42649=CARTESIAN_POINT ( 'NONE',  ( 188.2950976467626560, 87.71503060978557187, -14.79773892726507611 ) ) ;
#42650=CARTESIAN_POINT ( 'NONE',  ( 208.5936709733499015, 113.6229123546138453, 3.440378187112652419 ) ) ;
#42651=CARTESIAN_POINT ( 'NONE',  ( -85.53181628782058965, 26.14670395349505583, -93.27685199465567223 ) ) ;
#42652=CARTESIAN_POINT ( 'NONE',  ( 44.35071890818840501, 9.104600422692255890, -10.61849397789796967 ) ) ;
#42653=CARTESIAN_POINT ( 'NONE',  ( -31.43908319763709969, 10.61114334766715928, 57.06100499665286208 ) ) ;
#42655=CARTESIAN_POINT ( 'NONE',  ( 161.1112535418156426, 61.83422628788728304, 70.31501105061632018 ) ) ;
#42659=CARTESIAN_POINT ( 'NONE',  ( 94.11733320392094981, 23.18939451097131865, -43.81524227077105138 ) ) ;
#42662=CARTESIAN_POINT ( 'NONE',  ( 150.5550643769628323, 52.46819381604269239, 7.149426911769203308 ) ) ;
#42664=CARTESIAN_POINT ( 'NONE',  ( -14.92342969503865469, 8.468308978091254602, 93.81261129068334981 ) ) ;
#42665=ORIENTED_EDGE ( 'NONE', *, *, #41286, .F. ) ;
#42668=CARTESIAN_POINT ( 'NONE',  ( -62.53989795537026453, 16.81768094534200131, 65.16712804106848012 ) ) ;
#42671=CARTESIAN_POINT ( 'NONE',  ( 35.07875163271969399, 8.898953321987049137, 84.96543998221538629 ) ) ;
#42673=CARTESIAN_POINT ( 'NONE',  ( 8.000000000000007105, 249.8719672152120381, -95.00000000000133582 ) ) ;
#42676=CARTESIAN_POINT ( 'NONE',  ( -0.7211439451572434489, 7.539282923622933730, 13.18759299316698552 ) ) ;
#42677=CARTESIAN_POINT ( 'NONE',  ( 177.7886308167536242, 76.74396398590877766, -36.97273068449148781 ) ) ;
#42680=CARTESIAN_POINT ( 'NONE',  ( 89.21005684773504640, 20.31770592753387206, 30.16603058232306367 ) ) ;
#42681=ORIENTED_EDGE ( 'NONE', *, *, #12, .T. ) ;
#42684=CARTESIAN_POINT ( 'NONE',  ( 10.31616749326173732, 7.393414706728907326, 32.37994498868797422 ) ) ;
#42685=CARTESIAN_POINT ( 'NONE',  ( 199.7291770695760533, 101.4092159658447372, 42.33109527906247394 ) ) ;
#42686=CARTESIAN_POINT ( 'NONE',  ( -86.17314828412035865, 26.41592763503389207, 91.53058199398142847 ) ) ;
#42688=ORIENTED_EDGE ( 'NONE', *, *, #14696, .F. ) ;
#42689=VERTEX_POINT ( 'NONE', #13213 ) ;
#42692=ORIENTED_EDGE ( 'NONE', *, *, #47258, .F. ) ;
#42693=CARTESIAN_POINT ( 'NONE',  ( 117.4806398654733783, 33.50379325299403632, -72.30120517819882764 ) ) ;
#42696=CARTESIAN_POINT ( 'NONE',  ( -37.05762690088739930, 11.60527003175540806, 59.58680104041130221 ) ) ;
#42697=EDGE_CURVE ( 'NONE', #47148, #22089, #47410, .T. ) ;
#42698=CARTESIAN_POINT ( 'NONE',  ( -15.27594996066617661, 8.502079791899639361, -17.06292143071024725 ) ) ;
#42704=VERTEX_POINT ( 'NONE', #8280 ) ;
#42705=CARTESIAN_POINT ( 'NONE',  ( 69.72789637502502558, 15.37065610545704075, -19.73133222002547171 ) ) ;
#42708=CARTESIAN_POINT ( 'NONE',  ( -24.54245881417235609, 9.575750052011494873, 94.42483238541157675 ) ) ;
#42709=CARTESIAN_POINT ( 'NONE',  ( -150.3831389294225573, 66.25266777263976792, 3.924350373141658466 ) ) ;
#42714=ORIENTED_EDGE ( 'NONE', *, *, #48872, .F. ) ;
#42717=CARTESIAN_POINT ( 'NONE',  ( 34.45158752686798209, 8.829194381142000836, -37.46439019260278513 ) ) ;
#42719=ADVANCED_FACE ( 'NONE', ( #35707 ), #30418, .F. ) ;
#42720=CARTESIAN_POINT ( 'NONE',  ( -38.87848244732138880, 10.93141945332449794, 63.57758875895522266 ) ) ;
#42721=CARTESIAN_POINT ( 'NONE',  ( 199.7286177451875915, 101.4075663537892211, 57.91560235614644370 ) ) ;
#42723=VERTEX_POINT ( 'NONE', #57158 ) ;
#42724=B_SPLINE_CURVE_WITH_KNOTS ( 'NONE', 3,
 ( #38071, #69394, #59866, #26832, #16270, #5709, #48260, #47924, #65160, #16614, #88, #49308, #21541, #21888, #21214, #65514, #33155, #43341, #59513, #42988, #54231, #64813, #11683, #42659, #16953, #64460, #54592, #6416, #53886, #27869, #1140, #22591, #44031, #17311, #38781, #19052, #18359, #44390, #61952, #29265, #60574, #56004, #60919, #28568, #61272 ),
 .UNSPECIFIED., .F., .F.,
 ( 4, 2, 2, 2, 2, 2, 2, 2, 2, 2, 2, 1, 2, 2, 2, 2, 2, 2, 2, 2, 2, 2, 4 ),
 ( 0.000000000000000000, 0.001510509505236005533, 0.002265764257853987700, 0.003021019010471969433, 0.004531528515707886930, 0.005286783268325868229, 0.006042038020943850396, 0.007552547526179788709, 0.009063057031415727022, 0.01057356653665166533, 0.01132882128926963536, 0.01208407604188760538, 0.01283933079450557367, 0.01359458554712354196, 0.01510509505235946466, 0.01586034980497742428, 0.01661560455759538563, 0.01812611406283129445, 0.01963662356806720327, 0.02039187832068514034, 0.02114713307330307393, 0.02265764257853898622, 0.02416815208377489851 ),
 .UNSPECIFIED. ) ;
#42725=CARTESIAN_POINT ( 'NONE',  ( 175.0857681883884140, 72.74906374897946648, 94.99999999999866418 ) ) ;
#42726=CARTESIAN_POINT ( 'NONE',  ( -156.9406434201983984, 70.74968524571474404, 66.21526506586671701 ) ) ;
#42727=CARTESIAN_POINT ( 'NONE',  ( 19.11382977197791888, 7.636807742668408672, 17.41050504540015353 ) ) ;
#42728=CARTESIAN_POINT ( 'NONE',  ( 182.7789203043890041, 80.33475476315294372, 70.97149666712105898 ) ) ;
#42730=CARTESIAN_POINT ( 'NONE',  ( -86.06489347855098515, 25.27905598459107139, -43.87173148075923734 ) ) ;
#42731=CARTESIAN_POINT ( 'NONE',  ( 19.10216788411013411, 6.629360741291161929, 57.62663534263347032 ) ) ;
#42733=CARTESIAN_POINT ( 'NONE',  ( 8.540853903193189822, 6.376814430361480213, -67.91796824995262227 ) ) ;
#42735=CARTESIAN_POINT ( 'NONE',  ( 187.8959968237854241, 85.77553094678179946, 6.814269787780084187 ) ) ;
#42737=CARTESIAN_POINT ( 'NONE',  ( 177.0075766083211875, 74.58167636505950782, 30.50888549528974281 ) ) ;
#42738=CARTESIAN_POINT ( 'NONE',  ( -149.5074843970971301, -170.0000000000000000, 45.72082123989907387 ) ) ;
#42739=CARTESIAN_POINT ( 'NONE',  ( 41.33692564073606235, 8.668977654195476390, -77.21459316755360192 ) ) ;
#42743=CARTESIAN_POINT ( 'NONE',  ( -25.50312845906833914, 8.692070753302656883, -20.56343087316415819 ) ) ;
#42744=CARTESIAN_POINT ( 'NONE',  ( 204.6977192012829789, 108.0580384837234931, 17.36317014830577321 ) ) ;
#42745=EDGE_LOOP ( 'NONE', ( #20106, #15973 ) ) ;
#42746=B_SPLINE_CURVE_WITH_KNOTS ( 'NONE', 3,
 ( #13237, #7951, #49096, #39613, #60007, #17092, #935, #22383, #1628, #33304, #22738, #38926, #23093, #44540, #66022, #12532, #55432, #7263, #50165, #61064, #13572, #36068, #13915, #14605, #61749, #14948, #30793, #24136, #3369, #46262, #36411, #67739, #29749, #56838, #57867, #29404, #4062, #57179, #51212, #68425, #63146, #3024, #57525, #62099 ),
 .UNSPECIFIED., .F., .F.,
 ( 4, 2, 2, 2, 2, 2, 2, 2, 2, 2, 2, 2, 2, 2, 2, 2, 2, 2, 2, 2, 2, 4 ),
 ( 0.02638217555535140105, 0.02805347641364870290, 0.02972477727194600128, 0.03139607813024330313, 0.03306737898854060498, 0.03390302941768924549, 0.03473867984683789295, 0.03640998070513518092, 0.03724563113428379368, 0.03808128156343241338, 0.03891693199258103308, 0.03975258242172964585, 0.04058823285087826555, 0.04142388328002688525, 0.04225953370917549801, 0.04309518413832411771, 0.04476648499662130853, 0.04643778585491847855, 0.04810908671321565550, 0.04978038757151283245, 0.05145168842981000246, 0.05312298928810717941 ),
 .UNSPECIFIED. ) ;
#42748=CARTESIAN_POINT ( 'NONE',  ( 114.4640969196986191, 30.88424258798506372, 57.75175038263319038 ) ) ;
#42751=CARTESIAN_POINT ( 'NONE',  ( 140.5958192060901126, 46.84598876498520781, 60.55316104302657720 ) ) ;
#42754=CARTESIAN_POINT ( 'NONE',  ( 83.90793350743913948, 18.51008205890721214, -90.01042505155271556 ) ) ;
#42759=CARTESIAN_POINT ( 'NONE',  ( -169.1122507277983402, 84.24359299875008844, 5.123006575244060556 ) ) ;
#42761=CARTESIAN_POINT ( 'NONE',  ( -178.5790738944853331, 93.41591512785083751, -10.21774767167227616 ) ) ;
#42763=CARTESIAN_POINT ( 'NONE',  ( -142.3393481102175429, 58.33014244976926932, -44.53616841364604539 ) ) ;
#42765=DIRECTION ( 'NONE',  ( -0.000000000000000000, 1.000000000000000000, -0.000000000000000000 ) ) ;
#42770=CARTESIAN_POINT ( 'NONE',  ( 82.13067365723603075, 17.93447087949265395, -22.49758088646247600 ) ) ;
#42771=CARTESIAN_POINT ( 'NONE',  ( 134.7708899521910837, 43.15864772107690328, 29.56272650432242699 ) ) ;
#42772=CARTESIAN_POINT ( 'NONE',  ( 56.35108009888376301, 11.22498869437516866, -93.44476644971953760 ) ) ;
#42774=CARTESIAN_POINT ( 'NONE',  ( -94.89192151156323973, 29.18342430963126688, 9.858383265542547846 ) ) ;
#42775=CARTESIAN_POINT ( 'NONE',  ( -94.85061234775062644, 29.16417548023187578, -70.41713452772432902 ) ) ;
#42776=ORIENTED_EDGE ( 'NONE', *, *, #27605, .T. ) ;
#42779=CYLINDRICAL_SURFACE ( 'NONE', #67532, 7.500000000000020428 ) ;
#42781=CARTESIAN_POINT ( 'NONE',  ( -166.7068579965637127, 80.26142964949322334, -46.10773525000625739 ) ) ;
#42783=CARTESIAN_POINT ( 'NONE',  ( -71.42007367207962432, 20.75704712149297748, 35.91863450065896046 ) ) ;
#42784=CARTESIAN_POINT ( 'NONE',  ( 79.82127737190243977, 17.20935440217364487, 34.05564977191748000 ) ) ;
#42786=CARTESIAN_POINT ( 'NONE',  ( -121.5680658099884113, 44.89994870382101055, 31.97482362736482031 ) ) ;
#42787=CARTESIAN_POINT ( 'NONE',  ( 209.6877167158271220, 113.4449353909247691, 69.15631450432505289 ) ) ;
#42788=ORIENTED_EDGE ( 'NONE', *, *, #36037, .F. ) ;
#42789=CARTESIAN_POINT ( 'NONE',  ( -105.4556185321791588, 34.42302275449794990, -8.858947522874947467 ) ) ;
#42793=CARTESIAN_POINT ( 'NONE',  ( -86.10037789697233279, 25.29391845275002737, 90.56095318331921362 ) ) ;
#42794=CARTESIAN_POINT ( 'NONE',  ( 86.62931800182293784, 20.48449268398423229, 56.55663816294300261 ) ) ;
#42796=CARTESIAN_POINT ( 'NONE',  ( 156.5909039492009640, 56.96742803863246252, -9.279633708673955539 ) ) ;
#42797=CARTESIAN_POINT ( 'NONE',  ( 32.15613847490628530, 8.588587416860168133, 8.617515965834311231 ) ) ;
#42798=CARTESIAN_POINT ( 'NONE',  ( 32.67604596315971577, 7.629767358313821468, -73.29199647863042344 ) ) ;
#42799=CARTESIAN_POINT ( 'NONE',  ( -97.88021438939452423, 31.71889184683102059, -63.26670929094522933 ) ) ;
#42800=AXIS2_PLACEMENT_3D ( 'NONE', #16310, #49693, #54631 ) ;
#42804=ORIENTED_EDGE ( 'NONE', *, *, #25098, .F. ) ;
#42806=CARTESIAN_POINT ( 'NONE',  ( 8.480977594057447888, 7.382886909400594888, -71.57027735648773614 ) ) ;
#42808=CYLINDRICAL_SURFACE ( 'NONE', #24374, 7.500000000000013323 ) ;
#42809=CARTESIAN_POINT ( 'NONE',  ( -4.513903087372268530, 6.697902023160576590, 30.88178378492203890 ) ) ;
#42810=CARTESIAN_POINT ( 'NONE',  ( -95.52163045714287648, 29.47808868198296040, -18.93148129228250554 ) ) ;
#42811=CARTESIAN_POINT ( 'NONE',  ( 79.17772719511384594, 18.06403411472781428, 91.81807103218608290 ) ) ;
#42813=ORIENTED_EDGE ( 'NONE', *, *, #28421, .F. ) ;
#42816=CARTESIAN_POINT ( 'NONE',  ( -133.0808647576833721, 51.41195281028755915, 13.43549370681501109 ) ) ;
#42817=CARTESIAN_POINT ( 'NONE',  ( -108.9145525555662317, 37.42858360505775295, 61.35666273033913143 ) ) ;
#42821=CARTESIAN_POINT ( 'NONE',  ( 91.13361825170463248, 21.00701373666981553, 70.07319469683858415 ) ) ;
#42822=CARTESIAN_POINT ( 'NONE',  ( 197.9843579228224542, 99.18296459057400227, -13.62550849792877727 ) ) ;
#42823=CARTESIAN_POINT ( 'NONE',  ( -156.6452887561481191, 70.47820714639399853, 89.58194124164906214 ) ) ;
#42827=CARTESIAN_POINT ( 'NONE',  ( 79.13041963748372609, 18.04952109592810316, 9.847327292909767493 ) ) ;
#42828=CARTESIAN_POINT ( 'NONE',  ( 164.9547823171480161, 65.03046442419433504, 9.505235400904521015 ) ) ;
#42837=CARTESIAN_POINT ( 'NONE',  ( -107.0751323097254755, 35.28386110859232616, -48.30244191324285197 ) ) ;
#42838=CARTESIAN_POINT ( 'NONE',  ( 68.61679388097590504, 14.04192738700837673, -75.05900237351899307 ) ) ;
#42840=CARTESIAN_POINT ( 'NONE',  ( 149.9883446984744637, 53.30011109831375649, 9.477168676321245044 ) ) ;
#42842=CARTESIAN_POINT ( 'NONE',  ( -175.1920326508032986, 89.46239303019291356, 31.10066421722925867 ) ) ;
#42845=CARTESIAN_POINT ( 'NONE',  ( 117.3246714514015849, 33.42485879931865611, -45.94399363046861140 ) ) ;
#42848=EDGE_CURVE ( 'NONE', #66081, #12944, #52404, .T. ) ;
#42849=EDGE_CURVE ( 'NONE', #9033, #3775, #27451, .T. ) ;
#42852=CARTESIAN_POINT ( 'NONE',  ( 126.3732561463888118, 38.23795180971326602, 63.29033028859080900 ) ) ;
#42857=CARTESIAN_POINT ( 'NONE',  ( 204.6977192012829789, -170.0000000000000000, 71.05227132923315025 ) ) ;
#42861=CARTESIAN_POINT ( 'NONE',  ( 67.87214640187850989, 13.85168242453936216, 85.27733058027321533 ) ) ;
#42863=CARTESIAN_POINT ( 'NONE',  ( -132.4819073909166320, 50.98736898418875541, 68.58703093612896851 ) ) ;
#42864=DIRECTION ( 'NONE',  ( 0.000000000000000000, 0.000000000000000000, 1.000000000000000000 ) ) ;
#42866=CARTESIAN_POINT ( 'NONE',  ( -96.89873354725229149, 31.24547541778401794, -90.96072102636905754 ) ) ;
#42868=CARTESIAN_POINT ( 'NONE',  ( -71.17846906053300415, 20.67346400882179935, 64.26825347421748802 ) ) ;
#42869=CARTESIAN_POINT ( 'NONE',  ( 212.0180052085438263, 116.9552462415715013, -69.00676071747216156 ) ) ;
#42870=EDGE_CURVE ( 'NONE', #42507, #52659, #2089, .T. ) ;
#42873=CARTESIAN_POINT ( 'NONE',  ( -34.73655621045444519, 10.15566554627628371, -89.75670392811869647 ) ) ;
#42878=EDGE_CURVE ( 'NONE', #44611, #34598, #40689, .T. ) ;
#42879=CARTESIAN_POINT ( 'NONE',  ( 164.4760519199595592, 64.62478832434436526, -67.73851987524837170 ) ) ;
#42881=AXIS2_PLACEMENT_3D ( 'NONE', #16475, #33366, #37582 ) ;
#42883=CARTESIAN_POINT ( 'NONE',  ( 8.000000000000007105, 249.8719672152120381, -95.00000000000133582 ) ) ;
#42886=CARTESIAN_POINT ( 'NONE',  ( -28.13128612339710344, 10.08889185338653327, -62.91279178769815417 ) ) ;
#42887=CARTESIAN_POINT ( 'NONE',  ( 56.66438910147189034, 11.28870326331392704, -47.21719651937512197 ) ) ;
#42891=VECTOR ( 'NONE', #20366, 1000.000000000000000 ) ;
#42892=ORIENTED_EDGE ( 'NONE', *, *, #65928, .F. ) ;
#42895=CARTESIAN_POINT ( 'NONE',  ( -126.7944042662569046, 48.29830493043729689, 30.66038275586655359 ) ) ;
#42898=CARTESIAN_POINT ( 'NONE',  ( 187.1539087446606118, 86.45467532021284285, -92.98937004433818743 ) ) ;
#42899=CARTESIAN_POINT ( 'NONE',  ( 59.29597493004737174, 11.84030339376940510, 70.68833123368655436 ) ) ;
#42903=CYLINDRICAL_SURFACE ( 'NONE', #9904, 7.500000000000013323 ) ;
#42905=ORIENTED_EDGE ( 'NONE', *, *, #64505, .T. ) ;
#42911=CARTESIAN_POINT ( 'NONE',  ( 19.83783859368179492, 7.671370827793382752, 84.88257075276666797 ) ) ;
#42913=ADVANCED_FACE ( 'NONE', ( #24980 ), #56280, .T. ) ;
#42914=FACE_OUTER_BOUND ( 'NONE', #7500, .T. ) ;
#42916=CARTESIAN_POINT ( 'NONE',  ( -71.96390573417173186, 19.88067451234326199, 41.32151012117945754 ) ) ;
#42921=CARTESIAN_POINT ( 'NONE',  ( 14.80205238535217127, 6.470775952815777998, -50.46994021608795578 ) ) ;
#42922=CARTESIAN_POINT ( 'NONE',  ( -178.7483298110140311, 93.61800926271537548, 60.20166031997415956 ) ) ;
#42923=CARTESIAN_POINT ( 'NONE',  ( 18.21423326326597802, 6.590134686181412960, 17.78374723810611258 ) ) ;
#42931=CARTESIAN_POINT ( 'NONE',  ( 70.26639875985991068, 15.51307715494295891, 39.29493570883701636 ) ) ;
#42936=CARTESIAN_POINT ( 'NONE',  ( -27.70562707895080123, 9.007984652865420827, 31.19301926817212944 ) ) ;
#42940=CARTESIAN_POINT ( 'NONE',  ( -5.871577929436020860, 6.771181646175758573, -62.50473750044589849 ) ) ;
#42941=CARTESIAN_POINT ( 'NONE',  ( -173.9526029538035914, 89.57590038685106038, 57.70062692409361205 ) ) ;
#42943=CARTESIAN_POINT ( 'NONE',  ( -120.6739978760426482, 44.33795494230364653, -37.02276080820320203 ) ) ;
#42944=CARTESIAN_POINT ( 'NONE',  ( -83.13046924527391468, 25.15778674529013870, 5.041952259388867041 ) ) ;
#42947=CARTESIAN_POINT ( 'NONE',  ( -124.7710763417278059, 46.96042092553522451, -76.67722191208665095 ) ) ;
#42948=CARTESIAN_POINT ( 'NONE',  ( 68.93219921887765622, 14.12322281954859804, 5.852687346813395308 ) ) ;
#42950=CARTESIAN_POINT ( 'NONE',  ( 91.49210130311621469, 22.20929244416438664, -10.76186516580451524 ) ) ;
#42952=CARTESIAN_POINT ( 'NONE',  ( -37.93379515072632557, 11.77251734620211110, 7.088915133309215300 ) ) ;
#42955=EDGE_LOOP ( 'NONE', ( #44979, #28304, #33028, #5577 ) ) ;
#42957=CARTESIAN_POINT ( 'NONE',  ( 103.0533600994152295, 26.78891014864192499, 88.63686854957322225 ) ) ;
#42958=CARTESIAN_POINT ( 'NONE',  ( -147.7925265216585444, 64.04960911618972830, 57.76075631580095404 ) ) ;
#42962=CARTESIAN_POINT ( 'NONE',  ( 141.2801018238827169, 47.29457739955284978, -42.42097328515919941 ) ) ;
#42963=CARTESIAN_POINT ( 'NONE',  ( -47.65155309726507937, 13.85482731128118239, -70.79954927902053896 ) ) ;
#42965=EDGE_CURVE ( 'NONE', #6792, #36547, #443, .T. ) ;
#42966=DIRECTION ( 'NONE',  ( 0.000000000000000000, 0.000000000000000000, 1.000000000000000000 ) ) ;
#42969=CARTESIAN_POINT ( 'NONE',  ( 32.38493285958205803, 8.611594965040680449, 61.59909279486555533 ) ) ;
#42970=CARTESIAN_POINT ( 'NONE',  ( 185.0682806122092927, 84.19715153078853120, 84.13611250625842786 ) ) ;
#42974=ORIENTED_EDGE ( 'NONE', *, *, #65680, .T. ) ;
#42975=CARTESIAN_POINT ( 'NONE',  ( 93.08174259058942823, 22.79847752828721852, 14.22235957612315005 ) ) ;
#42976=CARTESIAN_POINT ( 'NONE',  ( 181.5079096844945923, 80.47139261082469375, -24.38050707541594875 ) ) ;
#42977=CARTESIAN_POINT ( 'NONE',  ( 208.9583973663597760, 114.1615900753670871, 3.674711021178045822 ) ) ;
#42979=CYLINDRICAL_SURFACE ( 'NONE', #41955, 7.500000000000013323 ) ;
#42980=CARTESIAN_POINT ( 'NONE',  ( 42.70988075781784232, 8.862408058333477001, -23.02393441155776088 ) ) ;
#42983=CARTESIAN_POINT ( 'NONE',  ( 164.4761273435911164, 64.62485394454741083, 61.02434369218256904 ) ) ;
#42985=AXIS2_PLACEMENT_3D ( 'NONE', #27583, #26894, #11057 ) ;
#42987=CARTESIAN_POINT ( 'NONE',  ( -149.5074843970971017, 64.17983161892348676, -22.96827994102829962 ) ) ;
#42988=CARTESIAN_POINT ( 'NONE',  ( 94.02499804464933675, 23.15433260743127519, -42.04956284518182485 ) ) ;
#42992=CARTESIAN_POINT ( 'NONE',  ( 150.0433793199863999, 52.09973307442957235, 8.984650821496048323 ) ) ;
#42993=CARTESIAN_POINT ( 'NONE',  ( -15.30860234794697128, 8.505246639038775314, 91.90313363028508320 ) ) ;
#42996=CARTESIAN_POINT ( 'NONE',  ( 110.2429982417149574, -170.0000000000000000, -35.92243756565368784 ) ) ;
#42998=ORIENTED_EDGE ( 'NONE', *, *, #38644, .T. ) ;
#43000=CARTESIAN_POINT ( 'NONE',  ( 39.74315982117121138, 9.468838313655563610, 83.60352190905523173 ) ) ;
#43002=CARTESIAN_POINT ( 'NONE',  ( 91.49210130311617206, 22.20929244416436887, -64.45096634673186031 ) ) ;
#43004=CARTESIAN_POINT ( 'NONE',  ( -61.38706483483510823, 16.47181058798476272, -65.53751323400399542 ) ) ;
#43005=CARTESIAN_POINT ( 'NONE',  ( -1.328627985309863258, 7.561890325089884790, 7.015677182669254996 ) ) ;
#43006=CARTESIAN_POINT ( 'NONE',  ( 178.1888264190354221, 77.13727704498026583, -36.79301795762072658 ) ) ;
#43007=CARTESIAN_POINT ( 'NONE',  ( 161.5764509652428558, 60.91546192849696695, 84.31444485276320222 ) ) ;
#43008=CARTESIAN_POINT ( 'NONE',  ( 94.12811352634518869, 22.11743943276050217, 36.68810650112212812 ) ) ;
#43011=CARTESIAN_POINT ( 'NONE',  ( -47.94536219817736367, 13.92422159065987586, -45.16206988751260099 ) ) ;
#43013=CARTESIAN_POINT ( 'NONE',  ( -173.1211646369891355, -170.0000000000000000, 38.32169460664103156 ) ) ;
#43015=CARTESIAN_POINT ( 'NONE',  ( 8.679939806240504652, 7.383357464882123189, 39.91928050070973200 ) ) ;
#43018=CARTESIAN_POINT ( 'NONE',  ( 79.17818378172918869, 17.01182329587643238, 91.82197126792017627 ) ) ;
#43023=EDGE_CURVE ( 'NONE', #35894, #49086, #50234, .T. ) ;
#43025=AXIS2_PLACEMENT_3D ( 'NONE', #67829, #15046, #19276 ) ;
#43027=CARTESIAN_POINT ( 'NONE',  ( -166.2780847427887352, 81.26478456797779870, 88.92219257149233158 ) ) ;
#43031=CARTESIAN_POINT ( 'NONE',  ( -38.68632430131781064, 11.91908191268693251, 66.50744903314554790 ) ) ;
#43033=CARTESIAN_POINT ( 'NONE',  ( -12.78319349481551725, 8.274445259016797394, -10.42464620885755266 ) ) ;
#43034=CARTESIAN_POINT ( 'NONE',  ( 153.8366942494330942, 54.87992279068316037, -63.90365245542865580 ) ) ;
#43038=CARTESIAN_POINT ( 'NONE',  ( -156.4841188516942907, 70.33041971808550841, -45.07929577857993308 ) ) ;
#43039=VERTEX_POINT ( 'NONE', #60074 ) ;
#43041=CARTESIAN_POINT ( 'NONE',  ( 9.319975126229035567, 7.386007236262731368, 94.99999999999866418 ) ) ;
#43042=CARTESIAN_POINT ( 'NONE',  ( -81.90760111942957167, 24.66532273091449312, -35.83518030727707071 ) ) ;
#43044=CARTESIAN_POINT ( 'NONE',  ( -23.94713223918401823, 9.496086756559476427, 90.93069671979091595 ) ) ;
#43045=CARTESIAN_POINT ( 'NONE',  ( -150.5993571094983281, 66.43939758484178526, 3.952979209143682837 ) ) ;
#43050=CARTESIAN_POINT ( 'NONE',  ( -146.9440914296272354, 63.34059920040223091, 84.83934254479170534 ) ) ;
#43054=CARTESIAN_POINT ( 'NONE',  ( -156.4797890011541313, 71.69341087347109465, -18.24543932660331080 ) ) ;
#43055=CARTESIAN_POINT ( 'NONE',  ( 87.42982051347729566, 20.76007613954182318, -89.54297233556741276 ) ) ;
#43061=CARTESIAN_POINT ( 'NONE',  ( -149.9449619562961402, 64.55090813009800854, 57.56537183036274996 ) ) ;
#43063=CARTESIAN_POINT ( 'NONE',  ( 22.62427395637551086, 7.823784829753561709, 7.575073927682081987 ) ) ;
#43066=CARTESIAN_POINT ( 'NONE',  ( -84.97622048504842951, 24.82614411847759683, -46.67722756215049884 ) ) ;
#43067=CARTESIAN_POINT ( 'NONE',  ( 19.75784582661439970, 6.660183274347837745, 70.72739093580082681 ) ) ;
#43069=CARTESIAN_POINT ( 'NONE',  ( 8.528421445032392967, 6.376778749352034481, -71.80901206443022033 ) ) ;
#43077=CARTESIAN_POINT ( 'NONE',  ( 46.41758729921146198, 9.425975226414248453, -72.62734698405610345 ) ) ;
#43078=CARTESIAN_POINT ( 'NONE',  ( 55.56634333706183781, 12.09342294753929714, -71.06672960848410980 ) ) ;
#43079=VERTEX_POINT ( 'NONE', #6265 ) ;
#43085=B_SPLINE_CURVE_WITH_KNOTS ( 'NONE', 3,
 ( #46398, #56267, #3497, #24275, #4198, #51001, #63283, #18985, #8084, #68557, #29889, #51691, #30239, #35160, #25662, #14409, #61885, #67878, #24623, #20031, #62936, #56617, #14053, #46057, #8792, #29531, #52031, #56975, #51353, #45722, #35513, #8439, #20360, #47094, #13707, #3165, #19674, #41827, #67528, #36206, #41134, #15093, #57661, #30583, #41484, #62601, #35860, #9473, #40437, #3851, #57314, #9129, #46750, #14740, #2812, #68223, #19328, #30934 ),
 .UNSPECIFIED., .F., .F.,
 ( 4, 2, 2, 2, 2, 2, 2, 2, 2, 2, 2, 2, 2, 2, 2, 2, 2, 2, 2, 2, 2, 2, 2, 2, 2, 2, 2, 2, 4 ),
 ( 0.000000000000000000, 0.002174461951613288098, 0.003261692927419951663, 0.004348923903226615227, 0.005436154879033277924, 0.006523385854839942356, 0.007610616830646605054, 0.008697847806453268618, 0.009785078782259933050, 0.01087230975806659575, 0.01195954073387325844, 0.01304677170967992288, 0.01522123366129330725, 0.01630846463709996821, 0.01739569561290663091, 0.01957015756451988345, 0.02065738854032650451, 0.02174461951613312558, 0.02391908146774630525, 0.02609354341935948840, 0.02718077439516605742, 0.02826800537097262644, 0.02881162085887593177, 0.02935523634677923710, 0.03044246732258585816, 0.03152969829839247229, 0.03261692927419908988, 0.03370416025000570748, 0.03479139122581232507 ),
 .UNSPECIFIED. ) ;
#43086=VECTOR ( 'NONE', #63176, 1000.000000000000000 ) ;
#43087=CARTESIAN_POINT ( 'NONE',  ( 197.4121679705847896, 98.46451029407256783, 8.075550651409916014 ) ) ;
#43089=ORIENTED_EDGE ( 'NONE', *, *, #33274, .F. ) ;
#43090=EDGE_CURVE ( 'NONE', #40950, #16235, #14656, .T. ) ;
#43092=CARTESIAN_POINT ( 'NONE',  ( 117.3110050642448243, 32.29133253383017177, 61.39698313137674290 ) ) ;
#43094=CARTESIAN_POINT ( 'NONE',  ( 116.8917656767876565, 33.20682060519245482, 67.43530244170412402 ) ) ;
#43095=CARTESIAN_POINT ( 'NONE',  ( 103.0463737467386665, 26.78595250599333255, -95.00000000000133582 ) ) ;
#43096=CARTESIAN_POINT ( 'NONE',  ( 138.5684226926155418, 45.53585076428268508, 69.70997248683153202 ) ) ;
#43102=EDGE_LOOP ( 'NONE', ( #10465, #13359, #5434, #37827 ) ) ;
#43106=ADVANCED_FACE ( 'NONE', ( #12958 ), #34758, .F. ) ;
#43107=CARTESIAN_POINT ( 'NONE',  ( -145.3246383987844297, 62.00818849034185121, -48.54254619255401337 ) ) ;
#43110=CARTESIAN_POINT ( 'NONE',  ( -144.9287131874382055, 60.39056348581544853, -36.35316711580674820 ) ) ;
#43114=LINE ( 'NONE', #30594, #50330 ) ;
#43116=CARTESIAN_POINT ( 'NONE',  ( 79.14129363775931836, 17.00055658855363916, -16.97005576640699331 ) ) ;
#43121=CARTESIAN_POINT ( 'NONE',  ( -94.79534239005255358, 29.13842790650045700, -69.90232742285510881 ) ) ;
#43123=ORIENTED_EDGE ( 'NONE', *, *, #2276, .T. ) ;
#43127=CARTESIAN_POINT ( 'NONE',  ( 39.40195752203892710, -170.0000000000000000, 56.75838489642694640 ) ) ;
#43129=CARTESIAN_POINT ( 'NONE',  ( 107.9342863085848450, 28.93180871323605174, -77.41840800766151176 ) ) ;
#43130=CARTESIAN_POINT ( 'NONE',  ( 80.30232379693109124, 17.35837133860831116, 33.17720279973744368 ) ) ;
#43133=CARTESIAN_POINT ( 'NONE',  ( 46.84154678921878912, 10.51341196666389521, -44.10166628834166147 ) ) ;
#43134=CARTESIAN_POINT ( 'NONE',  ( 204.6977192012829789, 106.3443248447423315, 71.05227132923315025 ) ) ;
#43137=CARTESIAN_POINT ( 'NONE',  ( -109.5142642360664667, 36.61018064014776741, -17.71775249749087067 ) ) ;
#43139=CARTESIAN_POINT ( 'NONE',  ( -15.32520546926283345, 7.495995523981875408, -42.42519461880208809 ) ) ;
#43141=CARTESIAN_POINT ( 'NONE',  ( -81.10316978278179079, 23.26460499017369798, 84.50753759321933956 ) ) ;
#43142=CARTESIAN_POINT ( 'NONE',  ( 93.08073375333748345, 22.79826000593200774, 60.22361380431165401 ) ) ;
#43143=CARTESIAN_POINT ( 'NONE',  ( 150.2809931605061990, 52.27058242113236020, -18.93275037951032758 ) ) ;
#43144=CARTESIAN_POINT ( 'NONE',  ( 32.89501968360929851, 8.663558833820818705, 14.33097644123245828 ) ) ;
#43145=CARTESIAN_POINT ( 'NONE',  ( -95.20053778133916467, 30.43887292928076960, -71.88691849379360121 ) ) ;
#43147=ORIENTED_EDGE ( 'NONE', *, *, #34391, .T. ) ;
#43148=CARTESIAN_POINT ( 'NONE',  ( 212.1414097338564488, 117.1449328067268993, 89.45312194060214495 ) ) ;
#43153=CARTESIAN_POINT ( 'NONE',  ( -10.23531775138760658, 8.068923942586298637, 3.664519661588847121 ) ) ;
#43154=CARTESIAN_POINT ( 'NONE',  ( 45.04020069093783007, 10.22779424730543063, -64.99450957612113200 ) ) ;
#43155=CARTESIAN_POINT ( 'NONE',  ( -2.174378755909792460, 6.588636630831476992, 42.57095561852364085 ) ) ;
#43157=CARTESIAN_POINT ( 'NONE',  ( 84.41121179164569810, 19.73587740566237159, 83.72931267887217643 ) ) ;
#43160=CARTESIAN_POINT ( 'NONE',  ( -149.5074843970971017, 65.50121172469319220, 72.56537183036277838 ) ) ;
#43161=CARTESIAN_POINT ( 'NONE',  ( -131.3154845336013068, 50.16828105866954246, 6.070552893135558570 ) ) ;
#43162=CARTESIAN_POINT ( 'NONE',  ( -166.7136514167008556, 81.71618216218797670, -46.11898781893540900 ) ) ;
#43163=EDGE_CURVE ( 'NONE', #7668, #9033, #49955, .T. ) ;
#43165=CARTESIAN_POINT ( 'NONE',  ( -180.5628792467297501, 95.81282809867099104, 91.05901154845440715 ) ) ;
#43170=CARTESIAN_POINT ( 'NONE',  ( -156.8688717293649972, 70.68369417233287777, 93.38775103858958460 ) ) ;
#43172=B_SPLINE_CURVE_WITH_KNOTS ( 'NONE', 3,
 ( #16980, #10665, #65185, #38450, #53572, #113, #11709, #53911, #6079, #6784, #49681, #59539, #21916, #5402, #11357, #27539, #32134, #21568, #5734, #27190, #59887, #48622, #64839, #48979, #6445, #60251, #43011, #64489, #16301, #37749, #59196, #12070, #33539, #32478, #54967, #32825, #466, #54253, #7502, #45460, #66942, #60947, #17699, #8536 ),
 .UNSPECIFIED., .F., .F.,
 ( 4, 2, 2, 2, 2, 2, 2, 2, 2, 2, 2, 2, 2, 2, 2, 2, 2, 2, 2, 2, 2, 4 ),
 ( 0.000000000000000000, 0.001488594467279787332, 0.002232891700919671998, 0.002977188934559557316, 0.004465783401839307568, 0.005954377869119058253, 0.007442972336398808071, 0.008187269570038688618, 0.008931566803678568298, 0.01042016127095831204, 0.01190875573823805232, 0.01265305297187791292, 0.01339735020551777699, 0.01488594467279747389, 0.01563024190643732408, 0.01637453914007717254, 0.01786313360735686598, 0.01935172807463656636, 0.02009602530827640440, 0.02084032254191624939, 0.02232891700919594283, 0.02381751147647563974 ),
 .UNSPECIFIED. ) ;
#43173=CARTESIAN_POINT ( 'NONE',  ( 134.3159642998340644, 41.70198410084979201, 29.51034083899532590 ) ) ;
#43176=CARTESIAN_POINT ( 'NONE',  ( 79.91920957766411959, 18.29292522273509647, 13.75549202193108833 ) ) ;
#43177=CARTESIAN_POINT ( 'NONE',  ( 164.8914542114683570, 64.97670918603526502, 8.943675762355397296 ) ) ;
#43178=EDGE_CURVE ( 'NONE', #31575, #67718, #6161, .T. ) ;
#43184=ORIENTED_EDGE ( 'NONE', *, *, #64969, .F. ) ;
#43185=CARTESIAN_POINT ( 'NONE',  ( -72.21652659655759976, 19.96855882996550235, -19.63090997373414481 ) ) ;
#43188=CARTESIAN_POINT ( 'NONE',  ( 150.0516754638055943, 53.34587188591231666, 8.929522449978659182 ) ) ;
#43190=CARTESIAN_POINT ( 'NONE',  ( 163.1495034066983862, 62.20479872133083177, 41.83434947820244787 ) ) ;
#43195=CARTESIAN_POINT ( 'NONE',  ( -31.43908319763710679, 9.591432048623756756, -8.472646774738153752 ) ) ;
#43196=CARTESIAN_POINT ( 'NONE',  ( -180.4614954900548298, 97.28277348252828460, 36.75295334209538112 ) ) ;
#43197=CARTESIAN_POINT ( 'NONE',  ( 140.0012045870120687, 46.45892655944614091, 94.99999999999866418 ) ) ;
#43200=ORIENTED_EDGE ( 'NONE', *, *, #3335, .T. ) ;
#43205=CARTESIAN_POINT ( 'NONE',  ( 70.50670201344738075, 14.53584474203976917, 90.50562999910829376 ) ) ;
#43207=CARTESIAN_POINT ( 'NONE',  ( -55.05276343752909440, 15.72344139423348430, -50.21632399845989170 ) ) ;
#43214=CARTESIAN_POINT ( 'NONE',  ( 188.0081045302011944, 85.89855126821618114, 33.91234789090425039 ) ) ;
#43217=CARTESIAN_POINT ( 'NONE',  ( -71.43874587651171737, 19.69883891272895227, 9.055200870754841702 ) ) ;
#43218=CARTESIAN_POINT ( 'NONE',  ( -123.0348077379026392, 45.83489305753317922, 71.90199806622466383 ) ) ;
#43219=DIRECTION ( 'NONE',  ( 0.000000000000000000, 0.000000000000000000, 1.000000000000000000 ) ) ;
#43223=VECTOR ( 'NONE', #64110, 1000.000000000000000 ) ;
#43224=EDGE_LOOP ( 'NONE', ( #31538, #18923, #62872, #44785 ) ) ;
#43233=CARTESIAN_POINT ( 'NONE',  ( 39.88975917505624835, 9.487965272711656795, 29.91383430596323834 ) ) ;
#43236=CARTESIAN_POINT ( 'NONE',  ( -145.9095871962850310, 61.18682730038537443, 17.96100122531099075 ) ) ;
#43237=ORIENTED_EDGE ( 'NONE', *, *, #4786, .T. ) ;
#43239=CARTESIAN_POINT ( 'NONE',  ( -132.5976199670998881, 52.30296609017644016, 34.74704912185334393 ) ) ;
#43241=CARTESIAN_POINT ( 'NONE',  ( -166.2425995121691642, -170.0000000000000000, 94.99999999999866418 ) ) ;
#43243=CARTESIAN_POINT ( 'NONE',  ( 61.10129719786242219, 12.23677173834304810, 71.41316413118165940 ) ) ;
#43244=CARTESIAN_POINT ( 'NONE',  ( -7.330587818645181386, 7.867004275019543691, 71.96013162991091860 ) ) ;
#43245=EDGE_CURVE ( 'NONE', #24506, #18617, #34730, .T. ) ;
#43249=ORIENTED_EDGE ( 'NONE', *, *, #16205, .F. ) ;
#43253=CARTESIAN_POINT ( 'NONE',  ( 135.4423125506058625, 42.39015362494583883, -77.70187412784397907 ) ) ;
#43255=CARTESIAN_POINT ( 'NONE',  ( 69.73342236697678231, 14.33173522011652778, 33.94168038989159442 ) ) ;
#43257=CARTESIAN_POINT ( 'NONE',  ( 79.11678589158262298, 16.99307320450158443, 10.37612617437139662 ) ) ;
#43259=CARTESIAN_POINT ( 'NONE',  ( -73.09185868250597196, 20.27574131633383558, 42.95950369064131280 ) ) ;
#43262=ADVANCED_FACE ( 'NONE', ( #54719 ), #27990, .F. ) ;
#43267=CARTESIAN_POINT ( 'NONE',  ( 90.30166390191403991, 20.70652093100729019, 3.810012513778408216 ) ) ;
#43268=EDGE_CURVE ( 'NONE', #63745, #52584, #41446, .T. ) ;
#43276=CARTESIAN_POINT ( 'NONE',  ( 151.7956716830626362, 53.36999433148312733, 41.81961525401386126 ) ) ;
#43278=CARTESIAN_POINT ( 'NONE',  ( 67.93154431625913503, 14.90489441944787430, 31.62713259101203178 ) ) ;
#43282=CARTESIAN_POINT ( 'NONE',  ( 134.3182571105338923, 42.88121222759018991, -62.86786152285935003 ) ) ;
#43285=FACE_BOUND ( 'NONE', #45208, .T. ) ;
#43286=CARTESIAN_POINT ( 'NONE',  ( -0.8011128725815451768, 6.535315321814158196, -67.12254502563429526 ) ) ;
#43287=CARTESIAN_POINT ( 'NONE',  ( -178.5848962563133568, 94.99295350784007042, 70.32832319493537909 ) ) ;
#43288=CARTESIAN_POINT ( 'NONE',  ( 113.9884483999549047, 30.65255989963792160, -90.56438067049403173 ) ) ;
#43289=CARTESIAN_POINT ( 'NONE',  ( -124.9915686518654780, 47.10215472274616388, -34.91370389823391918 ) ) ;
#43290=CARTESIAN_POINT ( 'NONE',  ( -84.55783695959765112, 25.74181993349144548, 15.74135957251160001 ) ) ;
#43291=CARTESIAN_POINT ( 'NONE',  ( 133.3990214534117058, 41.14886683286417224, 2.676281182479414156 ) ) ;
#43293=CARTESIAN_POINT ( 'NONE',  ( -73.58753291667264307, 20.45143618612268455, -90.76877822284814101 ) ) ;
#43294=CARTESIAN_POINT ( 'NONE',  ( 65.40032188136231639, 13.23841673691966925, 3.353476667165713465 ) ) ;
#43296=CARTESIAN_POINT ( 'NONE',  ( 93.43270425363543552, 22.93046121381056324, -19.64350642960366855 ) ) ;
#43297=ORIENTED_EDGE ( 'NONE', *, *, #11514, .F. ) ;
#43300=CARTESIAN_POINT ( 'NONE',  ( 108.3906473026529937, 28.03385344351494624, -62.98435907625002272 ) ) ;
#43301=VERTEX_POINT ( 'NONE', #59302 ) ;
#43302=B_SPLINE_CURVE_WITH_KNOTS ( 'NONE', 3,
 ( #65594, #65957, #59943, #29342, #17756, #39211, #12470, #33934, #50104, #1934, #66312, #18099, #12829, #34284, #55732, #7554, #29013, #35313 ),
 .UNSPECIFIED., .F., .F.,
 ( 4, 2, 2, 2, 2, 2, 2, 2, 4 ),
 ( 9.309503074677274191E-17, 0.002090076166982583316, 0.003135114250473834858, 0.003657633292219452607, 0.004180152333965070355, 0.005225190417456297177, 0.006270228500947524868, 0.007315266584438751690, 0.008360304667929979380 ),
 .UNSPECIFIED. ) ;
#43304=CARTESIAN_POINT ( 'NONE',  ( 107.7683756309525336, 28.85711661752776180, 83.71285356453704196 ) ) ;
#43305=CARTESIAN_POINT ( 'NONE',  ( -145.3246383987844581, 62.00818849034184410, 58.83565616930072650 ) ) ;
#43306=CARTESIAN_POINT ( 'NONE',  ( 86.62931800182293784, -170.0000000000000000, -35.82156419891171595 ) ) ;
#43307=CARTESIAN_POINT ( 'NONE',  ( -24.60892750534351237, 9.584951112520231575, -45.92522378588709842 ) ) ;
#43309=CARTESIAN_POINT ( 'NONE',  ( -47.56466076048273095, 13.83435953640667826, -70.05170999023415845 ) ) ;
#43312=CARTESIAN_POINT ( 'NONE',  ( -123.6618353044034535, 46.23845779494348562, -22.74412515443657767 ) ) ;
#43315=CARTESIAN_POINT ( 'NONE',  ( 32.09610685027467269, 8.582590950734816815, 62.54528762178141221 ) ) ;
#43318=CARTESIAN_POINT ( 'NONE',  ( -166.7050147108374460, 81.70694330787519277, 69.08965843878142721 ) ) ;
#43319=CARTESIAN_POINT ( 'NONE',  ( 130.9157159354502369, 40.84309122054532537, -90.30233232517586828 ) ) ;
#43326=CARTESIAN_POINT ( 'NONE',  ( 187.5246323291927126, 86.86207184872515086, -12.99861875644394971 ) ) ;
#43329=CARTESIAN_POINT ( 'NONE',  ( 39.88971011078924533, 8.472992116645418292, -23.77526687496409252 ) ) ;
#43330=CYLINDRICAL_SURFACE ( 'NONE', #6123, 7.500000000000013323 ) ;
#43334=CARTESIAN_POINT ( 'NONE',  ( 164.9540180502650912, 65.02981548735056094, 64.32247932210420061 ) ) ;
#43335=AXIS2_PLACEMENT_3D ( 'NONE', #3516, #14072, #46419 ) ;
#43336=EDGE_CURVE ( 'NONE', #3776, #62313, #62370, .T. ) ;
#43341=CARTESIAN_POINT ( 'NONE',  ( 93.72059824125564376, 23.03897520779758423, -40.82895870122177939 ) ) ;
#43342=CARTESIAN_POINT ( 'NONE',  ( -54.57263979903870421, 15.59415114099630983, 57.16187836339484107 ) ) ;
#43344=EDGE_CURVE ( 'NONE', #54626, #48794, #38063, .T. ) ;
#43345=CARTESIAN_POINT ( 'NONE',  ( -7.825402957745087207, -170.0000000000000000, -16.07352014148014163 ) ) ;
#43346=CARTESIAN_POINT ( 'NONE',  ( -12.63148932007802472, 8.261552044977213072, 85.53769020324797623 ) ) ;
#43348=CARTESIAN_POINT ( 'NONE',  ( 56.19211641164837090, 11.19288081156168246, 7.345765177167212556 ) ) ;
#43354=CARTESIAN_POINT ( 'NONE',  ( 103.9652201950894437, 26.08439499369982428, 41.22229790462832000 ) ) ;
#43357=CARTESIAN_POINT ( 'NONE',  ( -57.42615654242916889, 15.33060010148602892, -62.44219422609327808 ) ) ;
#43358=CARTESIAN_POINT ( 'NONE',  ( -2.873329055852804625, 7.626065826870669362, 5.116632491166936525 ) ) ;
#43360=CARTESIAN_POINT ( 'NONE',  ( 180.2494929075577943, 79.18888319146950039, -36.22505766587960352 ) ) ;
#43362=CARTESIAN_POINT ( 'NONE',  ( 164.2665160441432874, 63.13418342263689453, 93.79059897813883140 ) ) ;
#43367=CARTESIAN_POINT ( 'NONE',  ( 106.4072861358878299, 28.24787347451998798, -10.12839677197858812 ) ) ;
#43370=CARTESIAN_POINT ( 'NONE',  ( -29.03891846981456126, 10.22741474064059020, 30.59402320536396402 ) ) ;
#43372=CARTESIAN_POINT ( 'NONE',  ( 79.68455349783286579, 17.16711484584623904, 93.81489682416450648 ) ) ;
#43374=CYLINDRICAL_SURFACE ( 'NONE', #19706, 7.500000000000013323 ) ;
#43380=CARTESIAN_POINT ( 'NONE',  ( -53.13004807512038496, 14.17398740785106526, 45.08299798962536187 ) ) ;
#43381=CARTESIAN_POINT ( 'NONE',  ( -55.05276343752909440, 14.68156374112638929, -23.37177340799619785 ) ) ;
#43384=CARTESIAN_POINT ( 'NONE',  ( -55.05276343752909440, 15.72344139423348430, -50.21632399845989170 ) ) ;
#43385=CARTESIAN_POINT ( 'NONE',  ( -14.56631729561072675, 8.434645566888200108, -12.74894963134235049 ) ) ;
#43389=AXIS2_PLACEMENT_3D ( 'NONE', #47045, #5171, #26289 ) ;
#43393=CARTESIAN_POINT ( 'NONE',  ( 63.01563776193090405, 13.70579113808098093, -8.876140241706053757 ) ) ;
#43394=CARTESIAN_POINT ( 'NONE',  ( -57.96271610907653837, 16.52641986079314762, -89.48962646049473335 ) ) ;
#43395=CARTESIAN_POINT ( 'NONE',  ( -62.41990535723909517, 17.83270318706536983, -95.00000000000133582 ) ) ;
#43396=CARTESIAN_POINT ( 'NONE',  ( 110.7167338301703978, 30.21148223254618870, -9.077886975190001095 ) ) ;
#43397=CARTESIAN_POINT ( 'NONE',  ( -108.0980548770428271, 35.83569586822709141, 15.93332971359382988 ) ) ;
#43400=ORIENTED_EDGE ( 'NONE', *, *, #68025, .T. ) ;
#43404=CARTESIAN_POINT ( 'NONE',  ( -155.7455325080990747, 71.01834415181986060, -11.29636591650952582 ) ) ;
#43405=CARTESIAN_POINT ( 'NONE',  ( 89.73102809687581782, 21.57092797140214557, -90.17038539412145326 ) ) ;
#43406=CARTESIAN_POINT ( 'NONE',  ( -34.74740905761647269, 10.15745573515589406, 71.30966891704866839 ) ) ;
#43407=CARTESIAN_POINT ( 'NONE',  ( -153.6931187576189757, 67.81270084382354923, -21.69602582841185878 ) ) ;
#43409=CARTESIAN_POINT ( 'NONE',  ( 185.5412249395996582, 84.70425786166002524, 57.61695868165770662 ) ) ;
#43410=CARTESIAN_POINT ( 'NONE',  ( -156.1462053606562961, 70.02140399657017156, 68.56529437304638464 ) ) ;
#43413=CARTESIAN_POINT ( 'NONE',  ( 126.6904219525097659, 38.41566710102375737, -95.00000000000133582 ) ) ;
#43416=ADVANCED_FACE ( 'NONE', ( #3691 ), #36056, .F. ) ;
#43418=CARTESIAN_POINT ( 'NONE',  ( 15.78827728214693416, 6.500811158483284835, -77.36349468914950478 ) ) ;
#43424=CARTESIAN_POINT ( 'NONE',  ( -133.2698123908828620, 51.54642138335022850, -41.02960792264190104 ) ) ;
#43426=CARTESIAN_POINT ( 'NONE',  ( 56.52205390515080552, 12.28646189164057745, -66.28031366309063799 ) ) ;
#43431=CARTESIAN_POINT ( 'NONE',  ( -24.32937228292060539, 8.531905774118438757, -18.41076230671387037 ) ) ;
#43432=CARTESIAN_POINT ( 'NONE',  ( 185.0770371948367199, 82.73585087248531522, 84.12142509379798128 ) ) ;
#43433=VERTEX_POINT ( 'NONE', #21251 ) ;
#43436=CARTESIAN_POINT ( 'NONE',  ( 186.5979919519638486, 85.84756789133375321, 41.89830629180269739 ) ) ;
#43438=VERTEX_POINT ( 'NONE', #15633 ) ;
#43439=CARTESIAN_POINT ( 'NONE',  ( 116.5100763992442836, 33.01539745157281658, 68.08308399614098505 ) ) ;
#43443=CARTESIAN_POINT ( 'NONE',  ( 164.4645769411267793, 63.30014054308799842, -94.56787564473663110 ) ) ;
#43445=CARTESIAN_POINT ( 'NONE',  ( -47.60266343315662851, 13.84328785304053078, -14.87255105764826446 ) ) ;
#43450=DIRECTION ( 'NONE',  ( -0.8118923937861950435, -0.5838071093367415143, 0.000000000000000000 ) ) ;
#43452=CARTESIAN_POINT ( 'NONE',  ( -166.7050147108374460, 81.70694330787516435, -65.13309451353698876 ) ) ;
#43453=CARTESIAN_POINT ( 'NONE',  ( -146.7345109736526183, 61.86270848728295135, -35.34073819673365335 ) ) ;
#43456=ORIENTED_EDGE ( 'NONE', *, *, #4841, .T. ) ;
#43457=FACE_OUTER_BOUND ( 'NONE', #66786, .T. ) ;
#43459=CYLINDRICAL_SURFACE ( 'NONE', #44604, 7.500000000000013323 ) ;
#43461=CARTESIAN_POINT ( 'NONE',  ( 79.53408731553403754, 17.12082763744058411, -13.99589305005577877 ) ) ;
#43464=CYLINDRICAL_SURFACE ( 'NONE', #59500, 7.500000000000013323 ) ;
#43470=CARTESIAN_POINT ( 'NONE',  ( 46.64694836521739774, 9.462741877720624473, 35.45895907357519405 ) ) ;
#43476=CARTESIAN_POINT ( 'NONE',  ( 212.1669304543881651, 119.0398299474538533, -44.52663591005489963 ) ) ;
#43477=PLANE ( 'NONE',  #46110 ) ;
#43479=CARTESIAN_POINT ( 'NONE',  ( 67.93154431625912082, 14.90489441944787075, -48.90651918037900003 ) ) ;
#43480=CARTESIAN_POINT ( 'NONE',  ( -118.8392474096542202, 43.20060570451234838, 35.52071490940999610 ) ) ;
#43483=EDGE_LOOP ( 'NONE', ( #43583, #6062 ) ) ;
#43484=CARTESIAN_POINT ( 'NONE',  ( -24.18270484670773257, 9.527492911955587118, 12.83203105897101892 ) ) ;
#43486=CARTESIAN_POINT ( 'NONE',  ( -11.14445507968271976, 7.129894202659276203, -49.64817737260776198 ) ) ;
#43490=CARTESIAN_POINT ( 'NONE',  ( 93.72059824125561533, 23.03897520779757357, 66.54924366063296759 ) ) ;
#43491=CARTESIAN_POINT ( 'NONE',  ( 151.3309484205705076, 53.03078371058071383, -12.46437990871518409 ) ) ;
#43492=DIRECTION ( 'NONE',  ( 0.000000000000000000, 0.000000000000000000, 1.000000000000000000 ) ) ;
#43493=CARTESIAN_POINT ( 'NONE',  ( -94.78138776532239262, 30.24234841992714706, -68.82308172911717747 ) ) ;
#43494=CARTESIAN_POINT ( 'NONE',  ( 110.2429982417149574, 29.99119854320845846, -89.61153874658103291 ) ) ;
#43499=CARTESIAN_POINT ( 'NONE',  ( -31.43908319763709258, 9.591432048623765638, 18.37190381572551701 ) ) ;
#43500=CARTESIAN_POINT ( 'NONE',  ( -125.8938041572051389, -170.0000000000000000, -34.91370389823391918 ) ) ;
#43504=CARTESIAN_POINT ( 'NONE',  ( 79.29204528441387367, 18.09916687801608504, 92.49219715506139039 ) ) ;
#43505=EDGE_CURVE ( 'NONE', #67008, #22304, #12034, .T. ) ;
#43507=ORIENTED_EDGE ( 'NONE', *, *, #43807, .F. ) ;
#43511=CARTESIAN_POINT ( 'NONE',  ( -168.7314919967217861, 83.83749564070829763, -36.11248519031690307 ) ) ;
#43512=CARTESIAN_POINT ( 'NONE',  ( -126.3495878770406193, 48.00153794568856114, -34.91370389823391918 ) ) ;
#43515=CARTESIAN_POINT ( 'NONE',  ( -5.871577929436022636, 6.771181646175757685, -8.815636319518523223 ) ) ;
#43517=CARTESIAN_POINT ( 'NONE',  ( 197.4121679705847612, 98.46451029407255362, -18.76899993905374586 ) ) ;
#43518=CARTESIAN_POINT ( 'NONE',  ( -144.4736899159893824, 60.02381438289076243, 86.31825897600546682 ) ) ;
#43520=CARTESIAN_POINT ( 'NONE',  ( 116.4569059613810680, -170.0000000000000000, 94.99999999999866418 ) ) ;
#43523=CARTESIAN_POINT ( 'NONE',  ( 84.27937148876361562, 19.69225537006225579, 3.241133752072656193 ) ) ;
#43524=VECTOR ( 'NONE', #48166, 1000.000000000000000 ) ;
#43525=CARTESIAN_POINT ( 'NONE',  ( -96.77705718164446580, 31.18700926299574050, 43.13870737491041041 ) ) ;
#43534=CARTESIAN_POINT ( 'NONE',  ( 178.1965488566140152, 77.14488558164482868, 29.87333967559920822 ) ) ;
#43535=DIRECTION ( 'NONE',  ( 0.000000000000000000, 0.000000000000000000, 1.000000000000000000 ) ) ;
#43538=CARTESIAN_POINT ( 'NONE',  ( 162.8142581494935826, 61.92799983924230389, 42.19344870861107921 ) ) ;
#43544=CARTESIAN_POINT ( 'NONE',  ( 152.6650207832379351, 54.00889961337554723, -91.54105675057486735 ) ) ;
#43545=CARTESIAN_POINT ( 'NONE',  ( -38.26732153931118319, 10.81230693396213027, -72.77399863615724485 ) ) ;
#43546=B_SPLINE_CURVE_WITH_KNOTS ( 'NONE', 3,
 ( #30341, #67983, #14841, #4303, #41245, #53144, #58104, #63388, #52135, #20461 ),
 .UNSPECIFIED., .F., .F.,
 ( 4, 2, 2, 2, 4 ),
 ( 0.000000000000000000, 0.002530181115235016244, 0.005060362230470032488, 0.007590543345705047865, 0.01012072446094006324 ),
 .UNSPECIFIED. ) ;
#43552=CARTESIAN_POINT ( 'NONE',  ( -47.90432812485480696, 12.88062469954617306, 93.79905434906177675 ) ) ;
#43555=CARTESIAN_POINT ( 'NONE',  ( -149.9449619562961118, 64.55090813009796591, -76.65738112195566600 ) ) ;
#43557=CARTESIAN_POINT ( 'NONE',  ( 70.09861411860619285, 14.42781432017776666, 93.49106116398942845 ) ) ;
#43560=CARTESIAN_POINT ( 'NONE',  ( -125.8938041572051105, 46.49392987655495091, 72.46449846362081360 ) ) ;
#43561=CARTESIAN_POINT ( 'NONE',  ( -47.78501581516121632, 13.88632236864699010, 89.62634416545391502 ) ) ;
#43563=CARTESIAN_POINT ( 'NONE',  ( 81.57482918025355900, 17.75786713398421313, 69.60303055166224340 ) ) ;
#43567=EDGE_CURVE ( 'NONE', #42077, #49905, #54985, .T. ) ;
#43569=CARTESIAN_POINT ( 'NONE',  ( 212.1931396682532807, 117.2245435827728954, -70.35676384241855885 ) ) ;
#43572=DIRECTION ( 'NONE',  ( -0.000000000000000000, 1.000000000000000000, -0.000000000000000000 ) ) ;
#43576=CARTESIAN_POINT ( 'NONE',  ( 197.1981527292630858, 96.59367172725642092, 90.15674701874463892 ) ) ;
#43577=CARTESIAN_POINT ( 'NONE',  ( 156.5909039492010209, 56.96742803863244831, -36.12418429913764584 ) ) ;
#43582=CARTESIAN_POINT ( 'NONE',  ( -173.1211646369891355, -170.0000000000000000, -42.21195716474999671 ) ) ;
#43583=ORIENTED_EDGE ( 'NONE', *, *, #51686, .F. ) ;
#43585=CARTESIAN_POINT ( 'NONE',  ( -85.35127931077731489, 24.98147633333000783, 34.50846909454845246 ) ) ;
#43586=CARTESIAN_POINT ( 'NONE',  ( -24.95010104166213694, 9.631487977190602123, -65.89293244537743988 ) ) ;
#43587=CARTESIAN_POINT ( 'NONE',  ( 46.80475532923157544, 10.50744084852537341, 36.18526792674665415 ) ) ;
#43588=CARTESIAN_POINT ( 'NONE',  ( -29.75049355503753290, 9.320234381800293733, 57.24947098832353731 ) ) ;
#43597=CARTESIAN_POINT ( 'NONE',  ( 35.66087318222938052, 8.964867769223227256, -22.79433549599965048 ) ) ;
#43598=CARTESIAN_POINT ( 'NONE',  ( 183.8582891103381201, 82.91081946035752992, -90.40977833027336885 ) ) ;
#43599=CARTESIAN_POINT ( 'NONE',  ( 60.63507185982727776, 12.13307030573223244, 71.27383786105745855 ) ) ;
#43600=CARTESIAN_POINT ( 'NONE',  ( 138.5824539808545239, 45.54502076838151226, 84.86660875767417167 ) ) ;
#43601=CARTESIAN_POINT ( 'NONE',  ( -27.05154547620706040, 9.929048335933888580, -90.41981277176407161 ) ) ;
#43607=CARTESIAN_POINT ( 'NONE',  ( 157.9130201331580849, 57.99550255803045218, -24.27963370867398041 ) ) ;
#43610=CARTESIAN_POINT ( 'NONE',  ( 134.7697261969508702, 41.97802808873666436, -77.82602812282750904 ) ) ;
#43612=ORIENTED_EDGE ( 'NONE', *, *, #8844, .F. ) ;
#43613=CARTESIAN_POINT ( 'NONE',  ( 79.19345177405118363, 17.01649702043280499, 11.37811128945321926 ) ) ;
#43615=CARTESIAN_POINT ( 'NONE',  ( -71.16770070143907390, 19.60548673929830343, 37.39342123284746577 ) ) ;
#43616=EDGE_LOOP ( 'NONE', ( #11455, #56382 ) ) ;
#43620=CARTESIAN_POINT ( 'NONE',  ( -55.05276343752909440, 14.68156374112637330, -8.371773407996169425 ) ) ;
#43626=CARTESIAN_POINT ( 'NONE',  ( 157.0336341255056141, 57.31169401067821667, 29.40946747225336111 ) ) ;
#43627=CARTESIAN_POINT ( 'NONE',  ( -173.9617926765113793, 89.58633395456783433, -34.74738087939574172 ) ) ;
#43629=CARTESIAN_POINT ( 'NONE',  ( -7.825402957745081878, 7.899365992529270741, -77.26262132240753999 ) ) ;
#43630=DIRECTION ( 'NONE',  ( 0.000000000000000000, 0.000000000000000000, 1.000000000000000000 ) ) ;
#43632=CARTESIAN_POINT ( 'NONE',  ( 139.3041645503688812, 46.00819478311336042, -75.52888872897204919 ) ) ;
#43633=CARTESIAN_POINT ( 'NONE',  ( -143.3980294393559802, 60.45217072626400068, -73.51509446168660133 ) ) ;
#43635=FACE_BOUND ( 'NONE', #5021, .T. ) ;
#43636=CARTESIAN_POINT ( 'NONE',  ( -1.088326810997879202, 6.545818265928948776, -73.09474285069318000 ) ) ;
#43637=CARTESIAN_POINT ( 'NONE',  ( -177.5288247523079690, 93.72924674643515175, 71.25209080205243595 ) ) ;
#43638=CARTESIAN_POINT ( 'NONE',  ( -144.9412191745148277, 61.69548892475974355, -9.498880540982458598 ) ) ;
#43639=CARTESIAN_POINT ( 'NONE',  ( -119.5563837756079550, 43.64229894412654431, -38.37123407000066777 ) ) ;
#43640=CARTESIAN_POINT ( 'NONE',  ( -79.14094329813313777, 23.58034730000058232, 3.573650549209439919 ) ) ;
#43641=CARTESIAN_POINT ( 'NONE',  ( 86.62931800182293784, 20.48449268398423939, -77.66611478937542756 ) ) ;
#43643=CARTESIAN_POINT ( 'NONE',  ( -121.1841775822197889, 44.65790002524553870, -75.11573309556970912 ) ) ;
#43644=EDGE_CURVE ( 'NONE', #57348, #46836, #31348, .T. ) ;
#43645=CARTESIAN_POINT ( 'NONE',  ( 63.01563776193090405, 12.67277567978497643, 17.96841034875761878 ) ) ;
#43647=CARTESIAN_POINT ( 'NONE',  ( 88.53025347111697840, 21.14438024052372711, -23.74787560486554838 ) ) ;
#43652=CARTESIAN_POINT ( 'NONE',  ( 79.91920957766414801, 18.29292522273511779, -66.77815974945997368 ) ) ;
#43653=CARTESIAN_POINT ( 'NONE',  ( 117.4401308804713437, 33.48331296629643816, 88.66182713554364625 ) ) ;
#43654=CARTESIAN_POINT ( 'NONE',  ( -142.5087559769085033, 59.74468185400780129, 67.81411370576715569 ) ) ;
#43656=CARTESIAN_POINT ( 'NONE',  ( 70.45466089417030275, 14.52203022703029589, -15.38972110680052374 ) ) ;
#43657=CARTESIAN_POINT ( 'NONE',  ( -30.94745021534356511, 10.53010394565407637, -35.31719736520184227 ) ) ;
#43658=CARTESIAN_POINT ( 'NONE',  ( -55.05276343752909440, 15.72344139423347364, -62.06087458892354647 ) ) ;
#43659=CARTESIAN_POINT ( 'NONE',  ( -71.79230326678022323, 20.88638099735849352, -93.27200592928129197 ) ) ;
#43660=CARTESIAN_POINT ( 'NONE',  ( -118.4709174626548531, 42.97515378817185194, -14.46299016164537754 ) ) ;
#43661=EDGE_LOOP ( 'NONE', ( #43714, #29205, #35382, #68426 ) ) ;
#43662=EDGE_LOOP ( 'NONE', ( #13192, #854 ) ) ;
#43663=CARTESIAN_POINT ( 'NONE',  ( 32.29578462738145817, 8.602609172809792426, 66.66940855545223599 ) ) ;
#43664=CARTESIAN_POINT ( 'NONE',  ( 173.7246046907419554, 71.47482343504563573, 65.12733704930907663 ) ) ;
#43665=CARTESIAN_POINT ( 'NONE',  ( -166.2053056899074761, 81.18967388993343093, -18.28366721520819027 ) ) ;
#43666=EDGE_CURVE ( 'NONE', #54090, #67063, #36519, .T. ) ;
#43667=B_SPLINE_CURVE_WITH_KNOTS ( 'NONE', 3,
 ( #51284, #35445, #62165, #3774, #30510, #46682, #35094, #56546, #46329, #35796, #29469, #47032, #9060, #51625, #41759, #67135, #62871, #3432, #51963, #25247, #19967, #61816, #68158, #41418, #45655, #56199, #9406, #63216, #15019, #24897, #14672, #30174, #30865, #8017, #13988, #52308, #25597, #24209, #24559, #36136, #20294, #45993, #56906, #50928 ),
 .UNSPECIFIED., .F., .F.,
 ( 4, 2, 2, 2, 2, 2, 2, 2, 2, 2, 2, 2, 2, 2, 2, 2, 2, 2, 2, 2, 2, 4 ),
 ( 0.000000000000000000, 0.001487235713946774259, 0.002230853570920142415, 0.002974471427893510354, 0.004461707141840224981, 0.005948942855786940043, 0.007436178569733655104, 0.008179796426707028681, 0.008923414283680403125, 0.01041064999762720579, 0.01189788571157400672, 0.01264150356854738637, 0.01338512142552076602, 0.01487235713946755827, 0.01561597499644096394, 0.01635959285341436961, 0.01784682856736117748, 0.01933406428130798882, 0.02007768213828138928, 0.02082129999525479322, 0.02230853570920154905, 0.02379577142314830487 ),
 .UNSPECIFIED. ) ;
#43668=VECTOR ( 'NONE', #17851, 1000.000000000000000 ) ;
#43670=CARTESIAN_POINT ( 'NONE',  ( 63.01563776193091826, 13.70579113808095073, -23.87614024170608218 ) ) ;
#43673=CARTESIAN_POINT ( 'NONE',  ( 103.0124792097646207, 26.77148435100180990, -45.48088717822322735 ) ) ;
#43674=CARTESIAN_POINT ( 'NONE',  ( -14.55425570676089286, 7.423011834016143951, 67.78171509784250759 ) ) ;
#43675=CARTESIAN_POINT ( 'NONE',  ( -79.61931371420118353, 22.68640080971621487, -8.316616331170878951 ) ) ;
#43676=CARTESIAN_POINT ( 'NONE',  ( -81.56869946242737512, 24.53041000886392808, -89.37576505892265288 ) ) ;
#43679=FACE_BOUND ( 'NONE', #53968, .T. ) ;
#43680=CARTESIAN_POINT ( 'NONE',  ( -59.36813706141740710, 15.88103696331963732, -36.57740707826144444 ) ) ;
#43681=B_SPLINE_CURVE_WITH_KNOTS ( 'NONE', 3,
 ( #58028, #9846, #53072, #26023, #4225, #35544, #52407, #3524, #26367, #30269, #42536, #67905, #8818, #69267, #9155, #30961, #9500, #14437, #63989, #63313, #41167, #3876, #68912, #42197, #20385, #35887, #62961, #25345, #25692, #51718, #31307, #47120, #30613, #24996, #68584, #52063, #46427, #19704, #62626, #46781, #41855, #4560, #68252, #47453, #15121, #36582, #20057, #41509 ),
 .UNSPECIFIED., .F., .F.,
 ( 4, 2, 2, 2, 2, 2, 2, 2, 2, 2, 2, 2, 2, 2, 2, 2, 2, 2, 2, 2, 2, 2, 2, 4 ),
 ( 0.000000000000000000, 0.003619254076116538554, 0.004524067595145629499, 0.005428881114174720010, 0.007238508152232927054, 0.008143321671262040984, 0.009048135190291153179, 0.01085776222834930992, 0.01176257574737839783, 0.01266738926640748400, 0.01357220278543657017, 0.01447701630446565635, 0.01538182982349474426, 0.01628664334252383217, 0.01719145686155291661, 0.01809627038058200452, 0.01900108389961108896, 0.01990589741864017687, 0.02171552445669841513, 0.02262033797572753774, 0.02352515149475665687, 0.02533477853281489514, 0.02714440557087313688, 0.02895403260893137515 ),
 .UNSPECIFIED. ) ;
#43682=EDGE_LOOP ( 'NONE', ( #34751, #39908, #3680, #13819 ) ) ;
#43683=FACE_OUTER_BOUND ( 'NONE', #37485, .T. ) ;
#43684=DIRECTION ( 'NONE',  ( 0.000000000000000000, 0.000000000000000000, 1.000000000000000000 ) ) ;
#43685=CARTESIAN_POINT ( 'NONE',  ( -48.23766733091050440, 13.99378332280059389, 67.80282971881165111 ) ) ;
#43688=CARTESIAN_POINT ( 'NONE',  ( -4.374019708349202951, 7.698173713297786769, 84.63809582392633502 ) ) ;
#43690=CARTESIAN_POINT ( 'NONE',  ( 56.30011474572734187, 11.21470186335419505, 7.119764699933178953 ) ) ;
#43694=CARTESIAN_POINT ( 'NONE',  ( -79.14678386417814693, 22.50468917936073154, -61.96000122218156747 ) ) ;
#43696=CARTESIAN_POINT ( 'NONE',  ( 109.7724924842965635, 28.66436020578542099, 44.61121420573732621 ) ) ;
#43699=DIRECTION ( 'NONE',  ( 0.000000000000000000, 0.000000000000000000, 1.000000000000000000 ) ) ;
#43700=AXIS2_PLACEMENT_3D ( 'NONE', #26013, #15109, #14067 ) ;
#43701=CARTESIAN_POINT ( 'NONE',  ( 159.6614743841975042, 60.66237087206238243, 29.72267884793179960 ) ) ;
#43703=CARTESIAN_POINT ( 'NONE',  ( 66.30636076182547356, 14.49616748423542134, 17.22552420475900448 ) ) ;
#43704=CARTESIAN_POINT ( 'NONE',  ( 91.51282003084290295, 21.14522045960330132, 42.92523528589520510 ) ) ;
#43705=EDGE_CURVE ( 'NONE', #15521, #41738, #37188, .T. ) ;
#43706=CARTESIAN_POINT ( 'NONE',  ( 107.2614272668149482, 28.62909081796206934, -9.691944018085198564 ) ) ;
#43709=CARTESIAN_POINT ( 'NONE',  ( -153.7711962260935650, 69.23055119419213099, -89.82806832391398189 ) ) ;
#43710=CARTESIAN_POINT ( 'NONE',  ( 70.26840926437850499, 14.47268499222803584, -95.00000000000133582 ) ) ;
#43712=CARTESIAN_POINT ( 'NONE',  ( 93.57270713017220487, 21.90807125275457423, 93.81897079287583097 ) ) ;
#43713=CYLINDRICAL_SURFACE ( 'NONE', #36633, 7.500000000000020428 ) ;
#43714=ORIENTED_EDGE ( 'NONE', *, *, #16522, .F. ) ;
#43719=CARTESIAN_POINT ( 'NONE',  ( -165.8134318330274652, 80.78594366325573617, 90.28324896190464699 ) ) ;
#43723=CARTESIAN_POINT ( 'NONE',  ( -61.52761555060400411, 17.56359742150277725, -46.53362156671873606 ) ) ;
#43724=EDGE_CURVE ( 'NONE', #52360, #34095, #52818, .T. ) ;
#43725=CARTESIAN_POINT ( 'NONE',  ( -11.79249160485393233, 8.191429102467060019, -9.703845154134903339 ) ) ;
#43734=CARTESIAN_POINT ( 'NONE',  ( 117.7237061126833026, 32.49927938580613329, 91.44293783028797407 ) ) ;
#43737=CARTESIAN_POINT ( 'NONE',  ( -95.63568360745009045, 29.53168204475776193, -46.00256717322782407 ) ) ;
#43738=CARTESIAN_POINT ( 'NONE',  ( -109.7816385129979011, 36.75776661907241305, 10.67383622189045767 ) ) ;
#43739=CARTESIAN_POINT ( 'NONE',  ( 22.89634831467700948, 6.832298124325685507, 39.92007651388386336 ) ) ;
#43740=CARTESIAN_POINT ( 'NONE',  ( 141.3586046882815026, 47.34625111366350581, -17.18765650132280953 ) ) ;
#43746=CARTESIAN_POINT ( 'NONE',  ( -10.46803069297986433, 7.077485182625209426, 17.79433764303042764 ) ) ;
#43747=CARTESIAN_POINT ( 'NONE',  ( 55.90536342106782541, 11.13510150712953539, -18.81323374408498950 ) ) ;
#43748=EDGE_CURVE ( 'NONE', #60940, #44163, #26103, .T. ) ;
#43753=EDGE_CURVE ( 'NONE', #34598, #44611, #4557, .T. ) ;
#43755=EDGE_CURVE ( 'NONE', #34459, #34109, #16259, .T. ) ;
#43756=CARTESIAN_POINT ( 'NONE',  ( 188.5842358232186200, 88.03712271786932320, 63.35372157011578764 ) ) ;
#43759=CARTESIAN_POINT ( 'NONE',  ( -1.455067768715155418, 7.566780179921179794, -38.95200498131430322 ) ) ;
#43761=CARTESIAN_POINT ( 'NONE',  ( -80.31691774066410971, 22.95709084517032039, -35.29547712760505362 ) ) ;
#43762=CARTESIAN_POINT ( 'NONE',  ( 16.77391662606469325, 6.533867394142987450, 71.81064437024208758 ) ) ;
#43763=LINE ( 'NONE', #23392, #29846 ) ;
#43764=CARTESIAN_POINT ( 'NONE',  ( 14.80582440982707482, 6.470883766728822373, -62.41208511885447052 ) ) ;
#43769=DIRECTION ( 'NONE',  ( -1.000000000000000000, 0.000000000000000000, 0.000000000000000000 ) ) ;
#43772=CARTESIAN_POINT ( 'NONE',  ( 61.09977118998600076, 13.26754120022605044, -77.32048710585367246 ) ) ;
#43774=B_SPLINE_CURVE_WITH_KNOTS ( 'NONE', 3,
 ( #66954, #54981, #18061, #38821, #13474, #50754, #66271, #7517, #12087, #2234, #18398, #49695, #39513, #29644, #44790, #55329, #28969, #7153, #60961, #29301, #8196, #1525, #39854, #1893, #2574, #22988, #45474, #34602, #51109, #12782, #24031, #34244, #61312, #45126, #23683, #23347, #60269, #50414, #13137, #28614, #6799, #2919, #50063, #61655 ),
 .UNSPECIFIED., .F., .F.,
 ( 4, 2, 2, 2, 2, 2, 2, 2, 2, 2, 2, 2, 2, 2, 2, 2, 2, 2, 2, 2, 2, 4 ),
 ( 1.440969542111313559E-17, 0.001533942663855621677, 0.003067885327711229043, 0.004601827991566837493, 0.005368799323494641285, 0.006135770655422445943, 0.007669713319278085618, 0.008436684651205906757, 0.009203655983133728763, 0.01073759864698935890, 0.01150456997891717396, 0.01227154131084498556, 0.01303851264277279542, 0.01380548397470060355, 0.01533942663855623195, 0.01687336930241186209, 0.01840731196626749222, 0.01994125463012312235, 0.02070822596205093569, 0.02147519729397874902, 0.02300913995783437915, 0.02454308262169000582 ),
 .UNSPECIFIED. ) ;
#43776=CARTESIAN_POINT ( 'NONE',  ( -133.3122825023497171, 51.57669324886579432, -95.00000000000133582 ) ) ;
#43780=CARTESIAN_POINT ( 'NONE',  ( 177.0024338932394414, 74.57605685449961186, -37.41665159782565553 ) ) ;
#43783=CARTESIAN_POINT ( 'NONE',  ( 117.7417271423230147, 33.63613196344608269, 64.49092239129596749 ) ) ;
#43784=CARTESIAN_POINT ( 'NONE',  ( 140.7888851157409817, 46.97220912571251716, 66.72935928051445842 ) ) ;
#43785=CARTESIAN_POINT ( 'NONE',  ( -71.16770070143911653, 19.60548673929830343, -43.14023053854354828 ) ) ;
#43786=CARTESIAN_POINT ( 'NONE',  ( 63.01563776193090405, 13.70579113808097738, 44.81296093922130552 ) ) ;
#43787=CARTESIAN_POINT ( 'NONE',  ( 91.51282003084287453, 21.14522045960330132, -37.60841648549585159 ) ) ;
#43788=CARTESIAN_POINT ( 'NONE',  ( -48.58011387679029269, 14.07568064779664141, -19.66872259271415757 ) ) ;
#43789=EDGE_CURVE ( 'NONE', #50390, #10221, #35452, .T. ) ;
#43790=ORIENTED_EDGE ( 'NONE', *, *, #22416, .F. ) ;
#43798=CARTESIAN_POINT ( 'NONE',  ( 61.08522853873729730, 13.26388801693373409, 17.73216832077243410 ) ) ;
#43799=AXIS2_PLACEMENT_3D ( 'NONE', #25525, #51559, #14268 ) ;
#43801=CARTESIAN_POINT ( 'NONE',  ( -144.7571537022064376, 60.25265659240449168, 59.25656382279842660 ) ) ;
#43803=CARTESIAN_POINT ( 'NONE',  ( 86.62931800182292363, 20.48449268398425716, -89.51066537983906812 ) ) ;
#43806=CARTESIAN_POINT ( 'NONE',  ( 92.95016907945944240, 22.74936990452174967, 33.16759907785775141 ) ) ;
#43807=EDGE_CURVE ( 'NONE', #41847, #62155, #56509, .T. ) ;
#43808=CARTESIAN_POINT ( 'NONE',  ( 80.30232379693107703, 17.35837133860831827, -20.51189838118990494 ) ) ;
#43809=CARTESIAN_POINT ( 'NONE',  ( 46.90170507415072620, 10.52318308703818062, 11.06461444427903373 ) ) ;
#43810=CARTESIAN_POINT ( 'NONE',  ( 93.63037639125408873, 21.92981100938039063, -67.46451625388530715 ) ) ;
#43812=CARTESIAN_POINT ( 'NONE',  ( -156.4819242240389769, 70.32841519459755375, -93.23206903001478452 ) ) ;
#43816=CARTESIAN_POINT ( 'NONE',  ( 42.70988075781784232, 8.862408058333477001, 30.66516676936959485 ) ) ;
#43817=CARTESIAN_POINT ( 'NONE',  ( 12.69192874957005124, 6.421326776602847453, 30.67927649405437407 ) ) ;
#43819=CARTESIAN_POINT ( 'NONE',  ( -78.66644367742111399, -170.0000000000000000, -42.61545063171789849 ) ) ;
#43821=CARTESIAN_POINT ( 'NONE',  ( 211.4997502125519020, 118.0043045815490501, -46.99967683100181404 ) ) ;
#43824=CARTESIAN_POINT ( 'NONE',  ( -125.4463376280758951, 47.40387005565906975, 30.62991178436581663 ) ) ;
#43825=LINE ( 'NONE', #44888, #66689 ) ;
#43826=ORIENTED_EDGE ( 'NONE', *, *, #59156, .T. ) ;
#43827=CARTESIAN_POINT ( 'NONE',  ( 133.8566784816069060, 42.60093787723653236, 2.665790248531674678 ) ) ;
#43829=CARTESIAN_POINT ( 'NONE',  ( -9.763294602873864747, 7.024900256480052896, -35.66858442679837538 ) ) ;
#43830=DIRECTION ( 'NONE',  ( 0.000000000000000000, 0.000000000000000000, 1.000000000000000000 ) ) ;
#43831=CARTESIAN_POINT ( 'NONE',  ( 87.58754341703161117, 20.81465688423119431, 71.51040371463716383 ) ) ;
#43832=CARTESIAN_POINT ( 'NONE',  ( 129.4887940973039520, 40.01039828304091373, 43.12603597457647453 ) ) ;
#43840=CARTESIAN_POINT ( 'NONE',  ( 210.3791065492700909, 114.4724634728603121, 85.49048150234845878 ) ) ;
#43845=CARTESIAN_POINT ( 'NONE',  ( -13.45956523846225039, 8.333781915634244086, 5.814511151728004812 ) ) ;
#43847=CARTESIAN_POINT ( 'NONE',  ( 45.76405797021009647, 10.34101216371941767, -65.98511464492352729 ) ) ;
#43848=CARTESIAN_POINT ( 'NONE',  ( -4.725257700475992806, 6.708862164351558910, 44.44922483199589891 ) ) ;
#43850=CARTESIAN_POINT ( 'NONE',  ( 94.05217532500763866, 23.16464989206124159, 89.77431030042610871 ) ) ;
#43856=CARTESIAN_POINT ( 'NONE',  ( -172.3127615181935823, 87.73358064377643473, -49.67956037655144996 ) ) ;
#43860=B_SPLINE_CURVE_WITH_KNOTS ( 'NONE', 3,
 ( #29917, #67904, #58027, #46780, #63312, #9845, #41853, #24305, #51377, #30611, #9499, #14083, #25691, #47119, #20055, #9154, #15119, #40464, #61908, #41508, #3193, #3522, #14767, #24995, #35543, #46084, #67554, #19702, #56999, #40809, #30268, #46426, #36920, #11203, #59394, #31635, #48139, #42861, #41200, #37945, #64331, #663, #64684, #15802, #15467, #22113, #26707, #10175, #16142, #43205, #37594, #303, #32672, #43557, #21417, #47452, #65030, #32334 ),
 .UNSPECIFIED., .F., .F.,
 ( 4, 2, 2, 2, 2, 2, 2, 2, 2, 2, 2, 2, 2, 2, 2, 2, 2, 2, 2, 2, 2, 2, 2, 2, 2, 2, 2, 2, 4 ),
 ( 0.000000000000000000, 0.002011202885851239280, 0.003016804328776875616, 0.004022405771702512386, 0.005028007214628148723, 0.006033608657553785060, 0.007039210100479421396, 0.008044811543405057733, 0.009050412986330693202, 0.01005601442925633041, 0.01206721731510760308, 0.01307281875803323855, 0.01407842020095887402, 0.01508402164388450949, 0.01608962308681014669, 0.01709522452973578216, 0.01810082597266142110, 0.02011202885851270244, 0.02111763030143834138, 0.02212323174436398379, 0.02312883318728962620, 0.02413443463021526514, 0.02514003607314090755, 0.02614563751606654649, 0.02715123895899218889, 0.02815684040191783130, 0.03016804328776911265, 0.03117364473069475159, 0.03217924617362039746 ),
 .UNSPECIFIED. ) ;
#43863=CARTESIAN_POINT ( 'NONE',  ( -7.336630171688593549, 7.867399454768214895, -77.26262132240753999 ) ) ;
#43864=LINE ( 'NONE', #43520, #43668 ) ;
#43867=CARTESIAN_POINT ( 'NONE',  ( 199.3671895066314619, 99.30947926630328482, -49.12614233709344802 ) ) ;
#43871=EDGE_LOOP ( 'NONE', ( #51104, #47458, #13954, #9051 ) ) ;
#43874=EDGE_LOOP ( 'NONE', ( #13904, #11184, #13400, #8848 ) ) ;
#43875=CARTESIAN_POINT ( 'NONE',  ( -125.0772643754502411, 45.95811963572885617, -88.63583198122191220 ) ) ;
#43877=DIRECTION ( 'NONE',  ( -0.000000000000000000, 1.000000000000000000, -0.000000000000000000 ) ) ;
#43878=CARTESIAN_POINT ( 'NONE',  ( -12.39770133248888584, 8.241491894828993026, -75.72815778851469304 ) ) ;
#43883=CARTESIAN_POINT ( 'NONE',  ( -76.33235143960693847, 22.51916353135074900, -35.48390396204494124 ) ) ;
#43889=CARTESIAN_POINT ( 'NONE',  ( -38.93922791710218689, 10.94334660650242341, -16.21455789437017359 ) ) ;
#43891=CARTESIAN_POINT ( 'NONE',  ( -35.99019277275119322, 10.38248800679341954, -63.68048773888882153 ) ) ;
#43892=EDGE_CURVE ( 'NONE', #14549, #33459, #24632, .T. ) ;
#43893=CARTESIAN_POINT ( 'NONE',  ( 23.28845814680232351, 7.864847136539610872, 63.87262545100447397 ) ) ;
#43900=CARTESIAN_POINT ( 'NONE',  ( 86.62931800182293784, -170.0000000000000000, -77.66611478937542756 ) ) ;
#43902=CARTESIAN_POINT ( 'NONE',  ( -31.43908319763709258, 9.591432048623767415, -35.31719736520183517 ) ) ;
#43906=CARTESIAN_POINT ( 'NONE',  ( -62.39620438142541303, 17.82550490656933917, 89.94779769255055157 ) ) ;
#43907=CARTESIAN_POINT ( 'NONE',  ( 86.15410276028856629, 19.25894675708889991, 56.55663816294299551 ) ) ;
#43908=ORIENTED_EDGE ( 'NONE', *, *, #22078, .F. ) ;
#43911=CARTESIAN_POINT ( 'NONE',  ( 212.0850679406003678, 117.0583048437722340, -69.33104460838883654 ) ) ;
#43912=B_SPLINE_CURVE_WITH_KNOTS ( 'NONE', 3,
 ( #551, #38180, #59620, #38894, #11434, #22355, #17058, #11790, #33272, #27976, #49419, #17414, #60337, #28321, #33622, #6871, #67709, #62065, #62424, #24109, #29042, #18821, #8626, #7922, #66681, #13547, #55763, #35002, #50827, #12861, #46233, #56445, #50483, #2305, #45200, #34670, #3336, #23419, #24795, #66341 ),
 .UNSPECIFIED., .F., .F.,
 ( 4, 2, 2, 2, 2, 2, 2, 2, 2, 2, 2, 2, 2, 2, 2, 2, 2, 2, 2, 4 ),
 ( 0.02454308262168999541, 0.02608670964102888234, 0.02685852315069834143, 0.02763033666036780051, 0.02917396367970670826, 0.02994577718937616387, 0.03071759069904561948, 0.03226121771838449948, 0.03303303122805391345, 0.03380484473772334131, 0.03534847175706214845, 0.03689209877640095558, 0.03843572579573976272, 0.03997935281507856986, 0.04152297983441737700, 0.04306660685375618414, 0.04461023387309499821, 0.04615386089243381229, 0.04769748791177262637, 0.04924111493111144044 ),
 .UNSPECIFIED. ) ;
#43915=CARTESIAN_POINT ( 'NONE',  ( 37.47081272996201307, 8.166145978397519656, 17.82054918726932513 ) ) ;
#43916=CARTESIAN_POINT ( 'NONE',  ( -49.11825192196924661, 13.17012322555988213, 15.58522413457026623 ) ) ;
#43918=CARTESIAN_POINT ( 'NONE',  ( 157.4703587214989113, 58.92748579479258808, -77.96873488960135035 ) ) ;
#43923=LINE ( 'NONE', #60112, #21850 ) ;
#43930=CARTESIAN_POINT ( 'NONE',  ( 132.0582325211144905, 40.34869848118181324, -9.383526223381995379 ) ) ;
#43939=CARTESIAN_POINT ( 'NONE',  ( 56.30011474572734187, 11.21470186335419683, 60.80886588086055156 ) ) ;
#43940=CARTESIAN_POINT ( 'NONE',  ( -2.873329055852808622, 7.626065826870669362, 58.80573367209430558 ) ) ;
#43944=FILL_AREA_STYLE_COLOUR ( '', #45168 ) ;
#43947=CARTESIAN_POINT ( 'NONE',  ( -124.1094910780272329, 45.33021696310841975, -76.54648126837901145 ) ) ;
#43951=DIRECTION ( 'NONE',  ( -0.000000000000000000, 0.000000000000000000, -1.000000000000000000 ) ) ;
#43953=CARTESIAN_POINT ( 'NONE',  ( 135.6647932137617829, 43.70902528961477884, 17.45871630207848924 ) ) ;
#43958=CARTESIAN_POINT ( 'NONE',  ( 82.94943325692328528, 18.19803534719806848, 3.827846601591828879 ) ) ;
#43961=CARTESIAN_POINT ( 'NONE',  ( -78.18913509716432486, 22.13995206110505976, 45.41820113967313688 ) ) ;
#43962=ORIENTED_EDGE ( 'NONE', *, *, #66545, .F. ) ;
#43964=CARTESIAN_POINT ( 'NONE',  ( 127.3650620767373738, 37.64047374603843110, -93.43272312347599495 ) ) ;
#43966=CARTESIAN_POINT ( 'NONE',  ( -124.7710763417278486, 46.96042092553522451, 3.856429859304379093 ) ) ;
#43967=CARTESIAN_POINT ( 'NONE',  ( 90.31682503704259091, 20.71196693118262644, 16.91658005194965142 ) ) ;
#43971=CARTESIAN_POINT ( 'NONE',  ( 36.09469435220862010, 9.015003538710487874, 30.66481460161145378 ) ) ;
#43972=CARTESIAN_POINT ( 'NONE',  ( -179.8989115484066303, 96.59045402602905028, -38.98901376945831032 ) ) ;
#43973=CARTESIAN_POINT ( 'NONE',  ( -128.1384526288949814, 47.98891607499720635, -22.74005215996440299 ) ) ;
#43980=CARTESIAN_POINT ( 'NONE',  ( -149.5074843970971017, 65.50121172469319220, -76.65738112195568021 ) ) ;
#43984=FACE_BOUND ( 'NONE', #23160, .T. ) ;
#43985=CARTESIAN_POINT ( 'NONE',  ( -4.725257700476004352, 6.708862164351561574, -62.92897752985880544 ) ) ;
#43990=CYLINDRICAL_SURFACE ( 'NONE', #59086, 7.500000000000013323 ) ;
#43991=DIRECTION ( 'NONE',  ( 0.000000000000000000, 0.000000000000000000, 1.000000000000000000 ) ) ;
#43993=CARTESIAN_POINT ( 'NONE',  ( -123.6618353044034819, 46.23845779494351405, -76.43322633536396893 ) ) ;
#43994=VECTOR ( 'NONE', #47280, 1000.000000000000000 ) ;
#43995=CARTESIAN_POINT ( 'NONE',  ( -13.77312480593389310, 8.361845410302541026, 33.04005123776303066 ) ) ;
#43997=CARTESIAN_POINT ( 'NONE',  ( 163.1495034066983294, 62.20479872133084598, 14.98979888773876468 ) ) ;
#43998=CARTESIAN_POINT ( 'NONE',  ( 93.72687053612524721, 23.04134601640626911, -18.95203141322158658 ) ) ;
#44000=CARTESIAN_POINT ( 'NONE',  ( -37.52119286077852678, 11.69341290629619934, 6.476620693246999849 ) ) ;
#44004=CARTESIAN_POINT ( 'NONE',  ( 103.9212167174977282, 27.16063360973579321, 86.75032792527655090 ) ) ;
#44006=CARTESIAN_POINT ( 'NONE',  ( 68.45098769362923008, 13.99935947269946368, -21.54976275930446405 ) ) ;
#44008=CARTESIAN_POINT ( 'NONE',  ( -23.93895920923072396, 9.495000752338448535, -43.05927999758113600 ) ) ;
#44011=CARTESIAN_POINT ( 'NONE',  ( -119.1605144823340225, 43.39823405392969846, -18.88291338966152466 ) ) ;
#44014=CARTESIAN_POINT ( 'NONE',  ( 36.99999522780155559, 9.122638774496635961, 57.14919926213968182 ) ) ;
#44015=CARTESIAN_POINT ( 'NONE',  ( 177.7960900018545090, 75.34533826015461955, 70.39765848647137148 ) ) ;
#44016=CARTESIAN_POINT ( 'NONE',  ( 110.2429982417149432, 28.88204397445230853, -89.61153874658103291 ) ) ;
#44018=CARTESIAN_POINT ( 'NONE',  ( -169.8885678771097787, 85.07765565657315676, -22.14949854782897987 ) ) ;
#44021=CARTESIAN_POINT ( 'NONE',  ( 110.2429982417149574, 29.99119854320846201, -50.92243756565370916 ) ) ;
#44022=CARTESIAN_POINT ( 'NONE',  ( 188.2086267457325448, 87.61890531228284829, -19.24083152260686447 ) ) ;
#44023=CARTESIAN_POINT ( 'NONE',  ( -85.34215807311488788, 24.97769003780923924, -12.34335653950498646 ) ) ;
#44026=CARTESIAN_POINT ( 'NONE',  ( 204.6977192012829789, 106.3443248447423173, -9.481380442157895772 ) ) ;
#44027=FACE_BOUND ( 'NONE', #19530, .T. ) ;
#44028=CARTESIAN_POINT ( 'NONE',  ( -61.52143283897135007, 16.51181063611435107, -46.52005420056815410 ) ) ;
#44031=CARTESIAN_POINT ( 'NONE',  ( 92.53033045403537926, 22.59263332688195547, -47.97690888582502566 ) ) ;
#44032=AXIS2_PLACEMENT_3D ( 'NONE', #26752, #37290, #16876 ) ;
#44033=CARTESIAN_POINT ( 'NONE',  ( -51.13576748034040520, 14.70354244225167406, 58.26138747146119101 ) ) ;
#44035=CARTESIAN_POINT ( 'NONE',  ( 152.8430172091322845, 54.14068524174417973, 4.157737500947386700 ) ) ;
#44036=CARTESIAN_POINT ( 'NONE',  ( -102.2801239173131194, -170.0000000000000000, -35.01457726497591239 ) ) ;
#44040=CARTESIAN_POINT ( 'NONE',  ( 57.39083379741712321, 11.43779987330584191, 5.482692190092026685 ) ) ;
#44042=EDGE_CURVE ( 'NONE', #25434, #40816, #16127, .T. ) ;
#44045=VERTEX_POINT ( 'NONE', #33183 ) ;
#44048=ADVANCED_FACE ( 'NONE', ( #22619 ), #28600, .F. ) ;
#44049=CARTESIAN_POINT ( 'NONE',  ( 90.30732934992394689, 21.77797012484621320, -63.61215870629216340 ) ) ;
#44052=VERTEX_POINT ( 'NONE', #50051 ) ;
#44054=CARTESIAN_POINT ( 'NONE',  ( 164.0105905242218682, 64.23277447906895077, 33.22940987375192634 ) ) ;
#44055=CARTESIAN_POINT ( 'NONE',  ( -154.0833774771448930, 69.51012195447344766, -63.19600284746142194 ) ) ;
#44056=CARTESIAN_POINT ( 'NONE',  ( 68.62997155117723480, 15.08415013720829378, 15.46527518503070731 ) ) ;
#44058=CARTESIAN_POINT ( 'NONE',  ( 103.1534365798308102, 26.83148826706845824, -14.07784702132055443 ) ) ;
#44060=CARTESIAN_POINT ( 'NONE',  ( -133.3799602664182373, 52.86209125874978554, -15.03899668926757549 ) ) ;
#44064=CARTESIAN_POINT ( 'NONE',  ( 90.10670619348783816, 20.63680950852241125, 84.24788275468904430 ) ) ;
#44065=FACE_OUTER_BOUND ( 'NONE', #5671, .T. ) ;
#44066=ORIENTED_EDGE ( 'NONE', *, *, #43344, .F. ) ;
#44068=EDGE_LOOP ( 'NONE', ( #7075, #14587 ) ) ;
#44069=CARTESIAN_POINT ( 'NONE',  ( -10.23867141318105745, 7.059827648235816433, -23.19163774689041091 ) ) ;
#44070=CARTESIAN_POINT ( 'NONE',  ( -165.6444900061506758, 80.61247689992478627, 91.39031826811293513 ) ) ;
#44073=CARTESIAN_POINT ( 'NONE',  ( -57.42826130032239007, 16.37596353166459906, -49.83430089818286035 ) ) ;
#44075=CARTESIAN_POINT ( 'NONE',  ( -74.19961951691011848, 20.67022044985850826, -75.48968614315221259 ) ) ;
#44087=LINE ( 'NONE', #38477, #30452 ) ;
#44088=DIRECTION ( 'NONE',  ( 0.000000000000000000, 0.000000000000000000, 1.000000000000000000 ) ) ;
#44089=CARTESIAN_POINT ( 'NONE',  ( 141.3556389957210229, 47.34429831367557284, -16.38285624325062528 ) ) ;
#44095=CARTESIAN_POINT ( 'NONE',  ( -9.525868120571907127, 7.007646177566257961, 18.07979315870208481 ) ) ;
#44098=CARTESIAN_POINT ( 'NONE',  ( 55.76298701799387203, 11.10663440745154062, -14.40127503394189645 ) ) ;
#44101=EDGE_LOOP ( 'NONE', ( #26142, #56499, #16458, #31691 ) ) ;
#44103=CARTESIAN_POINT ( 'NONE',  ( 204.3129818922373602, 107.5244029525888294, -78.17048162308530834 ) ) ;
#44106=CARTESIAN_POINT ( 'NONE',  ( -1.454841858088672613, 7.566772088227303072, -46.88363903783812248 ) ) ;
#44107=CARTESIAN_POINT ( 'NONE',  ( 103.1653143050726271, 25.74301230421574971, 12.79924877302471842 ) ) ;
#44108=CARTESIAN_POINT ( 'NONE',  ( -166.3175803736862406, 79.86140754556167565, 14.64531061278483293 ) ) ;
#44109=CARTESIAN_POINT ( 'NONE',  ( -81.67992981004169906, 23.49232121719083821, -49.48758314069756636 ) ) ;
#44110=FACE_BOUND ( 'NONE', #22528, .T. ) ;
#44114=CARTESIAN_POINT ( 'NONE',  ( -126.3508039230933093, 46.79479538767115798, -61.75825448869760947 ) ) ;
#44115=CARTESIAN_POINT ( 'NONE',  ( -128.7810612886106298, 48.42424427998341940, -49.33947501303506300 ) ) ;
#44116=CARTESIAN_POINT ( 'NONE',  ( -125.8938041572051105, 47.69968343338781835, -34.91370389823391918 ) ) ;
#44118=VERTEX_POINT ( 'NONE', #65903 ) ;
#44120=CARTESIAN_POINT ( 'NONE',  ( -102.2801239173131194, -170.0000000000000000, 38.01907450641511588 ) ) ;
#44121=CARTESIAN_POINT ( 'NONE',  ( -55.05276343752910151, -170.0000000000000000, -23.37177340799619785 ) ) ;
#44122=EDGE_CURVE ( 'NONE', #39310, #34701, #32951, .T. ) ;
#44129=CARTESIAN_POINT ( 'NONE',  ( 113.4418023215250173, 31.50656691678297605, 57.15562911881430352 ) ) ;
#44131=CARTESIAN_POINT ( 'NONE',  ( -71.67841390531691559, 19.78168466957078309, -45.35036129474283229 ) ) ;
#44134=CARTESIAN_POINT ( 'NONE',  ( -102.2801239173131194, 33.91021738430207222, -35.01457726497591239 ) ) ;
#44137=CARTESIAN_POINT ( 'NONE',  ( -54.56685407443681157, 15.59259313022788085, -8.371773407996171201 ) ) ;
#44140=DIRECTION ( 'NONE',  ( -0.8160245890732938934, -0.5780171883497599028, 0.000000000000000000 ) ) ;
#44143=EDGE_CURVE ( 'NONE', #50735, #780, #57254, .T. ) ;
#44144=CARTESIAN_POINT ( 'NONE',  ( -147.3669217311067996, 63.69361261596463919, -49.50424762432383119 ) ) ;
#44148=LINE ( 'NONE', #21317, #17321 ) ;
#44153=CARTESIAN_POINT ( 'NONE',  ( -144.2188519266539970, 59.82027639618912929, 59.74168973493228663 ) ) ;
#44154=CYLINDRICAL_SURFACE ( 'NONE', #60380, 7.500000000000013323 ) ;
#44157=CARTESIAN_POINT ( 'NONE',  ( 85.67138972405901143, 19.09593469918316089, -23.93094700892396887 ) ) ;
#44163=VERTEX_POINT ( 'NONE', #37663 ) ;
#44164=CARTESIAN_POINT ( 'NONE',  ( 46.84183314611287585, 9.494161546644496852, 38.39310041101741433 ) ) ;
#44166=DIRECTION ( 'NONE',  ( -0.000000000000000000, 1.000000000000000000, -0.000000000000000000 ) ) ;
#44167=CARTESIAN_POINT ( 'NONE',  ( -190.4968431727838833, 108.8425311198514862, 61.08946333816734153 ) ) ;
#44168=CARTESIAN_POINT ( 'NONE',  ( 208.5936709733498446, 113.6229123546138169, -50.24872299381472374 ) ) ;
#44169=CARTESIAN_POINT ( 'NONE',  ( -71.57025115638938928, 20.80908992785613520, -71.93917367057966317 ) ) ;
#44170=CARTESIAN_POINT ( 'NONE',  ( -109.7647482398635645, 36.74843029291201191, 65.41115726635926819 ) ) ;
#44171=CARTESIAN_POINT ( 'NONE',  ( -28.81317668042939317, 9.175023678939295380, -49.84668732688152915 ) ) ;
#44174=CARTESIAN_POINT ( 'NONE',  ( -25.49247221749737591, 9.706368398275740716, 15.46881133980917333 ) ) ;
#44178=CARTESIAN_POINT ( 'NONE',  ( -83.28416304016923277, 24.13400259533326775, 85.66394350348330988 ) ) ;
#44179=CARTESIAN_POINT ( 'NONE',  ( -83.69653436244857403, 24.30167057287990673, 70.33125617411978681 ) ) ;
#44180=CARTESIAN_POINT ( 'NONE',  ( 131.6115093721024891, 41.25402743071402512, 29.85055241671198090 ) ) ;
#44181=CARTESIAN_POINT ( 'NONE',  ( 33.75794032130627187, 8.754084575552406378, 15.53265863234151212 ) ) ;
#44189=EDGE_LOOP ( 'NONE', ( #5401, #27767 ) ) ;
#44192=CARTESIAN_POINT ( 'NONE',  ( -14.84452950307166041, 8.460866451887698148, 8.117316759835038198 ) ) ;
#44197=CARTESIAN_POINT ( 'NONE',  ( 86.33664277319749658, 20.38412364599995641, 83.39993048091545802 ) ) ;
#44199=AXIS2_PLACEMENT_3D ( 'NONE', #3310, #15250, #63437 ) ;
#44202=AXIS2_PLACEMENT_3D ( 'NONE', #33746, #11224, #5601 ) ;
#44204=CARTESIAN_POINT ( 'NONE',  ( -129.6001310305489369, 48.98284622040326042, 17.79976323783206027 ) ) ;
#44207=CARTESIAN_POINT ( 'NONE',  ( -167.1169587990081595, 80.68480154570059426, 87.50472330615433236 ) ) ;
#44210=CARTESIAN_POINT ( 'NONE',  ( -6.840981040171511651, 6.828436339979224279, -8.621995243679700494 ) ) ;
#44212=CARTESIAN_POINT ( 'NONE',  ( -149.5074843970971017, 64.17983161892348676, -22.96827994102829962 ) ) ;
#44213=CARTESIAN_POINT ( 'NONE',  ( -0.3732240621745021025, 7.527003275829101447, -68.78330978471883839 ) ) ;
#44216=ADVANCED_FACE ( 'NONE', ( #9914 ), #734, .F. ) ;
#44218=CARTESIAN_POINT ( 'NONE',  ( 161.0086191018871205, 61.75036325654523495, -90.68964922113312355 ) ) ;
#44219=CARTESIAN_POINT ( 'NONE',  ( 197.3685896092616190, 96.80423329231987850, -45.44928297951660312 ) ) ;
#44220=CARTESIAN_POINT ( 'NONE',  ( -94.78138776532239262, 30.24234841992714706, 38.55512063273754109 ) ) ;
#44221=EDGE_CURVE ( 'NONE', #61334, #49747, #55632, .T. ) ;
#44223=CARTESIAN_POINT ( 'NONE',  ( 112.1009898303695849, 30.86414810229296890, 17.54788357748616789 ) ) ;
#44228=CARTESIAN_POINT ( 'NONE',  ( -71.21970990337017327, 19.62334883444992784, -16.79706233958787820 ) ) ;
#44229=DIRECTION ( 'NONE',  ( -0.8118923937861950435, -0.5838071093367415143, 0.000000000000000000 ) ) ;
#44231=CARTESIAN_POINT ( 'NONE',  ( -11.14668121284976543, 8.139398342256731311, -63.03362835402993625 ) ) ;
#44233=CARTESIAN_POINT ( 'NONE',  ( 164.8886903222557407, 63.65672212134879260, 35.77000457521792498 ) ) ;
#44238=VECTOR ( 'NONE', #50091, 1000.000000000000114 ) ;
#44241=CARTESIAN_POINT ( 'NONE',  ( -142.8234585218669679, 59.99418748542435509, -92.56481087250594442 ) ) ;
#44245=CARTESIAN_POINT ( 'NONE',  ( 150.6506100456012973, 52.53711661296497226, -94.16253627988041330 ) ) ;
#44248=CARTESIAN_POINT ( 'NONE',  ( 19.54326199789020890, 7.657220834818547317, 57.86229037013161758 ) ) ;
#44254=CARTESIAN_POINT ( 'NONE',  ( -48.33978239863299819, 12.98353572341707363, 88.09987427823563166 ) ) ;
#44257=CARTESIAN_POINT ( 'NONE',  ( -101.1432610527352836, 32.20700799924091484, 84.28889895904916330 ) ) ;
#44261=CARTESIAN_POINT ( 'NONE',  ( 79.82127737190242556, 17.20935440217363066, 60.90020036238115608 ) ) ;
#44263=CARTESIAN_POINT ( 'NONE',  ( -173.5143455280199873, 87.56649811480131973, -88.40105834567731335 ) ) ;
#44268=DIRECTION ( 'NONE',  ( -0.000000000000000000, 1.000000000000000000, -0.000000000000000000 ) ) ;
#44269=CARTESIAN_POINT ( 'NONE',  ( -118.5151419614604720, 43.00218563933587035, 66.33403389341971490 ) ) ;
#44270=CARTESIAN_POINT ( 'NONE',  ( -52.66507163626137356, 14.05394608175174653, 18.09895399749082401 ) ) ;
#44271=CARTESIAN_POINT ( 'NONE',  ( 151.1873096904021452, 52.92629247302096474, -39.52043524289759802 ) ) ;
#44272=CARTESIAN_POINT ( 'NONE',  ( 161.7006237583813402, 62.31514460450497950, -76.67892487292121473 ) ) ;
#44276=ORIENTED_EDGE ( 'NONE', *, *, #23826, .F. ) ;
#44281=CARTESIAN_POINT ( 'NONE',  ( 155.2870855780214754, 57.23765125306422163, -63.27940277120605828 ) ) ;
#44285=ORIENTED_EDGE ( 'NONE', *, *, #38935, .T. ) ;
#44293=CARTESIAN_POINT ( 'NONE',  ( -5.183193881612056408, 7.740932022135017299, 17.79449844124656011 ) ) ;
#44296=EDGE_CURVE ( 'NONE', #4538, #44045, #21981, .T. ) ;
#44298=AXIS2_PLACEMENT_3D ( 'NONE', #31871, #63195, #53651 ) ;
#44303=CARTESIAN_POINT ( 'NONE',  ( -118.6288898061518609, 41.89286798341289852, -71.14046227876613671 ) ) ;
#44310=CARTESIAN_POINT ( 'NONE',  ( 141.3403471770513420, 46.13063628128489313, -70.93045427954361060 ) ) ;
#44313=CARTESIAN_POINT ( 'NONE',  ( 80.17205177205137545, 17.31791394718354837, 6.544383460469372693 ) ) ;
#44315=CARTESIAN_POINT ( 'NONE',  ( 13.14401442664831166, 6.430459733718342008, 44.53740620683903018 ) ) ;
#44319=CARTESIAN_POINT ( 'NONE',  ( -145.3279998500303236, 60.71393190715790666, -75.38937528560870760 ) ) ;
#44326=CARTESIAN_POINT ( 'NONE',  ( 70.29000978231910324, 15.51935254053008251, 92.85854150907050553 ) ) ;
#44327=CARTESIAN_POINT ( 'NONE',  ( 36.08914434112043779, 9.014684630517862729, 44.14699482183696944 ) ) ;
#44328=CARTESIAN_POINT ( 'NONE',  ( -177.1381400275771796, 93.26609858452819424, -48.56046632885807668 ) ) ;
#44329=CARTESIAN_POINT ( 'NONE',  ( -132.2199390322348904, 50.80243550247269013, -11.50942145384449766 ) ) ;
#44331=DIRECTION ( 'NONE',  ( -0.000000000000000000, 1.000000000000000000, -0.000000000000000000 ) ) ;
#44333=DIRECTION ( 'NONE',  ( 0.000000000000000000, 0.000000000000000000, 1.000000000000000000 ) ) ;
#44336=CARTESIAN_POINT ( 'NONE',  ( -156.9900125991010498, 72.16580261738673130, -42.89949303315771090 ) ) ;
#44337=CARTESIAN_POINT ( 'NONE',  ( -2.174378755909785355, 6.588636630831476104, -64.80724674333109192 ) ) ;
#44338=AXIS2_PLACEMENT_3D ( 'NONE', #2662, #24122, #33637 ) ;
#44340=CARTESIAN_POINT ( 'NONE',  ( -175.9864315813574080, 91.91454246454364352, 58.22230986313539347 ) ) ;
#44341=CARTESIAN_POINT ( 'NONE',  ( 14.94351112032491002, 7.480372597427133563, -89.20804527961313113 ) ) ;
#44342=CARTESIAN_POINT ( 'NONE',  ( -122.8011284400168108, 45.68452922414293482, -49.26186152409542274 ) ) ;
#44343=CARTESIAN_POINT ( 'NONE',  ( 181.0840389613909736, -170.0000000000000000, -9.380507075415927432 ) ) ;
#44347=CARTESIAN_POINT ( 'NONE',  ( -119.2804658695888236, 43.47213805166349943, -72.80517393614263710 ) ) ;
#44349=CARTESIAN_POINT ( 'NONE',  ( -9.524904342798459211, 8.016391612076533946, 30.30652578697153388 ) ) ;
#44350=CARTESIAN_POINT ( 'NONE',  ( 117.4696399285658686, 32.37118663718647582, 8.193927448285345250 ) ) ;
#44351=CARTESIAN_POINT ( 'NONE',  ( 151.3976820382521851, -170.0000000000000000, 94.99999999999866418 ) ) ;
#44352=ORIENTED_EDGE ( 'NONE', *, *, #58111, .F. ) ;
#44353=CARTESIAN_POINT ( 'NONE',  ( -38.88884187334146247, 11.95889603743730234, 9.875062609561268800 ) ) ;
#44355=DIRECTION ( 'NONE',  ( 0.000000000000000000, 0.000000000000000000, 1.000000000000000000 ) ) ;
#44356=CARTESIAN_POINT ( 'NONE',  ( 79.52639011421919690, 18.17129627604989750, -67.70599084128726020 ) ) ;
#44357=CARTESIAN_POINT ( 'NONE',  ( 117.0726165202673172, 33.29780331829707762, 87.68152807156005224 ) ) ;
#44359=CARTESIAN_POINT ( 'NONE',  ( -14.67600094096871111, 7.434177657339199108, 94.42751904206191682 ) ) ;
#44360=CARTESIAN_POINT ( 'NONE',  ( -26.88635117726413171, 9.904687797303052932, -36.83709584847830598 ) ) ;
#44363=LINE ( 'NONE', #65846, #38685 ) ;
#44364=CARTESIAN_POINT ( 'NONE',  ( 133.8566784816069344, -170.0000000000000000, 37.01034083899534721 ) ) ;
#44367=EDGE_CURVE ( 'NONE', #67063, #54901, #6919, .T. ) ;
#44374=DIRECTION ( 'NONE',  ( -0.000000000000000000, 1.000000000000000000, -0.000000000000000000 ) ) ;
#44375=VERTEX_POINT ( 'NONE', #25328 ) ;
#44376=CARTESIAN_POINT ( 'NONE',  ( 107.0555969502564437, 28.53646637607230829, -50.22783466578279388 ) ) ;
#44377=CARTESIAN_POINT ( 'NONE',  ( -11.57808265946730231, 7.164483090579921942, 57.96183666591232253 ) ) ;
#44378=CARTESIAN_POINT ( 'NONE',  ( -86.15441609607630369, 25.31657638323078174, -16.26595699322537314 ) ) ;
#44380=CYLINDRICAL_SURFACE ( 'NONE', #4873, 7.500000000000013323 ) ;
#44381=CARTESIAN_POINT ( 'NONE',  ( 210.1954643503415241, 114.1986276268023772, -11.87401850716117124 ) ) ;
#44382=FACE_BOUND ( 'NONE', #2762, .T. ) ;
#44383=CARTESIAN_POINT ( 'NONE',  ( -60.66241560458681192, 16.25736033771447353, -47.71895337534586190 ) ) ;
#44390=CARTESIAN_POINT ( 'NONE',  ( 90.30840373526892506, 21.77864858272153725, -49.86167802567979379 ) ) ;
#44392=CARTESIAN_POINT ( 'NONE',  ( -48.58011387679029980, 14.07568064779664674, 60.86492917867685293 ) ) ;
#44393=CARTESIAN_POINT ( 'NONE',  ( 86.62931800182292363, 19.42108912189597092, 44.71208757247933363 ) ) ;
#44394=CARTESIAN_POINT ( 'NONE',  ( 212.0075063341773784, 118.7912820769029594, 61.84339564076807960 ) ) ;
#44395=DIRECTION ( 'NONE',  ( -0.000000000000000000, 1.000000000000000000, -0.000000000000000000 ) ) ;
#44401=CARTESIAN_POINT ( 'NONE',  ( -14.35185884954381308, -170.0000000000000000, 94.99999999999866418 ) ) ;
#44407=CARTESIAN_POINT ( 'NONE',  ( -62.50103539982528389, 17.85731685071833752, -16.88267018884844362 ) ) ;
#44408=CARTESIAN_POINT ( 'NONE',  ( 88.28889510440060917, 21.05995314109331318, -62.84815687393930972 ) ) ;
#44410=ORIENTED_EDGE ( 'NONE', *, *, #33673, .T. ) ;
#44414=CARTESIAN_POINT ( 'NONE',  ( 108.3942953861066627, 29.14039925067523384, 2.982985333465853373 ) ) ;
#44415=CARTESIAN_POINT ( 'NONE',  ( 69.83260694998128315, 15.39825517924929699, 13.60525356106382766 ) ) ;
#44418=CARTESIAN_POINT ( 'NONE',  ( 109.7732660198864494, 29.77277639096406148, -9.077886975189999319 ) ) ;
#44419=CARTESIAN_POINT ( 'NONE',  ( -54.08816720029308556, 15.46531105893041591, 18.42599816275528113 ) ) ;
#44420=CARTESIAN_POINT ( 'NONE',  ( -128.3448054685827344, 49.34430406923177514, -22.66102150948377769 ) ) ;
#44421=CARTESIAN_POINT ( 'NONE',  ( 14.80291736570134375, 7.477373894757628037, 44.96613339589305269 ) ) ;
#44423=B_SPLINE_CURVE_WITH_KNOTS ( 'NONE', 3,
 ( #31271, #14402, #4186, #64913, #9464, #20022, #15082, #41477, #36544, #47085, #52369, #43436, #57993, #67868, #68549, #30232, #63620, #57653, #9812, #41125, #20698, #20350, #35852, #41819, #16707, #46389, #57306, #9116, #36888, #38165, #52698, #19665, #4525, #25990, #30574, #52024, #46740, #47419, #53977, #59606, #5804, #68873, #51681, #42158, #68213, #58323, #11084, #27258 ),
 .UNSPECIFIED., .F., .F.,
 ( 4, 2, 2, 2, 2, 2, 2, 2, 2, 2, 2, 2, 2, 2, 2, 2, 2, 2, 2, 2, 2, 2, 2, 4 ),
 ( 0.000000000000000000, 0.003619254076116462226, 0.004524067595145588733, 0.005428881114174714806, 0.007238508152232894094, 0.008143321671262013228, 0.009048135190291132363, 0.01085776222834935155, 0.01176257574737844466, 0.01266738926640753778, 0.01357220278543663089, 0.01447701630446572400, 0.01538182982349481885, 0.01628664334252390850, 0.01719145686155300334, 0.01809627038058209819, 0.01900108389961118957, 0.01990589741864028095, 0.02171552445669847412, 0.02262033797572757937, 0.02352515149475668810, 0.02533477853281489861, 0.02714440557087311259, 0.02895403260893131964 ),
 .UNSPECIFIED. ) ;
#44424=CARTESIAN_POINT ( 'NONE',  ( 92.18363589146608206, 21.39143322710240724, 85.85047583112388736 ) ) ;
#44429=CARTESIAN_POINT ( 'NONE',  ( -15.32520546926283345, 7.495995523981876296, -15.58064402833840489 ) ) ;
#44430=CARTESIAN_POINT ( 'NONE',  ( -171.2900812578366754, 86.60412786162308407, 84.73309799929434405 ) ) ;
#44431=CARTESIAN_POINT ( 'NONE',  ( -52.45215874217870322, 13.99961488531757148, -22.91060012390807543 ) ) ;
#44433=CARTESIAN_POINT ( 'NONE',  ( -56.02289203441037557, 15.98631679403370320, -35.26344691231105344 ) ) ;
#44435=CARTESIAN_POINT ( 'NONE',  ( 181.0840389613909736, 78.60582251573003987, -36.22505766587961062 ) ) ;
#44436=CARTESIAN_POINT ( 'NONE',  ( -15.26524495591508845, 7.490231452641283205, 36.63582166737488421 ) ) ;
#44440=ORIENTED_EDGE ( 'NONE', *, *, #38350, .F. ) ;
#44443=AXIS2_PLACEMENT_3D ( 'NONE', #62007, #18412, #52152 ) ;
#44444=CARTESIAN_POINT ( 'NONE',  ( -55.26629345812349925, 15.78094189665235980, -88.90542517938722256 ) ) ;
#44445=CARTESIAN_POINT ( 'NONE',  ( -166.0031475600389115, 80.98114714564768235, 40.70217298635069625 ) ) ;
#44446=CARTESIAN_POINT ( 'NONE',  ( 116.9197133427646804, 33.22079464767576695, -20.03184353198292911 ) ) ;
#44461=CARTESIAN_POINT ( 'NONE',  ( -12.77647591501652791, 7.263973827022344842, 5.115775066274252936 ) ) ;
#44462=PLANE ( 'NONE',  #3045 ) ;
#44464=CARTESIAN_POINT ( 'NONE',  ( 56.53635105806415595, 11.26263375223563656, -20.16170768551763004 ) ) ;
#44468=CARTESIAN_POINT ( 'NONE',  ( 204.3091227790963273, 107.5190503136782922, 71.05227132923317868 ) ) ;
#44470=CARTESIAN_POINT ( 'NONE',  ( -58.75378739419587504, 16.75118858561005908, -76.10252817049797613 ) ) ;
#44471=CARTESIAN_POINT ( 'NONE',  ( 200.8303160266298732, 102.8412051751308809, -64.23028300416009984 ) ) ;
#44473=CARTESIAN_POINT ( 'NONE',  ( -0.7211439451572430048, 7.539282923622932842, -40.50150818776037909 ) ) ;
#44474=CARTESIAN_POINT ( 'NONE',  ( 127.7121523762017858, 38.99241938113798511, 94.99999999999866418 ) ) ;
#44475=CARTESIAN_POINT ( 'NONE',  ( -166.4832242797243964, 80.03142989439328403, -92.40010354986478092 ) ) ;
#44476=LINE ( 'NONE', #34639, #48646 ) ;
#44482=CARTESIAN_POINT ( 'NONE',  ( -133.3765738414514601, 51.62252165471728205, -68.68159762529066370 ) ) ;
#44483=CARTESIAN_POINT ( 'NONE',  ( -104.1225399044495816, 34.86084180570099278, -76.63309873828038121 ) ) ;
#44484=CARTESIAN_POINT ( 'NONE',  ( 46.42281973867196143, 9.426811321855161907, -67.31512451460598356 ) ) ;
#44489=CARTESIAN_POINT ( 'NONE',  ( 180.0913586328219083, 77.60790998934250240, 83.05812134022308157 ) ) ;
#44493=CARTESIAN_POINT ( 'NONE',  ( 174.6127059037622473, 72.30368563770915102, -47.55541787117397234 ) ) ;
#44494=CARTESIAN_POINT ( 'NONE',  ( -173.9656771507954431, 88.06879734510549440, -61.55650775521367990 ) ) ;
#44496=ORIENTED_EDGE ( 'NONE', *, *, #59844, .F. ) ;
#44499=CARTESIAN_POINT ( 'NONE',  ( -180.5230320745700681, 95.76406004447549947, 10.22830062411841290 ) ) ;
#44505=CARTESIAN_POINT ( 'NONE',  ( -189.9638655956220816, 108.0957249433520957, 35.19133789206601648 ) ) ;
#44508=ORIENTED_EDGE ( 'NONE', *, *, #13989, .T. ) ;
#44509=B_SPLINE_CURVE_WITH_KNOTS ( 'NONE', 3,
 ( #58957, #37160, #52646, #25929, #69167, #37857, #58607, #10772, #53325, #5155, #32242, #21672, #7604, #22372, #54721, #27992, #43812, #55420, #49788, #17438 ),
 .UNSPECIFIED., .F., .F.,
 ( 4, 2, 2, 2, 2, 2, 2, 2, 2, 4 ),
 ( 0.01250143415648050441, 0.01409579223316451656, 0.01489297127150652350, 0.01569015030984852871, 0.01887886646321665363, 0.02047322453990072649, 0.02206758261658480283, 0.02286476165492683926, 0.02366194069326887917, 0.02525629876995295203 ),
 .UNSPECIFIED. ) ;
#44512=CARTESIAN_POINT ( 'NONE',  ( -71.57025115638937507, 20.80908992785612455, 8.594478100811356214 ) ) ;
#44514=CARTESIAN_POINT ( 'NONE',  ( -146.5230751932348312, 62.99205605665035534, -49.20801219754704192 ) ) ;
#44515=CARTESIAN_POINT ( 'NONE',  ( -170.2856292770789253, 85.50720222068220266, -76.01299923972814554 ) ) ;
#44516=CARTESIAN_POINT ( 'NONE',  ( -132.3337749658410871, 50.88291293015778649, 87.95154732409349663 ) ) ;
#44517=EDGE_LOOP ( 'NONE', ( #51307, #40515, #59180, #1434 ) ) ;
#44520=CARTESIAN_POINT ( 'NONE',  ( -142.9728934044261734, 58.82891228489262403, 61.34574771090444756 ) ) ;
#44524=CARTESIAN_POINT ( 'NONE',  ( 183.1865184929770578, 80.75677158533827082, -24.08296830964977531 ) ) ;
#44525=CARTESIAN_POINT ( 'NONE',  ( 139.7928618793173143, 45.12615179300589574, -12.08803966520795825 ) ) ;
#44526=CARTESIAN_POINT ( 'NONE',  ( 41.34269507549199574, 9.685203600174691729, 3.308298053325811949 ) ) ;
#44530=VERTEX_POINT ( 'NONE', #43803 ) ;
#44532=CARTESIAN_POINT ( 'NONE',  ( 41.81982603358024875, 8.735900550613191484, 44.53007514971749004 ) ) ;
#44533=CARTESIAN_POINT ( 'NONE',  ( -55.05276343752909440, 15.72344139423348430, 18.47277718246750311 ) ) ;
#44536=CARTESIAN_POINT ( 'NONE',  ( 211.3710169359753763, 117.8057917113659272, -47.26017629441455625 ) ) ;
#44537=CARTESIAN_POINT ( 'NONE',  ( -71.42546113164834765, 20.75891408601218302, -67.44120922730739665 ) ) ;
#44539=DIRECTION ( 'NONE',  ( 0.000000000000000000, 0.000000000000000000, 1.000000000000000000 ) ) ;
#44540=CARTESIAN_POINT ( 'NONE',  ( 163.7464701930790056, 62.69993100427431898, -74.60574447506652973 ) ) ;
#44545=ORIENTED_EDGE ( 'NONE', *, *, #17513, .F. ) ;
#44547=CARTESIAN_POINT ( 'NONE',  ( -71.74169950304127497, 19.80353288478602636, 88.65348869463956305 ) ) ;
#44548=CARTESIAN_POINT ( 'NONE',  ( -85.90441187606242579, 25.21188850826090544, 66.79256356289977248 ) ) ;
#44549=CARTESIAN_POINT ( 'NONE',  ( 133.8566784816069060, 42.60093787723652525, 44.51034083899536142 ) ) ;
#44554=CARTESIAN_POINT ( 'NONE',  ( -95.04371414958066566, 30.36527049547256141, -17.70897442121572141 ) ) ;
#44557=CARTESIAN_POINT ( 'NONE',  ( 34.30379848636039952, 7.801021882850803557, 85.59205753501402114 ) ) ;
#44558=DIRECTION ( 'NONE',  ( 0.000000000000000000, 0.000000000000000000, 1.000000000000000000 ) ) ;
#44566=CARTESIAN_POINT ( 'NONE',  ( 129.1310456962234809, 39.80382822048402858, -22.52299050009668591 ) ) ;
#44571=CARTESIAN_POINT ( 'NONE',  ( -38.45778834351241926, 11.87434869453507247, -40.16219554672893821 ) ) ;
#44572=CARTESIAN_POINT ( 'NONE',  ( -165.7140086129056442, 80.68381997492572566, -43.42740335534784180 ) ) ;
#44573=CARTESIAN_POINT ( 'NONE',  ( -172.7827862703479411, 86.75267914668864933, 84.51416791675012519 ) ) ;
#44575=CARTESIAN_POINT ( 'NONE',  ( -118.6288898061518609, 41.89286798341291274, -44.29591168830246062 ) ) ;
#44577=CARTESIAN_POINT ( 'NONE',  ( -143.7151964745329735, 59.41799441280382155, -20.23954929768048316 ) ) ;
#44578=CARTESIAN_POINT ( 'NONE',  ( -0.3255842968951683791, 7.525381170773409956, -69.27034146520422553 ) ) ;
#44579=B_SPLINE_CURVE_WITH_KNOTS ( 'NONE', 3,
 ( #25769, #32067, #68330, #26099, #3957, #68655, #63393, #52814, #69352, #20130, #15883, #53503, #58781, #42276, #9581, #9234, #30689, #41583, #15547, #46508, #31381, #63038, #15199, #25074, #36312, #36998, #68991, #4635, #36659, #31717, #19787, #53149, #26449, #47886, #54187, #16226, #32418, #21848, #49265, #38736, #16916, #32757, #49615, #6008 ),
 .UNSPECIFIED., .F., .F.,
 ( 4, 2, 2, 2, 2, 2, 2, 2, 2, 2, 2, 2, 2, 2, 2, 2, 2, 2, 2, 2, 2, 4 ),
 ( 1.430489624538199204E-17, 0.003433139681083844253, 0.004291424601354751865, 0.005149709521625661646, 0.006866279362167396205, 0.007724564282438266954, 0.008582849202709135969, 0.009441134122980008453, 0.01029941904325087920, 0.01201598888379266580, 0.01373255872433445587, 0.01459084364460534744, 0.01544912856487623554, 0.01630741348514712710, 0.01716569840541801520, 0.01888226824595979486, 0.02059883808650157105, 0.02145712300677249038, 0.02231540792704340276, 0.02403197776758514773, 0.02574854760812689616, 0.02746511744866864113 ),
 .UNSPECIFIED. ) ;
#44581=VERTEX_POINT ( 'NONE', #20370 ) ;
#44582=CARTESIAN_POINT ( 'NONE',  ( -62.30163634902122993, 17.79682011226253380, 8.984685373998656743 ) ) ;
#44583=CARTESIAN_POINT ( 'NONE',  ( 198.7084915431530021, 98.47675983942190214, -48.34816613409072517 ) ) ;
#44585=CARTESIAN_POINT ( 'NONE',  ( 17.74393407086869345, 6.570779001277776032, -35.76153089853740141 ) ) ;
#44586=CARTESIAN_POINT ( 'NONE',  ( 110.2429982417149574, 29.99119854320843714, 17.76666361527367499 ) ) ;
#44590=EDGE_LOOP ( 'NONE', ( #23713, #40425 ) ) ;
#44592=CARTESIAN_POINT ( 'NONE',  ( 175.5498284945444425, 74.57669191966279243, 31.72087837615354644 ) ) ;
#44594=DIRECTION ( 'NONE',  ( 0.000000000000000000, 0.000000000000000000, 1.000000000000000000 ) ) ;
#44598=CARTESIAN_POINT ( 'NONE',  ( -31.43908319763709969, 9.591432048623756756, -89.00629854612920155 ) ) ;
#44604=AXIS2_PLACEMENT_3D ( 'NONE', #38542, #38192, #54353 ) ;
#44605=CARTESIAN_POINT ( 'NONE',  ( -31.43908319763709969, 9.591432048623758533, -23.47264677473818395 ) ) ;
#44607=CARTESIAN_POINT ( 'NONE',  ( -133.0921934900200085, 52.65587531157185452, 13.39783114184680457 ) ) ;
#44608=CARTESIAN_POINT ( 'NONE',  ( 22.62427395637551086, 7.823784829753559933, 61.26417510860944304 ) ) ;
#44609=ORIENTED_EDGE ( 'NONE', *, *, #23229, .T. ) ;
#44610=ORIENTED_EDGE ( 'NONE', *, *, #19714, .F. ) ;
#44611=VERTEX_POINT ( 'NONE', #68896 ) ;
#44613=CARTESIAN_POINT ( 'NONE',  ( -106.7004823116342322, 36.22460663120047286, 17.25249706529000449 ) ) ;
#44614=DIRECTION ( 'NONE',  ( 0.000000000000000000, 0.000000000000000000, 1.000000000000000000 ) ) ;
#44616=CARTESIAN_POINT ( 'NONE',  ( -37.38262509017739177, 10.64263598035110547, -38.21638920231944070 ) ) ;
#44617=CARTESIAN_POINT ( 'NONE',  ( -95.27094040074264569, 29.36050931297059208, 94.39711218672647419 ) ) ;
#44621=CARTESIAN_POINT ( 'NONE',  ( -71.17984086584780812, 20.67393782512343492, -15.25595357977673139 ) ) ;
#44622=ORIENTED_EDGE ( 'NONE', *, *, #10339, .F. ) ;
#44623=CARTESIAN_POINT ( 'NONE',  ( 79.19345177405118363, 17.01649702043280499, 65.06721247038061051 ) ) ;
#44626=CARTESIAN_POINT ( 'NONE',  ( 39.40195752203892710, 8.409560354027384221, 44.91383430596327742 ) ) ;
#44629=CARTESIAN_POINT ( 'NONE',  ( 187.2465631085773907, 85.06582225041682932, 41.11322305146563849 ) ) ;
#44632=CARTESIAN_POINT ( 'NONE',  ( -121.1841775822197746, 44.65790002524553870, 59.10701985674870684 ) ) ;
#44633=CARTESIAN_POINT ( 'NONE',  ( -7.825402957745083654, 6.891034867348166060, 30.11558103944718923 ) ) ;
#44639=CARTESIAN_POINT ( 'NONE',  ( -102.7007063459125789, 32.99469082455791380, -88.70367844590325035 ) ) ;
#44640=DIRECTION ( 'NONE',  ( 0.000000000000000000, 0.000000000000000000, 1.000000000000000000 ) ) ;
#44643=CARTESIAN_POINT ( 'NONE',  ( -7.825402957745085430, -170.0000000000000000, 3.271030448983517136 ) ) ;
#44646=CARTESIAN_POINT ( 'NONE',  ( -85.10774223992956422, 24.88053943842882987, 34.06813972546618174 ) ) ;
#44648=CARTESIAN_POINT ( 'NONE',  ( 62.04326772936978784, 12.44884401098615534, -50.67314713297363937 ) ) ;
#44650=CARTESIAN_POINT ( 'NONE',  ( -26.87327614295024603, 8.886070347947313763, 70.53135286019491446 ) ) ;
#44652=AXIS2_PLACEMENT_3D ( 'NONE', #2267, #66992, #32959 ) ;
#44653=ORIENTED_EDGE ( 'NONE', *, *, #21909, .T. ) ;
#44662=CARTESIAN_POINT ( 'NONE',  ( 32.66883187925818532, 8.640402022338111721, -19.61546109960840667 ) ) ;
#44664=CARTESIAN_POINT ( 'NONE',  ( -4.502148936856955608, 7.704491846230414609, 17.51250421026318094 ) ) ;
#44665=CARTESIAN_POINT ( 'NONE',  ( -6.840165690716692559, 7.836465889224641046, 57.00902819645234842 ) ) ;
#44672=CARTESIAN_POINT ( 'NONE',  ( 164.3702714028688376, 63.22112480708620552, -13.82798321502299110 ) ) ;
#44674=CARTESIAN_POINT ( 'NONE',  ( 66.72974708835177182, 13.56459745268607087, 57.62319218809916066 ) ) ;
#44675=CARTESIAN_POINT ( 'NONE',  ( 136.9934874058117771, 43.35050367224292955, -63.53966939834757000 ) ) ;
#44678=VERTEX_POINT ( 'NONE', #7598 ) ;
#44679=CARTESIAN_POINT ( 'NONE',  ( 8.480442907658519047, 6.376693431076495777, 39.21954576350441357 ) ) ;
#44681=CARTESIAN_POINT ( 'NONE',  ( 64.69738688745238164, 14.10375742873388560, 71.47051169446849883 ) ) ;
#44683=EDGE_LOOP ( 'NONE', ( #37142, #9769, #53642, #56261 ) ) ;
#44684=CARTESIAN_POINT ( 'NONE',  ( 86.62931800182293784, 20.48449268398423584, 17.86753698201564688 ) ) ;
#44688=AXIS2_PLACEMENT_3D ( 'NONE', #12149, #893, #65620 ) ;
#44690=CARTESIAN_POINT ( 'NONE',  ( 70.50468489774748093, 15.57653925086012769, 91.52810434581883214 ) ) ;
#44693=CARTESIAN_POINT ( 'NONE',  ( 66.94365390260637128, 14.65531706601760042, 30.91923626730180530 ) ) ;
#44694=CARTESIAN_POINT ( 'NONE',  ( -179.9693807058584980, 96.67690106241352055, -92.83178401929812651 ) ) ;
#44695=CARTESIAN_POINT ( 'NONE',  ( 154.4550750032601627, 55.34393534448157226, 70.62503253431717098 ) ) ;
#44696=CARTESIAN_POINT ( 'NONE',  ( 126.5880720616305553, 37.20544379858409911, -68.50076568904083274 ) ) ;
#44697=ORIENTED_EDGE ( 'NONE', *, *, #5490, .T. ) ;
#44700=ORIENTED_EDGE ( 'NONE', *, *, #39488, .F. ) ;
#44704=CARTESIAN_POINT ( 'NONE',  ( -35.17718245314462422, 11.25729435722175786, 44.22309306491955283 ) ) ;
#44705=CARTESIAN_POINT ( 'NONE',  ( -196.7348448768811409, -170.0000000000000000, 92.11166915431037694 ) ) ;
#44706=DIRECTION ( 'NONE',  ( 0.000000000000000000, 0.000000000000000000, 1.000000000000000000 ) ) ;
#44708=CARTESIAN_POINT ( 'NONE',  ( -55.05276343752909440, 14.68156374112637863, -62.06087458892354647 ) ) ;
#44710=CARTESIAN_POINT ( 'NONE',  ( -0.3252226420479323310, 7.525368746738509529, -16.56025891687170315 ) ) ;
#44712=CARTESIAN_POINT ( 'NONE',  ( -15.07533778868020491, 8.482826962130840087, 39.55181792566148857 ) ) ;
#44713=CARTESIAN_POINT ( 'NONE',  ( 110.7114632166112358, 29.09878355652111992, 2.766663615273642129 ) ) ;
#44715=CARTESIAN_POINT ( 'NONE',  ( -48.39213801251012370, 14.03057237515049138, -92.93003639517210956 ) ) ;
#44717=CARTESIAN_POINT ( 'NONE',  ( -102.2801239173131052, 33.91021738430207222, -50.01457726497594081 ) ) ;
#44721=CARTESIAN_POINT ( 'NONE',  ( 79.63513233364423627, 18.20496177163923690, -72.88516583624812029 ) ) ;
#44722=CARTESIAN_POINT ( 'NONE',  ( 46.64694836521738353, 9.462741877720629802, 62.30350966403887725 ) ) ;
#44723=DIRECTION ( 'NONE',  ( -0.8160245890732938934, -0.5780171883497599028, 0.000000000000000000 ) ) ;
#44727=CARTESIAN_POINT ( 'NONE',  ( 61.40682472845701767, 13.33642729942792649, -89.57322748555588987 ) ) ;
#44728=CARTESIAN_POINT ( 'NONE',  ( -119.9771613955297624, 43.90337778233484300, -20.18511414558994943 ) ) ;
#44729=ORIENTED_EDGE ( 'NONE', *, *, #29550, .T. ) ;
#44733=CARTESIAN_POINT ( 'NONE',  ( 41.04173437458232598, 8.628130879747104132, -89.47880143737668845 ) ) ;
#44734=CARTESIAN_POINT ( 'NONE',  ( -165.9121868482145601, 80.88751546905562861, 63.07590250008146882 ) ) ;
#44736=CARTESIAN_POINT ( 'NONE',  ( -172.7173255566597163, 88.18461381371099606, -22.86740657428632773 ) ) ;
#44741=CARTESIAN_POINT ( 'NONE',  ( 108.3942953861066485, 29.14039925067522319, -50.70611584746151834 ) ) ;
#44742=CARTESIAN_POINT ( 'NONE',  ( 16.77104078056616032, 7.540619757007627655, -35.56757450759191386 ) ) ;
#44743=CARTESIAN_POINT ( 'NONE',  ( -85.46258339457288855, 25.02772366257409686, -18.95299861283113074 ) ) ;
#44745=CARTESIAN_POINT ( 'NONE',  ( 212.0047492081760083, 116.9348962082588343, -18.70236844209925309 ) ) ;
#44746=FACE_BOUND ( 'NONE', #9985, .T. ) ;
#44748=CARTESIAN_POINT ( 'NONE',  ( -62.45356936877016096, 16.79156452995240656, -43.95760844768815190 ) ) ;
#44754=DIRECTION ( 'NONE',  ( -0.000000000000000000, 1.000000000000000000, -0.000000000000000000 ) ) ;
#44756=CARTESIAN_POINT ( 'NONE',  ( 212.0803491126036704, 118.9047894217573287, 64.91680770945086465 ) ) ;
#44760=CARTESIAN_POINT ( 'NONE',  ( 62.04326772936978784, 12.44884401098615534, 3.015954047953714579 ) ) ;
#44761=CARTESIAN_POINT ( 'NONE',  ( -60.97727891098333686, 16.35024395194892932, 60.03668883463657124 ) ) ;
#44762=VERTEX_POINT ( 'NONE', #50148 ) ;
#44767=CARTESIAN_POINT ( 'NONE',  ( 93.08073375333746924, 22.79826000593200774, -73.99913914800674775 ) ) ;
#44770=CARTESIAN_POINT ( 'NONE',  ( 42.71680114082827373, 9.880016734137541334, 71.00390679014272166 ) ) ;
#44772=CARTESIAN_POINT ( 'NONE',  ( -156.9232798886536671, 72.10386843399172108, -70.31426418089215247 ) ) ;
#44773=CARTESIAN_POINT ( 'NONE',  ( 70.41705859591012029, 15.55317472777717747, 9.231046305453860512 ) ) ;
#44778=CARTESIAN_POINT ( 'NONE',  ( -50.53243683205841563, 14.55237037207940531, 16.97720090376005686 ) ) ;
#44779=CARTESIAN_POINT ( 'NONE',  ( -130.5811943660945076, 50.88295841537573239, -21.44378994887165391 ) ) ;
#44781=CARTESIAN_POINT ( 'NONE',  ( 112.1012908502484464, 29.75117929736499889, -23.84786912706831785 ) ) ;
#44785=ORIENTED_EDGE ( 'NONE', *, *, #36605, .T. ) ;
#44788=CARTESIAN_POINT ( 'NONE',  ( 175.0696098417090809, 74.11936424544845181, 5.476034315764515270 ) ) ;
#44789=CARTESIAN_POINT ( 'NONE',  ( -49.43915770973591606, 13.24768844696975023, -10.87398376146266799 ) ) ;
#44790=CARTESIAN_POINT ( 'NONE',  ( 103.8317086685000135, 26.02720265156214197, -12.67800310554697241 ) ) ;
#44791=CARTESIAN_POINT ( 'NONE',  ( 199.3671895066314903, 99.30947926630329903, 4.562958843833921030 ) ) ;
#44793=CARTESIAN_POINT ( 'NONE',  ( 203.9193081356078494, 106.9838505030258489, 82.93253388923811542 ) ) ;
#44794=CARTESIAN_POINT ( 'NONE',  ( 110.2429982417149574, -170.0000000000000000, -70.26698815611737814 ) ) ;
#44795=CYLINDRICAL_SURFACE ( 'NONE', #15182, 7.500000000000013323 ) ;
#44796=CARTESIAN_POINT ( 'NONE',  ( -10.23402954931276554, 7.059791383763806216, 44.72254900470105810 ) ) ;
#44804=CARTESIAN_POINT ( 'NONE',  ( -147.7895256390024201, 64.04409735547015714, 18.73124213477483480 ) ) ;
#44806=CARTESIAN_POINT ( 'NONE',  ( -38.92978047220073279, 11.96698587041122330, 91.90144494392491481 ) ) ;
#44808=AXIS2_PLACEMENT_3D ( 'NONE', #1756, #40079, #45704 ) ;
#44811=CARTESIAN_POINT ( 'NONE',  ( 39.40195752203892710, 8.409560354027389550, 18.06928371549960133 ) ) ;
#44817=CARTESIAN_POINT ( 'NONE',  ( -15.26524495591508845, 7.490231452641285870, 9.791271076911209903 ) ) ;
#44820=CARTESIAN_POINT ( 'NONE',  ( -52.68007207639879397, 14.05813534436549972, 30.69840203706294446 ) ) ;
#44821=CARTESIAN_POINT ( 'NONE',  ( 199.7291770695760817, 101.4092159658447088, 69.17564586952617844 ) ) ;
#44824=CARTESIAN_POINT ( 'NONE',  ( 204.6977192012829789, 108.0580384837235073, -63.17048162308526571 ) ) ;
#44826=CARTESIAN_POINT ( 'NONE',  ( -4.072522659361693442, 7.683023425615342461, -49.41625453459061390 ) ) ;
#44827=CARTESIAN_POINT ( 'NONE',  ( -166.3188283541503267, 79.86268666707380248, 8.306259562134265195 ) ) ;
#44829=FACE_BOUND ( 'NONE', #24709, .T. ) ;
#44839=CARTESIAN_POINT ( 'NONE',  ( 187.9868792055843585, 85.87520301053052663, 93.45502771267183562 ) ) ;
#44843=CARTESIAN_POINT ( 'NONE',  ( -178.7458319892713803, 93.61502008198020519, -64.08897040876379947 ) ) ;
#44846=CARTESIAN_POINT ( 'NONE',  ( 115.7731501832036400, 32.64791439093736614, 58.86561899071531911 ) ) ;
#44853=CARTESIAN_POINT ( 'NONE',  ( -47.65155309726506516, 13.85482731128120193, -17.11044809809313705 ) ) ;
#44860=CARTESIAN_POINT ( 'NONE',  ( 44.34263167748004264, 9.103379693481560508, -48.78358003831574052 ) ) ;
#44861=DIRECTION ( 'NONE',  ( 0.000000000000000000, -1.000000000000000000, 0.000000000000000000 ) ) ;
#44862=CARTESIAN_POINT ( 'NONE',  ( -132.7788241241227070, 51.19755864769842901, 88.81639056320175030 ) ) ;
#44868=CARTESIAN_POINT ( 'NONE',  ( -142.3393481102175997, 58.33014244976925511, 62.84203394820867317 ) ) ;
#44869=CARTESIAN_POINT ( 'NONE',  ( 81.76212856587198985, 18.87332718082997474, 31.50068684092350324 ) ) ;
#44873=CARTESIAN_POINT ( 'NONE',  ( 137.4117721579687839, 43.61242559081430414, -10.05773480556120525 ) ) ;
#44875=CARTESIAN_POINT ( 'NONE',  ( -180.6021503146988891, 97.45669259943416307, -14.74712103546458764 ) ) ;
#44877=EDGE_LOOP ( 'NONE', ( #30366, #16041, #19390, #40216 ) ) ;
#44878=EDGE_CURVE ( 'NONE', #30296, #4017, #17888, .T. ) ;
#44881=CARTESIAN_POINT ( 'NONE',  ( 45.90693067088658097, 9.344800815249328707, 41.17893080460214605 ) ) ;
#44885=CARTESIAN_POINT ( 'NONE',  ( -75.00452312211126582, 22.03104735285382176, -76.00973837158169033 ) ) ;
#44886=CARTESIAN_POINT ( 'NONE',  ( -106.6781182590523684, 35.07133425426474815, 70.95721658968783174 ) ) ;
#44887=CARTESIAN_POINT ( 'NONE',  ( -30.47069031368416958, 9.433993659086578276, -50.27049686049341659 ) ) ;
#44888=CARTESIAN_POINT ( 'NONE',  ( -78.66644367742111399, -170.0000000000000000, -35.11545063171788428 ) ) ;
#44891=EDGE_LOOP ( 'NONE', ( #47797, #68870, #24, #13864 ) ) ;
#44893=DIRECTION ( 'NONE',  ( -0.000000000000000000, 1.000000000000000000, -0.000000000000000000 ) ) ;
#44894=CARTESIAN_POINT ( 'NONE',  ( -85.45399718454960691, 25.02415453493130926, 67.96308648905946370 ) ) ;
#44895=CARTESIAN_POINT ( 'NONE',  ( 32.12337157895397866, 7.574134358465434147, -95.00000000000133582 ) ) ;
#44896=CARTESIAN_POINT ( 'NONE',  ( 8.000000000000007105, 249.8719672152120381, -95.00000000000133582 ) ) ;
#44897=AXIS2_PLACEMENT_3D ( 'NONE', #21657, #59284, #43450 ) ;
#44899=CARTESIAN_POINT ( 'NONE',  ( -95.21085197937823352, 30.44372064875429018, -13.11308433111474692 ) ) ;
#44901=CARTESIAN_POINT ( 'NONE',  ( 36.76746179515744473, 8.081433644308901876, 71.28473465010155508 ) ) ;
#44906=DIRECTION ( 'NONE',  ( -0.000000000000000000, 1.000000000000000000, -0.000000000000000000 ) ) ;
#44909=CARTESIAN_POINT ( 'NONE',  ( -109.7793173546317149, 36.75648380851389163, -69.07549051878955026 ) ) ;
#44910=CARTESIAN_POINT ( 'NONE',  ( -97.89650780679127706, 30.60899921334456408, -90.10237382125301053 ) ) ;
#44913=VECTOR ( 'NONE', #67228, 1000.000000000000000 ) ;
#44915=CARTESIAN_POINT ( 'NONE',  ( -33.85171821065139852, 11.02091558840054120, -35.69924149714026385 ) ) ;
#44922=CARTESIAN_POINT ( 'NONE',  ( -142.6736406357357794, 58.59303246027003098, 94.99999999999866418 ) ) ;
#44926=CARTESIAN_POINT ( 'NONE',  ( 158.2042568976887082, 59.50370424804803093, -89.84040114574384006 ) ) ;
#44928=CARTESIAN_POINT ( 'NONE',  ( -95.52093927227217307, 30.58993121475388222, 41.27929887050821378 ) ) ;
#44930=CARTESIAN_POINT ( 'NONE',  ( 17.48889770758268014, 6.561062909825355227, -50.32774512300183289 ) ) ;
#44931=CARTESIAN_POINT ( 'NONE',  ( 117.4806398654733357, 33.50379325299402922, 8.232446593192225492 ) ) ;
#44932=ORIENTED_EDGE ( 'NONE', *, *, #48319, .F. ) ;
#44933=CARTESIAN_POINT ( 'NONE',  ( 59.29615173875419742, 11.84060224810188267, 30.79565124887290395 ) ) ;
#44937=CARTESIAN_POINT ( 'NONE',  ( 181.0840389613909736, 80.03940679743415387, 44.30859410551141764 ) ) ;
#44943=ADVANCED_FACE ( 'NONE', ( #6460 ), #47965, .F. ) ;
#44944=CARTESIAN_POINT ( 'NONE',  ( -31.43908319763709969, 10.61114334766716105, 45.21645440618919309 ) ) ;
#44946=CARTESIAN_POINT ( 'NONE',  ( -71.97171223898807568, 20.94894057408426136, -39.19762039591116576 ) ) ;
#44948=CARTESIAN_POINT ( 'NONE',  ( 180.7426746203128687, 79.69150696735539441, -89.91415884680699833 ) ) ;
#44949=CARTESIAN_POINT ( 'NONE',  ( 140.8855094313933307, 47.03549517811090652, 39.63981015661840956 ) ) ;
#44950=CARTESIAN_POINT ( 'NONE',  ( -177.1514380519393512, 93.28180884530864603, 44.66195762070336173 ) ) ;
#44951=CARTESIAN_POINT ( 'NONE',  ( 128.3889472838589541, 39.37765603157611594, 69.01175771905448642 ) ) ;
#44954=VERTEX_POINT ( 'NONE', #69430 ) ;
#44958=CARTESIAN_POINT ( 'NONE',  ( 211.7634543339367781, 116.5654349622355141, -95.00000000000133582 ) ) ;
#44961=CARTESIAN_POINT ( 'NONE',  ( -99.97240228788317040, 31.62311673723580085, 84.54697963296760577 ) ) ;
#44962=CARTESIAN_POINT ( 'NONE',  ( -144.3945994505580472, 59.96115386701889349, 32.72843562861698530 ) ) ;
#44964=CARTESIAN_POINT ( 'NONE',  ( -78.66644367742109978, 23.39876645725288640, -23.27090004125422595 ) ) ;
#44966=CARTESIAN_POINT ( 'NONE',  ( 84.27368848767932263, 18.63026910897604793, 56.91985697824755874 ) ) ;
#44968=CARTESIAN_POINT ( 'NONE',  ( -95.58372570396208801, 30.61946167424475362, -92.79505394063129131 ) ) ;
#44972=DIRECTION ( 'NONE',  ( 0.000000000000000000, 0.000000000000000000, 1.000000000000000000 ) ) ;
#44974=CARTESIAN_POINT ( 'NONE',  ( -119.2804658695888236, 43.47213805166352785, 61.41757901617579307 ) ) ;
#44975=CARTESIAN_POINT ( 'NONE',  ( -9.765753193741732119, 8.033970690975921869, -50.16687931305852288 ) ) ;
#44979=ORIENTED_EDGE ( 'NONE', *, *, #32153, .F. ) ;
#44981=CARTESIAN_POINT ( 'NONE',  ( -156.0171627975467459, 69.90368824761763733, -11.73444720282849474 ) ) ;
#44983=DIRECTION ( 'NONE',  ( -0.000000000000000000, 1.000000000000000000, -0.000000000000000000 ) ) ;
#44986=VERTEX_POINT ( 'NONE', #31803 ) ;
#44988=CARTESIAN_POINT ( 'NONE',  ( 151.7783534118501905, 54.60545177578659093, -65.57863077677340868 ) ) ;
#44990=CARTESIAN_POINT ( 'NONE',  ( 139.7928618793172859, 45.12615179300589574, -38.93259025567166276 ) ) ;
#44993=VERTEX_POINT ( 'NONE', #22284 ) ;
#44997=CARTESIAN_POINT ( 'NONE',  ( 141.3587662457627232, 47.34635740004710414, 90.65385063068173110 ) ) ;
#45001=ORIENTED_EDGE ( 'NONE', *, *, #54068, .T. ) ;
#45005=CARTESIAN_POINT ( 'NONE',  ( 141.3445468829085314, 46.13338528906589886, -69.86407327641063603 ) ) ;
#45011=CARTESIAN_POINT ( 'NONE',  ( 160.2883311361769927, 61.16711613734478448, -9.825516263918585125 ) ) ;
#45014=CARTESIAN_POINT ( 'NONE',  ( 14.80582440982707837, 6.470883766728821485, 44.96611724300024804 ) ) ;
#45016=CARTESIAN_POINT ( 'NONE',  ( -57.65733424639443427, 15.39521790791523159, -62.52345615960770431 ) ) ;
#45017=CARTESIAN_POINT ( 'NONE',  ( 128.3516609434389011, 38.19824209820340144, -92.10286917565350961 ) ) ;
#45019=CARTESIAN_POINT ( 'NONE',  ( -142.0081215801269536, 58.07066293384865219, -69.45719805043682982 ) ) ;
#45021=VECTOR ( 'NONE', #14617, 1000.000000000000000 ) ;
#45023=CARTESIAN_POINT ( 'NONE',  ( 157.9160637431159557, 57.99786926216935257, -36.12418429913763873 ) ) ;
#45025=CARTESIAN_POINT ( 'NONE',  ( -95.86163447241557378, 30.75089131639700213, 7.262573566396630653 ) ) ;
#45026=CARTESIAN_POINT ( 'NONE',  ( 70.37411710121934050, 15.54173091717098210, 89.51384947277743720 ) ) ;
#45028=CARTESIAN_POINT ( 'NONE',  ( 66.07923263163412742, 14.44036440558002177, 30.46288473904308702 ) ) ;
#45029=CARTESIAN_POINT ( 'NONE',  ( -132.4951995226844872, 50.99687809989499243, -19.13814356169182318 ) ) ;
#45030=CARTESIAN_POINT ( 'NONE',  ( -147.5180482799911488, 62.50984070207314858, -88.75905994936287868 ) ) ;
#45031=CARTESIAN_POINT ( 'NONE',  ( 128.9253503890652723, 38.52561778336672660, -76.02404744399288461 ) ) ;
#45034=CARTESIAN_POINT ( 'NONE',  ( 139.1306635769909974, 45.89653412152171086, -75.70587900743647936 ) ) ;
#45036=ORIENTED_EDGE ( 'NONE', *, *, #63990, .T. ) ;
#45039=CARTESIAN_POINT ( 'NONE',  ( -156.8773151811562911, 72.06122063279302381, -40.89328888528041972 ) ) ;
#45040=CARTESIAN_POINT ( 'NONE',  ( 206.3053863259449656, 110.3084416756849180, -9.610806492142495827 ) ) ;
#45041=CARTESIAN_POINT ( 'NONE',  ( -38.88884187334145537, 11.95889603743730234, 36.71961320002495199 ) ) ;
#45043=CARTESIAN_POINT ( 'NONE',  ( -1.327237339234996982, 7.561837009978233048, 41.36847194710579600 ) ) ;
#45045=CARTESIAN_POINT ( 'NONE',  ( -47.95468448182521115, 12.89252559348045857, -67.12589513619153081 ) ) ;
#45050=CARTESIAN_POINT ( 'NONE',  ( -95.52093927227218728, 30.58993121475389287, -39.25435290088285001 ) ) ;
#45052=CARTESIAN_POINT ( 'NONE',  ( 103.8317086684999850, 26.02720265156213486, -66.36710428647430149 ) ) ;
#45054=CARTESIAN_POINT ( 'NONE',  ( 46.90222083990963853, 9.503928413859233260, 64.49857371303593823 ) ) ;
#45055=CYLINDRICAL_SURFACE ( 'NONE', #2044, 7.500000000000013323 ) ;
#45058=CARTESIAN_POINT ( 'NONE',  ( 110.2429982417149432, 28.88204397445228722, 44.61121420573733332 ) ) ;
#45060=CARTESIAN_POINT ( 'NONE',  ( -77.72491324796695267, 21.96482567905605521, 57.30687935295142665 ) ) ;
#45061=CARTESIAN_POINT ( 'NONE',  ( -167.9889421625798889, 81.59140042431232587, 59.67682617645385790 ) ) ;
#45062=ORIENTED_EDGE ( 'NONE', *, *, #67449, .F. ) ;
#45065=CARTESIAN_POINT ( 'NONE',  ( 173.9413349464226997, 71.67637800842359752, 61.34821181573801141 ) ) ;
#45066=CIRCLE ( 'NONE', #25947, 242.4895526022646379 ) ;
#45069=CARTESIAN_POINT ( 'NONE',  ( 103.1534365798308528, 26.83148826706847956, 66.45580475007047028 ) ) ;
#45070=CARTESIAN_POINT ( 'NONE',  ( -166.0012244511291613, 80.97916541034756222, -17.74230296181466926 ) ) ;
#45071=VECTOR ( 'NONE', #13910, 1000.000000000000000 ) ;
#45074=CARTESIAN_POINT ( 'NONE',  ( 103.8055367708241477, 27.11070767929350822, -39.54200133079056911 ) ) ;
#45075=CARTESIAN_POINT ( 'NONE',  ( 19.11382977197791533, 7.636807742668411336, -36.27859613552720930 ) ) ;
#45080=FACE_BOUND ( 'NONE', #54381, .T. ) ;
#45086=CARTESIAN_POINT ( 'NONE',  ( -180.3114074031036296, 97.09758726817787533, 9.322656802965427758 ) ) ;
#45087=CARTESIAN_POINT ( 'NONE',  ( 211.4997502125519304, 118.0043045815490359, 60.37852553085293295 ) ) ;
#45088=CARTESIAN_POINT ( 'NONE',  ( 86.14852828165525978, 19.25704475759650691, -62.66611478937537782 ) ) ;
#45091=ADVANCED_FACE ( 'NONE', ( #53585 ), #37078, .T. ) ;
#45093=EDGE_LOOP ( 'NONE', ( #63494, #46933, #32678, #45492, #58218, #40201, #55508, #56526, #32545, #16483, #2818, #28681, #61178, #16009, #50400, #56626, #31390, #1210, #40803, #32029, #7210, #191, #24779, #50763, #58608, #47470, #50239, #21439, #12236, #66635, #44545, #15621, #18510, #49211, #8607, #14658, #18237, #60244, #40492, #12806, #62912, #45786, #49716, #56602, #24780, #48660, #66180, #43089, #27214, #46684, #56921, #15352, #69228, #64823, #51930, #33406, #4585, #66762, #24492, #42263, #44066, #65061, #52769, #37777, #54710, #8442, #39386, #61206, #62655, #43507, #48222, #32732, #49046, #10323, #68634, #41900, #43962, #50847, #25207, #30829, #23486, #57052, #45062, #25565, #68931, #54639, #29815, #10764, #68517 ) ) ;
#45094=EDGE_CURVE ( 'NONE', #37531, #18323, #43774, .T. ) ;
#45095=FACE_OUTER_BOUND ( 'NONE', #49006, .T. ) ;
#45097=CARTESIAN_POINT ( 'NONE',  ( -84.97622048504841530, 24.82614411847756841, -73.52177815261417493 ) ) ;
#45098=CARTESIAN_POINT ( 'NONE',  ( -60.47589866267035319, 17.25153113855766662, -21.05818846266538458 ) ) ;
#45099=CARTESIAN_POINT ( 'NONE',  ( 91.50468583833759340, 22.21368636549397380, -75.88665251703855574 ) ) ;
#45106=CARTESIAN_POINT ( 'NONE',  ( 102.7414208686707724, 26.65627265923297173, 10.75606379640384525 ) ) ;
#45108=ORIENTED_EDGE ( 'NONE', *, *, #68677, .T. ) ;
#45112=CARTESIAN_POINT ( 'NONE',  ( -47.55256438668344288, 13.83151366677316219, 10.73057395638927325 ) ) ;
#45113=CARTESIAN_POINT ( 'NONE',  ( -129.6079169496901216, 50.20899308323959787, -9.049169391184644695 ) ) ;
#45114=CARTESIAN_POINT ( 'NONE',  ( -152.6692566860463955, 68.24922339534836624, -89.18787451257621512 ) ) ;
#45115=CARTESIAN_POINT ( 'NONE',  ( 112.5554747942046134, 29.96654954475020105, -23.71639831171845003 ) ) ;
#45116=CARTESIAN_POINT ( 'NONE',  ( 93.47084677873587566, 21.86992891175610865, 87.80919612172070288 ) ) ;
#45117=CARTESIAN_POINT ( 'NONE',  ( -149.5074843970971301, -170.0000000000000000, -7.968279941028271196 ) ) ;
#45124=CARTESIAN_POINT ( 'NONE',  ( 174.9161599490640526, 73.97365196673301568, 5.688883349119021382 ) ) ;
#45126=CARTESIAN_POINT ( 'NONE',  ( 105.4193882736795871, 26.71329717705293660, -22.34225740095065404 ) ) ;
#45128=CARTESIAN_POINT ( 'NONE',  ( -55.05276343752910151, 14.68156374112636797, 72.16187836339486239 ) ) ;
#45129=CARTESIAN_POINT ( 'NONE',  ( 210.6189312023034574, 116.6550319566545539, 94.99999999999866418 ) ) ;
#45130=FACE_OUTER_BOUND ( 'NONE', #15830, .T. ) ;
#45134=CARTESIAN_POINT ( 'NONE',  ( 8.287863202055540057, 7.382585476140731906, -15.68614915429326473 ) ) ;
#45139=CARTESIAN_POINT ( 'NONE',  ( -170.2951623264597174, 85.51757001115473145, 45.28173547561066670 ) ) ;
#45140=CARTESIAN_POINT ( 'NONE',  ( -100.4466073551323007, 31.85873123265079698, -49.80183754970560273 ) ) ;
#45142=CARTESIAN_POINT ( 'NONE',  ( -109.5142642360664240, 36.61018064014775319, 9.126798092972807197 ) ) ;
#45143=DIRECTION ( 'NONE',  ( -0.000000000000000000, 1.000000000000000000, -0.000000000000000000 ) ) ;
#45144=CARTESIAN_POINT ( 'NONE',  ( 135.6647932137618113, 43.70902528961477174, -9.385834288385190405 ) ) ;
#45147=CYLINDRICAL_SURFACE ( 'NONE', #39499, 7.500000000000020428 ) ;
#45150=CARTESIAN_POINT ( 'NONE',  ( 56.30171512200998052, 11.21502580416398587, -13.02431553323698132 ) ) ;
#45152=VECTOR ( 'NONE', #61542, 1000.000000000000000 ) ;
#45155=VERTEX_POINT ( 'NONE', #12434 ) ;
#45156=CARTESIAN_POINT ( 'NONE',  ( 157.4703587214989398, -170.0000000000000000, -24.27963370867398396 ) ) ;
#45157=CARTESIAN_POINT ( 'NONE',  ( -56.96436614829622158, 16.24647150911285109, -76.81720701772762538 ) ) ;
#45158=CARTESIAN_POINT ( 'NONE',  ( 199.7286177451875062, 101.4075663537891643, -76.30715059617197937 ) ) ;
#45163=CARTESIAN_POINT ( 'NONE',  ( -167.6413528428655582, 81.22881971256911982, 6.330796842060393281 ) ) ;
#45164=DIRECTION ( 'NONE',  ( 0.000000000000000000, -1.000000000000000000, 0.000000000000000000 ) ) ;
#45165=FACE_BOUND ( 'NONE', #49543, .T. ) ;
#45168=COLOUR_RGB ( '',0.7921568627450980005, 0.8196078431372548767, 0.9333333333333333481 ) ;
#45175=CARTESIAN_POINT ( 'NONE',  ( 150.2805372522807374, 53.51147386362154634, 65.90567756530964516 ) ) ;
#45184=EDGE_LOOP ( 'NONE', ( #38352, #31228, #68303, #12792 ) ) ;
#45186=DIRECTION ( 'NONE',  ( 0.000000000000000000, 0.000000000000000000, 1.000000000000000000 ) ) ;
#45187=CARTESIAN_POINT ( 'NONE',  ( 150.9128604434957879, 53.97103482421773890, 33.23130411755268909 ) ) ;
#45191=LINE ( 'NONE', #8612, #31242 ) ;
#45192=ADVANCED_FACE ( 'NONE', ( #9579 ), #19430, .F. ) ;
#45193=CARTESIAN_POINT ( 'NONE',  ( -178.0633751203918678, 92.80295726428050784, 17.12321454651181796 ) ) ;
#45194=CARTESIAN_POINT ( 'NONE',  ( -0.5183605925912000423, 6.525266619725953454, 9.063124254828315074 ) ) ;
#45196=CARTESIAN_POINT ( 'NONE',  ( -25.49247221749737946, 9.706368398275717624, -11.37573925065449743 ) ) ;
#45199=SHAPE_REPRESENTATION ( 'SIEVE', ( #66832 ), #5131 ) ;
#45200=CARTESIAN_POINT ( 'NONE',  ( 113.4493678088378203, 30.39339414805072792, -36.62597440105078306 ) ) ;
#45201=CARTESIAN_POINT ( 'NONE',  ( -76.33235143960695268, 22.51916353135075255, 18.20519721888241449 ) ) ;
#45202=CARTESIAN_POINT ( 'NONE',  ( 44.35071890818840501, 9.104600422692270101, -37.46304456836167418 ) ) ;
#45203=CARTESIAN_POINT ( 'NONE',  ( -172.7173255566597732, 88.18461381371098184, -76.55650775521371543 ) ) ;
#45204=CARTESIAN_POINT ( 'NONE',  ( -131.5964873355040368, 50.36491837697927565, 86.92810408690877466 ) ) ;
#45206=CARTESIAN_POINT ( 'NONE',  ( 84.74140601443113496, 18.78541996275573212, -36.05909698884106263 ) ) ;
#45208=EDGE_LOOP ( 'NONE', ( #69524, #36600 ) ) ;
#45209=CIRCLE ( 'NONE', #40741, 242.4895526022646379 ) ;
#45214=CARTESIAN_POINT ( 'NONE',  ( 181.5127080940606277, 79.03904173130082711, -9.380507075415927432 ) ) ;
#45216=CARTESIAN_POINT ( 'NONE',  ( -123.6699087229882110, 45.04696784753416239, 57.79816663664966825 ) ) ;
#45217=CARTESIAN_POINT ( 'NONE',  ( 44.34362023773822870, 10.12115849931653422, 4.905806151721804120 ) ) ;
#45218=CARTESIAN_POINT ( 'NONE',  ( -178.2328124332057087, 94.56955476227571467, -20.87550340617716671 ) ) ;
#45222=CARTESIAN_POINT ( 'NONE',  ( 103.8093541423579325, 26.01745837747062851, 60.06901032783780892 ) ) ;
#45224=CARTESIAN_POINT ( 'NONE',  ( 164.9534461562627712, 63.71129898458566032, 63.17659111825835083 ) ) ;
#45226=CARTESIAN_POINT ( 'NONE',  ( 66.29961816943398389, 13.45804302849873579, -23.13624938398751141 ) ) ;
#45227=CARTESIAN_POINT ( 'NONE',  ( 183.9986899696431522, 81.60141257362813860, -50.64888762674885925 ) ) ;
#45228=CARTESIAN_POINT ( 'NONE',  ( -105.8768181937898589, 34.64545164169047808, 71.46195835557104203 ) ) ;
#45230=DIRECTION ( 'NONE',  ( 0.000000000000000000, 0.000000000000000000, 1.000000000000000000 ) ) ;
#45231=VERTEX_POINT ( 'NONE', #35963 ) ;
#45233=ORIENTED_EDGE ( 'NONE', *, *, #22710, .T. ) ;
#45234=FACE_OUTER_BOUND ( 'NONE', #52768, .T. ) ;
#45235=CARTESIAN_POINT ( 'NONE',  ( -78.08539259565777968, 22.10035297730220805, 84.10499846222364795 ) ) ;
#45242=CARTESIAN_POINT ( 'NONE',  ( 56.94505604581134151, 12.37336791557969917, 32.90170006804437008 ) ) ;
#45245=CARTESIAN_POINT ( 'NONE',  ( -0.3734056954813056994, 6.520221844775928588, -41.93998480159426379 ) ) ;
#45247=CARTESIAN_POINT ( 'NONE',  ( -189.4223925288096382, 107.3427006758676328, -40.39023558151960458 ) ) ;
#45249=DIRECTION ( 'NONE',  ( -0.000000000000000000, 1.000000000000000000, -0.000000000000000000 ) ) ;
#45251=CARTESIAN_POINT ( 'NONE',  ( 197.2197025888162045, 96.62026035493818199, 62.89200297478758728 ) ) ;
#45252=CARTESIAN_POINT ( 'NONE',  ( 128.3889472838589256, 39.37765603157609462, -11.52189405233656139 ) ) ;
#45257=CARTESIAN_POINT ( 'NONE',  ( -37.52119286077851967, 11.69341290629620467, -47.21248048768034522 ) ) ;
#45258=DIRECTION ( 'NONE',  ( 0.000000000000000000, 0.000000000000000000, 1.000000000000000000 ) ) ;
#45262=CARTESIAN_POINT ( 'NONE',  ( -125.4481990864045287, 46.20056605584954923, -49.91370389823396891 ) ) ;
#45263=AXIS2_PLACEMENT_3D ( 'NONE', #20643, #53683, #36836 ) ;
#45264=LINE ( 'NONE', #60750, #30245 ) ;
#45271=CARTESIAN_POINT ( 'NONE',  ( -57.42826130032241849, 16.37596353166460617, 3.854800282744499818 ) ) ;
#45274=CARTESIAN_POINT ( 'NONE',  ( -155.5977325361978387, 70.88311713755702215, 42.60514736212469700 ) ) ;
#45277=CARTESIAN_POINT ( 'NONE',  ( 22.89234820949994642, 6.832052815347871011, -45.43617115817555430 ) ) ;
#45278=CARTESIAN_POINT ( 'NONE',  ( 115.7731501832036685, 32.64791439093737324, 5.176517809787929636 ) ) ;
#45279=ORIENTED_EDGE ( 'NONE', *, *, #16382, .F. ) ;
#45280=CARTESIAN_POINT ( 'NONE',  ( 58.47673920847984874, 11.66523265296355305, 31.32250200715353827 ) ) ;
#45282=VERTEX_POINT ( 'NONE', #56730 ) ;
#45283=CARTESIAN_POINT ( 'NONE',  ( 174.9161599490640526, 73.97365196673298726, 32.53343393958267882 ) ) ;
#45284=B_SPLINE_CURVE_WITH_KNOTS ( 'NONE', 3,
 ( #24871, #46308, #19582, #9730, #67786, #52621, #41041, #41733, #14316, #35775, #57226, #9040, #63192, #47336, #14652, #30486, #36114, #57570, #9381, #30841, #52284, #25569, #47008, #20274, #36456, #49062, #63533, #58581, #31869, #5475, #22000, #546, #42419, #48026, #59275, #188, #36805, #4781, #26250, #63878, #6156, #53986, #27618, #26930 ),
 .UNSPECIFIED., .F., .F.,
 ( 4, 2, 2, 2, 2, 2, 2, 2, 2, 2, 2, 2, 2, 2, 2, 2, 2, 2, 2, 2, 2, 4 ),
 ( 0.02495775893651561508, 0.02650251144344300744, 0.02804726395037039979, 0.02959201645729779215, 0.03113676896422518450, 0.03268152147115257339, 0.03345389772461627304, 0.03422627397807997268, 0.03577102648500738585, 0.03654340273847110632, 0.03731577899193481984, 0.03808815524539853337, 0.03886053149886224689, 0.04040528400578969476, 0.04117766025925341522, 0.04195003651271712874, 0.04349478901964452804, 0.04503954152657194121, 0.04581191778003564780, 0.04658429403349935438, 0.04812904654042681613, 0.04967379904735427787 ),
 .UNSPECIFIED. ) ;
#45285=CARTESIAN_POINT ( 'NONE',  ( 22.30016284075437483, 6.796348835713779124, -66.11047376476241766 ) ) ;
#45286=CARTESIAN_POINT ( 'NONE',  ( -10.92576759990585877, 8.121994053275065184, -62.92908167533382624 ) ) ;
#45287=VERTEX_POINT ( 'NONE', #67636 ) ;
#45288=CARTESIAN_POINT ( 'NONE',  ( 39.40195752203892710, -170.0000000000000000, -69.96436805589145536 ) ) ;
#45290=CARTESIAN_POINT ( 'NONE',  ( -73.81801970646053235, 21.60231032711190480, -36.88809761374765372 ) ) ;
#45291=EDGE_LOOP ( 'NONE', ( #46184, #18293, #68890, #19219 ) ) ;
#45292=CARTESIAN_POINT ( 'NONE',  ( 212.1488570093001726, 119.0116247937291121, -71.54201036058580598 ) ) ;
#45295=CARTESIAN_POINT ( 'NONE',  ( 116.5100763992442836, 33.01539745157280947, 41.23853340567732317 ) ) ;
#45296=CARTESIAN_POINT ( 'NONE',  ( -130.5811943660944223, 50.88295841537571818, 5.400760641591992872 ) ) ;
#45297=CARTESIAN_POINT ( 'NONE',  ( 16.28382582968306735, 7.523443033994205997, 71.85925826316895382 ) ) ;
#45299=VERTEX_POINT ( 'NONE', #68328 ) ;
#45302=B_SPLINE_CURVE_WITH_KNOTS ( 'NONE', 3,
 ( #981, #61111, #54776, #17495, #28398, #6602, #49139, #50208, #17854, #28048, #50555, #38608, #23134, #22429, #18547, #34396, #49844, #60756, #60050, #7300, #2034, #12231, #44219, #33346, #49489, #39312, #23488, #44583, #33695, #43867, #1321, #38968, #22776, #60414, #12577, #56174, #65703, #66062 ),
 .UNSPECIFIED., .F., .F.,
 ( 4, 2, 2, 2, 2, 2, 2, 2, 2, 2, 2, 2, 2, 2, 2, 2, 2, 2, 4 ),
 ( 1.387778780781445676E-17, 0.003908178031105357005, 0.005862267046658047216, 0.007816356062210738295, 0.009770445077763428507, 0.01172453409331611872, 0.01270157860109245862, 0.01367862310886879679, 0.01465566761664513669, 0.01563271212442147659, 0.01660975663219781476, 0.01758680113997415639, 0.01954089015552684314, 0.02051793466330320212, 0.02149497917107956457, 0.02344906818663228601, 0.02540315720218501092, 0.02735724621773773235, 0.03126542424884321686 ),
 .UNSPECIFIED. ) ;
#45304=AXIS2_PLACEMENT_3D ( 'NONE', #46179, #62366, #67652 ) ;
#45305=CARTESIAN_POINT ( 'NONE',  ( -31.43908319763709969, 9.591432048623767415, -50.31719736520186359 ) ) ;
#45306=CARTESIAN_POINT ( 'NONE',  ( -98.33320668777302842, 30.82058677165679939, 85.32320660558336556 ) ) ;
#45307=CARTESIAN_POINT ( 'NONE',  ( -147.3641864666714412, 62.38213854487951693, 31.02004508490727375 ) ) ;
#45308=VECTOR ( 'NONE', #9505, 1000.000000000000000 ) ;
#45313=CARTESIAN_POINT ( 'NONE',  ( -104.1225399044495958, 34.86084180570100699, 30.74510362357437288 ) ) ;
#45314=VERTEX_POINT ( 'NONE', #20128 ) ;
#45315=CARTESIAN_POINT ( 'NONE',  ( 36.08729376665095145, 8.001156100723207487, 44.15947279111765056 ) ) ;
#45316=VECTOR ( 'NONE', #38074, 1000.000000000000000 ) ;
#45319=B_SPLINE_CURVE_WITH_KNOTS ( 'NONE', 3,
 ( #43494, #6213, #27667, #26643, #59328, #48076, #32949, #11479, #16076, #5860, #49461, #49107, #48406, #54390, #22048, #16763, #22748, #65672 ),
 .UNSPECIFIED., .F., .F.,
 ( 4, 2, 2, 2, 2, 2, 2, 2, 4 ),
 ( 0.01015325708522461443, 0.01143429661445663145, 0.01271533614368864848, 0.01399637567292066377, 0.01527741520215268080, 0.01655845473138469609, 0.01783949426061671312, 0.01912053378984873014, 0.02040157331908074717 ),
 .UNSPECIFIED. ) ;
#45323=CARTESIAN_POINT ( 'NONE',  ( -50.51700111023804851, 13.51182830536852997, 16.96585246969117122 ) ) ;
#45324=VECTOR ( 'NONE', #34619, 1000.000000000000000 ) ;
#45331=DIRECTION ( 'NONE',  ( -0.000000000000000000, 1.000000000000000000, -0.000000000000000000 ) ) ;
#45332=CARTESIAN_POINT ( 'NONE',  ( -62.55320287144887459, 17.87319849854532450, 64.89944872409208187 ) ) ;
#45333=CARTESIAN_POINT ( 'NONE',  ( 204.6977192012829789, -170.0000000000000000, 63.55227132923313604 ) ) ;
#45336=CARTESIAN_POINT ( 'NONE',  ( 152.2924710224604610, 54.98503313872888043, -65.03745591564339179 ) ) ;
#45337=EDGE_CURVE ( 'NONE', #51958, #1836, #50969, .T. ) ;
#45338=CARTESIAN_POINT ( 'NONE',  ( -34.74740905761647269, 10.15745573515589406, 44.46511832658496388 ) ) ;
#45339=CARTESIAN_POINT ( 'NONE',  ( -29.02794087136069834, 9.207646203414356023, 71.67951027246965623 ) ) ;
#45344=CARTESIAN_POINT ( 'NONE',  ( -120.1497954511983437, 42.82624472369556656, 33.27088217181543683 ) ) ;
#45346=CARTESIAN_POINT ( 'NONE',  ( 39.40195752203891999, 9.424259417798147354, -8.775266874964067654 ) ) ;
#45349=CARTESIAN_POINT ( 'NONE',  ( 130.8606599820531926, 40.81082399113100934, 83.81639294592298484 ) ) ;
#45350=B_SPLINE_CURVE_WITH_KNOTS ( 'NONE', 3,
 ( #24828, #68429, #63153, #61755, #52917, #4742, #16338, #5088, #37792, #15988, #20926, #64879, #32178, #27580, #37437, #10030, #21609, #53259, #21958, #27229, #26553, #6119, #49019, #48318, #59235, #58212, #54296, #47986, #31827, #63496, #58890, #38133, #69452, #21269, #42717, #31484, #858, #10360, #10706, #36768, #506, #64174, #53611, #26206, #59575 ),
 .UNSPECIFIED., .F., .F.,
 ( 4, 2, 2, 2, 2, 2, 2, 2, 2, 2, 2, 2, 2, 1, 2, 2, 2, 2, 2, 2, 2, 2, 4 ),
 ( 0.02356759485890609976, 0.02503765354686412689, 0.02577268289084315434, 0.02650771223482217831, 0.02797777092278022279, 0.02944782961073826727, 0.03018285895471728084, 0.03091788829869629440, 0.03238794698665432847, 0.03312297633063336633, 0.03385800567461239030, 0.03532806436257047988, 0.03606309370654951774, 0.03679812305052856253, 0.03753315239450760732, 0.03826818173848664517, 0.03973824042644472782, 0.04120829911440281046, 0.04267835780236089310, 0.04341338714633992402, 0.04414841649031895493, 0.04561847517827700982, 0.04708853386623507165 ),
 .UNSPECIFIED. ) ;
#45351=CARTESIAN_POINT ( 'NONE',  ( -24.57945280941397215, 9.580546049925253271, -93.35324784431733747 ) ) ;
#45355=CARTESIAN_POINT ( 'NONE',  ( -125.4433371161043311, 46.19736518073186460, -61.75825448869758105 ) ) ;
#45360=CARTESIAN_POINT ( 'NONE',  ( -133.1180864139201390, 52.67432865667906583, -94.03100957856869968 ) ) ;
#45373=ORIENTED_EDGE ( 'NONE', *, *, #14159, .T. ) ;
#45374=CARTESIAN_POINT ( 'NONE',  ( 164.8914542114683002, 64.97670918603526502, -44.74542541857194067 ) ) ;
#45380=CARTESIAN_POINT ( 'NONE',  ( 64.34362785825726405, 14.01885293761273665, 83.61320876023768278 ) ) ;
#45382=CARTESIAN_POINT ( 'NONE',  ( 83.59652366361572717, 19.46709838196855102, -9.613360744613480335 ) ) ;
#45383=CARTESIAN_POINT ( 'NONE',  ( -133.0808647576834005, 51.41195281028756625, -13.40905688364864190 ) ) ;
#45385=CARTESIAN_POINT ( 'NONE',  ( 126.9201538765324386, 37.39093565120715112, -67.50410470727368306 ) ) ;
#45387=CARTESIAN_POINT ( 'NONE',  ( -101.8140949286062096, 33.67224128592400945, 72.36362509687882039 ) ) ;
#45388=CARTESIAN_POINT ( 'NONE',  ( -15.27594996066617483, 8.502079791899653571, 63.47073034068081654 ) ) ;
#45394=CARTESIAN_POINT ( 'NONE',  ( -0.5783162822156596716, 7.534184941292927817, 39.56237465081175486 ) ) ;
#45397=CARTESIAN_POINT ( 'NONE',  ( -4.731197926646204088, 7.716745361328043451, -22.90991753403145736 ) ) ;
#45399=CARTESIAN_POINT ( 'NONE',  ( -62.15799747763098537, 16.70234469631017404, 8.520624946596262461 ) ) ;
#45403=ORIENTED_EDGE ( 'NONE', *, *, #62259, .T. ) ;
#45404=CARTESIAN_POINT ( 'NONE',  ( 104.7034219878852355, 26.40210929103713511, -75.34717264657832914 ) ) ;
#45405=CARTESIAN_POINT ( 'NONE',  ( 43.96421756700841144, 10.06386361114659955, -22.24800231128863004 ) ) ;
#45407=CARTESIAN_POINT ( 'NONE',  ( 43.35980717318837918, 8.957244490220908517, 70.63379478250071486 ) ) ;
#45413=CARTESIAN_POINT ( 'NONE',  ( -169.8842709557924309, 83.59602878049473418, 58.38604360640643876 ) ) ;
#45415=ORIENTED_EDGE ( 'NONE', *, *, #53684, .F. ) ;
#45417=DIRECTION ( 'NONE',  ( -0.000000000000000000, 1.000000000000000000, -0.000000000000000000 ) ) ;
#45418=EDGE_CURVE ( 'NONE', #48695, #22683, #11013, .T. ) ;
#45421=CARTESIAN_POINT ( 'NONE',  ( 103.9685899589048148, 27.18106603025991319, 59.83941942854519169 ) ) ;
#45424=EDGE_CURVE ( 'NONE', #18637, #53396, #31047, .T. ) ;
#45425=CARTESIAN_POINT ( 'NONE',  ( 55.91133443650747381, 12.16263767238153193, -18.83026767310629879 ) ) ;
#45429=CARTESIAN_POINT ( 'NONE',  ( -84.97622048504842951, 24.82614411847756486, -19.83267697168680499 ) ) ;
#45431=CARTESIAN_POINT ( 'NONE',  ( 175.5429257635130682, 74.57009623370763052, -11.80030295197366996 ) ) ;
#45432=CARTESIAN_POINT ( 'NONE',  ( 9.034661095809960685, 6.378368787883688107, -93.41972067307213479 ) ) ;
#45438=CARTESIAN_POINT ( 'NONE',  ( -180.2188652555596775, 96.98354576637426305, 9.036536700887030094 ) ) ;
#45439=CARTESIAN_POINT ( 'NONE',  ( 152.6560521232695464, 54.00248515670892147, 4.308935166207688461 ) ) ;
#45442=ORIENTED_EDGE ( 'NONE', *, *, #41864, .T. ) ;
#45444=CARTESIAN_POINT ( 'NONE',  ( 200.4574930424075205, 102.3536505870638251, -37.62237834330278474 ) ) ;
#45449=CARTESIAN_POINT ( 'NONE',  ( -85.35127931077728647, 24.98147633332999717, -72.86973326730625899 ) ) ;
#45451=CARTESIAN_POINT ( 'NONE',  ( 94.02499804464936517, 23.15433260743126098, -68.89411343564552226 ) ) ;
#45454=CARTESIAN_POINT ( 'NONE',  ( 41.80869235728137312, 9.750404582811606602, 57.13814906687242257 ) ) ;
#45456=CARTESIAN_POINT ( 'NONE',  ( 23.23895241123075195, 6.853530908437178049, 9.681958699395883272 ) ) ;
#45459=AXIS2_PLACEMENT_3D ( 'NONE', #1735, #6304, #55533 ) ;
#45460=CARTESIAN_POINT ( 'NONE',  ( -52.67596829228262578, 15.09584868440939331, -49.84632435105815063 ) ) ;
#45461=CARTESIAN_POINT ( 'NONE',  ( 59.08202327466404569, 12.82375733818951247, -36.83031859667770647 ) ) ;
#45463=CARTESIAN_POINT ( 'NONE',  ( -9.510892918907986271, 8.014150818648904107, -89.24936681866903143 ) ) ;
#45471=FACE_OUTER_BOUND ( 'NONE', #59038, .T. ) ;
#45474=CARTESIAN_POINT ( 'NONE',  ( 102.8458551240039611, 25.60773946375957166, -17.84239502940274846 ) ) ;
#45475=CARTESIAN_POINT ( 'NONE',  ( 197.3707490726349931, 96.80690576410101755, 11.49558936419983546 ) ) ;
#45478=DIRECTION ( 'NONE',  ( 0.000000000000000000, 0.000000000000000000, 1.000000000000000000 ) ) ;
#45479=CARTESIAN_POINT ( 'NONE',  ( -15.32520546926283522, 7.495995523981878073, 38.10845715258894728 ) ) ;
#45482=CARTESIAN_POINT ( 'NONE',  ( 86.62931800182293784, -170.0000000000000000, 56.55663816294300261 ) ) ;
#45484=ORIENTED_EDGE ( 'NONE', *, *, #24502, .T. ) ;
#45486=CARTESIAN_POINT ( 'NONE',  ( 188.4920037102893957, 87.93425473911915446, -69.36007641940153690 ) ) ;
#45487=CARTESIAN_POINT ( 'NONE',  ( -34.85264071515286588, 11.19872911336657850, 84.71973201243903873 ) ) ;
#45488=CARTESIAN_POINT ( 'NONE',  ( -97.47339919287391297, 30.40512551257287299, -36.73650405462576884 ) ) ;
#45490=LINE ( 'NONE', #66288, #23600 ) ;
#45491=CARTESIAN_POINT ( 'NONE',  ( 126.3541873520043737, 37.07520218256170352, -44.02282603433466335 ) ) ;
#45492=ORIENTED_EDGE ( 'NONE', *, *, #3701, .T. ) ;
#45495=EDGE_CURVE ( 'NONE', #51871, #34356, #28526, .T. ) ;
#45497=CARTESIAN_POINT ( 'NONE',  ( 187.9556299234372148, 87.33837712034319622, 87.48685922188801101 ) ) ;
#45498=CARTESIAN_POINT ( 'NONE',  ( -15.22871623201694469, 7.486724405784662473, 9.545765994695932122 ) ) ;
#45500=CARTESIAN_POINT ( 'NONE',  ( -28.81317668042940738, 9.175023678939295380, -76.69123791734521944 ) ) ;
#45501=ADVANCED_FACE ( 'NONE', ( #39772 ), #43990, .F. ) ;
#45503=ADVANCED_FACE ( 'NONE', ( #18317 ), #33805, .F. ) ;
#45508=AXIS2_PLACEMENT_3D ( 'NONE', #25892, #25556, #68777 ) ;
#45509=CARTESIAN_POINT ( 'NONE',  ( -57.43883374585512769, 16.37892664338859205, -62.44644220765625420 ) ) ;
#45510=CARTESIAN_POINT ( 'NONE',  ( 199.7291770695760533, 101.4092159658447372, -65.04710708279223752 ) ) ;
#45513=CARTESIAN_POINT ( 'NONE',  ( -166.2028193222418793, 79.74385139484274987, 8.566800144892136260 ) ) ;
#45515=CARTESIAN_POINT ( 'NONE',  ( -47.80896875121164413, 12.85816703949530826, 66.62128856524451237 ) ) ;
#45516=AXIS2_PLACEMENT_3D ( 'NONE', #6256, #15446, #36897 ) ;
#45522=CARTESIAN_POINT ( 'NONE',  ( 15.78827728214693416, 7.507518794609596924, -89.20804527961313113 ) ) ;
#45526=ADVANCED_FACE ( 'NONE', ( #34516 ), #6718, .F. ) ;
#45529=CARTESIAN_POINT ( 'NONE',  ( -189.2776534485022069, 107.1424877329940841, -95.00000000000133582 ) ) ;
#45531=ORIENTED_EDGE ( 'NONE', *, *, #11573, .T. ) ;
#45534=CARTESIAN_POINT ( 'NONE',  ( 150.2060369882285329, 53.45752899907542144, 38.79508757824569898 ) ) ;
#45539=CARTESIAN_POINT ( 'NONE',  ( -0.8011128725815486185, 6.535315321814185729, 13.41110674575676853 ) ) ;
#45540=CARTESIAN_POINT ( 'NONE',  ( 55.91494169499919309, 12.16343363043256964, -40.79342870396418874 ) ) ;
#45541=CARTESIAN_POINT ( 'NONE',  ( -80.32755469740932597, 24.04130076192509335, 45.23585681520698643 ) ) ;
#45542=CARTESIAN_POINT ( 'NONE',  ( 152.9292068394840101, 54.20367164619623424, 84.59218010126255649 ) ) ;
#45543=CARTESIAN_POINT ( 'NONE',  ( 140.9169160367233360, 45.85398962664667977, 12.74973608567994354 ) ) ;
#45544=EDGE_LOOP ( 'NONE', ( #50748, #50594, #24223, #48246 ) ) ;
#45551=CARTESIAN_POINT ( 'NONE',  ( -118.5596554410405616, 41.85073040176283143, 93.41348078571337510 ) ) ;
#45552=ORIENTED_EDGE ( 'NONE', *, *, #9122, .F. ) ;
#45557=CARTESIAN_POINT ( 'NONE',  ( -142.8450945664714880, 58.72815783657286204, 68.52009029614266922 ) ) ;
#45558=CARTESIAN_POINT ( 'NONE',  ( 82.34401416830216647, 19.05992892018826623, 31.05207311871945564 ) ) ;
#45562=CARTESIAN_POINT ( 'NONE',  ( 188.5843222076478582, 86.53342480589847696, -16.58390079652848570 ) ) ;
#45563=CARTESIAN_POINT ( 'NONE',  ( 140.4586216751744701, 45.55624550472997925, -20.24665479566528248 ) ) ;
#45565=CARTESIAN_POINT ( 'NONE',  ( -180.5954680880247452, 97.44843622358463620, -16.00758145678837963 ) ) ;
#45566=EDGE_CURVE ( 'NONE', #21955, #60768, #65607, .T. ) ;
#45568=CARTESIAN_POINT ( 'NONE',  ( -48.34250119710923599, 14.01879126850789348, 34.45810225024617779 ) ) ;
#45569=ORIENTED_EDGE ( 'NONE', *, *, #39402, .T. ) ;
#45570=EDGE_LOOP ( 'NONE', ( #51776, #61305 ) ) ;
#45574=CARTESIAN_POINT ( 'NONE',  ( 188.4904153916304779, 86.42965364612516055, -44.94447516463474557 ) ) ;
#45575=CARTESIAN_POINT ( 'NONE',  ( -108.5289085648060592, 36.07014995015114778, 69.01860148035208908 ) ) ;
#45576=CARTESIAN_POINT ( 'NONE',  ( -24.32937228292060894, 8.531905774118440533, -45.25531289717756778 ) ) ;
#45580=EDGE_LOOP ( 'NONE', ( #34128, #21886 ) ) ;
#45585=CARTESIAN_POINT ( 'NONE',  ( -72.02029401400447739, 19.90008195119185075, 88.07226044993944924 ) ) ;
#45586=CARTESIAN_POINT ( 'NONE',  ( -79.14678386417816114, 22.50468917936073865, 72.26275173013684139 ) ) ;
#45587=DIRECTION ( 'NONE',  ( -0.000000000000000000, 1.000000000000000000, -0.000000000000000000 ) ) ;
#45590=CARTESIAN_POINT ( 'NONE',  ( -59.96408504033280451, 17.10126854471815605, 43.50660429605553503 ) ) ;
#45591=CARTESIAN_POINT ( 'NONE',  ( -95.86163447241558799, 30.75089131639704121, -19.58197702406704366 ) ) ;
#45592=CARTESIAN_POINT ( 'NONE',  ( 58.46823952472681896, 12.69204591816732552, 43.29726459483626400 ) ) ;
#45596=CARTESIAN_POINT ( 'NONE',  ( -6.126800896373026717, 6.786243985899687914, -50.22733277754976911 ) ) ;
#45602=B_SPLINE_CURVE_WITH_KNOTS ( 'NONE', 3,
 ( #57840, #46939, #3002, #47273, #20536, #52213, #67372, #25154, #25502, #20204, #31119, #30078, #35704, #41660, #67712, #63118, #19162, #25841, #62068, #19867, #46582, #42005, #52555, #4380, #56809, #3339, #24799, #46236, #19510, #68063, #40970, #62777, #14581, #37754, #64494, #21240, #26861, #48629, #59544, #15960, #42351, #20895, #31454, #59202, #10670, #26172, #52888, #42686, #5054, #16305, #4713, #58512, #6086, #11021, #48286, #32485 ),
 .UNSPECIFIED., .F., .F.,
 ( 4, 2, 2, 2, 2, 2, 2, 2, 2, 2, 2, 2, 2, 2, 2, 2, 2, 2, 2, 2, 2, 2, 2, 2, 2, 2, 2, 4 ),
 ( 0.000000000000000000, 0.001959203338812263041, 0.002938805008218370492, 0.003918406677624477509, 0.004898008347030584526, 0.005877610016436692411, 0.006857211685842799428, 0.007836813355248906446, 0.008816415024655013463, 0.009796016694061120481, 0.01175522003287333452, 0.01273482170227945888, 0.01371442337168558498, 0.01469402504109170761, 0.01567362671049783371, 0.01763283004931008244, 0.01959203338812233117, 0.02057163505752843818, 0.02155123672693454520, 0.02253083839634065569, 0.02351044006574676271, 0.02546964340455896286, 0.02644924507396507682, 0.02742884674337118731, 0.02840844841277729779, 0.02938805008218340481, 0.03036765175158951877, 0.03134725342099562578 ),
 .UNSPECIFIED. ) ;
#45603=CARTESIAN_POINT ( 'NONE',  ( 126.4219470349615619, 38.26519385429182307, -15.65615810876642655 ) ) ;
#45605=ORIENTED_EDGE ( 'NONE', *, *, #10010, .F. ) ;
#45608=CARTESIAN_POINT ( 'NONE',  ( 126.3732561463888402, 38.23795180971328023, -44.08787207326391666 ) ) ;
#45609=CARTESIAN_POINT ( 'NONE',  ( -38.68632430131782485, 11.91908191268691475, -40.87075332870919198 ) ) ;
#45613=CARTESIAN_POINT ( 'NONE',  ( -174.2769963701057634, 88.42283341462002966, 84.58341184452997652 ) ) ;
#45614=ORIENTED_EDGE ( 'NONE', *, *, #13111, .F. ) ;
#45615=VECTOR ( 'NONE', #45249, 1000.000000000000000 ) ;
#45616=CARTESIAN_POINT ( 'NONE',  ( 126.6464677212869532, 38.39096133771045061, 8.034511553305282661 ) ) ;
#45619=B_SPLINE_CURVE_WITH_KNOTS ( 'NONE', 3,
 ( #50134, #1959, #27972, #49416, #38890, #66336, #18128, #34310, #55758, #7584, #29038, #23750, #45196, #66675, #18472, #52206, #68053, #30758, #36030, #3670, #34999, #57488, #9295, #61719, #56440, #62061, #29369, #13876, #63107, #4022, #46576, #19857, #41314, #25491, #7919, #40961, #40271, #3331, #8959, #46230, #30406, #20196, #30072, #67706 ),
 .UNSPECIFIED., .F., .F.,
 ( 4, 2, 2, 2, 2, 2, 2, 2, 2, 2, 2, 2, 2, 2, 2, 2, 2, 2, 2, 2, 2, 4 ),
 ( 6.938893903907227607E-18, 0.001473754749730481336, 0.002210632124595723631, 0.002947509499460966142, 0.004421264249191440322, 0.005895018998921913202, 0.007368773748652386081, 0.008105651123517621653, 0.008842528498382856358, 0.01031628324811331883, 0.01179003799784377957, 0.01252691537270901080, 0.01326379274757424551, 0.01473754749730471839, 0.01547442487216995656, 0.01621130224703519473, 0.01768505699676566414, 0.01915881174649614049, 0.01989568912136138040, 0.02063256649622662031, 0.02210632124595709319, 0.02358007599568756954 ),
 .UNSPECIFIED. ) ;
#45621=VECTOR ( 'NONE', #65190, 1000.000000000000000 ) ;
#45623=CARTESIAN_POINT ( 'NONE',  ( 198.4045886930829283, 99.71425793793709147, 5.774369385283677047 ) ) ;
#45624=EDGE_LOOP ( 'NONE', ( #53392, #48606 ) ) ;
#45627=CARTESIAN_POINT ( 'NONE',  ( 163.5430354047457229, 63.84092878795252801, 94.99999999999866418 ) ) ;
#45629=CARTESIAN_POINT ( 'NONE',  ( -55.05276343752909440, 15.72344139423348430, 18.47277718246750311 ) ) ;
#45632=DIRECTION ( 'NONE',  ( 0.000000000000000000, -0.000000000000000000, -1.000000000000000000 ) ) ;
#45636=CARTESIAN_POINT ( 'NONE',  ( 55.57657751403269941, 11.06944050856661832, 36.32677378882770824 ) ) ;
#45639=CARTESIAN_POINT ( 'NONE',  ( -168.0052514572427071, 83.06849406765624622, 16.96694403013009733 ) ) ;
#45640=CARTESIAN_POINT ( 'NONE',  ( 19.74724861314306068, 6.659670522263893666, -76.23824785690877093 ) ) ;
#45641=CARTESIAN_POINT ( 'NONE',  ( -132.9227230387960788, 52.53474289881227577, 67.59429576175594434 ) ) ;
#45642=ORIENTED_EDGE ( 'NONE', *, *, #30434, .T. ) ;
#45643=CARTESIAN_POINT ( 'NONE',  ( -95.90733500870057071, 30.77270007533267560, 87.74079889594401038 ) ) ;
#45649=EDGE_CURVE ( 'NONE', #34130, #24352, #67243, .T. ) ;
#45652=ADVANCED_FACE ( 'NONE', ( #53413 ), #26365, .F. ) ;
#45653=CARTESIAN_POINT ( 'NONE',  ( 181.0840389613909451, 80.03940679743416808, -9.380507075415923879 ) ) ;
#45654=CARTESIAN_POINT ( 'NONE',  ( -133.1566699306513328, 52.70203339370770124, 9.385161963150576270 ) ) ;
#45655=CARTESIAN_POINT ( 'NONE',  ( 70.41705859591009187, 15.55317472777717569, -71.30260546593714821 ) ) ;
#45656=ORIENTED_EDGE ( 'NONE', *, *, #46793, .F. ) ;
#45660=DIRECTION ( 'NONE',  ( 0.000000000000000000, 0.000000000000000000, 1.000000000000000000 ) ) ;
#45662=CARTESIAN_POINT ( 'NONE',  ( -48.19921232700619385, 12.95035395002356182, -93.32826121341297210 ) ) ;
#45665=CARTESIAN_POINT ( 'NONE',  ( -148.6426981422628728, 63.44891673852537650, 30.75816665846506481 ) ) ;
#45666=CARTESIAN_POINT ( 'NONE',  ( -129.6165111262477296, 48.99406349865701316, 58.44935411866086383 ) ) ;
#45667=CARTESIAN_POINT ( 'NONE',  ( -76.79042791651912125, 22.68960395613480330, -8.505398727429060557 ) ) ;
#45670=CARTESIAN_POINT ( 'NONE',  ( -102.2801239173131194, 33.91021738430207932, 45.51907450641513009 ) ) ;
#45672=CARTESIAN_POINT ( 'NONE',  ( 33.44527180510250020, 7.709232309484709944, 32.83041950400863840 ) ) ;
#45674=CARTESIAN_POINT ( 'NONE',  ( 84.05289558242219528, 19.61733656419350424, 57.00898428369665538 ) ) ;
#45681=CARTESIAN_POINT ( 'NONE',  ( -11.57950265606958062, 8.174070387114795722, -36.42061191550288157 ) ) ;
#45682=CARTESIAN_POINT ( 'NONE',  ( 154.4429418375332830, 55.33424769452791736, -50.50089971109889575 ) ) ;
#45684=CARTESIAN_POINT ( 'NONE',  ( -108.6232015645744866, 36.12159103445661401, -92.19520623112163094 ) ) ;
#45685=CARTESIAN_POINT ( 'NONE',  ( -156.8764584803562343, 70.69066846313523911, -16.89224324630464835 ) ) ;
#45688=CARTESIAN_POINT ( 'NONE',  ( -60.47589866267034608, 17.25153113855766307, 59.47546330872564369 ) ) ;
#45692=CARTESIAN_POINT ( 'NONE',  ( 152.8373718734504507, 55.38925997611392660, -64.55073842685702346 ) ) ;
#45693=CARTESIAN_POINT ( 'NONE',  ( -31.43908319763709969, 9.591432048623765638, 30.21645440618916112 ) ) ;
#45694=CARTESIAN_POINT ( 'NONE',  ( 139.2921620648436942, 44.80435067172502528, -48.71413097721568874 ) ) ;
#45697=CARTESIAN_POINT ( 'NONE',  ( -152.9008427825210390, 68.45483453645053373, 58.37314777991063153 ) ) ;
#45698=CARTESIAN_POINT ( 'NONE',  ( -120.4816138481825050, 43.03185659245511374, 32.90506872955344875 ) ) ;
#45700=LINE ( 'NONE', #62576, #59342 ) ;
#45701=CARTESIAN_POINT ( 'NONE',  ( 127.7775657355649486, 39.02916686230897625, 86.25207957938988557 ) ) ;
#45704=DIRECTION ( 'NONE',  ( -1.000000000000000000, 0.000000000000000000, 0.000000000000000000 ) ) ;
#45708=VERTEX_POINT ( 'NONE', #54095 ) ;
#45709=CARTESIAN_POINT ( 'NONE',  ( 164.8886903222556839, 63.65672212134877839, -17.91909660570943430 ) ) ;
#45712=CARTESIAN_POINT ( 'NONE',  ( 68.93219921887765622, 14.12322281954860514, 59.54178852774079189 ) ) ;
#45713=CARTESIAN_POINT ( 'NONE',  ( 141.3400002717723112, 47.33399859146520328, 10.73346743848780704 ) ) ;
#45718=CARTESIAN_POINT ( 'NONE',  ( 164.6561571795775194, 64.77723933022095082, -14.56007165210607646 ) ) ;
#45720=AXIS2_PLACEMENT_3D ( 'NONE', #68891, #53057, #47104 ) ;
#45721=CARTESIAN_POINT ( 'NONE',  ( 68.62997155117719217, 15.08415013720828668, 69.15437636595807191 ) ) ;
#45722=CARTESIAN_POINT ( 'NONE',  ( 134.5554110091750601, 41.84687667739064665, 83.20593790981784821 ) ) ;
#45724=CARTESIAN_POINT ( 'NONE',  ( 163.7403496014744633, 64.00600007368876732, -47.74785624616011148 ) ) ;
#45727=CARTESIAN_POINT ( 'NONE',  ( 157.9130201331580849, 57.99550255803048771, -51.12418429913767426 ) ) ;
#45731=CARTESIAN_POINT ( 'NONE',  ( 67.36631071204163845, 14.76099193472943405, 84.85725114640790423 ) ) ;
#45733=CARTESIAN_POINT ( 'NONE',  ( 79.52639011421921111, 18.17129627604990816, -14.01688966035989559 ) ) ;
#45735=CARTESIAN_POINT ( 'NONE',  ( -166.7068579965637127, 80.26142964949322334, 34.42591652138479930 ) ) ;
#45736=CARTESIAN_POINT ( 'NONE',  ( -145.2470175691743748, 60.64833472287889293, -89.82575223439511092 ) ) ;
#45737=CARTESIAN_POINT ( 'NONE',  ( 129.1137093889808511, 38.63348691920620581, -76.18274731194584604 ) ) ;
#45740=CARTESIAN_POINT ( 'NONE',  ( -11.56945424397728495, 8.173256823723111353, 57.95689558190326096 ) ) ;
#45744=DIRECTION ( 'NONE',  ( 0.000000000000000000, 0.000000000000000000, 1.000000000000000000 ) ) ;
#45746=CARTESIAN_POINT ( 'NONE',  ( -0.5658006089934878302, 7.533733779014709420, 35.66903967604532255 ) ) ;
#45748=DIRECTION ( 'NONE',  ( -0.8118923937861950435, -0.5838071093367415143, 0.000000000000000000 ) ) ;
#45749=CARTESIAN_POINT ( 'NONE',  ( -48.56549579811110817, 13.03742088415616429, -65.76502786008495605 ) ) ;
#45750=CARTESIAN_POINT ( 'NONE',  ( -7.336630171688593549, 7.867399454768229106, -23.57352014148015584 ) ) ;
#45751=CARTESIAN_POINT ( 'NONE',  ( 175.5406524085946103, 73.17873692326776336, 4.886636635488581071 ) ) ;
#45752=CARTESIAN_POINT ( 'NONE',  ( -59.95707852844800811, 16.05120821151901822, 5.276972445045120530 ) ) ;
#45754=VECTOR ( 'NONE', #16074, 1000.000000000000000 ) ;
#45755=CARTESIAN_POINT ( 'NONE',  ( -97.86516199987804043, 31.71158167298306907, -48.59635491045797551 ) ) ;
#45756=ORIENTED_EDGE ( 'NONE', *, *, #27435, .F. ) ;
#45757=CARTESIAN_POINT ( 'NONE',  ( 103.0026233023292974, 25.67408295205787283, -72.29030188102200327 ) ) ;
#45763=CARTESIAN_POINT ( 'NONE',  ( 63.01563776193091826, 12.67277567978500308, 2.968410348757589023 ) ) ;
#45766=CIRCLE ( 'NONE', #6440, 242.4895526022646379 ) ;
#45769=VECTOR ( 'NONE', #22529, 1000.000000000000000 ) ;
#45770=CARTESIAN_POINT ( 'NONE',  ( -173.1211646369891071, 87.12891641440857882, 57.66624519710472185 ) ) ;
#45775=CARTESIAN_POINT ( 'NONE',  ( 175.8963338753314360, 73.51705463274396379, -11.45839974079307666 ) ) ;
#45776=CARTESIAN_POINT ( 'NONE',  ( -172.3127615181935539, 87.73358064377640630, 57.69864198530328991 ) ) ;
#45778=CARTESIAN_POINT ( 'NONE',  ( 57.41085175769454452, 12.46982565415947519, -21.36584457835558126 ) ) ;
#45781=CARTESIAN_POINT ( 'NONE',  ( 19.54452863209719382, 7.657034792877148277, -36.50889906614686709 ) ) ;
#45782=CARTESIAN_POINT ( 'NONE',  ( 8.537735592981553268, 7.383000420390735563, 66.29318622724315446 ) ) ;
#45784=FACE_BOUND ( 'NONE', #1402, .T. ) ;
#45785=VERTEX_POINT ( 'NONE', #59393 ) ;
#45786=ORIENTED_EDGE ( 'NONE', *, *, #68458, .F. ) ;
#45790=CARTESIAN_POINT ( 'NONE',  ( 37.70910994512003356, 9.209110272746707793, -77.27493779074411862 ) ) ;
#45791=CARTESIAN_POINT ( 'NONE',  ( -178.2448732545370547, 94.58403736950704399, 16.97374245720416752 ) ) ;
#45792=CARTESIAN_POINT ( 'NONE',  ( 8.619049365873218349, 6.376996852107025937, 88.97686130232474966 ) ) ;
#45793=DIRECTION ( 'NONE',  ( 0.000000000000000000, -1.000000000000000000, 0.000000000000000000 ) ) ;
#45795=ORIENTED_EDGE ( 'NONE', *, *, #3578, .T. ) ;
#45796=DIRECTION ( 'NONE',  ( -0.000000000000000000, 1.000000000000000000, -0.000000000000000000 ) ) ;
#45797=CARTESIAN_POINT ( 'NONE',  ( 197.2199569260503722, 98.22436319491366419, -43.16215066073257844 ) ) ;
#45800=DIRECTION ( 'NONE',  ( -0.000000000000000000, 1.000000000000000000, -0.000000000000000000 ) ) ;
#45802=CARTESIAN_POINT ( 'NONE',  ( -84.55373779407977963, 24.65190748253136377, -74.13279789683143406 ) ) ;
#45804=CARTESIAN_POINT ( 'NONE',  ( 87.10672734544988316, 20.64813880796638301, -77.66611478937542756 ) ) ;
#45808=CARTESIAN_POINT ( 'NONE',  ( 43.35536254672140899, 9.973606330917817786, 57.88029466200895001 ) ) ;
#45809=CARTESIAN_POINT ( 'NONE',  ( -103.9557308419433639, 34.77357682180773679, -88.88104893678155349 ) ) ;
#45810=CARTESIAN_POINT ( 'NONE',  ( 23.24028701062093205, 6.853614888934259852, 11.64810109089808066 ) ) ;
#45816=CARTESIAN_POINT ( 'NONE',  ( 117.6865880453676141, 32.48051379280605744, -17.63313866224432758 ) ) ;
#45817=CARTESIAN_POINT ( 'NONE',  ( 81.04027388895735839, 18.64386073872848826, -38.29630275601382294 ) ) ;
#45818=CARTESIAN_POINT ( 'NONE',  ( -168.2905794219380198, 83.36949033555949029, -90.14733823562677628 ) ) ;
#45819=VERTEX_POINT ( 'NONE', #11539 ) ;
#45821=EDGE_CURVE ( 'NONE', #7307, #46840, #1011, .T. ) ;
#45822=ORIENTED_EDGE ( 'NONE', *, *, #11286, .T. ) ;
#45823=CARTESIAN_POINT ( 'NONE',  ( 45.04360969585142271, 9.210232288266691825, 15.53527602477098135 ) ) ;
#45825=CARTESIAN_POINT ( 'NONE',  ( -51.35181696773306470, 13.72007042346227124, -22.41355051264525500 ) ) ;
#45827=CARTESIAN_POINT ( 'NONE',  ( 199.7278513351970730, 99.76879341361765796, 15.49925635273226376 ) ) ;
#45828=CARTESIAN_POINT ( 'NONE',  ( -25.25491181982865285, 8.657665838245407031, -92.24093140373469168 ) ) ;
#45829=CARTESIAN_POINT ( 'NONE',  ( 207.0530270305075078, 111.3805688245614363, 83.25676956866661271 ) ) ;
#45831=CARTESIAN_POINT ( 'NONE',  ( -75.64857587248464199, 21.19501514561450506, -62.58980599074443063 ) ) ;
#45832=CARTESIAN_POINT ( 'NONE',  ( -15.32550079334879278, 7.496023944924843363, 37.37366452483693990 ) ) ;
#45833=ORIENTED_EDGE ( 'NONE', *, *, #38766, .T. ) ;
#45836=CARTESIAN_POINT ( 'NONE',  ( 197.6145711261844724, 97.10888456119684520, -19.52788035905484776 ) ) ;
#45839=FACE_OUTER_BOUND ( 'NONE', #48360, .T. ) ;
#45840=CARTESIAN_POINT ( 'NONE',  ( 185.1710994180822638, 84.30654632312744923, -64.26513029063508498 ) ) ;
#45841=CARTESIAN_POINT ( 'NONE',  ( -165.6208371326873703, 80.58821715390999429, 38.02385811616766631 ) ) ;
#45845=CARTESIAN_POINT ( 'NONE',  ( 8.683910719548894264, 7.383368463746302623, -45.43529509856040249 ) ) ;
#45846=CARTESIAN_POINT ( 'NONE',  ( 130.7260704202054455, 39.56565398554878499, -50.35476434615378594 ) ) ;
#45850=CARTESIAN_POINT ( 'NONE',  ( 188.0498085889633728, 87.44272287964741963, 93.28420891864679731 ) ) ;
#45854=B_SPLINE_CURVE_WITH_KNOTS ( 'NONE', 3,
 ( #18140, #13558, #8285, #34681, #50147, #7597, #39595, #2316, #1607, #45558, #50494, #44869, #39253, #29053, #1972, #62078, #40622, #7239, #66353, #39937, #13897, #7932, #18485, #61394, #61046, #35360, #56820, #56116, #67041, #65997, #8636, #34329, #12871, #55777, #24468, #35012, #60697, #49781, #23069, #2657, #12513, #23766, #33973, #50839 ),
 .UNSPECIFIED., .F., .F.,
 ( 4, 2, 2, 2, 2, 2, 2, 2, 2, 2, 2, 2, 2, 2, 2, 2, 2, 2, 2, 2, 2, 4 ),
 ( 0.02416815208377490892, 0.02567033257376875877, 0.02642142281876568716, 0.02717251306376261208, 0.02867469355375646192, 0.02942578379875337297, 0.03017687404375027707, 0.03167905453374409569, 0.03318123502373791778, 0.03393232526873483229, 0.03468341551373174680, 0.03618559600372561053, 0.03693668624872255279, 0.03768777649371949506, 0.03918995698371335878, 0.04069213747370722944, 0.04219431796370108623, 0.04369649845369495689, 0.04444758869869189222, 0.04519867894368882755, 0.04670085943368268433, 0.04820303992367654111 ),
 .UNSPECIFIED. ) ;
#45857=CARTESIAN_POINT ( 'NONE',  ( 10.83418588031599228, 6.392467435475930770, 5.017533756073925488 ) ) ;
#45862=CARTESIAN_POINT ( 'NONE',  ( 200.4590013143046292, 102.3556155835302945, -76.87509902206629420 ) ) ;
#45863=CARTESIAN_POINT ( 'NONE',  ( -178.7458319892713519, 93.61502008198021940, -37.24441981830012338 ) ) ;
#45865=CARTESIAN_POINT ( 'NONE',  ( -23.95089599695169014, 9.496585844566174828, 64.07248978537857909 ) ) ;
#45867=CARTESIAN_POINT ( 'NONE',  ( -49.11825192196928214, 13.17012322555986970, 69.27432531549762018 ) ) ;
#45868=AXIS2_PLACEMENT_3D ( 'NONE', #38205, #60709, #54369 ) ;
#45869=CARTESIAN_POINT ( 'NONE',  ( -5.885876544836654567, 6.772369038004114827, 57.21109972859309778 ) ) ;
#45872=CARTESIAN_POINT ( 'NONE',  ( -128.7810612886105446, 48.42424427998344783, -76.18402560349873909 ) ) ;
#45874=CARTESIAN_POINT ( 'NONE',  ( -53.13004807512037786, 14.17398740785106526, -35.45065378176567350 ) ) ;
#45875=B_SPLINE_CURVE_WITH_KNOTS ( 'NONE', 3,
 ( #5687, #16596, #48931, #21524, #38052, #44014, #27147, #5357, #66, #32781, #10972, #11309, #65142, #33135, #419, #16249, #38760, #42969, #1466, #21870, #43315, #64792, #33493, #16936, #59497, #28188, #60202, #773, #43663, #38400, #59841, #54209, #11662, #6033, #22225, #54569, #54916, #39118, #6396, #6740, #48578, #32438, #64440, #65491, #27848 ),
 .UNSPECIFIED., .F., .F.,
 ( 4, 2, 2, 2, 2, 2, 2, 2, 2, 2, 2, 2, 2, 1, 2, 2, 2, 2, 2, 2, 2, 2, 4 ),
 ( 0.02356759485890611364, 0.02503765354686409914, 0.02577268289084310229, 0.02650771223482210198, 0.02797777092278013258, 0.02944782961073816319, 0.03018285895471718369, 0.03091788829869620420, 0.03238794698665421745, 0.03312297633063322755, 0.03385800567461224458, 0.03532806436257030641, 0.03606309370654933733, 0.03679812305052836824, 0.03753315239450739915, 0.03826818173848643700, 0.03973824042644454047, 0.04120829911440264393, 0.04267835780236074045, 0.04341338714633979912, 0.04414841649031885779, 0.04561847517827697512, 0.04708853386623509246 ),
 .UNSPECIFIED. ) ;
#45880=CARTESIAN_POINT ( 'NONE',  ( -189.3836756007636950, 107.2890649608328459, -94.27226266387080500 ) ) ;
#45886=CARTESIAN_POINT ( 'NONE',  ( 155.7167524447090443, 57.56687707799948583, 44.21502333676962593 ) ) ;
#45890=CARTESIAN_POINT ( 'NONE',  ( -180.6011569556095537, 95.85968111394264213, 10.84709140346148715 ) ) ;
#45891=CARTESIAN_POINT ( 'NONE',  ( -2.355184675731022192, 6.596450510445357907, 5.634252349864039999 ) ) ;
#45892=CARTESIAN_POINT ( 'NONE',  ( 57.07246224906423748, 12.39953617563784682, -38.61949813100464013 ) ) ;
#45894=CARTESIAN_POINT ( 'NONE',  ( 157.2737841094199780, 57.49822297871171628, 83.09519871651045264 ) ) ;
#45895=CARTESIAN_POINT ( 'NONE',  ( 136.9934874058118339, 43.35050367224294376, 16.99398237304345827 ) ) ;
#45896=EDGE_CURVE ( 'NONE', #59205, #30284, #51278, .T. ) ;
#45897=ORIENTED_EDGE ( 'NONE', *, *, #16102, .F. ) ;
#45901=CARTESIAN_POINT ( 'NONE',  ( -76.79042791651912125, 22.68960395613480330, 18.33915186303461553 ) ) ;
#45904=CARTESIAN_POINT ( 'NONE',  ( -190.6985136298601731, 109.1272424661242582, -95.00000000000133582 ) ) ;
#45907=CARTESIAN_POINT ( 'NONE',  ( 81.74909803672913711, 17.81295302817862947, -49.03814682348451726 ) ) ;
#45910=CARTESIAN_POINT ( 'NONE',  ( -149.5074843970971017, 64.17983161892347255, 72.56537183036277838 ) ) ;
#45911=CARTESIAN_POINT ( 'NONE',  ( 157.4703587214989398, -170.0000000000000000, 2.564916881789689462 ) ) ;
#45915=CARTESIAN_POINT ( 'NONE',  ( -80.31482177285911916, 24.03632224640838544, -23.09139861995610232 ) ) ;
#45916=CARTESIAN_POINT ( 'NONE',  ( -173.1211646369891355, 88.63826465341151106, -22.86740657428632773 ) ) ;
#45917=CARTESIAN_POINT ( 'NONE',  ( -52.00092620775817664, 14.92276858858357258, 30.96201563046714256 ) ) ;
#45921=CARTESIAN_POINT ( 'NONE',  ( -109.7811201291769692, 37.90784085457602970, 11.40485209265354172 ) ) ;
#45922=CARTESIAN_POINT ( 'NONE',  ( 103.8317086684999850, 26.02720265156212776, 67.85564866584407184 ) ) ;
#45923=CARTESIAN_POINT ( 'NONE',  ( 164.0158927577712973, 62.92463143894071465, 60.05433321578705375 ) ) ;
#45924=CARTESIAN_POINT ( 'NONE',  ( -190.4966031023458584, 108.8421921967458985, 69.44444822291313812 ) ) ;
#45925=ADVANCED_FACE ( 'NONE', ( #3104 ), #40379, .F. ) ;
#45926=EDGE_CURVE ( 'NONE', #8631, #17554, #18633, .T. ) ;
#45927=CARTESIAN_POINT ( 'NONE',  ( 187.5272808203428383, 85.37192123373907293, -47.60191362853060326 ) ) ;
#45928=FACE_OUTER_BOUND ( 'NONE', #57703, .T. ) ;
#45929=CARTESIAN_POINT ( 'NONE',  ( -142.1220711180391731, 59.43943186025860825, 90.55661759554712376 ) ) ;
#45933=CARTESIAN_POINT ( 'NONE',  ( -7.825402957745087207, -170.0000000000000000, 64.46013162991090439 ) ) ;
#45934=CARTESIAN_POINT ( 'NONE',  ( 181.0840389613909736, 78.60582251573003987, -89.91415884680696990 ) ) ;
#45935=CARTESIAN_POINT ( 'NONE',  ( 68.93219921887762780, 14.12322281954860337, -47.83641383411398351 ) ) ;
#45937=CARTESIAN_POINT ( 'NONE',  ( 8.000000000000007105, 249.8719672152120381, 94.99999999999866418 ) ) ;
#45938=CARTESIAN_POINT ( 'NONE',  ( -94.83794676023107684, 30.26879337035744300, -14.60722893403272415 ) ) ;
#45939=CARTESIAN_POINT ( 'NONE',  ( 55.99998955208976525, 12.18058389017405041, 39.97614766549666143 ) ) ;
#45940=CARTESIAN_POINT ( 'NONE',  ( 32.64625186056120043, 7.626510506539066370, 94.42831398130083187 ) ) ;
#45941=ORIENTED_EDGE ( 'NONE', *, *, #18110, .F. ) ;
#45942=CARTESIAN_POINT ( 'NONE',  ( -0.5183605925911975998, 6.525266619725955231, -44.62597692609903532 ) ) ;
#45944=CARTESIAN_POINT ( 'NONE',  ( -121.5921196778231348, 43.72569502503144179, 5.113650806495113166 ) ) ;
#45947=CARTESIAN_POINT ( 'NONE',  ( 19.10949903373831305, 7.636938177523838078, -22.90343416015605271 ) ) ;
#45954=CARTESIAN_POINT ( 'NONE',  ( -128.1384526288950099, 47.98891607499718504, 4.104498430499266881 ) ) ;
#45960=CARTESIAN_POINT ( 'NONE',  ( 133.8566784816069060, 42.60093787723653236, 2.665790248531674678 ) ) ;
#45964=CARTESIAN_POINT ( 'NONE',  ( 203.1423857108908351, 105.9238244286949708, 2.515585502045935673 ) ) ;
#45967=CARTESIAN_POINT ( 'NONE',  ( 154.6089187792045436, 56.72139871926570009, 83.65894979668894393 ) ) ;
#45969=CARTESIAN_POINT ( 'NONE',  ( 130.7457207912711112, 40.74300766298684096, -77.20782277390614468 ) ) ;
#45971=CARTESIAN_POINT ( 'NONE',  ( -156.6644740249450365, 71.86407434531899696, 35.96180702756684866 ) ) ;
#45977=CARTESIAN_POINT ( 'NONE',  ( 56.53776994993147298, 11.26292242501182628, 41.10093067265479050 ) ) ;
#45979=EDGE_CURVE ( 'NONE', #67324, #63280, #46689, .T. ) ;
#45981=CARTESIAN_POINT ( 'NONE',  ( -165.7149569557575717, 80.68479365246975021, 12.69795252626694726 ) ) ;
#45982=CARTESIAN_POINT ( 'NONE',  ( 22.53041628628730209, 6.810083298012988173, -66.54146030137279411 ) ) ;
#45984=CARTESIAN_POINT ( 'NONE',  ( -133.3220917939970036, 52.82057604964899156, 66.03414425393503961 ) ) ;
#45986=CARTESIAN_POINT ( 'NONE',  ( -95.74211766252655309, 30.69445205485278905, 88.01871795480677463 ) ) ;
#45987=CARTESIAN_POINT ( 'NONE',  ( -78.19438069111008360, 23.21811806230640585, -50.11545063171791270 ) ) ;
#45989=CARTESIAN_POINT ( 'NONE',  ( 179.7110760798946103, 78.65068260568622804, -90.03270647271450855 ) ) ;
#45990=CARTESIAN_POINT ( 'NONE',  ( 140.0820590176526252, 46.51134312115248548, 32.82017767266312802 ) ) ;
#45992=CARTESIAN_POINT ( 'NONE',  ( -131.3096895243911320, 51.39228038925229924, 16.48646959509930454 ) ) ;
#45993=CARTESIAN_POINT ( 'NONE',  ( 63.99027454648602031, 13.93445177372599275, -77.51741006307621262 ) ) ;
#45996=CARTESIAN_POINT ( 'NONE',  ( -148.6471085600700235, 64.76880961642447687, -22.93139458300547062 ) ) ;
#45997=CARTESIAN_POINT ( 'NONE',  ( 104.0290905220488469, 27.20720373712009987, 94.99999999999866418 ) ) ;
#46000=VECTOR ( 'NONE', #58238, 1000.000000000000000 ) ;
#46001=DIRECTION ( 'NONE',  ( -0.000000000000000000, 1.000000000000000000, -0.000000000000000000 ) ) ;
#46002=CARTESIAN_POINT ( 'NONE',  ( -52.14348496666676169, 14.95896524672374106, -89.47939421337314059 ) ) ;
#46005=CARTESIAN_POINT ( 'NONE',  ( 70.26639875985992489, 15.51307715494295891, -41.23871606255404032 ) ) ;
#46006=CARTESIAN_POINT ( 'NONE',  ( -122.3994536713185681, 45.42826354555018042, 44.76030098624846687 ) ) ;
#46007=CARTESIAN_POINT ( 'NONE',  ( 206.6955592216989714, 109.1214665502617578, 56.31174107073355373 ) ) ;
#46009=CARTESIAN_POINT ( 'NONE',  ( -109.7156874346698032, 37.87149323084329211, 39.03482595553440859 ) ) ;
#46011=CARTESIAN_POINT ( 'NONE',  ( -37.92511097250854135, 10.74631978746599614, 14.64581220136760109 ) ) ;
#46012=EDGE_LOOP ( 'NONE', ( #66839, #50096 ) ) ;
#46018=CARTESIAN_POINT ( 'NONE',  ( -9.779603649692296230, 8.034615131607072414, -35.66029398720795029 ) ) ;
#46022=CARTESIAN_POINT ( 'NONE',  ( -108.9724455943903934, 36.31238718243987051, -92.78713564447804174 ) ) ;
#46024=CARTESIAN_POINT ( 'NONE',  ( -56.97107423601133291, 15.20373812575556194, 30.55074923349853577 ) ) ;
#46025=CARTESIAN_POINT ( 'NONE',  ( -61.52761555060400411, 17.56359742150279857, 60.84458079513598250 ) ) ;
#46029=CARTESIAN_POINT ( 'NONE',  ( -15.22871623201694113, 7.486724405784663361, -70.98788577669509436 ) ) ;
#46030=CARTESIAN_POINT ( 'NONE',  ( -37.07086358537073068, 10.58360809068249786, 42.69363681085601314 ) ) ;
#46032=CARTESIAN_POINT ( 'NONE',  ( 141.0645618855930081, 45.95036951196539832, -45.66291655381088077 ) ) ;
#46036=CARTESIAN_POINT ( 'NONE',  ( -125.4433371161043880, 46.19736518073188591, 45.61994787315710909 ) ) ;
#46037=CARTESIAN_POINT ( 'NONE',  ( -60.97011009284707939, 16.34812508431679490, -38.08186052385045883 ) ) ;
#46039=CARTESIAN_POINT ( 'NONE',  ( 8.000000000000007105, 249.8719672152120381, -95.00000000000133582 ) ) ;
#46040=CARTESIAN_POINT ( 'NONE',  ( 93.08533330311587406, 21.72562315962719381, 60.20712453432130218 ) ) ;
#46042=CARTESIAN_POINT ( 'NONE',  ( 91.76185853696540562, 21.23554806651647908, -91.48147536935182700 ) ) ;
#46044=CARTESIAN_POINT ( 'NONE',  ( -125.8938041572051105, 46.49392987655492959, -61.75825448869760237 ) ) ;
#46045=ORIENTED_EDGE ( 'NONE', *, *, #2975, .T. ) ;
#46046=CARTESIAN_POINT ( 'NONE',  ( 198.4017331595409246, 98.09114638179336509, 32.62335811823028564 ) ) ;
#46048=CARTESIAN_POINT ( 'NONE',  ( 69.74037587279242700, 14.33355757956376308, 67.51542470792016104 ) ) ;
#46049=CARTESIAN_POINT ( 'NONE',  ( 187.8408212037641363, 85.71485242454924958, -94.12920833377788199 ) ) ;
#46052=ORIENTED_EDGE ( 'NONE', *, *, #63990, .F. ) ;
#46053=ADVANCED_FACE ( 'NONE', ( #10431 ), #48060, .T. ) ;
#46054=CARTESIAN_POINT ( 'NONE',  ( 160.4986104110022609, 61.33701824525267199, -9.914387348297012181 ) ) ;
#46056=CARTESIAN_POINT ( 'NONE',  ( 69.83260694998124052, 15.39825517924928633, 67.29435474199121359 ) ) ;
#46057=CARTESIAN_POINT ( 'NONE',  ( 130.8547135988932837, 39.64036133002733919, 83.79612325623102720 ) ) ;
#46058=EDGE_CURVE ( 'NONE', #18538, #65633, #32591, .T. ) ;
#46062=CARTESIAN_POINT ( 'NONE',  ( 164.9540180502650628, 65.02981548735053252, -43.05572303975047532 ) ) ;
#46065=EDGE_CURVE ( 'NONE', #5954, #29355, #26838, .T. ) ;
#46066=CARTESIAN_POINT ( 'NONE',  ( 158.3595886390531859, 58.34525996025800509, -51.08445656034285065 ) ) ;
#46069=CARTESIAN_POINT ( 'NONE',  ( 56.05126732939165635, 12.19092237165827797, 93.80575097029306164 ) ) ;
#46071=CARTESIAN_POINT ( 'NONE',  ( 80.16761386260783695, 18.37011649821943848, -20.31712373240189606 ) ) ;
#46072=CARTESIAN_POINT ( 'NONE',  ( -176.9221788447023584, 93.01200774825315420, -89.43217687938971494 ) ) ;
#46073=CARTESIAN_POINT ( 'NONE',  ( 154.4429418375333114, 55.33424769452792447, 56.87730265075583702 ) ) ;
#46074=CARTESIAN_POINT ( 'NONE',  ( 93.08174259058947086, 22.79847752828721141, 41.06691016658683679 ) ) ;
#46075=ORIENTED_EDGE ( 'NONE', *, *, #52860, .F. ) ;
#46076=CARTESIAN_POINT ( 'NONE',  ( -95.60805465865861663, 30.63099276904602775, 61.40042467303059226 ) ) ;
#46077=CARTESIAN_POINT ( 'NONE',  ( -13.77312480593388955, 8.361845410302542803, 59.88460182822674227 ) ) ;
#46080=CARTESIAN_POINT ( 'NONE',  ( 150.4542242713869484, 53.63744268572191487, -14.11560879282218650 ) ) ;
#46084=CARTESIAN_POINT ( 'NONE',  ( 61.40252071262365519, 12.30418078306080432, 83.67024983266009031 ) ) ;
#46086=CARTESIAN_POINT ( 'NONE',  ( -54.08504625707234226, 14.42374043447185450, -62.10766578188960807 ) ) ;
#46087=CARTESIAN_POINT ( 'NONE',  ( -1.866625526081660214, 7.583073082893622363, -11.49243256803911706 ) ) ;
#46088=CARTESIAN_POINT ( 'NONE',  ( 177.5945652320813792, 75.14951358071816401, 16.60670449205189669 ) ) ;
#46089=CARTESIAN_POINT ( 'NONE',  ( -31.43908319763709969, 10.61114334766715928, -50.31719736520186359 ) ) ;
#46090=EDGE_LOOP ( 'NONE', ( #37435, #42031, #41001, #3615 ) ) ;
#46093=CARTESIAN_POINT ( 'NONE',  ( 106.6228877857910931, 27.24245963308690932, -63.68110863517714648 ) ) ;
#46094=CARTESIAN_POINT ( 'NONE',  ( 45.76405797021010358, 10.34101216371941945, -12.29601346399615736 ) ) ;
#46095=CARTESIAN_POINT ( 'NONE',  ( 45.04360969585140850, 9.210232288266707812, 69.22437720569834596 ) ) ;
#46097=CARTESIAN_POINT ( 'NONE',  ( -0.3308315265093308422, 6.518779160332018208, 90.59193596399374826 ) ) ;
#46099=CARTESIAN_POINT ( 'NONE',  ( -109.7790042512817905, 37.90666514836946988, -15.96121214152020151 ) ) ;
#46102=CARTESIAN_POINT ( 'NONE',  ( -171.0814041607219735, 84.88598211196834598, 57.93652428202116766 ) ) ;
#46103=EDGE_LOOP ( 'NONE', ( #14802, #16331, #10923, #36774 ) ) ;
#46106=DIRECTION ( 'NONE',  ( 0.000000000000000000, 0.000000000000000000, 1.000000000000000000 ) ) ;
#46108=CARTESIAN_POINT ( 'NONE',  ( 105.2529848321548229, 27.73895015262025510, 58.35137084276885133 ) ) ;
#46110=AXIS2_PLACEMENT_3D ( 'NONE', #64955, #6200, #49093 ) ;
#46111=CARTESIAN_POINT ( 'NONE',  ( 62.05396267233470553, 13.48332220860127251, -23.83009510918770602 ) ) ;
#46116=CARTESIAN_POINT ( 'NONE',  ( 16.27775141556967498, 7.523247835309956777, -50.51894409868579316 ) ) ;
#46117=CARTESIAN_POINT ( 'NONE',  ( -146.1201263095600211, 62.66021356509619977, 44.91613754074177933 ) ) ;
#46118=CARTESIAN_POINT ( 'NONE',  ( 212.1700216741374447, 117.1889356120871497, 35.98003273437689131 ) ) ;
#46119=FACE_BOUND ( 'NONE', #23786, .T. ) ;
#46120=EDGE_CURVE ( 'NONE', #9716, #53253, #37797, .T. ) ;
#46121=EDGE_CURVE ( 'NONE', #65685, #50735, #55428, .T. ) ;
#46123=ORIENTED_EDGE ( 'NONE', *, *, #16522, .T. ) ;
#46124=EDGE_LOOP ( 'NONE', ( #1519, #21732, #53327, #40318 ) ) ;
#46126=CARTESIAN_POINT ( 'NONE',  ( -133.4012201662767154, 52.87735233434317905, 91.74459345490905093 ) ) ;
#46128=CARTESIAN_POINT ( 'NONE',  ( 133.8566784816069060, 42.60093787723652525, -36.02331093239566684 ) ) ;
#46129=CARTESIAN_POINT ( 'NONE',  ( 9.116793664011934695, 6.378730188587224958, 87.76143697225847973 ) ) ;
#46131=CARTESIAN_POINT ( 'NONE',  ( 79.92465405224848496, 17.24122384219593584, -66.76821263654514382 ) ) ;
#46132=ORIENTED_EDGE ( 'NONE', *, *, #28778, .T. ) ;
#46137=ORIENTED_EDGE ( 'NONE', *, *, #42335, .T. ) ;
#46138=CARTESIAN_POINT ( 'NONE',  ( -85.09761763353358788, 24.87634954265997678, -65.59306203265751378 ) ) ;
#46139=DIRECTION ( 'NONE',  ( -0.000000000000000000, 1.000000000000000000, -0.000000000000000000 ) ) ;
#46141=EDGE_LOOP ( 'NONE', ( #64386, #12688 ) ) ;
#46144=CARTESIAN_POINT ( 'NONE',  ( 42.48820792780865219, 9.847387255477759282, 57.41842209376518014 ) ) ;
#46147=CARTESIAN_POINT ( 'NONE',  ( 21.73827885904429991, 6.764046335627708295, 6.097589566770120761 ) ) ;
#46149=CARTESIAN_POINT ( 'NONE',  ( -34.56779088559552804, 10.12574264174958927, 84.58167098002580531 ) ) ;
#46150=CARTESIAN_POINT ( 'NONE',  ( 180.6713229637342408, 79.61878926895391828, -78.06960825634332934 ) ) ;
#46152=CARTESIAN_POINT ( 'NONE',  ( 114.6890011751076202, 30.99337387307411262, -10.51847467832273431 ) ) ;
#46153=CARTESIAN_POINT ( 'NONE',  ( 84.97658021689287011, 19.92447159015900837, -50.64111290637077900 ) ) ;
#46154=DIRECTION ( 'NONE',  ( -0.000000000000000000, 1.000000000000000000, -0.000000000000000000 ) ) ;
#46158=CARTESIAN_POINT ( 'NONE',  ( 45.34143264614439772, 9.256465810451190990, 5.983062029440628926 ) ) ;
#46160=CARTESIAN_POINT ( 'NONE',  ( -178.9955247929450195, 95.48949252708244728, 87.33860847132339700 ) ) ;
#46163=CARTESIAN_POINT ( 'NONE',  ( 137.5001123695281819, 43.66803101819199640, -90.64561015475420902 ) ) ;
#46164=CARTESIAN_POINT ( 'NONE',  ( -31.43908319763709969, 9.591432048623756756, -89.00629854612920155 ) ) ;
#46165=CARTESIAN_POINT ( 'NONE',  ( 211.6185147280479839, 118.1878708275672381, 93.29378292525510119 ) ) ;
#46167=CARTESIAN_POINT ( 'NONE',  ( 212.0803491126036420, 118.9047894217572860, 38.07225711898713172 ) ) ;
#46169=CARTESIAN_POINT ( 'NONE',  ( -108.5289085648060308, 36.07014995015116199, 42.17405088988840589 ) ) ;
#46171=CARTESIAN_POINT ( 'NONE',  ( 9.275903038161098735, 7.385619229189522628, -12.42222294732710530 ) ) ;
#46173=CARTESIAN_POINT ( 'NONE',  ( 197.1980152960110502, 96.59350208824305639, -16.64405865593795752 ) ) ;
#46177=CARTESIAN_POINT ( 'NONE',  ( -145.9181947914995021, 62.49417193455356312, 71.65474024834820455 ) ) ;
#46179=CARTESIAN_POINT ( 'NONE',  ( -149.5074843970971301, -170.0000000000000000, -69.15738112195565179 ) ) ;
#46180=CARTESIAN_POINT ( 'NONE',  ( 37.70762885381311946, 8.195134395012285466, -35.80965490857880695 ) ) ;
#46181=CARTESIAN_POINT ( 'NONE',  ( -103.2169245450825770, 33.25885825286822950, 3.718631916029228268 ) ) ;
#46182=CARTESIAN_POINT ( 'NONE',  ( 8.337549025192453556, 7.382630697225777361, -44.00666453551739465 ) ) ;
#46184=ORIENTED_EDGE ( 'NONE', *, *, #30107, .F. ) ;
#46191=CARTESIAN_POINT ( 'NONE',  ( 8.000000000000007105, 249.8719672152120381, -95.00000000000133582 ) ) ;
#46192=CARTESIAN_POINT ( 'NONE',  ( -102.2801239173131194, -170.0000000000000000, 11.17452391595143091 ) ) ;
#46193=CARTESIAN_POINT ( 'NONE',  ( 177.7889574972182345, 75.33777460203563692, -77.32201188078130372 ) ) ;
#46195=CARTESIAN_POINT ( 'NONE',  ( 93.70675391435744928, 21.95852801827563283, -18.97173053105346341 ) ) ;
#46196=CARTESIAN_POINT ( 'NONE',  ( -29.04400972079233156, 10.22852224114065400, 71.67251108405717730 ) ) ;
#46202=ORIENTED_EDGE ( 'NONE', *, *, #29460, .T. ) ;
#46206=CARTESIAN_POINT ( 'NONE',  ( -126.3458714439411068, 46.79154809309480356, -76.75825448869765921 ) ) ;
#46208=CARTESIAN_POINT ( 'NONE',  ( -48.33725449172838751, 12.98311179783358860, -46.09223612232730716 ) ) ;
#46213=CARTESIAN_POINT ( 'NONE',  ( -189.9209858985310291, 108.0357717895543743, -92.64894649195353793 ) ) ;
#46215=ORIENTED_EDGE ( 'NONE', *, *, #29609, .F. ) ;
#46218=ORIENTED_EDGE ( 'NONE', *, *, #43090, .T. ) ;
#46220=DIRECTION ( 'NONE',  ( -0.000000000000000000, 1.000000000000000000, -0.000000000000000000 ) ) ;
#46221=CARTESIAN_POINT ( 'NONE',  ( 157.4703587214989113, 58.92748579479258808, 56.25401806271706562 ) ) ;
#46228=CARTESIAN_POINT ( 'NONE',  ( 61.33840119549016379, 13.32121602003046767, -50.53478291774639786 ) ) ;
#46230=CARTESIAN_POINT ( 'NONE',  ( -29.03891846981456837, 10.22741474064059020, -23.09507797556338105 ) ) ;
#46231=CARTESIAN_POINT ( 'NONE',  ( 141.2811136745703209, 46.09188267874202438, 9.070541501198734480 ) ) ;
#46233=CARTESIAN_POINT ( 'NONE',  ( 115.7746371641014917, 31.52600568297706118, -38.33433772466845113 ) ) ;
#46235=CARTESIAN_POINT ( 'NONE',  ( 46.89006465517228861, 9.501960077668737625, -42.63097907811025067 ) ) ;
#46236=CARTESIAN_POINT ( 'NONE',  ( -78.09558237016243254, 23.18089682183424571, 84.12268224481751133 ) ) ;
#46237=CARTESIAN_POINT ( 'NONE',  ( -118.4451797092949477, 41.78112676557538663, 92.74816161723661878 ) ) ;
#46242=CARTESIAN_POINT ( 'NONE',  ( -142.0902782307734924, 58.13494170556001706, 63.91892788494654809 ) ) ;
#46244=CARTESIAN_POINT ( 'NONE',  ( 197.2197025888162329, 96.62026035493821041, -71.33074997753084290 ) ) ;
#46245=CARTESIAN_POINT ( 'NONE',  ( 188.5662303205147055, 86.51341602961787203, -16.28199567469592424 ) ) ;
#46246=CARTESIAN_POINT ( 'NONE',  ( -118.8504142000305279, 42.02789424825279951, 67.55506623760311413 ) ) ;
#46247=CARTESIAN_POINT ( 'NONE',  ( -86.11230725916331608, 26.39026888680172434, -16.80460309939184071 ) ) ;
#46249=CARTESIAN_POINT ( 'NONE',  ( -154.7934364910360614, 68.79594655117534785, -36.98658425784656600 ) ) ;
#46250=ORIENTED_EDGE ( 'NONE', *, *, #24669, .T. ) ;
#46255=CARTESIAN_POINT ( 'NONE',  ( 103.0026233023292832, 25.67408295205786928, 61.93245107129636295 ) ) ;
#46256=CARTESIAN_POINT ( 'NONE',  ( 164.8407099662994995, 63.61629583487393802, 62.33837009251364947 ) ) ;
#46262=CARTESIAN_POINT ( 'NONE',  ( 164.4728833318992258, 63.30716077995682411, -67.76901369371475425 ) ) ;
#46268=CARTESIAN_POINT ( 'NONE',  ( -153.1031717208031750, 68.63449618039565792, -22.05411808047816891 ) ) ;
#46269=CARTESIAN_POINT ( 'NONE',  ( -84.23431294393863311, 24.52078568147205573, 59.71377569600485913 ) ) ;
#46270=CARTESIAN_POINT ( 'NONE',  ( 64.94794467308301478, 13.12874966082104855, -35.95744817871243981 ) ) ;
#46273=CARTESIAN_POINT ( 'NONE',  ( -56.73868929054669508, 16.18382781951277494, 45.12942635042991668 ) ) ;
#46275=CARTESIAN_POINT ( 'NONE',  ( 34.45500533947588195, 7.817363290423888778, 69.91678222496804551 ) ) ;
#46276=CARTESIAN_POINT ( 'NONE',  ( 8.336882341125877005, 6.376438415325264231, -17.15788629728112724 ) ) ;
#46281=CARTESIAN_POINT ( 'NONE',  ( -122.3745688183165754, 44.21964839958060622, 17.91535119075751581 ) ) ;
#46282=CARTESIAN_POINT ( 'NONE',  ( 64.94794467308304320, 13.12874966082103079, -62.80199876917609458 ) ) ;
#46284=CARTESIAN_POINT ( 'NONE',  ( 22.51849650178395024, 7.817407610814550267, -12.85559206638460950 ) ) ;
#46285=CARTESIAN_POINT ( 'NONE',  ( 197.3059626281005592, 96.72682679064189415, 64.86311202157818911 ) ) ;
#46289=ADVANCED_FACE ( 'NONE', ( #63409 ), #68670, .F. ) ;
#46293=CARTESIAN_POINT ( 'NONE',  ( 187.6511924654682844, 87.00187850361888309, -47.35777523915407983 ) ) ;
#46301=EDGE_LOOP ( 'NONE', ( #11535, #15944 ) ) ;
#46302=CARTESIAN_POINT ( 'NONE',  ( -60.98168946575808747, 17.40090852531920262, 15.59240914876137651 ) ) ;
#46308=CARTESIAN_POINT ( 'NONE',  ( -101.8191498210054959, 32.54686850610963234, 30.51907450641511232 ) ) ;
#46309=CARTESIAN_POINT ( 'NONE',  ( -78.66644367742111399, -170.0000000000000000, -96.30455181264525777 ) ) ;
#46313=CARTESIAN_POINT ( 'NONE',  ( 55.76066037845577483, 11.10616952318092210, 35.34777878534185902 ) ) ;
#46316=CARTESIAN_POINT ( 'NONE',  ( 179.4074606910091916, 78.34362448405029511, 44.16935534552229115 ) ) ;
#46318=CARTESIAN_POINT ( 'NONE',  ( 21.42484406671928454, 6.746536496442161912, -74.81728185975761392 ) ) ;
#46319=CARTESIAN_POINT ( 'NONE',  ( -128.9843070188473177, 49.78011598923035308, 58.11564453485428317 ) ) ;
#46321=CARTESIAN_POINT ( 'NONE',  ( -100.8612319006215472, 33.19127816346582449, 84.33756607052741572 ) ) ;
#46325=CARTESIAN_POINT ( 'NONE',  ( 211.8382652195006415, 118.5282575235989668, -68.35397587044393219 ) ) ;
#46326=CARTESIAN_POINT ( 'NONE',  ( 134.3182571105339207, 42.88121222759020412, 44.51034083899536142 ) ) ;
#46329=CARTESIAN_POINT ( 'NONE',  ( 66.73467315386237431, 14.60276727483218018, -63.53416605551942808 ) ) ;
#46332=CARTESIAN_POINT ( 'NONE',  ( 187.0823097343935331, 84.88801889414973800, 94.99999999999866418 ) ) ;
#46333=CARTESIAN_POINT ( 'NONE',  ( -170.2801941679960009, 84.02053682015869640, -49.16597572273842331 ) ) ;
#46336=CARTESIAN_POINT ( 'NONE',  ( -52.95640735647533148, 15.16886689662459275, -89.20118622082404158 ) ) ;
#46338=CARTESIAN_POINT ( 'NONE',  ( 15.78827728214693416, -170.0000000000000000, -69.86349468914949057 ) ) ;
#46339=CARTESIAN_POINT ( 'NONE',  ( -149.5074843970971017, 64.17983161892347255, 45.72082123989907387 ) ) ;
#46340=CARTESIAN_POINT ( 'NONE',  ( -125.8938041572051105, 47.69968343338781835, 45.61994787315711619 ) ) ;
#46341=CARTESIAN_POINT ( 'NONE',  ( -165.6212796729685124, 79.15047440262054579, -69.36342526124160202 ) ) ;
#46343=CARTESIAN_POINT ( 'NONE',  ( -106.4728934171453858, 36.10295170132725673, 31.79594541829927579 ) ) ;
#46345=EDGE_CURVE ( 'NONE', #45819, #50285, #2558, .T. ) ;
#46346=CARTESIAN_POINT ( 'NONE',  ( -38.84150381976579069, 10.92416363971238802, 9.640924607406274660 ) ) ;
#46349=CARTESIAN_POINT ( 'NONE',  ( -82.52059008511432125, 23.82719274235528317, -89.86705382797902075 ) ) ;
#46354=CARTESIAN_POINT ( 'NONE',  ( -8.810383862755514883, 7.965311326754783927, -35.46662548705337059 ) ) ;
#46355=CARTESIAN_POINT ( 'NONE',  ( -37.52119286077854099, 11.69341290629620289, -20.36792989721667269 ) ) ;
#46356=ORIENTED_EDGE ( 'NONE', *, *, #46932, .T. ) ;
#46357=CARTESIAN_POINT ( 'NONE',  ( -123.8554280348324852, 46.36425916468965625, -88.88211011207803836 ) ) ;
#46360=CARTESIAN_POINT ( 'NONE',  ( -56.02289203441036847, 15.98631679403369255, 72.11475544954369354 ) ) ;
#46361=CARTESIAN_POINT ( 'NONE',  ( -24.70911172866235006, 8.583078995053019966, 7.525281538729513997 ) ) ;
#46365=CARTESIAN_POINT ( 'NONE',  ( -60.43659296547055249, 16.19120964214080161, -91.16608923734209213 ) ) ;
#46366=CARTESIAN_POINT ( 'NONE',  ( -38.26732153931116898, 10.81230693396213915, 34.60420372569744529 ) ) ;
#46368=EDGE_CURVE ( 'NONE', #47148, #1332, #37343, .T. ) ;
#46369=CARTESIAN_POINT ( 'NONE',  ( 153.2208437558771834, 55.67531116261156399, -37.42660832897070122 ) ) ;
#46371=EDGE_CURVE ( 'NONE', #28945, #35894, #63680, .T. ) ;
#46376=CARTESIAN_POINT ( 'NONE',  ( -156.9262190792700267, 72.10659547035874084, 66.20392794627127842 ) ) ;
#46377=CARTESIAN_POINT ( 'NONE',  ( -124.3331814159187587, 45.47486189329070783, 30.78061265518531187 ) ) ;
#46379=ORIENTED_EDGE ( 'NONE', *, *, #26459, .F. ) ;
#46380=CARTESIAN_POINT ( 'NONE',  ( -180.4651598106647725, 97.28730001475653921, -67.50490632099327115 ) ) ;
#46381=CARTESIAN_POINT ( 'NONE',  ( 126.5079999146319381, 38.31335175111690461, 89.15821877620250291 ) ) ;
#46382=CARTESIAN_POINT ( 'NONE',  ( 117.3110050642448243, 32.29133253383016466, 34.55243254091307392 ) ) ;
#46384=CARTESIAN_POINT ( 'NONE',  ( -124.3250225421925563, 45.46958056770279910, -61.92067255773788048 ) ) ;
#46386=ORIENTED_EDGE ( 'NONE', *, *, #24217, .F. ) ;
#46389=CARTESIAN_POINT ( 'NONE',  ( 188.4918087359956758, 87.93403732562659059, 35.59746311784228112 ) ) ;
#46390=CARTESIAN_POINT ( 'NONE',  ( 185.7741388806743998, 83.47871114541692350, -91.54853474465144814 ) ) ;
#46391=CARTESIAN_POINT ( 'NONE',  ( -78.66644367742111399, 22.32174330031316956, -8.270900041254197532 ) ) ;
#46395=CARTESIAN_POINT ( 'NONE',  ( 160.9099843287285410, 61.67000084894971934, -23.46024577593901483 ) ) ;
#46397=CARTESIAN_POINT ( 'NONE',  ( 68.94948716683069279, 15.16699441119056679, 59.54438869000860279 ) ) ;
#46398=CARTESIAN_POINT ( 'NONE',  ( 127.7121523762017858, 37.83617439506281244, 94.99999999999866418 ) ) ;
#46403=CARTESIAN_POINT ( 'NONE',  ( -142.0902782307735492, 58.13494170556001706, -70.30382506737186077 ) ) ;
#46405=CARTESIAN_POINT ( 'NONE',  ( 162.1014732644455307, 61.34312237409766055, -37.70552761938252928 ) ) ;
#46410=CARTESIAN_POINT ( 'NONE',  ( -129.3963145237380843, 48.84337839101545597, 44.75594546263260298 ) ) ;
#46411=CARTESIAN_POINT ( 'NONE',  ( 151.7945360828342700, 54.61722255954529004, -92.39293117455194704 ) ) ;
#46412=CARTESIAN_POINT ( 'NONE',  ( 82.95856197793165165, 19.25847567427441831, -23.03551787981482235 ) ) ;
#46413=CARTESIAN_POINT ( 'NONE',  ( -167.1540252468941787, 80.72321878831098729, 33.77097442923315640 ) ) ;
#46415=CARTESIAN_POINT ( 'NONE',  ( 151.7819978880463339, 53.35998893001570309, 58.85968254170387581 ) ) ;
#46419=DIRECTION ( 'NONE',  ( 0.000000000000000000, 0.000000000000000000, 1.000000000000000000 ) ) ;
#46420=VERTEX_POINT ( 'NONE', #11651 ) ;
#46421=AXIS2_PLACEMENT_3D ( 'NONE', #65302, #45230, #34353 ) ;
#46422=CARTESIAN_POINT ( 'NONE',  ( 157.4703587214989113, 58.92748579479260229, -9.279633708673953763 ) ) ;
#46423=CARTESIAN_POINT ( 'NONE',  ( 212.1734186221015648, 119.0499290057855291, -16.28920841871465441 ) ) ;
#46424=CARTESIAN_POINT ( 'NONE',  ( 103.8325688302027459, 27.12251147381403271, 33.20992942965430927 ) ) ;
#46425=CARTESIAN_POINT ( 'NONE',  ( -2.172839205444465183, 7.595638683704371452, 32.66141357948582424 ) ) ;
#46426=CARTESIAN_POINT ( 'NONE',  ( 64.33924340318904456, 12.98343211571920008, 83.61250075476556276 ) ) ;
#46427=CARTESIAN_POINT ( 'NONE',  ( 186.2680729609085120, 85.48839327635670315, 4.523648567817806665 ) ) ;
#46428=CARTESIAN_POINT ( 'NONE',  ( 212.1931396682533659, 117.2245435827729665, -43.51221325195484724 ) ) ;
#46429=CARTESIAN_POINT ( 'NONE',  ( 174.9053416555736646, 72.57849647436442808, 5.682350544106838264 ) ) ;
#46430=CARTESIAN_POINT ( 'NONE',  ( -62.48965350618345838, 16.80247907725182088, 11.97533722146177304 ) ) ;
#46436=CARTESIAN_POINT ( 'NONE',  ( 103.4696172145934980, 25.87254488218942328, -67.03655338143190079 ) ) ;
#46438=CARTESIAN_POINT ( 'NONE',  ( -75.43953471071002070, 21.11829282998125734, 4.286557885301053084 ) ) ;
#46439=CARTESIAN_POINT ( 'NONE',  ( -31.86754543663846562, 9.661758835099860221, -89.00629854612918734 ) ) ;
#46440=CARTESIAN_POINT ( 'NONE',  ( -13.97284672409966433, 7.369429924072608884, 86.95875599126263467 ) ) ;
#46443=CARTESIAN_POINT ( 'NONE',  ( -71.41745561414265353, 19.69148172991712542, 66.75175318804630820 ) ) ;
#46444=CARTESIAN_POINT ( 'NONE',  ( -166.9982296371935035, 80.56207291422410322, 60.82688077875437216 ) ) ;
#46445=ORIENTED_EDGE ( 'NONE', *, *, #56638, .T. ) ;
#46446=ORIENTED_EDGE ( 'NONE', *, *, #64944, .T. ) ;
#46450=CARTESIAN_POINT ( 'NONE',  ( 175.5406524085946103, 73.17873692326779178, -21.95791395497509413 ) ) ;
#46451=CARTESIAN_POINT ( 'NONE',  ( -168.0003605155415300, 83.06333427281273885, 59.68102058965342849 ) ) ;
#46453=ADVANCED_FACE ( 'NONE', ( #7445 ), #29239, .F. ) ;
#46455=AXIS2_PLACEMENT_3D ( 'NONE', #28445, #22823, #1719 ) ;
#46457=CARTESIAN_POINT ( 'NONE',  ( 110.2429982417149432, 29.99119854320846201, -35.92243756565368784 ) ) ;
#46459=CARTESIAN_POINT ( 'NONE',  ( 210.4897348480409391, 114.6382060222044856, 5.092056172177173323 ) ) ;
#46460=CARTESIAN_POINT ( 'NONE',  ( 9.837735240994035735, 7.389327806910502616, 59.78739175200453104 ) ) ;
#46463=DIRECTION ( 'NONE',  ( 1.000000000000000000, 0.000000000000000000, 0.000000000000000000 ) ) ;
#46470=CARTESIAN_POINT ( 'NONE',  ( 32.66883187925818532, 8.640402022338115273, -73.30456228053577661 ) ) ;
#46471=DIRECTION ( 'NONE',  ( -0.000000000000000000, 1.000000000000000000, -0.000000000000000000 ) ) ;
#46472=CARTESIAN_POINT ( 'NONE',  ( 19.82795039379812607, 6.663502596869125050, 84.87619840072350996 ) ) ;
#46474=CARTESIAN_POINT ( 'NONE',  ( 80.30232379693109124, 17.35837133860834314, -74.20099956211727488 ) ) ;
#46478=B_SPLINE_CURVE_WITH_KNOTS ( 'NONE', 3,
 ( #54250, #6072, #48976, #44414, #65897, #22268, #60597, #16974, #27893, #49328, #12417, #55312, #1159, #65536, #17329, #38804, #62689, #40525, #29284, #61974, #40873, #45106, #14147, #13794, #62328, #8534, #29978, #14490, #67616, #19416, #35946, #35608, #35252, #66592, #56711, #13118, #41227, #39835, #52119, #7836 ),
 .UNSPECIFIED., .F., .F.,
 ( 4, 2, 2, 2, 2, 2, 2, 2, 2, 2, 2, 2, 2, 2, 2, 2, 2, 2, 2, 4 ),
 ( 0.02472759712254455136, 0.02626001169882804381, 0.02779242627511153627, 0.02932484085139502872, 0.03009104813953675933, 0.03085725542767848995, 0.03238967000396195117, 0.03315587729210368872, 0.03392208458024543322, 0.03545449915652893608, 0.03698691373281243200, 0.03851932830909592792, 0.04005174288537943078, 0.04158415746166292670, 0.04311657203794642262, 0.04464898661422991855, 0.04541519390237166998, 0.04618140119051342141, 0.04771381576679691733, 0.04924623034308041325 ),
 .UNSPECIFIED. ) ;
#46479=CARTESIAN_POINT ( 'NONE',  ( 198.8752826725511227, 100.3130050945023584, -48.56026461867841704 ) ) ;
#46481=CARTESIAN_POINT ( 'NONE',  ( -82.93267503967653909, 23.99263498936122474, 17.24672781033775948 ) ) ;
#46488=CARTESIAN_POINT ( 'NONE',  ( 22.80839748737788497, 6.826915557457463812, 8.019082751123264075 ) ) ;
#46490=CARTESIAN_POINT ( 'NONE',  ( -25.17576297385273065, 8.646815144065621794, 87.26720278706356737 ) ) ;
#46491=CARTESIAN_POINT ( 'NONE',  ( -53.13788504024112314, 15.21566150156364294, 3.705312443272094303 ) ) ;
#46494=CARTESIAN_POINT ( 'NONE',  ( 104.7147873368644753, 26.40702926859708910, -38.33007957820842648 ) ) ;
#46495=CARTESIAN_POINT ( 'NONE',  ( 84.72546926745367557, 19.84015517905185888, -36.05123878307442453 ) ) ;
#46496=CARTESIAN_POINT ( 'NONE',  ( -165.6754884515988522, 80.64428675972324356, -95.00000000000133582 ) ) ;
#46502=CARTESIAN_POINT ( 'NONE',  ( -85.64924756730684408, 26.19583280090852639, -72.20824660844574794 ) ) ;
#46503=CARTESIAN_POINT ( 'NONE',  ( 174.1422537179814753, 73.24254491731250027, 7.110486902026410760 ) ) ;
#46506=CARTESIAN_POINT ( 'NONE',  ( 126.3580543567275356, 37.07735301062817967, 10.46969542368406536 ) ) ;
#46508=CARTESIAN_POINT ( 'NONE',  ( -156.9406434201984268, 70.74968524571472983, 12.52616388493933464 ) ) ;
#46512=CARTESIAN_POINT ( 'NONE',  ( 210.9608386442062624, 117.1762372255315938, 40.84185146199625649 ) ) ;
#46513=CARTESIAN_POINT ( 'NONE',  ( -84.21836162213170951, 25.60181819557222838, 59.69698668375344397 ) ) ;
#46514=DIRECTION ( 'NONE',  ( -0.000000000000000000, 1.000000000000000000, -0.000000000000000000 ) ) ;
#46519=CARTESIAN_POINT ( 'NONE',  ( 9.837735240994035735, 7.389327806910502616, -20.74626001938653630 ) ) ;
#46521=CARTESIAN_POINT ( 'NONE',  ( 45.80999061969644970, 10.34829880103435507, 94.99999999999866418 ) ) ;
#46525=CARTESIAN_POINT ( 'NONE',  ( -142.8556048422595381, 60.01994222009837898, 68.54020186033872619 ) ) ;
#46527=CARTESIAN_POINT ( 'NONE',  ( -29.03891846981456126, 10.22741474064058487, 3.749472614900290601 ) ) ;
#46530=CARTESIAN_POINT ( 'NONE',  ( -7.825402957745087207, -170.0000000000000000, -96.60717191287118055 ) ) ;
#46532=VERTEX_POINT ( 'NONE', #60891 ) ;
#46536=CARTESIAN_POINT ( 'NONE',  ( -30.46060138092288838, 9.432375387772216513, -62.20961696371778515 ) ) ;
#46539=CARTESIAN_POINT ( 'NONE',  ( 11.21653854975268949, 6.397128675385708618, 16.63585048340505423 ) ) ;
#46542=CARTESIAN_POINT ( 'NONE',  ( 207.4610690199662315, 111.9701171077052209, 16.84735845215860905 ) ) ;
#46544=CARTESIAN_POINT ( 'NONE',  ( -179.6470915626257465, 94.69856161161348496, -45.91846509321587178 ) ) ;
#46545=CARTESIAN_POINT ( 'NONE',  ( 89.88695630745283438, 20.55793566325394650, -9.704490825940514043 ) ) ;
#46546=CARTESIAN_POINT ( 'NONE',  ( -26.50207385662994497, 9.849226639603646305, 58.89342097685724298 ) ) ;
#46547=CYLINDRICAL_SURFACE ( 'NONE', #62137, 7.500000000000020428 ) ;
#46548=CARTESIAN_POINT ( 'NONE',  ( -50.51700111023803430, 13.51182830536854595, 70.65495365061850919 ) ) ;
#46550=CARTESIAN_POINT ( 'NONE',  ( -0.7215816834507520205, 6.532459459468099361, 62.04215831576383522 ) ) ;
#46553=CARTESIAN_POINT ( 'NONE',  ( 151.1827182658834090, 54.16800928478853194, 59.63366074271394979 ) ) ;
#46554=CARTESIAN_POINT ( 'NONE',  ( -108.0902552660050446, 36.97681740369920078, -74.12781022651168428 ) ) ;
#46555=CARTESIAN_POINT ( 'NONE',  ( -48.57297291660696459, 13.03920345822338689, -46.52532158187338496 ) ) ;
#46560=VECTOR ( 'NONE', #26978, 1000.000000000000000 ) ;
#46562=CARTESIAN_POINT ( 'NONE',  ( -190.0608188262619365, 108.2310236786209146, -92.36485475830178871 ) ) ;
#46567=CARTESIAN_POINT ( 'NONE',  ( 181.0840389613909736, 78.60582251573005408, -51.22505766587963905 ) ) ;
#46569=CARTESIAN_POINT ( 'NONE',  ( 8.000000000000007105, 249.8719672152120381, -95.00000000000133582 ) ) ;
#46572=CARTESIAN_POINT ( 'NONE',  ( -55.54058841405665703, 14.81234591756537888, -62.06087458892353936 ) ) ;
#46574=CARTESIAN_POINT ( 'NONE',  ( 56.94505604581134861, 12.37336791557970095, -47.63195170334665818 ) ) ;
#46575=CARTESIAN_POINT ( 'NONE',  ( -85.35172689181703731, 26.07142112926218758, 34.48212782639603802 ) ) ;
#46576=CARTESIAN_POINT ( 'NONE',  ( -25.07735481787161191, 9.648965052008778187, -19.95240735271818622 ) ) ;
#46577=CARTESIAN_POINT ( 'NONE',  ( 133.8566784816069628, 41.42467568809806977, 17.66579024853170310 ) ) ;
#46580=CARTESIAN_POINT ( 'NONE',  ( 8.670103207226933506, 6.377073801252349128, 61.94615088279628878 ) ) ;
#46581=CARTESIAN_POINT ( 'NONE',  ( 200.4590013143046576, 102.3556155835303088, 30.50310333978841726 ) ) ;
#46582=CARTESIAN_POINT ( 'NONE',  ( -74.59410384915268821, 21.88130278302777754, 85.27819964176909195 ) ) ;
#46589=CARTESIAN_POINT ( 'NONE',  ( -145.3109762780891288, 60.69959559383374170, 71.29862809856072658 ) ) ;
#46594=CARTESIAN_POINT ( 'NONE',  ( -121.1775535805057160, 43.46577565517554831, 70.81645009186183870 ) ) ;
#46596=CARTESIAN_POINT ( 'NONE',  ( 23.09119322872580682, 7.852465917941087170, -95.00000000000133582 ) ) ;
#46598=EDGE_CURVE ( 'NONE', #44052, #41887, #67969, .T. ) ;
#46602=CARTESIAN_POINT ( 'NONE',  ( -109.0291978193666722, 37.49173305805087608, 7.893610283594471255 ) ) ;
#46604=EDGE_CURVE ( 'NONE', #6351, #28945, #30282, .T. ) ;
#46605=CARTESIAN_POINT ( 'NONE',  ( 105.8203563788590742, 26.88901185006200123, 70.01787404090897837 ) ) ;
#46606=CARTESIAN_POINT ( 'NONE',  ( 111.8863762173178316, 29.64954938250774674, 83.47565785988531673 ) ) ;
#46607=CARTESIAN_POINT ( 'NONE',  ( -189.2346268516247108, 107.0830361517164846, 65.47910114476307797 ) ) ;
#46610=CARTESIAN_POINT ( 'NONE',  ( 181.5072453427590915, 79.03352099595188918, -51.22505766587964615 ) ) ;
#46611=CARTESIAN_POINT ( 'NONE',  ( 110.2429982417149574, -170.0000000000000000, -16.57788697519001175 ) ) ;
#46613=CARTESIAN_POINT ( 'NONE',  ( -142.3799050480288031, 59.64294364584055330, 89.55052947415697417 ) ) ;
#46615=EDGE_LOOP ( 'NONE', ( #36043, #28915 ) ) ;
#46621=EDGE_CURVE ( 'NONE', #66651, #62757, #63324, .T. ) ;
#46622=CARTESIAN_POINT ( 'NONE',  ( 65.40032188136233060, 13.23841673691966925, -50.33562451376164404 ) ) ;
#46624=CARTESIAN_POINT ( 'NONE',  ( -62.50103539982530521, 17.85731685071834107, 36.80643099207888724 ) ) ;
#46625=CARTESIAN_POINT ( 'NONE',  ( -38.93938005333175312, 11.96888249046461361, -69.42206000664089061 ) ) ;
#46626=CARTESIAN_POINT ( 'NONE',  ( 34.83825437341839404, 7.859462995505743343, 58.28670175242805129 ) ) ;
#46627=CARTESIAN_POINT ( 'NONE',  ( 45.76539630260660374, 9.322640236743859887, 87.11983195816242187 ) ) ;
#46632=CARTESIAN_POINT ( 'NONE',  ( 188.2950202724320832, 86.21411212788221690, 61.57030577803965343 ) ) ;
#46633=CARTESIAN_POINT ( 'NONE',  ( -124.3250225421926132, 45.46958056770283463, 18.61297921365314778 ) ) ;
#46634=CARTESIAN_POINT ( 'NONE',  ( 68.63487067129267416, 14.04635751989140147, -65.07391997778475456 ) ) ;
#46635=CARTESIAN_POINT ( 'NONE',  ( 15.78827728214693416, 6.500811158483284835, 56.85925826316891829 ) ) ;
#46637=CARTESIAN_POINT ( 'NONE',  ( 204.6977192012829789, 106.3443248447423599, 56.05227132923312183 ) ) ;
#46639=CARTESIAN_POINT ( 'NONE',  ( 187.9007786055418592, 85.78077355327279463, 13.10349074316396489 ) ) ;
#46641=CARTESIAN_POINT ( 'NONE',  ( 130.7457207912711112, 40.74300766298684806, -50.36327218344248280 ) ) ;
#46642=CARTESIAN_POINT ( 'NONE',  ( -127.6861178856153742, 47.68458428355324941, -35.11711282288931812 ) ) ;
#46643=B_SPLINE_CURVE_WITH_KNOTS ( 'NONE', 3,
 ( #19449, #31400, #9944, #46180, #14184, #9250, #52831, #68004, #47213, #52157, #19809, #47548, #20148, #67653, #62720, #35984, #46883, #63411, #40913, #58128, #4653, #4324, #56748, #19105, #40559, #41600, #3287, #57439, #57783, #9598, #41947, #35644, #41265, #25787, #3620, #20483, #24745, #62011, #62369, #25444, #30707, #13829, #8567, #57094, #8911 ),
 .UNSPECIFIED., .F., .F.,
 ( 4, 2, 2, 2, 2, 2, 2, 2, 1, 2, 2, 2, 2, 2, 2, 2, 2, 2, 2, 2, 2, 2, 4 ),
 ( 0.000000000000000000, 0.001470449819620675991, 0.002205674729431024612, 0.002940899639241372800, 0.004411349458862050092, 0.005881799278482727385, 0.007352249098103403810, 0.008087474007913734650, 0.008822698917724065490, 0.009557923827534394595, 0.01029314873734472544, 0.01176359855696536630, 0.01249882346677567459, 0.01323404837658598461, 0.01470449819620660813, 0.01543972310601693203, 0.01617494801582725766, 0.01764539783544792628, 0.01911584765506859490, 0.01985107256487891880, 0.02058629747468924617, 0.02205674729430990091, 0.02352719711393055912 ),
 .UNSPECIFIED. ) ;
#46644=CARTESIAN_POINT ( 'NONE',  ( -104.5740066103012822, 35.09687312794777370, -49.65903324600630953 ) ) ;
#46645=CARTESIAN_POINT ( 'NONE',  ( 184.5867277229703518, 83.68414666546578928, -37.08944934118979830 ) ) ;
#46648=CARTESIAN_POINT ( 'NONE',  ( -147.7845268487069461, 62.73119438705056439, -8.155966956317975303 ) ) ;
#46652=CARTESIAN_POINT ( 'NONE',  ( 163.4829520545006289, 63.79049927423832855, 86.10267534221468111 ) ) ;
#46654=CARTESIAN_POINT ( 'NONE',  ( -62.55320287144887459, 17.87319849854529608, 11.21034754316474746 ) ) ;
#46655=CARTESIAN_POINT ( 'NONE',  ( 129.1381264900934411, 38.64720302602604107, 42.86026151076471535 ) ) ;
#46656=VECTOR ( 'NONE', #3616, 1000.000000000000000 ) ;
#46657=CARTESIAN_POINT ( 'NONE',  ( -152.9008427825210674, 68.45483453645054794, 31.52859718944691636 ) ) ;
#46658=LINE ( 'NONE', #8699, #21387 ) ;
#46660=AXIS2_PLACEMENT_3D ( 'NONE', #173, #43769, #11771 ) ;
#46661=CARTESIAN_POINT ( 'NONE',  ( -102.2801239173131194, -170.0000000000000000, -96.20367844590329298 ) ) ;
#46663=EDGE_LOOP ( 'NONE', ( #15099, #57461, #5308, #4833 ) ) ;
#46668=CARTESIAN_POINT ( 'NONE',  ( -171.0950923142954139, 86.38958441093225815, 4.243329981061625844 ) ) ;
#46670=APPLICATION_CONTEXT ( 'automotive_design' ) ;
#46671=CARTESIAN_POINT ( 'NONE',  ( -33.12934624031570507, 10.89552623243536900, -89.18697688497687182 ) ) ;
#46672=CARTESIAN_POINT ( 'NONE',  ( -133.1640943168119122, 52.70734926280008636, 66.82601452699702804 ) ) ;
#46674=CARTESIAN_POINT ( 'NONE',  ( -109.7346721907204028, 37.88203613721440632, 90.81995025446376246 ) ) ;
#46677=CARTESIAN_POINT ( 'NONE',  ( -56.96214175905168275, 15.20165595797839408, -8.614853995199030834 ) ) ;
#46679=CARTESIAN_POINT ( 'NONE',  ( -129.3970594949620079, 50.06339481638098476, -75.90617434883772319 ) ) ;
#46680=CARTESIAN_POINT ( 'NONE',  ( 117.3145357257065342, 33.41973663092564095, 39.66135912721455981 ) ) ;
#46682=CARTESIAN_POINT ( 'NONE',  ( 65.39792658623289867, 14.27332852928128126, -62.94950063402156104 ) ) ;
#46684=ORIENTED_EDGE ( 'NONE', *, *, #38763, .F. ) ;
#46685=EDGE_CURVE ( 'NONE', #44375, #63280, #10881, .T. ) ;
#46689=LINE ( 'NONE', #25604, #65902 ) ;
#46690=CARTESIAN_POINT ( 'NONE',  ( -47.68562151781910785, 13.86286849776707797, -95.00000000000133582 ) ) ;
#46694=CARTESIAN_POINT ( 'NONE',  ( 211.0967808702090736, 115.5516932918876876, 59.63059121463253121 ) ) ;
#46696=CARTESIAN_POINT ( 'NONE',  ( -108.9444157621018405, 37.44493815491210853, 41.49818020471239777 ) ) ;
#46699=CARTESIAN_POINT ( 'NONE',  ( -180.3451190839052458, 95.54664796532459548, -93.86486230744075954 ) ) ;
#46700=CARTESIAN_POINT ( 'NONE',  ( 84.72546926745364715, 19.84015517905186243, 71.32696357878030824 ) ) ;
#46705=CARTESIAN_POINT ( 'NONE',  ( 37.46876540261052924, 9.179568636624020783, 3.318579510039644909 ) ) ;
#46708=CARTESIAN_POINT ( 'NONE',  ( 32.90953848114694580, 7.653665824624198422, 6.806373642810018332 ) ) ;
#46709=CARTESIAN_POINT ( 'NONE',  ( -13.29455179262033404, 8.319166883236668752, -48.05598062864418551 ) ) ;
#46710=CARTESIAN_POINT ( 'NONE',  ( -33.83721310978700814, 11.01869210665939036, -23.08310314977254052 ) ) ;
#46714=CARTESIAN_POINT ( 'NONE',  ( -125.8938041572051105, 47.69968343338781125, -88.60280507916129977 ) ) ;
#46716=CARTESIAN_POINT ( 'NONE',  ( -61.39252081892701796, 16.47343302442957835, 33.80259966407439265 ) ) ;
#46717=CARTESIAN_POINT ( 'NONE',  ( 11.82929895397812992, 7.412564870773605818, -76.23824787671220804 ) ) ;
#46718=CARTESIAN_POINT ( 'NONE',  ( -24.93568128341082968, 8.613819379861695325, 14.63976890511303885 ) ) ;
#46721=CARTESIAN_POINT ( 'NONE',  ( -14.76369756425704161, 7.442560416198670481, -66.88354962501738044 ) ) ;
#46722=CARTESIAN_POINT ( 'NONE',  ( -94.85061234775061223, 29.16417548023185091, -16.72803334679694487 ) ) ;
#46723=CARTESIAN_POINT ( 'NONE',  ( 92.91022130985207639, 22.73448145304546131, 94.99999999999866418 ) ) ;
#46725=EDGE_LOOP ( 'NONE', ( #64874, #23040, #32352, #64304 ) ) ;
#46728=CARTESIAN_POINT ( 'NONE',  ( 174.6242782760049863, 73.69713439533575183, -13.06059959078580412 ) ) ;
#46729=CARTESIAN_POINT ( 'NONE',  ( -118.8504142000305421, 42.02789424825277109, 40.71051564713940962 ) ) ;
#46732=CARTESIAN_POINT ( 'NONE',  ( -178.2448732545370831, 94.58403736950704399, -63.55990931418686785 ) ) ;
#46733=CARTESIAN_POINT ( 'NONE',  ( 127.3286037854883830, 38.77506637992906491, 94.40897935295708976 ) ) ;
#46734=CARTESIAN_POINT ( 'NONE',  ( 201.4634861300068565, 103.6729577544787162, -90.70809642864092837 ) ) ;
#46736=CARTESIAN_POINT ( 'NONE',  ( -118.4063383664800142, 41.75753822095642676, -68.74786715921418079 ) ) ;
#46737=ORIENTED_EDGE ( 'NONE', *, *, #62259, .F. ) ;
#46738=DIRECTION ( 'NONE',  ( -0.000000000000000000, 1.000000000000000000, -0.000000000000000000 ) ) ;
#46739=CARTESIAN_POINT ( 'NONE',  ( 117.4830770399667870, 32.37795270233553424, -68.24308158718707773 ) ) ;
#46740=CARTESIAN_POINT ( 'NONE',  ( 186.2680729609085120, 85.48839327635674579, 31.36819915828147742 ) ) ;
#46741=CARTESIAN_POINT ( 'NONE',  ( 187.5166849924263204, 85.36068406478833026, -93.55154100713149035 ) ) ;
#46743=VERTEX_POINT ( 'NONE', #47819 ) ;
#46744=ADVANCED_FACE ( 'NONE', ( #20750 ), #5595, .F. ) ;
#46745=CARTESIAN_POINT ( 'NONE',  ( 175.5498284945444709, 74.57669191966282085, 58.56542896661724029 ) ) ;
#46747=EDGE_CURVE ( 'NONE', #48407, #28889, #7556, .T. ) ;
#46750=CARTESIAN_POINT ( 'NONE',  ( 141.0679329045600809, 45.95256892154834816, 92.79094832732447173 ) ) ;
#46752=CARTESIAN_POINT ( 'NONE',  ( 157.4703587214989113, 58.92748579479258808, 2.564916881789689462 ) ) ;
#46753=ORIENTED_EDGE ( 'NONE', *, *, #46345, .T. ) ;
#46754=CARTESIAN_POINT ( 'NONE',  ( -179.0654441437004891, 93.99779465816536117, 33.74156010598665745 ) ) ;
#46756=CARTESIAN_POINT ( 'NONE',  ( 115.0606351894211485, 32.29586232625066344, -49.19153966712070059 ) ) ;
#46759=ORIENTED_EDGE ( 'NONE', *, *, #25989, .F. ) ;
#46762=VECTOR ( 'NONE', #46867, 1000.000000000000000 ) ;
#46764=CARTESIAN_POINT ( 'NONE',  ( -132.8123438040339863, 51.22132183644641401, 41.02731276053570753 ) ) ;
#46768=CARTESIAN_POINT ( 'NONE',  ( -169.1041038606267080, 82.76530082651281361, 31.97253426586447844 ) ) ;
#46769=CARTESIAN_POINT ( 'NONE',  ( 150.4544126017351005, 52.39556706174411715, 61.08955027113243119 ) ) ;
#46770=LINE ( 'NONE', #14423, #2395 ) ;
#46772=CARTESIAN_POINT ( 'NONE',  ( -102.2801239173131052, 33.91021738430207222, 72.36362509687883460 ) ) ;
#46774=ORIENTED_EDGE ( 'NONE', *, *, #20668, .T. ) ;
#46775=ADVANCED_FACE ( 'NONE', ( #64342 ), #4915, .T. ) ;
#46776=CARTESIAN_POINT ( 'NONE',  ( 151.8005253678161921, 54.62151558044535449, -21.71570063336847412 ) ) ;
#46777=CARTESIAN_POINT ( 'NONE',  ( -51.16680845348332696, 13.67385610796032402, 85.08383212419218466 ) ) ;
#46778=CARTESIAN_POINT ( 'NONE',  ( 105.8229724512850964, 27.98935528750252288, 31.04713432260220429 ) ) ;
#46780=CARTESIAN_POINT ( 'NONE',  ( 55.74003717006368674, 11.10204531284817264, 92.85377417485183571 ) ) ;
#46781=CARTESIAN_POINT ( 'NONE',  ( 185.1660960081723886, 84.30194217633003007, 3.668103655852483325 ) ) ;
#46782=CARTESIAN_POINT ( 'NONE',  ( 210.5178985598940926, 114.6803933586780886, -39.08928032852175960 ) ) ;
#46783=CARTESIAN_POINT ( 'NONE',  ( 179.4207200232660568, 76.93724985992177778, 17.32800239155928068 ) ) ;
#46785=CARTESIAN_POINT ( 'NONE',  ( 133.8566784816069344, -170.0000000000000000, 90.69944201992272781 ) ) ;
#46786=ORIENTED_EDGE ( 'NONE', *, *, #54208, .T. ) ;
#46787=CARTESIAN_POINT ( 'NONE',  ( -71.26746920569851795, 20.70422440535243069, 63.50986984570365479 ) ) ;
#46789=CARTESIAN_POINT ( 'NONE',  ( 58.09436971064712907, 11.58462396079456802, -64.38444416366542100 ) ) ;
#46792=CARTESIAN_POINT ( 'NONE',  ( -12.63247621924076114, 7.251801145016834482, 85.53860919323375356 ) ) ;
#46793=EDGE_CURVE ( 'NONE', #36510, #46532, #57133, .T. ) ;
#46795=EDGE_CURVE ( 'NONE', #48827, #64204, #49540, .T. ) ;
#46796=CARTESIAN_POINT ( 'NONE',  ( -109.5157885508426716, 37.76058765671429995, -13.62891770046948636 ) ) ;
#46798=CARTESIAN_POINT ( 'NONE',  ( -78.18913509716429644, 22.13995206110505265, 72.26275173013681297 ) ) ;
#46799=CARTESIAN_POINT ( 'NONE',  ( -171.0758681675585251, 84.87997360100519018, 72.39440660477549727 ) ) ;
#46801=EDGE_LOOP ( 'NONE', ( #11001, #51528 ) ) ;
#46804=CARTESIAN_POINT ( 'NONE',  ( 178.1903523079566583, 75.72906488635184985, -23.81340345046014306 ) ) ;
#46806=FACE_OUTER_BOUND ( 'NONE', #17093, .T. ) ;
#46813=CARTESIAN_POINT ( 'NONE',  ( 212.1535111375854683, 117.1635556319084657, 10.69408520456943990 ) ) ;
#46814=CARTESIAN_POINT ( 'NONE',  ( 8.767814708128303991, 7.383611927972574485, 61.70909310710061391 ) ) ;
#46819=ORIENTED_EDGE ( 'NONE', *, *, #276, .F. ) ;
#46823=CARTESIAN_POINT ( 'NONE',  ( -166.9969673948021125, 80.56076768517786491, -11.02977705128494357 ) ) ;
#46824=CARTESIAN_POINT ( 'NONE',  ( -173.1211646369891071, 88.63826465341152527, 18.97714401617737323 ) ) ;
#46825=CARTESIAN_POINT ( 'NONE',  ( 23.20798354347975589, 6.851551394716612897, 89.92625127541417385 ) ) ;
#46829=CARTESIAN_POINT ( 'NONE',  ( -100.4262673593280368, 31.84860241619272969, 72.14605430199947023 ) ) ;
#46830=EDGE_LOOP ( 'NONE', ( #3028, #67417, #63440, #11729 ) ) ;
#46831=CARTESIAN_POINT ( 'NONE',  ( -85.34215807311491631, 24.97769003780923569, 14.50119405095866831 ) ) ;
#46834=LINE ( 'NONE', #20437, #27620 ) ;
#46835=EDGE_LOOP ( 'NONE', ( #5299, #56334, #58046, #1815 ) ) ;
#46836=VERTEX_POINT ( 'NONE', #44633 ) ;
#46837=CARTESIAN_POINT ( 'NONE',  ( 46.12582897016705630, 10.39833982076225460, 67.59008823216548478 ) ) ;
#46838=CARTESIAN_POINT ( 'NONE',  ( -106.3047475500521557, 36.01269213589261398, -89.86034216495879434 ) ) ;
#46839=CARTESIAN_POINT ( 'NONE',  ( 130.7260704202054455, 39.56565398554879920, 57.02343801570094683 ) ) ;
#46840=VERTEX_POINT ( 'NONE', #39706 ) ;
#46843=EDGE_CURVE ( 'NONE', #3682, #34095, #41910, .T. ) ;
#46844=ADVANCED_FACE ( 'NONE', ( #20320 ), #24234, .F. ) ;
#46845=CARTESIAN_POINT ( 'NONE',  ( -24.22878282689200446, 8.518516047505652722, 93.49511739771224939 ) ) ;
#46847=CARTESIAN_POINT ( 'NONE',  ( 176.6156959113760365, 75.60152827082544036, -64.52720677928732584 ) ) ;
#46849=CARTESIAN_POINT ( 'NONE',  ( 106.6192711434718632, 27.24117154335862168, -49.99331757005764842 ) ) ;
#46852=AXIS2_PLACEMENT_3D ( 'NONE', #5787, #27244, #48678 ) ;
#46858=CARTESIAN_POINT ( 'NONE',  ( -81.23268307104842734, 24.39742801172155140, -76.51131192360561784 ) ) ;
#46860=CARTESIAN_POINT ( 'NONE',  ( 133.8566784816069060, 42.60093787723656789, -89.71241211332301191 ) ) ;
#46863=CARTESIAN_POINT ( 'NONE',  ( 126.3737790127712799, 37.08609730334947585, 10.73674426291554873 ) ) ;
#46865=CARTESIAN_POINT ( 'NONE',  ( -120.0051930351106932, 43.92079660368833061, -64.60660167447554159 ) ) ;
#46866=LINE ( 'NONE', #41252, #61338 ) ;
#46867=DIRECTION ( 'NONE',  ( -0.000000000000000000, 1.000000000000000000, -0.000000000000000000 ) ) ;
#46869=EDGE_LOOP ( 'NONE', ( #32126, #6172, #60390, #1121 ) ) ;
#46872=CARTESIAN_POINT ( 'NONE',  ( -57.54960251878999600, 16.40992651131772817, 84.42727806790901468 ) ) ;
#46873=ORIENTED_EDGE ( 'NONE', *, *, #61849, .T. ) ;
#46874=CARTESIAN_POINT ( 'NONE',  ( 201.6034029841262907, 102.1956603101140928, -10.13592553938994101 ) ) ;
#46875=ORIENTED_EDGE ( 'NONE', *, *, #66338, .F. ) ;
#46876=CARTESIAN_POINT ( 'NONE',  ( 16.77480716385437276, 7.540753720029939267, -77.31445149746915035 ) ) ;
#46880=ADVANCED_FACE ( 'NONE', ( #4157 ), #14365, .F. ) ;
#46882=CARTESIAN_POINT ( 'NONE',  ( 140.7888851157410386, 46.97220912571248874, -40.64884308134027435 ) ) ;
#46883=CARTESIAN_POINT ( 'NONE',  ( 32.46582151331404731, 7.608418548522502434, -40.23543673364789441 ) ) ;
#46884=CARTESIAN_POINT ( 'NONE',  ( 197.5101196254995841, 96.97937853946277187, 92.57920919658415926 ) ) ;
#46885=CARTESIAN_POINT ( 'NONE',  ( 8.537735592981560373, 7.383000420390740004, -41.08501613461158541 ) ) ;
#46888=FACE_OUTER_BOUND ( 'NONE', #59519, .T. ) ;
#46889=ORIENTED_EDGE ( 'NONE', *, *, #14460, .F. ) ;
#46891=CARTESIAN_POINT ( 'NONE',  ( 173.7992108938316846, 72.92047568072842978, 88.67055234059489521 ) ) ;
#46893=CARTESIAN_POINT ( 'NONE',  ( 9.827939172326075834, 6.382931149346554811, 15.24920466621778203 ) ) ;
#46895=B_SPLINE_CURVE_WITH_KNOTS ( 'NONE', 3,
 ( #67932, #8490, #30984, #19033, #51740, #2862, #47141, #14791, #30291, #41187, #45775, #35912, #52081, #13756, #3546, #63334, #8841, #19377, #62649, #62293, #25017, #51051, #29939, #35214, #3901, #35565, #36254, #51405, #9523, #68273, #15144, #46450, #62983, #19729, #25369, #9177, #57364, #14457, #46804, #14105, #57710, #3217, #24329, #36603 ),
 .UNSPECIFIED., .F., .F.,
 ( 4, 2, 2, 2, 2, 2, 2, 2, 2, 2, 2, 2, 2, 2, 2, 2, 2, 2, 2, 2, 2, 4 ),
 ( 0.000000000000000000, 0.003518733725596298340, 0.004398417156995381057, 0.005278100588394462472, 0.007037467451192679080, 0.007917150882591750954, 0.008796834313990822829, 0.01055620117678900995, 0.01231556803958719880, 0.01319525147098629322, 0.01407493490238538765, 0.01495461833378448034, 0.01583430176518357130, 0.01671398519658266746, 0.01759366862798176015, 0.01935303549077993165, 0.02111240235357809969, 0.02199208578497716463, 0.02287176921637622609, 0.02463113607917437331, 0.02639050294197252053, 0.02814986980477066775 ),
 .UNSPECIFIED. ) ;
#46901=CARTESIAN_POINT ( 'NONE',  ( -24.60892750534350881, 9.584951112520228023, 61.45297857596762725 ) ) ;
#46910=CYLINDRICAL_SURFACE ( 'NONE', #54822, 7.500000000000027534 ) ;
#46913=VECTOR ( 'NONE', #27108, 1000.000000000000000 ) ;
#46915=CARTESIAN_POINT ( 'NONE',  ( -190.3636887049961786, 108.6554956426205933, -91.83124475734037162 ) ) ;
#46916=CARTESIAN_POINT ( 'NONE',  ( -59.36813706141737867, 15.88103696331963377, 70.80079528359327412 ) ) ;
#46917=EDGE_LOOP ( 'NONE', ( #39261, #23579, #37265, #15294 ) ) ;
#46922=CARTESIAN_POINT ( 'NONE',  ( -175.9970298498767534, 90.38640259140140643, -75.99633293260467326 ) ) ;
#46923=CARTESIAN_POINT ( 'NONE',  ( 138.7757999158632742, 45.66865872093048750, -91.53672265411847775 ) ) ;
#46927=B_SPLINE_CURVE_WITH_KNOTS ( 'NONE', 3,
 ( #26065, #63350, #9191, #20094, #24689, #14804, #9541, #62308, #52101, #67948, #35928, #19743, #35585, #41206, #3916, #41890, #20776, #31000, #42238, #57729, #52448, #14122, #58072, #47157, #63701, #30650, #15161, #25388, #4265, #25728, #36268, #57380, #3232, #41547, #68621, #62665, #8857, #63002, #8507, #57043, #67597, #20426, #47492, #40855, #46126, #68289, #36622, #14473, #36966, #9890, #30307, #31343 ),
 .UNSPECIFIED., .F., .F.,
 ( 4, 2, 2, 2, 2, 2, 2, 2, 2, 2, 2, 2, 2, 2, 2, 2, 2, 2, 2, 2, 2, 2, 2, 2, 2, 4 ),
 ( 0.000000000000000000, 0.002032670951089465741, 0.003049006426634202297, 0.004065341902178939287, 0.005081677377723675844, 0.006098012853268411533, 0.007114348328813148090, 0.008130683804357885514, 0.009147019279902621203, 0.01016335475544735863, 0.01219602570653683001, 0.01422869665762630312, 0.01626136760871577797, 0.01727770308426054835, 0.01829403855980532220, 0.02032670951089484562, 0.02134304498643961254, 0.02235938046198437598, 0.02337571593752914290, 0.02439205141307390634, 0.02642472236416344364, 0.02845739331525297400, 0.02947372879079776173, 0.03049006426634255293, 0.03150639974188734066, 0.03252273521743212492 ),
 .UNSPECIFIED. ) ;
#46928=CARTESIAN_POINT ( 'NONE',  ( 55.52751777340358785, 12.08567914268656374, -42.73101172783196233 ) ) ;
#46929=CARTESIAN_POINT ( 'NONE',  ( -84.21836162213176635, 25.60181819557222127, 32.85243609328976788 ) ) ;
#46930=CARTESIAN_POINT ( 'NONE',  ( 150.9834489474288830, 52.77764236634784112, 94.42848054783445377 ) ) ;
#46931=CARTESIAN_POINT ( 'NONE',  ( 94.06703982324142999, 22.09435144471462564, 38.20947434515352370 ) ) ;
#46932=EDGE_CURVE ( 'NONE', #22488, #14559, #57957, .T. ) ;
#46933=ORIENTED_EDGE ( 'NONE', *, *, #17569, .T. ) ;
#46934=CARTESIAN_POINT ( 'NONE',  ( 15.78827728214693060, 6.500811158483329244, 71.85925826316895382 ) ) ;
#46936=CARTESIAN_POINT ( 'NONE',  ( -29.74902699556086816, 10.33856194202125600, 45.02758640895530817 ) ) ;
#46939=CARTESIAN_POINT ( 'NONE',  ( -71.68176805937196150, 20.84773878116192947, 94.41661040422935969 ) ) ;
#46942=CARTESIAN_POINT ( 'NONE',  ( 63.50537371531940778, 13.81987663608981798, 44.81296093922130552 ) ) ;
#46944=VERTEX_POINT ( 'NONE', #37185 ) ;
#46948=CARTESIAN_POINT ( 'NONE',  ( 197.9847015768255005, 97.56951352050450055, -67.31407702796413162 ) ) ;
#46949=CARTESIAN_POINT ( 'NONE',  ( -35.17296606710974061, 11.25626711331309338, 58.03790650501060355 ) ) ;
#46951=CARTESIAN_POINT ( 'NONE',  ( -84.53753601793930272, 25.73343139558518544, -20.46458922348523046 ) ) ;
#46953=CARTESIAN_POINT ( 'NONE',  ( -156.4960819023051783, 70.34114605623875605, -39.53833954081760993 ) ) ;
#46957=CARTESIAN_POINT ( 'NONE',  ( -109.4995148930278361, 37.75156937139181679, 9.075767506675283869 ) ) ;
#46960=CARTESIAN_POINT ( 'NONE',  ( -190.3061188229048639, 108.5745819235682035, 69.14762690905678255 ) ) ;
#46971=CARTESIAN_POINT ( 'NONE',  ( -84.55373779407986490, 24.65190748253135666, 60.08995505548700322 ) ) ;
#46974=CARTESIAN_POINT ( 'NONE',  ( -152.2964402771109178, 66.58174574061953876, -8.502547355955140773 ) ) ;
#46975=CARTESIAN_POINT ( 'NONE',  ( 33.75639351246965703, 7.742023566824295600, 59.29622260418393154 ) ) ;
#46978=CARTESIAN_POINT ( 'NONE',  ( 16.77480716385437276, 7.540753720029938378, 3.219200273921916544 ) ) ;
#46980=CARTESIAN_POINT ( 'NONE',  ( -122.7930600691577752, 44.48546375740916403, 18.12006331166574924 ) ) ;
#46981=CARTESIAN_POINT ( 'NONE',  ( 63.01563776193091826, 12.67277567978498709, -62.56524142263340593 ) ) ;
#46982=CARTESIAN_POINT ( 'NONE',  ( 16.27765348919938049, 6.516472002017813736, 56.85925826316893961 ) ) ;
#46983=FACE_OUTER_BOUND ( 'NONE', #2858, .T. ) ;
#46984=CARTESIAN_POINT ( 'NONE',  ( 8.288696687633805738, 7.382586467017838494, 10.16927303540167671 ) ) ;
#46986=CYLINDRICAL_SURFACE ( 'NONE', #10245, 7.500000000000013323 ) ;
#46988=CARTESIAN_POINT ( 'NONE',  ( 131.6115093721024607, 41.25402743071400380, -50.68309935467904381 ) ) ;
#46992=CARTESIAN_POINT ( 'NONE',  ( 187.5246323291927126, 86.86207184872510823, -39.84316934690760803 ) ) ;
#46994=ORIENTED_EDGE ( 'NONE', *, *, #1780, .T. ) ;
#47000=VECTOR ( 'NONE', #23820, 1000.000000000000000 ) ;
#47002=CARTESIAN_POINT ( 'NONE',  ( 115.0692128464502559, 31.17922615202196113, 69.71731335093312509 ) ) ;
#47003=VERTEX_POINT ( 'NONE', #21351 ) ;
#47004=CARTESIAN_POINT ( 'NONE',  ( -62.41727141396691536, 17.83188754031767687, 12.45580772492516708 ) ) ;
#47005=CARTESIAN_POINT ( 'NONE',  ( 126.6395826915640015, 37.23416510613628105, 34.95296513652632342 ) ) ;
#47008=CARTESIAN_POINT ( 'NONE',  ( -94.79166046756729713, 29.13671350128076654, 38.51002725759197887 ) ) ;
#47014=ORIENTED_EDGE ( 'NONE', *, *, #37624, .T. ) ;
#47016=CARTESIAN_POINT ( 'NONE',  ( -168.0003605155415869, 83.06333427281272463, 5.991919408726039009 ) ) ;
#47019=CARTESIAN_POINT ( 'NONE',  ( -148.6426892915312408, 64.76241938621075178, -34.81283053149196860 ) ) ;
#47020=EDGE_CURVE ( 'NONE', #3542, #24590, #57863, .T. ) ;
#47022=CARTESIAN_POINT ( 'NONE',  ( -132.8150886319751294, 52.45790550853839562, 62.06390996835829554 ) ) ;
#47023=VERTEX_POINT ( 'NONE', #49459 ) ;
#47024=DIRECTION ( 'NONE',  ( 0.000000000000000000, 0.000000000000000000, 1.000000000000000000 ) ) ;
#47026=EDGE_LOOP ( 'NONE', ( #60917, #598 ) ) ;
#47028=CARTESIAN_POINT ( 'NONE',  ( -61.75629144857964548, 16.58190704077737720, -12.49911615342323579 ) ) ;
#47029=CARTESIAN_POINT ( 'NONE',  ( -133.2787743207941276, 52.78950725740546090, -67.92237397683200584 ) ) ;
#47030=CARTESIAN_POINT ( 'NONE',  ( 61.01086442919169883, 12.21637211111878862, -89.67119804626783264 ) ) ;
#47032=CARTESIAN_POINT ( 'NONE',  ( 68.62997155117719217, 15.08415013720829023, -65.06837658636030142 ) ) ;
#47035=CARTESIAN_POINT ( 'NONE',  ( 184.0013086981202548, 81.60415045669142842, -63.64686322466085500 ) ) ;
#47036=CARTESIAN_POINT ( 'NONE',  ( -165.9122696334865168, 79.44688201528256855, -44.30228794590340868 ) ) ;
#47039=CARTESIAN_POINT ( 'NONE',  ( -71.57660578921961303, 20.81129687646280146, 40.41523763771648703 ) ) ;
#47043=CARTESIAN_POINT ( 'NONE',  ( -169.8842709557924593, 83.59602878049473418, -75.83670934591202695 ) ) ;
#47045=CARTESIAN_POINT ( 'NONE',  ( -149.5074843970971301, -170.0000000000000000, -42.31283053149197571 ) ) ;
#47046=ORIENTED_EDGE ( 'NONE', *, *, #46621, .T. ) ;
#47047=CARTESIAN_POINT ( 'NONE',  ( -38.55214349681827457, 10.86754840574841907, 8.443293971405456233 ) ) ;
#47051=CARTESIAN_POINT ( 'NONE',  ( 32.90051628396145844, 8.664124555952446016, 6.797922165733859323 ) ) ;
#47053=B_SPLINE_CURVE_WITH_KNOTS ( 'NONE', 3,
 ( #3144, #35839, #8771, #8057, #41801, #24256, #68198, #40411, #62211, #45697, #67502, #63260, #8413, #57291, #15066, #30217, #25290, #67176, #52007, #9447, #3822, #30907, #35489, #52354, #51669, #35139, #4170, #62571, #3475, #46376, #25638, #47070, #61858, #67853, #13681, #36523, #19299, #64284, #68859, #48421, #31939, #63604, #63941, #48772, #52684, #42140, #20683, #43160 ),
 .UNSPECIFIED., .F., .F.,
 ( 4, 2, 2, 2, 2, 2, 2, 2, 2, 2, 2, 2, 2, 2, 2, 2, 2, 2, 2, 2, 2, 2, 2, 4 ),
 ( 0.02698595842317762922, 0.02784423243973397494, 0.02870250645629031719, 0.03041905448940304679, 0.03127732850595942027, 0.03213560252251579374, 0.03385215055562854763, 0.03471042457218491417, 0.03556869858874128071, 0.03728524662185400684, 0.03814352063841035256, 0.03900179465496669828, 0.03986006867152304400, 0.04071834268807938972, 0.04157661670463573544, 0.04243489072119208810, 0.04415143875430482118, 0.04500971277086116690, 0.04586798678741751956, 0.04758453482053019712, 0.04930108285364286774, 0.05101763088675554531, 0.05273417891986822287, 0.05445072695298090043 ),
 .UNSPECIFIED. ) ;
#47056=CARTESIAN_POINT ( 'NONE',  ( -13.47517652744367034, 8.334971000693554899, -37.96130542306915601 ) ) ;
#47057=CARTESIAN_POINT ( 'NONE',  ( -31.43908319763709969, 10.61114334766716105, -23.47264677473818395 ) ) ;
#47061=CARTESIAN_POINT ( 'NONE',  ( 63.01563776193091826, 13.70579113808095251, 56.65751152968497451 ) ) ;
#47062=CARTESIAN_POINT ( 'NONE',  ( 9.819093282782493048, 7.389085782749409859, -65.29636817529980419 ) ) ;
#47063=CARTESIAN_POINT ( 'NONE',  ( -28.81317668042940028, 9.175023678939295380, 3.842413854045814148 ) ) ;
#47065=CARTESIAN_POINT ( 'NONE',  ( -61.71141560932036185, 16.56840812182238309, -92.92626464638486539 ) ) ;
#47067=CARTESIAN_POINT ( 'NONE',  ( 152.1153500913667074, 54.85403770686896507, -38.36719606911704972 ) ) ;
#47068=ORIENTED_EDGE ( 'NONE', *, *, #63763, .F. ) ;
#47070=CARTESIAN_POINT ( 'NONE',  ( -156.6862310659955995, 71.88416263379568250, 67.30894339101347157 ) ) ;
#47071=CARTESIAN_POINT ( 'NONE',  ( 181.0840389613909736, 80.03940679743416808, -24.38050707541595230 ) ) ;
#47072=CARTESIAN_POINT ( 'NONE',  ( -105.4487797565984408, 35.55724615608638572, 58.04979929862538768 ) ) ;
#47073=CARTESIAN_POINT ( 'NONE',  ( -126.7944042662568478, 48.29830493043728268, -49.87326901552447822 ) ) ;
#47074=ORIENTED_EDGE ( 'NONE', *, *, #64995, .T. ) ;
#47076=CARTESIAN_POINT ( 'NONE',  ( 88.30010642107258434, 19.99780058782975090, 71.37213675879502262 ) ) ;
#47077=CARTESIAN_POINT ( 'NONE',  ( 117.3281529665582070, 32.29994712002881840, 39.62392251532779142 ) ) ;
#47078=EDGE_CURVE ( 'NONE', #41738, #51274, #23797, .T. ) ;
#47083=CARTESIAN_POINT ( 'NONE',  ( -196.7348448768811409, -170.0000000000000000, 65.26711856384670796 ) ) ;
#47085=CARTESIAN_POINT ( 'NONE',  ( 186.0827296088606602, 85.28826835108064586, 42.40481399445034327 ) ) ;
#47086=CARTESIAN_POINT ( 'NONE',  ( 158.3636111008086687, 59.62671916656142201, 17.56491688178971700 ) ) ;
#47091=CARTESIAN_POINT ( 'NONE',  ( 177.0110682437507990, 75.98481089748385386, 57.33934894850843023 ) ) ;
#47092=EDGE_LOOP ( 'NONE', ( #51116, #3611, #60587, #20752 ) ) ;
#47093=CARTESIAN_POINT ( 'NONE',  ( -109.7290872258107157, 36.72869630780159156, -43.53384799749126444 ) ) ;
#47094=CARTESIAN_POINT ( 'NONE',  ( 136.9580891181123548, 43.32873266151486291, 83.86339557539821499 ) ) ;
#47096=CARTESIAN_POINT ( 'NONE',  ( -62.48965350618345127, 16.80247907725180667, 38.81988781192542604 ) ) ;
#47097=CARTESIAN_POINT ( 'NONE',  ( 157.2533363798600021, 58.75760182111575602, 2.564916881789686798 ) ) ;
#47099=CYLINDRICAL_SURFACE ( 'NONE', #4967, 7.500000000000013323 ) ;
#47100=LINE ( 'NONE', #36900, #42891 ) ;
#47102=CARTESIAN_POINT ( 'NONE',  ( 112.5612011511790058, 31.08353758940340938, -50.57087292189984140 ) ) ;
#47104=DIRECTION ( 'NONE',  ( 0.000000000000000000, 0.000000000000000000, 1.000000000000000000 ) ) ;
#47107=CARTESIAN_POINT ( 'NONE',  ( 141.2811136745702640, 46.09188267874201728, 62.75964268212607067 ) ) ;
#47108=CARTESIAN_POINT ( 'NONE',  ( -165.7138623879809529, 79.24467249981145756, 39.53662309097534688 ) ) ;
#47110=CARTESIAN_POINT ( 'NONE',  ( 91.49210130311617206, 22.20929244416437953, 42.92723601512285114 ) ) ;
#47112=CARTESIAN_POINT ( 'NONE',  ( 44.34689728705969003, 10.12166135033765180, 16.22939414383014878 ) ) ;
#47113=VERTEX_POINT ( 'NONE', #7628 ) ;
#47115=CARTESIAN_POINT ( 'NONE',  ( 157.0357419681844249, 58.58786672900117765, -24.27023266159657666 ) ) ;
#47116=CARTESIAN_POINT ( 'NONE',  ( -58.12888781187205467, 15.52769087903062406, 84.65900618614021766 ) ) ;
#47119=CARTESIAN_POINT ( 'NONE',  ( 56.17239497942856019, 11.18888580659344179, 87.91446924145196817 ) ) ;
#47120=CARTESIAN_POINT ( 'NONE',  ( 187.6511924654682559, 87.00187850361885467, 6.331325941773287447 ) ) ;
#47126=CARTESIAN_POINT ( 'NONE',  ( -71.97658551692138929, 20.95070248419152747, 61.36288391214083049 ) ) ;
#47127=CARTESIAN_POINT ( 'NONE',  ( 43.35536254672138057, 9.973606330917816010, -22.65335710938210312 ) ) ;
#47130=CARTESIAN_POINT ( 'NONE',  ( 20.35964562795319566, 7.697260051881317899, 43.48066962168281435 ) ) ;
#47132=CARTESIAN_POINT ( 'NONE',  ( -104.5740066103012254, 35.09687312794776659, -22.81448265554261212 ) ) ;
#47135=CARTESIAN_POINT ( 'NONE',  ( -74.40004226286976063, 20.74218500375953766, 58.58967130592457551 ) ) ;
#47139=CARTESIAN_POINT ( 'NONE',  ( -154.0718453320783397, 68.14976693162391541, 32.26507081757433326 ) ) ;
#47140=CARTESIAN_POINT ( 'NONE',  ( 56.30171512200996631, 11.21502580416395567, -39.86886612370064853 ) ) ;
#47141=CARTESIAN_POINT ( 'NONE',  ( 177.5945652320813792, 75.14951358071813559, -10.23784609841178295 ) ) ;
#47143=CARTESIAN_POINT ( 'NONE',  ( -144.7571537022063808, 60.25265659240449168, 5.567462641871050444 ) ) ;
#47147=CARTESIAN_POINT ( 'NONE',  ( -127.6894679065405427, 48.89973668460849865, 45.41578626271343211 ) ) ;
#47148=VERTEX_POINT ( 'NONE', #22397 ) ;
#47149=CARTESIAN_POINT ( 'NONE',  ( 16.77480716385436921, 7.540753720029938378, -50.46990090700543874 ) ) ;
#47150=CARTESIAN_POINT ( 'NONE',  ( -143.7133518487516994, 60.70463114991425613, 42.98969525936463043 ) ) ;
#47154=ORIENTED_EDGE ( 'NONE', *, *, #2529, .T. ) ;
#47157=CARTESIAN_POINT ( 'NONE',  ( -124.8392882614943602, 47.00413044825191378, 84.36113447088062856 ) ) ;
#47158=LINE ( 'NONE', #20777, #40850 ) ;
#47159=CARTESIAN_POINT ( 'NONE',  ( -180.0154536325058245, 96.73346874014741559, 14.44416461865400869 ) ) ;
#47161=CARTESIAN_POINT ( 'NONE',  ( 14.15607123919027188, 6.453851046686879478, 83.87628020752921998 ) ) ;
#47162=AXIS2_PLACEMENT_3D ( 'NONE', #17530, #28434, #22462 ) ;
#47163=CARTESIAN_POINT ( 'NONE',  ( 10.70820696327198895, 7.397428319378121842, 85.67662758554656932 ) ) ;
#47167=CARTESIAN_POINT ( 'NONE',  ( -101.8191498210055101, 32.54686850610961812, 57.36362509687882039 ) ) ;
#47169=CARTESIAN_POINT ( 'NONE',  ( -79.14127775978542445, 22.50259208414362178, 3.573650549209442584 ) ) ;
#47175=CARTESIAN_POINT ( 'NONE',  ( -121.5928001448269100, 44.91559452735374691, 17.43750400987426374 ) ) ;
#47177=EDGE_CURVE ( 'NONE', #41403, #47540, #7273, .T. ) ;
#47178=CARTESIAN_POINT ( 'NONE',  ( -180.5230320745700396, 95.76406004447548526, 63.91740180504579172 ) ) ;
#47179=EDGE_CURVE ( 'NONE', #26262, #2286, #60019, .T. ) ;
#47180=CARTESIAN_POINT ( 'NONE',  ( 127.4750938923429402, 37.70245908594340989, 59.90632388648024431 ) ) ;
#47182=DIRECTION ( 'NONE',  ( -0.000000000000000000, 1.000000000000000000, -0.000000000000000000 ) ) ;
#47183=CARTESIAN_POINT ( 'NONE',  ( -51.77779688167512262, 14.86590802019196822, 4.221165638100599082 ) ) ;
#47185=CARTESIAN_POINT ( 'NONE',  ( 105.2506154496929582, 26.63995206619728506, -37.82003446714997352 ) ) ;
#47186=B_SPLINE_CURVE_WITH_KNOTS ( 'NONE', 3,
 ( #8098, #13721, #29548, #35177, #60519, #2825, #66174, #56631, #34151, #51365, #24294, #12336, #45736, #50659, #18306, #33793, #28871, #45030, #67214, #7056, #28513, #2479 ),
 .UNSPECIFIED., .F., .F.,
 ( 4, 2, 2, 2, 2, 2, 2, 2, 2, 2, 4 ),
 ( 0.000000000000000000, 0.001562679269560080398, 0.003125358539120160796, 0.003906698173900237207, 0.004688037808680313619, 0.006250717078240390981, 0.007032056713020401473, 0.007813396347800413699, 0.009376075617360434683, 0.01093875488692046954, 0.01250143415648050441 ),
 .UNSPECIFIED. ) ;
#47187=CARTESIAN_POINT ( 'NONE',  ( -28.13852122803040601, 9.072484007196642608, 30.96421423579666765 ) ) ;
#47193=CARTESIAN_POINT ( 'NONE',  ( -82.32006615997346444, 24.83050031643766076, -76.02779720937938635 ) ) ;
#47194=CARTESIAN_POINT ( 'NONE',  ( 174.6242782760050432, 73.69713439533578025, 13.78395099967788440 ) ) ;
#47197=CARTESIAN_POINT ( 'NONE',  ( 127.4953815656694758, 37.71366486045442201, 14.17018500853721008 ) ) ;
#47198=CARTESIAN_POINT ( 'NONE',  ( 35.12301194579454489, 7.891331172724800780, -90.63528273682473468 ) ) ;
#47200=CARTESIAN_POINT ( 'NONE',  ( 210.6584452238134588, 116.7138338345753539, 32.12903558767059309 ) ) ;
#47201=CARTESIAN_POINT ( 'NONE',  ( 162.7921669283191761, 61.91024532638674316, 4.774496695581312622 ) ) ;
#47202=CARTESIAN_POINT ( 'NONE',  ( -108.0980548770427561, 35.83569586822708430, 42.77788030405751840 ) ) ;
#47203=VERTEX_POINT ( 'NONE', #65314 ) ;
#47204=CARTESIAN_POINT ( 'NONE',  ( -58.96642505241147347, 16.81239758210119817, 85.10078055707477063 ) ) ;
#47207=EDGE_LOOP ( 'NONE', ( #45415, #52508 ) ) ;
#47208=CARTESIAN_POINT ( 'NONE',  ( 23.23965501943000689, 7.861749956303023978, -70.84722685082371640 ) ) ;
#47210=CARTESIAN_POINT ( 'NONE',  ( -144.3939084932120807, 61.25241660819417433, 70.55718103091443538 ) ) ;
#47212=CARTESIAN_POINT ( 'NONE',  ( 141.1220430186942565, 47.19066702031172866, -41.64338897693998831 ) ) ;
#47213=CARTESIAN_POINT ( 'NONE',  ( 35.65685430025424552, 7.951642554322392087, -36.60339655490213318 ) ) ;
#47215=CARTESIAN_POINT ( 'NONE',  ( 150.0889146124742695, 52.13243511955543141, -44.98044688291916060 ) ) ;
#47216=DIRECTION ( 'NONE',  ( -0.8118923937861950435, -0.5838071093367415143, 0.000000000000000000 ) ) ;
#47221=CARTESIAN_POINT ( 'NONE',  ( 177.3158870624719725, 76.28207752284875198, 84.00542473672297206 ) ) ;
#47227=CARTESIAN_POINT ( 'NONE',  ( 46.12611922993086466, 10.39838587005582404, -73.29553601737912061 ) ) ;
#47229=CARTESIAN_POINT ( 'NONE',  ( 173.6718135456486607, 71.42581476597408141, -69.38831629246477917 ) ) ;
#47231=CARTESIAN_POINT ( 'NONE',  ( 94.12811352634520290, 22.11743943276051638, -17.00099467980526313 ) ) ;
#47232=CARTESIAN_POINT ( 'NONE',  ( -29.51272929882557605, 10.30144624948894361, 71.81352569274244502 ) ) ;
#47239=CARTESIAN_POINT ( 'NONE',  ( 126.4318266066171930, 38.27072266789465260, 9.074042217399220789 ) ) ;
#47242=CARTESIAN_POINT ( 'NONE',  ( -109.5157885508426716, 37.76058765671429285, -67.31801888139685275 ) ) ;
#47243=CARTESIAN_POINT ( 'NONE',  ( -51.77439426130689526, 13.82695438436704016, -35.96638716134758340 ) ) ;
#47245=EDGE_LOOP ( 'NONE', ( #3495, #54792 ) ) ;
#47247=CARTESIAN_POINT ( 'NONE',  ( -59.94781924509481286, 16.04872117907065743, 70.34947420817375985 ) ) ;
#47249=ORIENTED_EDGE ( 'NONE', *, *, #55104, .F. ) ;
#47250=CARTESIAN_POINT ( 'NONE',  ( 32.21871194187785648, 8.594856915925895180, 88.92095415218777532 ) ) ;
#47252=CARTESIAN_POINT ( 'NONE',  ( 110.2429982417149432, 28.88204397445228722, 44.61121420573733332 ) ) ;
#47257=CARTESIAN_POINT ( 'NONE',  ( 33.44983424733138122, 7.709709042132399937, -11.68551422328344280 ) ) ;
#47258=EDGE_CURVE ( 'NONE', #36885, #17268, #62852, .T. ) ;
#47260=EDGE_CURVE ( 'NONE', #29791, #67595, #69334, .T. ) ;
#47262=CARTESIAN_POINT ( 'NONE',  ( -153.1031717208031750, 68.63449618039564371, -75.74321926140552819 ) ) ;
#47263=CARTESIAN_POINT ( 'NONE',  ( 90.91465859190770971, 20.92790537681856478, 31.05212256305487983 ) ) ;
#47264=VECTOR ( 'NONE', #5621, 1000.000000000000000 ) ;
#47269=LINE ( 'NONE', #9298, #37919 ) ;
#47270=CARTESIAN_POINT ( 'NONE',  ( 8.848532605049253874, 6.377649401037234433, 67.23478819807002083 ) ) ;
#47272=CARTESIAN_POINT ( 'NONE',  ( 199.2049631873263422, 100.7347227143600037, 41.82079194744246564 ) ) ;
#47273=CARTESIAN_POINT ( 'NONE',  ( -71.26176386603191304, 20.70224608353110796, 92.84341710835518313 ) ) ;
#47278=CARTESIAN_POINT ( 'NONE',  ( 86.62931800182293784, 19.42108912189596381, 56.55663816294300261 ) ) ;
#47279=CARTESIAN_POINT ( 'NONE',  ( 197.3054165770396082, 96.72615186924558373, -71.97836107770491765 ) ) ;
#47280=DIRECTION ( 'NONE',  ( -0.000000000000000000, 1.000000000000000000, -0.000000000000000000 ) ) ;
#47282=CARTESIAN_POINT ( 'NONE',  ( 150.4550062612853480, 52.39582885725847916, -67.76395233042956079 ) ) ;
#47283=CARTESIAN_POINT ( 'NONE',  ( 20.36314374176838982, 6.689939636827348046, -22.13797671587966320 ) ) ;
#47284=CARTESIAN_POINT ( 'NONE',  ( -155.7433525314458791, 69.65452735858369238, -38.13774150188479695 ) ) ;
#47286=ORIENTED_EDGE ( 'NONE', *, *, #46065, .T. ) ;
#47288=CARTESIAN_POINT ( 'NONE',  ( -85.10909119100207931, 25.97025675005451717, -46.48749614101045324 ) ) ;
#47289=CARTESIAN_POINT ( 'NONE',  ( 162.1014732644455023, 61.34312237409763213, 69.67267474247222481 ) ) ;
#47290=CARTESIAN_POINT ( 'NONE',  ( -154.0716379918897019, 69.49957566103795159, 5.406051683299049060 ) ) ;
#47294=ORIENTED_EDGE ( 'NONE', *, *, #39111, .F. ) ;
#47296=ORIENTED_EDGE ( 'NONE', *, *, #30895, .T. ) ;
#47298=CARTESIAN_POINT ( 'NONE',  ( -85.91089317961399274, 25.21459833389208782, 62.75547607985773624 ) ) ;
#47301=CARTESIAN_POINT ( 'NONE',  ( -34.74563762132953570, 11.17960945723136668, -62.92554498051175216 ) ) ;
#47303=CARTESIAN_POINT ( 'NONE',  ( 32.09567473596477782, 7.571373529017938253, 65.97000810165883422 ) ) ;
#47304=CARTESIAN_POINT ( 'NONE',  ( 13.84937401517046673, 6.446378549072246500, -8.925169506644754946 ) ) ;
#47307=CARTESIAN_POINT ( 'NONE',  ( 181.5072453427590347, 79.03352099595187497, 56.15314469597510083 ) ) ;
#47310=CARTESIAN_POINT ( 'NONE',  ( -0.4996266546846072631, 6.524616273922395848, -95.00000000000133582 ) ) ;
#47312=CARTESIAN_POINT ( 'NONE',  ( 17.73567516211396011, 7.577454475141601975, -23.43370752981164884 ) ) ;
#47313=CARTESIAN_POINT ( 'NONE',  ( 198.4017331595408962, 98.09114638179335088, 59.46790870869396883 ) ) ;
#47314=VECTOR ( 'NONE', #62950, 1000.000000000000000 ) ;
#47321=CARTESIAN_POINT ( 'NONE',  ( 174.1364721914477229, 71.85829564941444403, 33.96918356720905763 ) ) ;
#47323=CARTESIAN_POINT ( 'NONE',  ( -103.8932886509197004, 34.74144483217663293, -49.84274311153227188 ) ) ;
#47324=CARTESIAN_POINT ( 'NONE',  ( 184.3879440808139805, 83.47316703125157744, -36.98841972577437787 ) ) ;
#47327=CARTESIAN_POINT ( 'NONE',  ( -27.48703802937314933, 8.975952825337591534, -9.593638160064255516 ) ) ;
#47328=CARTESIAN_POINT ( 'NONE',  ( 203.1414537950835779, 105.9225671689748367, 17.21051589850434382 ) ) ;
#47332=CARTESIAN_POINT ( 'NONE',  ( 114.6659427952414632, 32.10199811723105512, 70.03145237251035837 ) ) ;
#47333=FACE_OUTER_BOUND ( 'NONE', #54957, .T. ) ;
#47336=CARTESIAN_POINT ( 'NONE',  ( -95.63568360745007624, 29.53168204475776548, 34.53108459816321130 ) ) ;
#47341=B_SPLINE_CURVE_WITH_KNOTS ( 'NONE', 3,
 ( #52793, #26081, #47511, #14821, #10922, #63372, #63717, #36295, #5311, #20443, #57749, #15861, #36982, #68970, #10235, #31699, #64393, #21477, #21154, #37308, #53133, #15181, #58763, #26771, #52464, #42598, #53823, #4962, #10577, #47180, #26427, #47868, #37656, #32045, #48197, #9909, #59109, #25408, #46839, #36643, #68311, #9560, #31025, #4287, #25749, #41909 ),
 .UNSPECIFIED., .F., .F.,
 ( 4, 2, 2, 2, 2, 2, 2, 2, 2, 2, 2, 2, 2, 2, 2, 2, 2, 2, 2, 2, 2, 2, 4 ),
 ( 6.938893903907228378E-18, 0.001572224531395625307, 0.003144449062791243674, 0.004716673594186861392, 0.006288898125582480410, 0.007861122656978098561, 0.009433347188373715844, 0.01021945945407154617, 0.01100557171976937303, 0.01179168398546720162, 0.01257779625116503194, 0.01415002078256068739, 0.01493613304825850557, 0.01572224531395632549, 0.01650835757965414888, 0.01729446984535196533, 0.01886669437674765026, 0.01965280664244548059, 0.02043891890814331438, 0.02201114343953897504, 0.02358336797093463916, 0.02436948023663243132, 0.02515559250233022348 ),
 .UNSPECIFIED. ) ;
#47345=CARTESIAN_POINT ( 'NONE',  ( -124.3331814159187303, 45.47486189329070783, -22.90848852574204031 ) ) ;
#47346=DIRECTION ( 'NONE',  ( -0.000000000000000000, 1.000000000000000000, -0.000000000000000000 ) ) ;
#47347=CARTESIAN_POINT ( 'NONE',  ( -179.8996803435689174, 95.00451760716448746, -12.14598228191335849 ) ) ;
#47348=CARTESIAN_POINT ( 'NONE',  ( -148.6409722988649946, 63.44808865916659357, -34.85989714948443918 ) ) ;
#47350=CARTESIAN_POINT ( 'NONE',  ( 58.47885130911549112, 12.69429933094348328, 4.475850833756106262 ) ) ;
#47354=B_SPLINE_CURVE_WITH_KNOTS ( 'NONE', 3,
 ( #52395, #35532, #56986, #8097, #30255, #61569, #4212, #46768, #51704, #24981, #56281, #46413, #62613, #45735, #35873, #57329, #9141, #20044, #67213, #41497, #62948, #18661, #13384, #25677, #13720, #47108, #40112, #52720, #48457, #37586, #54088, #21079, #32322, #69252, #64320, #48127, #5236, #26355, #63299, #10504, #26695, #20725, #68899, #42180, #5575, #41842 ),
 .UNSPECIFIED., .F., .F.,
 ( 4, 2, 2, 2, 2, 2, 2, 2, 2, 2, 2, 2, 2, 2, 2, 2, 2, 2, 2, 2, 2, 2, 4 ),
 ( 0.02989107162308292723, 0.03170280136394034581, 0.03351453110479776093, 0.03532626084565517605, 0.03713799058651259116, 0.03894972032737000628, 0.03985558519779868608, 0.04076145006822736588, 0.04166731493865603875, 0.04257317980908471855, 0.04347904467951339835, 0.04438490954994207816, 0.04529077442037075796, 0.04619663929079943776, 0.04710250416122811756, 0.04800836903165679737, 0.04891423390208547717, 0.04982009877251415697, 0.05163182851337153045, 0.05344355825422891781, 0.05525528799508629130, 0.05706701773594367866, 0.05887874747680105214 ),
 .UNSPECIFIED. ) ;
#47355=CARTESIAN_POINT ( 'NONE',  ( -57.42615654242919021, 15.33060010148602892, -8.753093045165913466 ) ) ;
#47357=CARTESIAN_POINT ( 'NONE',  ( -128.3448054685827913, 49.34430406923178225, -76.35012269041114052 ) ) ;
#47360=CARTESIAN_POINT ( 'NONE',  ( -97.88309373898363219, 30.60238467438962928, -75.45378525617154253 ) ) ;
#47361=VERTEX_POINT ( 'NONE', #44016 ) ;
#47363=CARTESIAN_POINT ( 'NONE',  ( 187.5325688887158151, 85.37769363979911930, -66.70143880898807254 ) ) ;
#47368=CARTESIAN_POINT ( 'NONE',  ( 104.3759779378692372, 27.35691041569132409, -65.56839599289385490 ) ) ;
#47370=CARTESIAN_POINT ( 'NONE',  ( 79.14129363775930415, 17.00055658855363205, 36.71904541452036597 ) ) ;
#47372=CARTESIAN_POINT ( 'NONE',  ( -118.4709174626548673, 42.97515378817186615, 39.22611101928199417 ) ) ;
#47373=CARTESIAN_POINT ( 'NONE',  ( -169.8791831685530553, 83.59058982490282119, -62.27878394338570445 ) ) ;
#47376=CARTESIAN_POINT ( 'NONE',  ( -107.0751323097254613, 35.28386110859231906, -21.45789132277915456 ) ) ;
#47378=CARTESIAN_POINT ( 'NONE',  ( -34.06864996337443330, 10.03773626259442331, 17.90007924047801779 ) ) ;
#47380=CARTESIAN_POINT ( 'NONE',  ( 79.19119222799088220, 18.06817527909835164, 65.05072483751119705 ) ) ;
#47383=FACE_OUTER_BOUND ( 'NONE', #41823, .T. ) ;
#47385=CARTESIAN_POINT ( 'NONE',  ( 36.09137906183515554, 8.001963043161770983, -76.69864084344654032 ) ) ;
#47387=CARTESIAN_POINT ( 'NONE',  ( -36.38071096718369546, 11.47804921491337815, -10.30964823013966303 ) ) ;
#47391=CARTESIAN_POINT ( 'NONE',  ( 57.41085175769453741, 12.46982565415947697, 59.16780719303546476 ) ) ;
#47393=CARTESIAN_POINT ( 'NONE',  ( -29.75049355503753645, 9.320234381800291956, 3.560369807396146502 ) ) ;
#47394=FACE_OUTER_BOUND ( 'NONE', #27717, .T. ) ;
#47397=CARTESIAN_POINT ( 'NONE',  ( 153.4509883044095773, 55.84811350575044031, -49.96048919769913255 ) ) ;
#47399=EDGE_CURVE ( 'NONE', #59711, #59702, #51142, .T. ) ;
#47404=CARTESIAN_POINT ( 'NONE',  ( 176.6156959113759513, 75.60152827082542615, -10.83810559835997900 ) ) ;
#47405=CARTESIAN_POINT ( 'NONE',  ( -109.7686203588201295, 37.90089348911613598, 65.35533321413022634 ) ) ;
#47408=CARTESIAN_POINT ( 'NONE',  ( -78.66644367742109978, 23.39876645725288284, 3.573650549209446137 ) ) ;
#47410=B_SPLINE_CURVE_WITH_KNOTS ( 'NONE', 3,
 ( #40619, #60692, #12868, #23425, #45206, #39249, #39590, #7928, #23763, #34323, #1602, #65992, #18137, #55408, #61042, #35008, #33968, #29726, #40285, #35355, #2312, #51190, #62071, #39932, #17793, #13892, #50835, #12510, #66349, #61390, #1968, #7234, #8632, #55771, #45907, #7593, #61728, #67375, #28691, #50144, #29381, #56452, #13554, #19165, #23066 ),
 .UNSPECIFIED., .F., .F.,
 ( 4, 2, 2, 2, 2, 2, 2, 2, 2, 2, 2, 1, 2, 2, 2, 2, 2, 2, 2, 2, 2, 2, 4 ),
 ( 1.430489624538199204E-17, 0.001502898956853382460, 0.002254348435280062631, 0.003005797913706743235, 0.004508696870560142608, 0.005260146348986859642, 0.006011595827413576676, 0.007514494784267024621, 0.009017393741120474301, 0.01052029269797392051, 0.01127174217640065229, 0.01202319165482738407, 0.01277464113325411238, 0.01352609061168084242, 0.01502898956853430251, 0.01578043904696103256, 0.01653188852538776260, 0.01803478748224122269, 0.01953768643909467931, 0.02028913591752141629, 0.02104058539594814981, 0.02254348435280158561, 0.02404638330965502488 ),
 .UNSPECIFIED. ) ;
#47411=CARTESIAN_POINT ( 'NONE',  ( -1.314022807222071432, 6.554273999800675377, -12.31960447689811389 ) ) ;
#47412=CARTESIAN_POINT ( 'NONE',  ( 198.7129816317745963, 100.1061386900356069, -12.45321170628048080 ) ) ;
#47414=CARTESIAN_POINT ( 'NONE',  ( -152.9869010856123452, 67.18780492383567093, 85.26019206469960920 ) ) ;
#47415=CARTESIAN_POINT ( 'NONE',  ( 22.25657943806483274, 6.793941046373902282, 94.99999999999866418 ) ) ;
#47419=CARTESIAN_POINT ( 'NONE',  ( 185.7267155939802024, 84.90388481853123892, 30.91358943140728499 ) ) ;
#47420=CARTESIAN_POINT ( 'NONE',  ( 154.4617654203035499, 56.60942201271839025, 30.02488550039760895 ) ) ;
#47426=CARTESIAN_POINT ( 'NONE',  ( -73.81689110552359523, 20.53332132481500594, -21.49728268473057113 ) ) ;
#47428=CARTESIAN_POINT ( 'NONE',  ( -61.75956139478098095, 16.58288496614412466, 34.45118629696971624 ) ) ;
#47429=B_SPLINE_CURVE_WITH_KNOTS ( 'NONE', 3,
 ( #61302, #29631, #34593, #50405, #44781, #45115, #29986, #33882, #23337, #66258, #24372, #56720, #23671, #55320, #2222, #66945, #18048, #7141, #39504, #18738, #61982, #45816, #2563, #56364, #3259, #56029, #12772, #60951, #67295, #24719, #34234, #13126, #46152, #40531, #13800, #61646, #55675, #7841, #35261, #19079 ),
 .UNSPECIFIED., .F., .F.,
 ( 4, 2, 2, 2, 2, 2, 2, 2, 2, 2, 2, 2, 2, 2, 2, 2, 2, 2, 2, 4 ),
 ( 0.02454308262169000582, 0.02608670964102882336, 0.02685852315069824775, 0.02763033666036767214, 0.02917396367970651744, 0.02994577718937594529, 0.03071759069904536968, 0.03226121771838418029, 0.03303303122805360120, 0.03380484473772302212, 0.03534847175706185701, 0.03689209877640069885, 0.03843572579573954068, 0.03997935281507837557, 0.04152297983441721740, 0.04306660685375605924, 0.04461023387309490107, 0.04615386089243374290, 0.04769748791177259167, 0.04924111493111144044 ),
 .UNSPECIFIED. ) ;
#47432=CARTESIAN_POINT ( 'NONE',  ( -176.3896317155480062, 90.84057090619019448, 31.55718514125764074 ) ) ;
#47434=CARTESIAN_POINT ( 'NONE',  ( 116.8917656767876565, 33.20682060519246903, -39.94289992015058743 ) ) ;
#47438=CARTESIAN_POINT ( 'NONE',  ( 141.0645618855930934, 45.95036951196541963, 61.71528580804383068 ) ) ;
#47439=DIRECTION ( 'NONE',  ( 0.000000000000000000, 0.000000000000000000, 1.000000000000000000 ) ) ;
#47445=AXIS2_PLACEMENT_3D ( 'NONE', #62678, #14483, #59447 ) ;
#47446=CARTESIAN_POINT ( 'NONE',  ( 156.5993887774280324, 58.24868799840903932, -24.23210818043918025 ) ) ;
#47449=CARTESIAN_POINT ( 'NONE',  ( 110.2429982417149574, 29.99119854320843714, 44.61121420573733332 ) ) ;
#47451=CARTESIAN_POINT ( 'NONE',  ( -149.5074843970971301, 64.17983161892345834, -76.65738112195568021 ) ) ;
#47452=CARTESIAN_POINT ( 'NONE',  ( 69.70008851143845163, 14.32304089804287806, 94.41978594955163828 ) ) ;
#47453=CARTESIAN_POINT ( 'NONE',  ( 183.1873354889582686, 82.20882912211249050, 2.752098851290597725 ) ) ;
#47458=ORIENTED_EDGE ( 'NONE', *, *, #21899, .T. ) ;
#47459=CYLINDRICAL_SURFACE ( 'NONE', #17228, 7.500000000000020428 ) ;
#47462=CYLINDRICAL_SURFACE ( 'NONE', #45304, 7.500000000000013323 ) ;
#47463=CARTESIAN_POINT ( 'NONE',  ( 59.72526569420001152, 11.93313563009889222, -63.30790693026741422 ) ) ;
#47467=CARTESIAN_POINT ( 'NONE',  ( -1.515478260543418498, 6.562165592639543021, 87.23764935852220503 ) ) ;
#47470=ORIENTED_EDGE ( 'NONE', *, *, #19439, .T. ) ;
#47474=ORIENTED_EDGE ( 'NONE', *, *, #45926, .F. ) ;
#47475=CARTESIAN_POINT ( 'NONE',  ( -30.46358361599563480, 10.45190018822943756, -62.20962308564316601 ) ) ;
#47476=CARTESIAN_POINT ( 'NONE',  ( 59.72526569420001863, 11.93313563009889222, -36.46335633980373814 ) ) ;
#47480=EDGE_CURVE ( 'NONE', #51871, #53693, #46895, .T. ) ;
#47482=CARTESIAN_POINT ( 'NONE',  ( -125.8938041572051105, 47.69968343338781835, 45.61994787315711619 ) ) ;
#47484=CARTESIAN_POINT ( 'NONE',  ( 211.8476521439973794, 116.6941316755176956, 12.15074821135860894 ) ) ;
#47492=CARTESIAN_POINT ( 'NONE',  ( -133.2885345616805068, 52.79649921787450495, 90.38452661033592506 ) ) ;
#47494=CARTESIAN_POINT ( 'NONE',  ( 38.42095780754792145, 9.297684251045549075, -62.51249201856361282 ) ) ;
#47496=CARTESIAN_POINT ( 'NONE',  ( 65.41496713438829147, 13.24164235279043922, 44.43526210712943936 ) ) ;
#47497=CARTESIAN_POINT ( 'NONE',  ( 13.20823635526162931, 7.437507787974027451, 84.13046171212820923 ) ) ;
#47499=EDGE_LOOP ( 'NONE', ( #59102, #67882, #23661, #13261 ) ) ;
#47504=CARTESIAN_POINT ( 'NONE',  ( -85.91089317961400695, 25.21459833389208072, 9.066374898930352089 ) ) ;
#47509=CARTESIAN_POINT ( 'NONE',  ( -118.4106078162223383, 42.93830006159886636, 11.84514837596003822 ) ) ;
#47510=CARTESIAN_POINT ( 'NONE',  ( -180.3158531669106424, 95.51092859788506928, 63.02641839755398934 ) ) ;
#47511=CARTESIAN_POINT ( 'NONE',  ( 132.9485794245231887, 40.87843215479638559, 71.31345729829673985 ) ) ;
#47514=CARTESIAN_POINT ( 'NONE',  ( -35.41676323786686709, 10.27805710077606172, 85.03917892935545808 ) ) ;
#47515=CARTESIAN_POINT ( 'NONE',  ( 153.8366942494330658, 54.87992279068315327, 43.47454990642605566 ) ) ;
#47517=B_SPLINE_CURVE_WITH_KNOTS ( 'NONE', 3,
 ( #66902, #29249, #19034, #23969, #66554, #14106, #34544, #51053, #56672, #8842, #46108, #24674, #40487, #45421, #29941, #18697, #51406, #67579, #39453, #34191, #2863, #35215, #2518, #13757, #45069, #24331, #67251, #3218, #35567, #61259, #30292, #19378, #40152, #40835, #7455, #28911, #2176, #18340, #50360, #13080 ),
 .UNSPECIFIED., .F., .F.,
 ( 4, 2, 2, 2, 2, 2, 2, 2, 2, 2, 2, 2, 2, 2, 2, 2, 2, 2, 2, 4 ),
 ( 0.02472759712254455136, 0.02626001169882808198, 0.02779242627511161259, 0.02932484085139513974, 0.03009104813953688423, 0.03085725542767862525, 0.03238967000396209689, 0.03315587729210384138, 0.03392208458024558587, 0.03545449915652906098, 0.03698691373281253608, 0.03851932830909601813, 0.04005174288537949323, 0.04158415746166296834, 0.04311657203794644344, 0.04464898661422991855, 0.04541519390237165610, 0.04618140119051339365, 0.04771381576679689651, 0.04924623034308039243 ),
 .UNSPECIFIED. ) ;
#47518=CARTESIAN_POINT ( 'NONE',  ( 102.7425154123292828, 25.56407025871219574, -43.66414440344461667 ) ) ;
#47520=CARTESIAN_POINT ( 'NONE',  ( -142.3260422482981085, 59.60034523324940636, -66.92270134455016262 ) ) ;
#47523=CARTESIAN_POINT ( 'NONE',  ( -86.15466590221105037, 26.40813842494318209, -68.96785203774670947 ) ) ;
#47524=CARTESIAN_POINT ( 'NONE',  ( 174.9099402067543565, 73.96774984027643995, 14.23027204521179279 ) ) ;
#47526=CARTESIAN_POINT ( 'NONE',  ( -80.32755469740936860, 24.04130076192507204, 18.39130622474332100 ) ) ;
#47528=CARTESIAN_POINT ( 'NONE',  ( 37.76166711006369070, 8.201557253608928733, -89.47894714693738649 ) ) ;
#47531=CARTESIAN_POINT ( 'NONE',  ( 70.11766033381772445, 14.43277633974326690, 8.007630405225276249 ) ) ;
#47532=CARTESIAN_POINT ( 'NONE',  ( 158.3595886390531575, 58.34525996025799799, 2.604644620584485093 ) ) ;
#47534=ORIENTED_EDGE ( 'NONE', *, *, #32799, .T. ) ;
#47540=VERTEX_POINT ( 'NONE', #25712 ) ;
#47541=CARTESIAN_POINT ( 'NONE',  ( 21.43750346857337874, 7.754771113113079650, -64.90611682194166576 ) ) ;
#47546=CARTESIAN_POINT ( 'NONE',  ( 65.62848231372475993, 13.29388722724788963, -23.41044504611049248 ) ) ;
#47547=DIRECTION ( 'NONE',  ( 0.000000000000000000, -0.000000000000000000, -1.000000000000000000 ) ) ;
#47548=CARTESIAN_POINT ( 'NONE',  ( 33.76124497394583557, 7.742545529019357886, -38.15270983885158529 ) ) ;
#47550=CARTESIAN_POINT ( 'NONE',  ( -48.41612563322100016, -170.0000000000000000, 94.99999999999866418 ) ) ;
#47564=CARTESIAN_POINT ( 'NONE',  ( 63.01563776193090405, 13.70579113808096672, -89.40979201309708913 ) ) ;
#47566=CARTESIAN_POINT ( 'NONE',  ( 182.7745872728868051, 81.77554423487161728, -9.523131544683039351 ) ) ;
#47567=CARTESIAN_POINT ( 'NONE',  ( 181.0840389613909736, 78.60582251573003987, -78.06960825634331513 ) ) ;
#47569=CARTESIAN_POINT ( 'NONE',  ( 88.53517449242357884, 20.08005703101044759, -9.219238925436826548 ) ) ;
#47572=CARTESIAN_POINT ( 'NONE',  ( 163.7379901688713630, 64.00402364591251114, 67.88120199201151195 ) ) ;
#47577=CARTESIAN_POINT ( 'NONE',  ( 133.8566784816069344, -170.0000000000000000, 56.35489142945903751 ) ) ;
#47579=CARTESIAN_POINT ( 'NONE',  ( 149.9838583332408462, 52.05699766415860097, 9.536419267673462485 ) ) ;
#47583=DIRECTION ( 'NONE',  ( -0.000000000000000000, 1.000000000000000000, -0.000000000000000000 ) ) ;
#47587=CARTESIAN_POINT ( 'NONE',  ( 31.97180862241589949, 8.570158524060584426, 89.88509897528000181 ) ) ;
#47591=CYLINDRICAL_SURFACE ( 'NONE', #30055, 7.500000000000020428 ) ;
#47592=CARTESIAN_POINT ( 'NONE',  ( -102.2801239173131052, 33.91021738430207222, 72.36362509687883460 ) ) ;
#47594=CARTESIAN_POINT ( 'NONE',  ( -0.7076388175553621762, 7.538734751903869657, 8.356667854065962686 ) ) ;
#47595=CARTESIAN_POINT ( 'NONE',  ( 173.6024011093111028, 72.73634049052009232, -44.32818560226256466 ) ) ;
#47596=CARTESIAN_POINT ( 'NONE',  ( -154.7826623253030220, 70.14150242829521176, -74.49430738417227360 ) ) ;
#47603=CARTESIAN_POINT ( 'NONE',  ( 106.6322547488295385, 28.34756922280617530, -23.16909260820694882 ) ) ;
#47607=CYLINDRICAL_SURFACE ( 'NONE', #12737, 7.500000000000013323 ) ;
#47615=CARTESIAN_POINT ( 'NONE',  ( 117.3145357257065484, 33.41973663092564095, -67.71684323464012323 ) ) ;
#47617=CARTESIAN_POINT ( 'NONE',  ( 199.3671895066314619, 99.30947926630331324, -75.97069292755713832 ) ) ;
#47621=CARTESIAN_POINT ( 'NONE',  ( -15.13464256769236016, 8.488509377255644139, -14.37503968884516858 ) ) ;
#47622=CARTESIAN_POINT ( 'NONE',  ( 153.4268936273268764, 54.57409659828384463, -76.78973794846126566 ) ) ;
#47628=CARTESIAN_POINT ( 'NONE',  ( 70.46579300139245561, 15.56614468937218909, -15.37766843719409593 ) ) ;
#47629=CARTESIAN_POINT ( 'NONE',  ( -81.23268307104841313, 24.39742801172156916, -49.66676133314191333 ) ) ;
#47630=CARTESIAN_POINT ( 'NONE',  ( 102.7985695539029791, 25.58774450393820388, 91.77657224901672350 ) ) ;
#47631=ADVANCED_FACE ( 'NONE', ( #4924 ), #37270, .T. ) ;
#47632=CARTESIAN_POINT ( 'NONE',  ( -152.9008427825211243, 68.45483453645057637, 4.684046598983249154 ) ) ;
#47635=CARTESIAN_POINT ( 'NONE',  ( 22.89234820949993576, 6.832052815347870123, 35.09748061321546686 ) ) ;
#47636=CARTESIAN_POINT ( 'NONE',  ( -189.4202820252412494, 108.5506294086428625, -93.67079659341260367 ) ) ;
#47637=ORIENTED_EDGE ( 'NONE', *, *, #12559, .F. ) ;
#47641=CARTESIAN_POINT ( 'NONE',  ( 91.73702110022665579, 22.29915270480343992, -91.50358301110458115 ) ) ;
#47642=CARTESIAN_POINT ( 'NONE',  ( 108.3281565346183015, 28.00578413698477931, -89.84965755605794868 ) ) ;
#47644=VECTOR ( 'NONE', #7008, 1000.000000000000000 ) ;
#47645=CARTESIAN_POINT ( 'NONE',  ( -36.89224332184166144, 11.57404295377976311, -74.81660943836889999 ) ) ;
#47647=CARTESIAN_POINT ( 'NONE',  ( 202.7540649946183464, 105.3989460363904840, 56.29713274085410291 ) ) ;
#47651=AXIS2_PLACEMENT_3D ( 'NONE', #10588, #5327, #26783 ) ;
#47652=CARTESIAN_POINT ( 'NONE',  ( 34.45817031441433897, 7.817703378455679086, 58.59672298083805231 ) ) ;
#47653=CARTESIAN_POINT ( 'NONE',  ( 9.058156535714475766, 6.378495712187264743, -19.49345657520668240 ) ) ;
#47654=CARTESIAN_POINT ( 'NONE',  ( 18.88468164817599160, 7.626722602998420086, 3.834753717211726087 ) ) ;
#47655=CARTESIAN_POINT ( 'NONE',  ( 187.9007786055418308, 85.78077355327278042, 66.79259192409129753 ) ) ;
#47657=CARTESIAN_POINT ( 'NONE',  ( -86.06016868996611890, 25.27707703029502184, -41.33193578213184338 ) ) ;
#47660=CARTESIAN_POINT ( 'NONE',  ( 12.91653430408660519, 7.431946598423013306, 3.728854190381519551 ) ) ;
#47661=AXIS2_PLACEMENT_3D ( 'NONE', #15608, #36725, #38349 ) ;
#47663=CARTESIAN_POINT ( 'NONE',  ( 181.0840389613909736, 78.60582251573002566, 17.46404351504774510 ) ) ;
#47665=CARTESIAN_POINT ( 'NONE',  ( 177.5945652320814361, 75.14951358071817822, 43.45125508251556568 ) ) ;
#47667=CARTESIAN_POINT ( 'NONE',  ( -104.1393288135078024, 34.86912007524090029, -35.23351094377062509 ) ) ;
#47668=DIRECTION ( 'NONE',  ( 0.000000000000000000, -1.000000000000000000, 0.000000000000000000 ) ) ;
#47669=VERTEX_POINT ( 'NONE', #33666 ) ;
#47671=CARTESIAN_POINT ( 'NONE',  ( -24.07146903340143851, 8.497560047608724076, -14.50675576945464051 ) ) ;
#47672=CARTESIAN_POINT ( 'NONE',  ( 174.1712199980251796, 71.89075529249559793, 87.58217343572140123 ) ) ;
#47673=ORIENTED_EDGE ( 'NONE', *, *, #52779, .T. ) ;
#47674=CARTESIAN_POINT ( 'NONE',  ( 111.1868021579656869, 29.32055685204858619, 71.41117935951764650 ) ) ;
#47676=CARTESIAN_POINT ( 'NONE',  ( 113.8626313173126050, 31.71036178495293711, 70.54171001663286233 ) ) ;
#47677=CARTESIAN_POINT ( 'NONE',  ( 133.8566784816069344, 41.42467568809808398, 29.51034083899533300 ) ) ;
#47686=CARTESIAN_POINT ( 'NONE',  ( -119.2982054035570911, 42.30181775808004829, -19.14876710156486794 ) ) ;
#47690=CARTESIAN_POINT ( 'NONE',  ( -180.2244609727085276, 95.39945930389644957, -17.79149012421619247 ) ) ;
#47691=CARTESIAN_POINT ( 'NONE',  ( 133.8566784816069060, 41.42467568809810530, 56.35489142945903751 ) ) ;
#47697=CARTESIAN_POINT ( 'NONE',  ( -61.51762070241279190, 16.51067482779403761, -12.06156012046973736 ) ) ;
#47700=EDGE_CURVE ( 'NONE', #12944, #66081, #9971, .T. ) ;
#47704=CARTESIAN_POINT ( 'NONE',  ( 59.86221654654867308, 11.96331997874669284, -90.10186521222453848 ) ) ;
#47706=CARTESIAN_POINT ( 'NONE',  ( -95.88718821240200896, 29.65015105908827309, 7.244506905266613117 ) ) ;
#47707=CARTESIAN_POINT ( 'NONE',  ( -97.85576954355164503, 30.58918648956191788, -63.28394810425090355 ) ) ;
#47711=CARTESIAN_POINT ( 'NONE',  ( 184.3994103300443044, 82.02159554764423888, -63.82720643750994327 ) ) ;
#47713=FACE_OUTER_BOUND ( 'NONE', #46663, .T. ) ;
#47714=EDGE_CURVE ( 'NONE', #37653, #805, #32558, .T. ) ;
#47715=CARTESIAN_POINT ( 'NONE',  ( 105.7953515382195917, 27.97683113100023178, -64.20869765785622008 ) ) ;
#47716=CARTESIAN_POINT ( 'NONE',  ( -71.26746920569853216, 20.70422440535243069, 36.66531925523995028 ) ) ;
#47717=CARTESIAN_POINT ( 'NONE',  ( -74.20136529587824725, 21.74007521413448885, -63.42900937661281802 ) ) ;
#47718=CARTESIAN_POINT ( 'NONE',  ( 67.55199883153194662, 14.80832170058782182, -49.21298022547202322 ) ) ;
#47719=CARTESIAN_POINT ( 'NONE',  ( -125.6703656163501392, 47.55170550253210848, 30.61994787315705935 ) ) ;
#47720=CARTESIAN_POINT ( 'NONE',  ( 212.1962110267000128, 117.2292732107321456, 63.17560925674016659 ) ) ;
#47724=CARTESIAN_POINT ( 'NONE',  ( -32.41982179707237322, 9.753975577087190985, 3.420357701285721141 ) ) ;
#47725=CARTESIAN_POINT ( 'NONE',  ( -149.5074843970971301, -170.0000000000000000, 38.22082123989905966 ) ) ;
#47726=CARTESIAN_POINT ( 'NONE',  ( 93.87650740736111743, 23.09802612281733758, 62.06025712787139526 ) ) ;
#47727=CARTESIAN_POINT ( 'NONE',  ( 150.4550062612853480, 52.39582885725847206, -14.07485114950216065 ) ) ;
#47730=CARTESIAN_POINT ( 'NONE',  ( 36.31593203568480988, 8.028139509847028066, -76.80444249456844830 ) ) ;
#47731=CARTESIAN_POINT ( 'NONE',  ( 63.01563776193091826, -170.0000000000000000, 56.65751152968497451 ) ) ;
#47732=CARTESIAN_POINT ( 'NONE',  ( -32.40928421737412890, 10.77259363352673560, -23.42573354065221025 ) ) ;
#47735=CARTESIAN_POINT ( 'NONE',  ( -125.0779128240347973, 47.16111191621167364, -88.63580480530789885 ) ) ;
#47738=CARTESIAN_POINT ( 'NONE',  ( 15.78827728214693416, 7.507518794609589818, -77.36349468914950478 ) ) ;
#47739=CARTESIAN_POINT ( 'NONE',  ( -189.9638655956220248, 108.0957249433520815, 8.346787301602333287 ) ) ;
#47742=CARTESIAN_POINT ( 'NONE',  ( -1.728570918131773881, 6.570609986804655023, 33.24078084807834443 ) ) ;
#47744=CARTESIAN_POINT ( 'NONE',  ( 157.4703587214989113, 58.92748579479261650, -51.12418429913766005 ) ) ;
#47749=CARTESIAN_POINT ( 'NONE',  ( -189.8071159312683847, 107.8771087123620021, -18.14639082933156189 ) ) ;
#47751=CARTESIAN_POINT ( 'NONE',  ( -102.2801239173131052, 33.91021738430207222, 57.36362509687880618 ) ) ;
#47754=VERTEX_POINT ( 'NONE', #25877 ) ;
#47756=CARTESIAN_POINT ( 'NONE',  ( 133.8566784816069344, -170.0000000000000000, -89.71241211332301191 ) ) ;
#47759=CARTESIAN_POINT ( 'NONE',  ( 94.06703982324148683, 22.09435144471461498, 65.05402493561722110 ) ) ;
#47760=B_SPLINE_CURVE_WITH_KNOTS ( 'NONE', 3,
 ( #44021, #781, #28559, #44741, #27854, #44376, #60212, #49645, #54928, #49297, #7805, #2184, #1130, #11672, #66220, #29256, #50003, #18007, #43673, #22233, #60908, #22581, #65863, #23636, #1473, #12730, #45074, #66558, #17660, #17298, #55280, #18347, #6749, #39809, #14110, #50705, #8144, #40157, #67255, #46457 ),
 .UNSPECIFIED., .F., .F.,
 ( 4, 2, 2, 2, 2, 2, 2, 2, 2, 2, 2, 2, 2, 2, 2, 2, 2, 2, 2, 4 ),
 ( 0.02472759712254455136, 0.02626001169882808198, 0.02779242627511160912, 0.02932484085139513974, 0.03009104813953688423, 0.03085725542767862872, 0.03238967000396208301, 0.03315587729210382750, 0.03392208458024557199, 0.03545449915652905404, 0.03698691373281252914, 0.03851932830909600425, 0.04005174288537947935, 0.04158415746166295446, 0.04311657203794642956, 0.04464898661422990467, 0.04541519390237164222, 0.04618140119051337977, 0.04771381576679689651, 0.04924623034308040631 ),
 .UNSPECIFIED. ) ;
#47762=CARTESIAN_POINT ( 'NONE',  ( 203.9203998321607685, 106.9845510704142129, -9.511358609132138042 ) ) ;
#47770=CARTESIAN_POINT ( 'NONE',  ( 161.7031777507227446, 62.31724004902784486, 16.27331598182586703 ) ) ;
#47771=CARTESIAN_POINT ( 'NONE',  ( -99.10904156412040322, 32.31949011661294691, 44.83230361419195731 ) ) ;
#47773=CARTESIAN_POINT ( 'NONE',  ( 174.2538192999569731, 73.34752463892027663, 60.54307137167467090 ) ) ;
#47774=ORIENTED_EDGE ( 'NONE', *, *, #40424, .F. ) ;
#47776=EDGE_CURVE ( 'NONE', #59523, #33643, #12380, .T. ) ;
#47777=CARTESIAN_POINT ( 'NONE',  ( 67.92995549349549833, 13.86623459444476225, -75.75181126496241291 ) ) ;
#47778=CARTESIAN_POINT ( 'NONE',  ( -59.56523643198714524, 15.93788386494078502, 43.81298497852716167 ) ) ;
#47779=B_SPLINE_CURVE_WITH_KNOTS ( 'NONE', 3,
 ( #49934, #7390, #34124, #24266, #55924, #13699, #13020, #62224, #44674, #35504, #2455, #35151, #50631, #45712, #14045, #56606, #50989, #18283, #7737, #8073, #51343, #66149, #56965, #34481, #34819, #24614, #8430, #66842, #46048, #29189, #40088, #2804, #23909, #61871, #18630, #29881, #3158, #13362, #67189, #8785, #61543, #56256, #29522 ),
 .UNSPECIFIED., .F., .F.,
 ( 4, 2, 2, 2, 2, 2, 2, 2, 2, 2, 2, 2, 1, 2, 2, 2, 2, 2, 2, 2, 2, 4 ),
 ( 0.02371951416048009159, 0.02520633211177543409, 0.02594974108742308799, 0.02669315006307074190, 0.02817996801436604623, 0.02966678596566135057, 0.03041019494130899753, 0.03115360391695664102, 0.03264042186825193148, 0.03412723981954722541, 0.03561405777084253321, 0.03635746674649016630, 0.03710087572213779938, 0.03784428469778543941, 0.03858769367343307249, 0.04007451162472835948, 0.04156132957602363953, 0.04304814752731893346, 0.04379155650296658042, 0.04453496547861424126, 0.04602178342990954213, 0.04750860138120484993 ),
 .UNSPECIFIED. ) ;
#47780=CARTESIAN_POINT ( 'NONE',  ( 157.0316110297314083, 58.58403635656379294, 17.56491688178972055 ) ) ;
#47781=VERTEX_POINT ( 'NONE', #54662 ) ;
#47782=CARTESIAN_POINT ( 'NONE',  ( 157.4703587214989113, 58.92748579479261650, -51.12418429913766005 ) ) ;
#47784=CARTESIAN_POINT ( 'NONE',  ( 111.1829448509513014, 30.43012797723691065, -35.96691630598188993 ) ) ;
#47789=CARTESIAN_POINT ( 'NONE',  ( 141.3707934840545022, 46.15056991286794386, 63.82522392161691016 ) ) ;
#47790=CARTESIAN_POINT ( 'NONE',  ( -175.1895962157337010, 90.99110972060688596, 31.10022776195569705 ) ) ;
#47791=CARTESIAN_POINT ( 'NONE',  ( -36.37371824399145481, 10.45334302951138561, -75.33134930568731136 ) ) ;
#47793=CARTESIAN_POINT ( 'NONE',  ( 188.2076037774874919, 86.11782719225436722, -19.24392630350066469 ) ) ;
#47795=CARTESIAN_POINT ( 'NONE',  ( 45.76553115525427273, 10.34124506813254918, 6.592493761944549391 ) ) ;
#47797=ORIENTED_EDGE ( 'NONE', *, *, #36619, .T. ) ;
#47801=CARTESIAN_POINT ( 'NONE',  ( 207.4566510040494904, 111.9649643341356438, -23.95860942766702806 ) ) ;
#47803=AXIS2_PLACEMENT_3D ( 'NONE', #55376, #7564, #34650 ) ;
#47806=CARTESIAN_POINT ( 'NONE',  ( -109.7047744410585608, 36.71529196001675643, 92.81931154901670311 ) ) ;
#47812=CARTESIAN_POINT ( 'NONE',  ( -97.90661117598844498, 31.73207306186866816, -90.10694785018394271 ) ) ;
#47814=CARTESIAN_POINT ( 'NONE',  ( -76.78104518372333587, 22.68568622761703324, 57.48804312598085176 ) ) ;
#47816=CARTESIAN_POINT ( 'NONE',  ( 61.09275639403233527, 12.23448398202909893, -77.33071701894527905 ) ) ;
#47817=CARTESIAN_POINT ( 'NONE',  ( -78.66644367742109978, 22.32174330031319442, 3.573650549209446137 ) ) ;
#47819=CARTESIAN_POINT ( 'NONE',  ( 86.62931800182293784, 19.42108912189599579, 71.55663816294304524 ) ) ;
#47820=CARTESIAN_POINT ( 'NONE',  ( 164.9700808964341547, 65.04346068891115351, -70.17999518051283303 ) ) ;
#47821=VERTEX_POINT ( 'NONE', #42725 ) ;
#47822=CARTESIAN_POINT ( 'NONE',  ( -71.22878586122430988, 19.62649588091169406, 65.76083851737067221 ) ) ;
#47825=EDGE_CURVE ( 'NONE', #6663, #11578, #38139, .T. ) ;
#47828=CARTESIAN_POINT ( 'NONE',  ( 61.10129719786244351, 12.23677173834305165, -35.96503823067305206 ) ) ;
#47832=ORIENTED_EDGE ( 'NONE', *, *, #63330, .T. ) ;
#47834=CARTESIAN_POINT ( 'NONE',  ( -131.2955621888335429, 51.38237199780174080, 32.89462560528686907 ) ) ;
#47836=CARTESIAN_POINT ( 'NONE',  ( 37.46876540261052924, 9.179568636624027889, -23.52597108042403207 ) ) ;
#47837=CARTESIAN_POINT ( 'NONE',  ( 188.1848725084043110, 87.59259440284084519, -95.00000000000133582 ) ) ;
#47838=CARTESIAN_POINT ( 'NONE',  ( 207.4867844023104624, 110.2451255333963616, 43.68190180099020381 ) ) ;
#47842=VERTEX_POINT ( 'NONE', #33232 ) ;
#47844=CARTESIAN_POINT ( 'NONE',  ( 159.6593397521790223, 59.37286298965126718, -23.96695613349937304 ) ) ;
#47846=AXIS2_PLACEMENT_3D ( 'NONE', #61507, #39703, #44972 ) ;
#47847=CARTESIAN_POINT ( 'NONE',  ( -165.9122696334864600, 79.44688201528256855, -17.45773735543971128 ) ) ;
#47849=DIRECTION ( 'NONE',  ( 0.000000000000000000, 0.000000000000000000, 1.000000000000000000 ) ) ;
#47850=CARTESIAN_POINT ( 'NONE',  ( -190.3074740493607351, 108.5764897054613414, -72.83801848297902382 ) ) ;
#47855=CARTESIAN_POINT ( 'NONE',  ( -125.8938041572051389, -170.0000000000000000, 72.46449846362081360 ) ) ;
#47856=AXIS2_PLACEMENT_3D ( 'NONE', #40200, #29633, #67629 ) ;
#47857=CARTESIAN_POINT ( 'NONE',  ( -99.10260179032840711, 31.19580119595417855, 71.66143382347762270 ) ) ;
#47860=CARTESIAN_POINT ( 'NONE',  ( -173.1211646369891355, -170.0000000000000000, -15.36740657428631351 ) ) ;
#47866=CARTESIAN_POINT ( 'NONE',  ( -120.5002574492098972, 44.22930148497321312, 16.49287155969762253 ) ) ;
#47867=CARTESIAN_POINT ( 'NONE',  ( -180.3153482337535536, 95.51031295027647161, 67.30752748117252793 ) ) ;
#47868=CARTESIAN_POINT ( 'NONE',  ( 128.0568017572569204, 38.03085713813912605, 59.07289773574036218 ) ) ;
#47869=VERTEX_POINT ( 'NONE', #21962 ) ;
#47871=DIRECTION ( 'NONE',  ( -0.000000000000000000, 1.000000000000000000, -0.000000000000000000 ) ) ;
#47874=CARTESIAN_POINT ( 'NONE',  ( -102.2801239173131052, 33.91021738430207932, 30.51907450641510522 ) ) ;
#47875=CARTESIAN_POINT ( 'NONE',  ( -31.43908319763710679, 9.591432048623758533, 45.21645440618919309 ) ) ;
#47877=EDGE_CURVE ( 'NONE', #56862, #1104, #7546, .T. ) ;
#47878=ORIENTED_EDGE ( 'NONE', *, *, #59156, .F. ) ;
#47879=FACE_BOUND ( 'NONE', #21423, .T. ) ;
#47882=CARTESIAN_POINT ( 'NONE',  ( 117.3188760168912523, 32.29536350891957142, -94.58846656126689822 ) ) ;
#47883=CARTESIAN_POINT ( 'NONE',  ( -119.1605144823340510, 43.39823405392971267, -45.72746398012520785 ) ) ;
#47886=CARTESIAN_POINT ( 'NONE',  ( -154.2585856850055279, 68.31650218414623055, 5.568140700381407626 ) ) ;
#47887=CARTESIAN_POINT ( 'NONE',  ( -118.5151419614604720, 43.00218563933586324, -67.88871905889871528 ) ) ;
#47889=CARTESIAN_POINT ( 'NONE',  ( -81.24432217070638274, 24.40203426192927338, 71.80983157096119385 ) ) ;
#47890=CARTESIAN_POINT ( 'NONE',  ( 90.51709546286271291, 21.85407654229979357, -22.89523223895175974 ) ) ;
#47892=AXIS2_PLACEMENT_3D ( 'NONE', #31222, #21002, #11127 ) ;
#47896=CARTESIAN_POINT ( 'NONE',  ( -196.7348448768811409, -170.0000000000000000, -42.11108379800802481 ) ) ;
#47902=CARTESIAN_POINT ( 'NONE',  ( -51.13576748034041941, 14.70354244225167584, -75.96136548085722495 ) ) ;
#47905=CARTESIAN_POINT ( 'NONE',  ( -122.8202784017355356, 45.69728649588467562, -8.723847309115170034 ) ) ;
#47906=ORIENTED_EDGE ( 'NONE', *, *, #70, .T. ) ;
#47908=CARTESIAN_POINT ( 'NONE',  ( 69.08240197259638649, 14.16210831900843381, -47.63718284325325669 ) ) ;
#47909=CARTESIAN_POINT ( 'NONE',  ( 173.7502847382833693, 72.87471067097989419, 92.08090874032060924 ) ) ;
#47915=CARTESIAN_POINT ( 'NONE',  ( -15.26524495591509201, 7.490231452641286758, 63.48037225783858872 ) ) ;
#47916=CARTESIAN_POINT ( 'NONE',  ( -83.12901536265222546, 24.07178615860086524, -9.738105063539622464 ) ) ;
#47919=CARTESIAN_POINT ( 'NONE',  ( -55.05276343752910151, -170.0000000000000000, -42.71632399845987749 ) ) ;
#47921=CARTESIAN_POINT ( 'NONE',  ( 164.4760519199596160, 64.62478832434433684, 66.48423307707000163 ) ) ;
#47922=ORIENTED_EDGE ( 'NONE', *, *, #54705, .F. ) ;
#47924=CARTESIAN_POINT ( 'NONE',  ( 89.88147981065576175, 21.62466191578946351, -36.54612782466419674 ) ) ;
#47925=CARTESIAN_POINT ( 'NONE',  ( 152.1153500913667642, 54.85403770686895086, 69.01100629273766174 ) ) ;
#47927=CARTESIAN_POINT ( 'NONE',  ( 150.2076397309211870, 52.21780102759854003, 8.173336009946826408 ) ) ;
#47928=CARTESIAN_POINT ( 'NONE',  ( -14.97009123890826032, 8.472783959029182910, 89.00005877110403674 ) ) ;
#47930=CARTESIAN_POINT ( 'NONE',  ( -56.72814287166057312, 15.13700122306437557, 71.97630986414527854 ) ) ;
#47932=ORIENTED_EDGE ( 'NONE', *, *, #26828, .T. ) ;
#47935=CARTESIAN_POINT ( 'NONE',  ( 46.77033063468804386, 10.50186244217540654, 92.54074439162803856 ) ) ;
#47937=EDGE_CURVE ( 'NONE', #16719, #18334, #4038, .T. ) ;
#47938=CARTESIAN_POINT ( 'NONE',  ( 139.6272612117789720, 46.21653985347571592, -92.40408479050303470 ) ) ;
#47941=CARTESIAN_POINT ( 'NONE',  ( -58.10608953386397957, 15.52134062643865242, -76.41550596808153273 ) ) ;
#47944=CARTESIAN_POINT ( 'NONE',  ( -7.825402957745081878, 7.899365992529268965, 3.271030448983517580 ) ) ;
#47945=DIRECTION ( 'NONE',  ( 0.000000000000000000, 0.000000000000000000, 1.000000000000000000 ) ) ;
#47947=CARTESIAN_POINT ( 'NONE',  ( 164.4953970817402933, 63.32598771815145255, 87.94741031797519781 ) ) ;
#47948=CARTESIAN_POINT ( 'NONE',  ( 87.10668362745096260, 19.58396519288863757, 29.71208757247931231 ) ) ;
#47950=EDGE_LOOP ( 'NONE', ( #62150, #68428, #23888, #63467 ) ) ;
#47954=CARTESIAN_POINT ( 'NONE',  ( -28.13527276074848871, 10.08983026464525068, 30.97886788483921805 ) ) ;
#47956=CARTESIAN_POINT ( 'NONE',  ( 197.1975259970232059, 98.19639476549653523, 37.03425924184826101 ) ) ;
#47965=CYLINDRICAL_SURFACE ( 'NONE', #61319, 7.500000000000020428 ) ;
#47967=CARTESIAN_POINT ( 'NONE',  ( -11.57950265606958062, 8.174070387114799274, -9.576061325039194827 ) ) ;
#47968=CARTESIAN_POINT ( 'NONE',  ( 157.0336341255056993, 57.31169401067820957, -77.96873488960137877 ) ) ;
#47969=DIRECTION ( 'NONE',  ( 0.000000000000000000, 0.000000000000000000, 1.000000000000000000 ) ) ;
#47970=CARTESIAN_POINT ( 'NONE',  ( -155.1355020251929773, 69.10372769512069624, -47.29556375445353211 ) ) ;
#47974=CARTESIAN_POINT ( 'NONE',  ( -79.14638003838382474, 23.58242782405879012, -35.11545063171788428 ) ) ;
#47975=CARTESIAN_POINT ( 'NONE',  ( 103.1602294306414933, 25.74091644446069083, 88.30902535134187303 ) ) ;
#47976=CARTESIAN_POINT ( 'NONE',  ( 113.4402889550712530, 31.50582881646777622, -9.776826010279577872 ) ) ;
#47979=CARTESIAN_POINT ( 'NONE',  ( 20.36314374176837916, 6.689939636827347158, 31.55112446504767476 ) ) ;
#47980=CARTESIAN_POINT ( 'NONE',  ( -156.3413281584584809, 71.56573911209629557, 94.99999999999866418 ) ) ;
#47985=CARTESIAN_POINT ( 'NONE',  ( -156.8773151811562627, 72.06122063279302381, -14.04873829481672054 ) ) ;
#47986=CARTESIAN_POINT ( 'NONE',  ( 32.15284246740100116, 8.588257691344876932, -41.18047241676685388 ) ) ;
#47988=CARTESIAN_POINT ( 'NONE',  ( -35.38560449531986052, 10.27249159032101922, 58.17866205316500583 ) ) ;
#47989=CYLINDRICAL_SURFACE ( 'NONE', #42985, 7.500000000000013323 ) ;
#47992=CARTESIAN_POINT ( 'NONE',  ( 186.7642514597452816, 86.02880938169741398, 68.55708177098027534 ) ) ;
#47993=CARTESIAN_POINT ( 'NONE',  ( -156.8764584803562343, 70.69066846313526753, 63.64140852508641188 ) ) ;
#47996=CARTESIAN_POINT ( 'NONE',  ( 17.73567516211396367, 7.577454475141601975, 3.410843060652023251 ) ) ;
#47997=CARTESIAN_POINT ( 'NONE',  ( 185.1802655733641529, 82.84606286178497214, 69.95176336533883443 ) ) ;
#47999=CARTESIAN_POINT ( 'NONE',  ( -81.90266786693715062, 23.58030232261292980, -35.83251721507301824 ) ) ;
#48000=CARTESIAN_POINT ( 'NONE',  ( 18.89064107370900913, 6.619789970027367687, 71.19189653376322724 ) ) ;
#48002=CARTESIAN_POINT ( 'NONE',  ( 203.1511228994173450, 104.2426341584999534, 56.16747440225678645 ) ) ;
#48005=EDGE_LOOP ( 'NONE', ( #41645, #38010 ) ) ;
#48008=CARTESIAN_POINT ( 'NONE',  ( 176.0745160362857860, 73.68684431790052258, 42.39531241251699356 ) ) ;
#48009=CARTESIAN_POINT ( 'NONE',  ( -131.3154845336012784, 50.16828105866952825, -47.61854828779179627 ) ) ;
#48010=CARTESIAN_POINT ( 'NONE',  ( -109.3386876948163433, 37.66246927061207117, -45.09996864586627652 ) ) ;
#48011=CARTESIAN_POINT ( 'NONE',  ( 55.57634120535664124, 12.09544293553732786, -69.08107002945564545 ) ) ;
#48015=CARTESIAN_POINT ( 'NONE',  ( -25.80058235236790054, 8.733375263008319678, -11.00299486492387757 ) ) ;
#48016=CARTESIAN_POINT ( 'NONE',  ( 174.2486163051500512, 71.96303772754802708, 87.40529692077977586 ) ) ;
#48019=CARTESIAN_POINT ( 'NONE',  ( 117.7411475730015553, 32.50808475802732289, 63.41313343984494821 ) ) ;
#48023=LINE ( 'NONE', #30838, #6136 ) ;
#48025=ADVANCED_FACE ( 'NONE', ( #30725 ), #25459, .F. ) ;
#48026=CARTESIAN_POINT ( 'NONE',  ( -97.47339919287391297, 30.40512551257287299, 43.79714771676525942 ) ) ;
#48027=CARTESIAN_POINT ( 'NONE',  ( 93.09528872995971938, 21.72934119836186184, -39.48931322913085751 ) ) ;
#48032=CARTESIAN_POINT ( 'NONE',  ( -118.4063383664800000, 41.75753822095644097, -15.05876597828681440 ) ) ;
#48035=CARTESIAN_POINT ( 'NONE',  ( -180.6209440844958465, 95.88392769199010957, -15.04742671162544632 ) ) ;
#48036=VECTOR ( 'NONE', #23121, 1000.000000000000000 ) ;
#48038=CARTESIAN_POINT ( 'NONE',  ( -147.7860806339125190, 62.73248524776227697, -49.62554806688481079 ) ) ;
#48039=ORIENTED_EDGE ( 'NONE', *, *, #48557, .F. ) ;
#48045=FACE_OUTER_BOUND ( 'NONE', #39757, .T. ) ;
#48046=CARTESIAN_POINT ( 'NONE',  ( -61.39252081892698953, 16.47343302442958901, -19.88650151685294531 ) ) ;
#48047=CARTESIAN_POINT ( 'NONE',  ( 79.38020582286195292, 17.07365509555548400, -18.46566652421186561 ) ) ;
#48048=VECTOR ( 'NONE', #44166, 1000.000000000000000 ) ;
#48049=CARTESIAN_POINT ( 'NONE',  ( -133.0921934900200085, 52.65587531157186874, -67.13582062954424146 ) ) ;
#48050=PLANE ( 'NONE',  #37028 ) ;
#48051=CARTESIAN_POINT ( 'NONE',  ( -97.88309373898358956, 30.60238467438963283, 5.079866515219528367 ) ) ;
#48052=CARTESIAN_POINT ( 'NONE',  ( -96.45845418068303445, 29.92035703021965176, -74.11387427670096884 ) ) ;
#48053=VERTEX_POINT ( 'NONE', #25110 ) ;
#48054=B_SPLINE_CURVE_WITH_KNOTS ( 'NONE', 3,
 ( #11894, #32323, #11532, #32663, #53751, #26356, #54089, #31974, #64674, #22105, #65022, #27724, #5237, #69253, #53403, #52388, #16817, #16132, #21408, #42852, #64321, #37587, #38278, #59034, #33010, #10856, #5576, #59723, #50578, #34421, #44951, #60438, #2745, #28420, #66782, #2058, #34061, #18571 ),
 .UNSPECIFIED., .F., .F.,
 ( 4, 2, 2, 2, 2, 2, 2, 2, 2, 2, 2, 2, 2, 2, 2, 2, 2, 2, 4 ),
 ( 0.02546424207107600771, 0.02703543426729205709, 0.02782103036540011995, 0.02860662646350817934, 0.03017781865972437444, 0.03174901085594056954, 0.03332020305215676464, 0.03489139524837295975, 0.03646258744458915485, 0.03724818354269723159, 0.03803377964080531526, 0.03881937573891339199, 0.03960497183702146873, 0.04117616403323766383, 0.04274735622945385893, 0.04431854842567005404, 0.04588974062188624914, 0.04746093281810244424, 0.05060331721053485526 ),
 .UNSPECIFIED. ) ;
#48055=EDGE_LOOP ( 'NONE', ( #22106, #66156, #68047, #54684 ) ) ;
#48056=DIRECTION ( 'NONE',  ( -0.000000000000000000, 1.000000000000000000, -0.000000000000000000 ) ) ;
#48057=CARTESIAN_POINT ( 'NONE',  ( 9.823983574062872037, 6.382904402091122087, 32.94129060586310231 ) ) ;
#48060=PLANE ( 'NONE',  #47892 ) ;
#48061=CARTESIAN_POINT ( 'NONE',  ( -71.97171223898807568, 20.94894057408425780, 41.33603137547984829 ) ) ;
#48062=CARTESIAN_POINT ( 'NONE',  ( 84.27368848767925158, 18.63026910897603727, 30.07530638778384358 ) ) ;
#48064=CARTESIAN_POINT ( 'NONE',  ( 39.88975917505626967, 9.487965272711662124, -50.61981746542780058 ) ) ;
#48069=CARTESIAN_POINT ( 'NONE',  ( -8.807541152391515027, 6.956521193351525412, -35.46664261147883934 ) ) ;
#48071=CARTESIAN_POINT ( 'NONE',  ( -85.85116202048752143, 25.18960254254224296, -94.10664488620292900 ) ) ;
#48074=CARTESIAN_POINT ( 'NONE',  ( 32.46582168790593670, 7.608418697099893713, -67.07998740085851352 ) ) ;
#48075=CARTESIAN_POINT ( 'NONE',  ( -100.4440683050664518, 32.98184228837416043, -62.07263191239334077 ) ) ;
#48076=CARTESIAN_POINT ( 'NONE',  ( 112.9086998128567672, 31.25010873462638727, -90.09042788728231699 ) ) ;
#48077=EDGE_LOOP ( 'NONE', ( #63994, #9424 ) ) ;
#48081=CARTESIAN_POINT ( 'NONE',  ( 57.57684776206768618, 12.50442334002049272, 58.98747899309388742 ) ) ;
#48084=DIRECTION ( 'NONE',  ( -0.000000000000000000, 1.000000000000000000, -0.000000000000000000 ) ) ;
#48085=CARTESIAN_POINT ( 'NONE',  ( -4.070918861171928249, 6.675509947362632701, 44.11282707256027180 ) ) ;
#48086=CARTESIAN_POINT ( 'NONE',  ( -95.86612279493104438, 29.64021615886204941, -11.77456874465409520 ) ) ;
#48087=CARTESIAN_POINT ( 'NONE',  ( 93.32575898730515007, 22.89018551198909535, 87.50692670039568100 ) ) ;
#48090=EDGE_LOOP ( 'NONE', ( #40471, #61306, #47046, #30772 ) ) ;
#48092=CARTESIAN_POINT ( 'NONE',  ( 133.8566784816069344, -170.0000000000000000, -97.21241211332302612 ) ) ;
#48094=CARTESIAN_POINT ( 'NONE',  ( -108.0902552660050588, 36.97681740369923631, 60.09494272580671748 ) ) ;
#48096=CARTESIAN_POINT ( 'NONE',  ( -133.0921934900200085, 52.65587531157188295, -40.29127003908051563 ) ) ;
#48099=CARTESIAN_POINT ( 'NONE',  ( 93.70675391435744928, 21.95852801827564349, 61.56192124033761104 ) ) ;
#48101=CARTESIAN_POINT ( 'NONE',  ( -148.2650023942115922, 63.13271795942794284, 84.50851806093228902 ) ) ;
#48102=EDGE_CURVE ( 'NONE', #34356, #5113, #51009, .T. ) ;
#48104=EDGE_CURVE ( 'NONE', #62594, #38367, #64447, .T. ) ;
#48106=FACE_OUTER_BOUND ( 'NONE', #42607, .T. ) ;
#48107=CARTESIAN_POINT ( 'NONE',  ( 80.73462811483979351, 18.54763808182593721, 5.703558285329590305 ) ) ;
#48108=CARTESIAN_POINT ( 'NONE',  ( 157.4703587214989113, 58.92748579479258808, 2.564916881789689462 ) ) ;
#48113=CARTESIAN_POINT ( 'NONE',  ( -108.1144194775597214, 35.84457139767598477, -47.25378443719495891 ) ) ;
#48114=CARTESIAN_POINT ( 'NONE',  ( 65.40032188136230218, 13.23841673691966925, -77.18017510422534144 ) ) ;
#48116=CARTESIAN_POINT ( 'NONE',  ( 157.4703587214989398, 58.92748579479258808, 17.56491688178971700 ) ) ;
#48122=CARTESIAN_POINT ( 'NONE',  ( 116.6436511186860798, 33.08230081168870385, -39.50517661178831474 ) ) ;
#48127=CARTESIAN_POINT ( 'NONE',  ( -167.6386155194958292, 81.22597462185134987, 43.46491529870461790 ) ) ;
#48128=CARTESIAN_POINT ( 'NONE',  ( -34.51918258780364823, 10.11719938103012240, -76.50446516501558847 ) ) ;
#48131=CARTESIAN_POINT ( 'NONE',  ( 46.51377856795991761, 10.46037936279323688, 13.00077528625720369 ) ) ;
#48132=VERTEX_POINT ( 'NONE', #40158 ) ;
#48136=CARTESIAN_POINT ( 'NONE',  ( -106.6711220790662651, 36.20923238211247508, 5.089478997775757740 ) ) ;
#48138=CARTESIAN_POINT ( 'NONE',  ( -155.1355020251929773, 69.10372769512071045, -74.14011434491720820 ) ) ;
#48139=CARTESIAN_POINT ( 'NONE',  ( 67.35224030275335849, 13.72040503854036331, 84.87408482119735709 ) ) ;
#48140=CYLINDRICAL_SURFACE ( 'NONE', #41521, 7.500000000000020428 ) ;
#48141=CARTESIAN_POINT ( 'NONE',  ( -131.7724154034330581, 50.48821165954354484, 69.62870055094876420 ) ) ;
#48142=CARTESIAN_POINT ( 'NONE',  ( 63.01563776193091826, 12.67277567978498176, 29.81296093922127710 ) ) ;
#48145=VERTEX_POINT ( 'NONE', #60909 ) ;
#48146=CARTESIAN_POINT ( 'NONE',  ( -75.43495400358860081, 22.18831810339352728, 57.99029328673930195 ) ) ;
#48147=CARTESIAN_POINT ( 'NONE',  ( 185.5415406465189676, 83.23025870924408309, 30.75849858761065292 ) ) ;
#48148=CARTESIAN_POINT ( 'NONE',  ( 59.29597493004737885, 11.84030339376943886, -63.53442171863188292 ) ) ;
#48149=CARTESIAN_POINT ( 'NONE',  ( -72.20490592113146988, 19.96451062593607872, 14.91352488762884931 ) ) ;
#48150=CARTESIAN_POINT ( 'NONE',  ( -119.2949674747224975, 43.48097822533565449, 68.56738607616526338 ) ) ;
#48152=CARTESIAN_POINT ( 'NONE',  ( 197.4024603413583350, 96.84614858128594506, 88.60102860378297862 ) ) ;
#48153=CARTESIAN_POINT ( 'NONE',  ( 15.78827728214693416, -170.0000000000000000, -35.51894409868578606 ) ) ;
#48154=ORIENTED_EDGE ( 'NONE', *, *, #38422, .T. ) ;
#48157=VERTEX_POINT ( 'NONE', #28560 ) ;
#48159=CARTESIAN_POINT ( 'NONE',  ( -23.93895920923072396, 9.495000752338453864, -69.90383058804481209 ) ) ;
#48160=CARTESIAN_POINT ( 'NONE',  ( 217.9999999999999716, 128.6235316737731296, 94.99999999999866418 ) ) ;
#48162=ADVANCED_FACE ( 'NONE', ( #50369 ), #50005, .T. ) ;
#48164=ORIENTED_EDGE ( 'NONE', *, *, #38350, .T. ) ;
#48165=ORIENTED_EDGE ( 'NONE', *, *, #3842, .F. ) ;
#48166=DIRECTION ( 'NONE',  ( -0.000000000000000000, 1.000000000000000000, -0.000000000000000000 ) ) ;
#48170=CARTESIAN_POINT ( 'NONE',  ( 204.6977192012829789, 106.3443248447423457, 44.20772073876944575 ) ) ;
#48172=EDGE_CURVE ( 'NONE', #39145, #47003, #35136, .T. ) ;
#48176=ORIENTED_EDGE ( 'NONE', *, *, #7720, .T. ) ;
#48178=EDGE_CURVE ( 'NONE', #22146, #56862, #54340, .T. ) ;
#48182=CARTESIAN_POINT ( 'NONE',  ( 35.44311777160620380, 8.940232499250161169, -63.58956774339669238 ) ) ;
#48185=CARTESIAN_POINT ( 'NONE',  ( -190.4968431727839402, 108.8425311198515004, -73.13328961415110996 ) ) ;
#48188=CARTESIAN_POINT ( 'NONE',  ( -96.45845418068304866, 29.92035703021964466, 60.10887867561745423 ) ) ;
#48189=ORIENTED_EDGE ( 'NONE', *, *, #42321, .T. ) ;
#48190=B_SPLINE_CURVE_WITH_KNOTS ( 'NONE', 3,
 ( #60505, #61205, #38708, #18640, #11972, #12670, #66159, #40101, #33442, #55932, #7749, #45017, #65440, #54868, #43964, #2125, #23239, #60151 ),
 .UNSPECIFIED., .F., .F.,
 ( 4, 2, 2, 2, 2, 2, 2, 2, 4 ),
 ( 0.01054411675784286233, 0.01184819941084477336, 0.01315228206384668266, 0.01445636471684859370, 0.01576044736985050473, 0.01706453002285241577, 0.01836861267585432334, 0.01967269532885623437, 0.02097677798185814541 ),
 .UNSPECIFIED. ) ;
#48191=CARTESIAN_POINT ( 'NONE',  ( -73.63346300764935393, 20.46798018699518096, 32.35235876508207298 ) ) ;
#48192=ORIENTED_EDGE ( 'NONE', *, *, #4674, .F. ) ;
#48194=CARTESIAN_POINT ( 'NONE',  ( -118.6302575928420424, 43.07263081214308897, 13.16250469874441009 ) ) ;
#48197=CARTESIAN_POINT ( 'NONE',  ( 129.1137093889807943, 38.63348691920619871, 58.04000564037256282 ) ) ;
#48198=VERTEX_POINT ( 'NONE', #59079 ) ;
#48201=CARTESIAN_POINT ( 'NONE',  ( 155.2910738464913436, 55.97560547655806573, 29.71883570028862920 ) ) ;
#48206=CARTESIAN_POINT ( 'NONE',  ( -24.94151142167916646, 8.614613465433006212, 33.93833259409825587 ) ) ;
#48207=CARTESIAN_POINT ( 'NONE',  ( -142.5087559769084748, 59.74468185400778708, -66.40863924655131711 ) ) ;
#48208=ORIENTED_EDGE ( 'NONE', *, *, #54705, .T. ) ;
#48212=CARTESIAN_POINT ( 'NONE',  ( -180.3161328724957855, 97.10341277064807741, 67.30497477601284118 ) ) ;
#48215=CARTESIAN_POINT ( 'NONE',  ( -81.23268307104841313, 24.39742801172156206, 4.022339847785443290 ) ) ;
#48218=CARTESIAN_POINT ( 'NONE',  ( -71.36003922708370339, 19.67168905366865772, -94.55123213910407287 ) ) ;
#48219=DIRECTION ( 'NONE',  ( 0.000000000000000000, 0.000000000000000000, 1.000000000000000000 ) ) ;
#48220=CARTESIAN_POINT ( 'NONE',  ( 160.9069879467681119, 60.37290772564306707, 3.382471444115906500 ) ) ;
#48221=CARTESIAN_POINT ( 'NONE',  ( 45.90675866695829654, 10.36357315963267922, -93.06977314594286099 ) ) ;
#48222=ORIENTED_EDGE ( 'NONE', *, *, #16274, .F. ) ;
#48223=CARTESIAN_POINT ( 'NONE',  ( -38.68632430131779643, 11.91908191268693074, 12.81834785221818684 ) ) ;
#48224=ORIENTED_EDGE ( 'NONE', *, *, #61362, .F. ) ;
#48226=ORIENTED_EDGE ( 'NONE', *, *, #62495, .T. ) ;
#48228=CARTESIAN_POINT ( 'NONE',  ( 19.54452863209719027, 7.657034792877146501, -63.35344965661052186 ) ) ;
#48229=CARTESIAN_POINT ( 'NONE',  ( 117.6076489466057780, 33.56811790321052058, 89.33957235143014941 ) ) ;
#48230=LINE ( 'NONE', #22562, #49045 ) ;
#48231=CARTESIAN_POINT ( 'NONE',  ( 67.56108154898467433, 13.77276756375644595, -10.39039143759568518 ) ) ;
#48233=CARTESIAN_POINT ( 'NONE',  ( 138.5943620234099001, 45.55242290395134575, -49.35784197316183253 ) ) ;
#48234=CARTESIAN_POINT ( 'NONE',  ( -54.56685407443680447, 15.59259313022788085, -62.06087458892354647 ) ) ;
#48237=EDGE_LOOP ( 'NONE', ( #8354, #709, #38616, #5695 ) ) ;
#48242=ADVANCED_FACE ( 'NONE', ( #54491 ), #54136, .T. ) ;
#48243=CARTESIAN_POINT ( 'NONE',  ( 129.8870388671970204, 40.24164088984107934, -90.83676810778949573 ) ) ;
#48246=ORIENTED_EDGE ( 'NONE', *, *, #34088, .T. ) ;
#48247=CARTESIAN_POINT ( 'NONE',  ( 91.11019107624152014, 22.06959540317786761, 16.38678607536089160 ) ) ;
#48248=CARTESIAN_POINT ( 'NONE',  ( 188.4920037102893957, 87.93425473911918289, -15.67097523847415808 ) ) ;
#48249=CARTESIAN_POINT ( 'NONE',  ( 206.2957331585308793, 110.2946564621822745, 2.490034632839250417 ) ) ;
#48251=CARTESIAN_POINT ( 'NONE',  ( 41.81982603358024875, 8.735900550613189708, -9.159026031209867469 ) ) ;
#48252=CARTESIAN_POINT ( 'NONE',  ( 208.9507214515059843, 112.3605999017434982, -23.17500676389725456 ) ) ;
#48254=CARTESIAN_POINT ( 'NONE',  ( 164.8444104055694766, 64.93678790243659193, 62.35759023313505622 ) ) ;
#48259=CARTESIAN_POINT ( 'NONE',  ( 130.7260570116704059, 40.73146260246712558, 16.99693353642962990 ) ) ;
#48260=CARTESIAN_POINT ( 'NONE',  ( 89.20981392318256553, 21.38519354635262815, -36.27533723528620158 ) ) ;
#48261=CARTESIAN_POINT ( 'NONE',  ( 155.7167524447090727, 57.56687707799954268, 71.05957392723330202 ) ) ;
#48263=DIRECTION ( 'NONE',  ( -0.8160245890732938934, -0.5780171883497599028, 0.000000000000000000 ) ) ;
#48265=CARTESIAN_POINT ( 'NONE',  ( -3.022581224654154131, 7.632926133645733024, 85.53503376044743334 ) ) ;
#48266=VERTEX_POINT ( 'NONE', #1049 ) ;
#48267=CARTESIAN_POINT ( 'NONE',  ( 63.01563776193090405, 12.67277567978497643, 17.96841034875761878 ) ) ;
#48271=CARTESIAN_POINT ( 'NONE',  ( 32.39877097090366931, 8.612975291426320013, 93.80784019633749438 ) ) ;
#48273=CARTESIAN_POINT ( 'NONE',  ( 105.8022841538864185, 26.88074187880708976, 31.04807806109887025 ) ) ;
#48275=CARTESIAN_POINT ( 'NONE',  ( -58.76006735892197241, 15.70681061434692261, -76.08508450424285741 ) ) ;
#48276=CARTESIAN_POINT ( 'NONE',  ( 38.90894112122322213, 8.345444037631242651, -8.775266874964067654 ) ) ;
#48279=CARTESIAN_POINT ( 'NONE',  ( 164.8121648350735882, 63.59223683144968220, 89.02090917915565171 ) ) ;
#48280=CARTESIAN_POINT ( 'NONE',  ( 93.70675391435746349, 21.95852801827565060, 34.71737064987392074 ) ) ;
#48282=CARTESIAN_POINT ( 'NONE',  ( 105.7953515382196059, 27.97683113100022467, -10.51959647692886080 ) ) ;
#48284=CARTESIAN_POINT ( 'NONE',  ( 9.689943677145727463, 7.388265075009367244, 33.14200807007561167 ) ) ;
#48285=CARTESIAN_POINT ( 'NONE',  ( 65.02380462922316440, 13.14718491827419555, -89.67200624934488928 ) ) ;
#48286=CARTESIAN_POINT ( 'NONE',  ( -85.50249391410862643, 26.13441511443011578, 94.70962812146305509 ) ) ;
#48291=CARTESIAN_POINT ( 'NONE',  ( -7.825402957745085430, 6.891034867348157178, -8.573520141480125645 ) ) ;
#48292=CARTESIAN_POINT ( 'NONE',  ( -166.7617689806962460, 81.76611317639944332, 88.02160040033108146 ) ) ;
#48294=CARTESIAN_POINT ( 'NONE',  ( -190.6985136298601731, 109.1272424661242582, -95.00000000000133582 ) ) ;
#48295=CARTESIAN_POINT ( 'NONE',  ( -37.93379515072631847, 11.77251734620211288, 60.77801631423660211 ) ) ;
#48297=CARTESIAN_POINT ( 'NONE',  ( 150.7926588734436280, 52.63999027731883729, -67.04403352340344213 ) ) ;
#48298=CARTESIAN_POINT ( 'NONE',  ( 17.74393407086870056, 6.570779001277778697, -8.916980308073734207 ) ) ;
#48299=ORIENTED_EDGE ( 'NONE', *, *, #33846, .F. ) ;
#48300=CARTESIAN_POINT ( 'NONE',  ( -156.9406434201983700, 70.74968524571475825, -41.16293729598802287 ) ) ;
#48303=CARTESIAN_POINT ( 'NONE',  ( 68.63585058221468671, 15.08566240483131438, -21.36693067117767697 ) ) ;
#48304=CARTESIAN_POINT ( 'NONE',  ( -82.32006615997346444, 24.83050031643765720, -49.18324661891568184 ) ) ;
#48305=CYLINDRICAL_SURFACE ( 'NONE', #40093, 7.500000000000020428 ) ;
#48307=CARTESIAN_POINT ( 'NONE',  ( -151.6648563624119106, 67.36546864992756412, 4.179678963093405919 ) ) ;
#48309=CARTESIAN_POINT ( 'NONE',  ( 183.1910712700537545, 80.76073941711165105, -36.51428264922770950 ) ) ;
#48311=CARTESIAN_POINT ( 'NONE',  ( -155.7884408287038696, 71.05759622589089020, 87.79867964050457374 ) ) ;
#48313=EDGE_LOOP ( 'NONE', ( #14645, #41911 ) ) ;
#48316=CARTESIAN_POINT ( 'NONE',  ( -156.0204364459164879, 71.27041535366186054, -11.74006770552829870 ) ) ;
#48318=CARTESIAN_POINT ( 'NONE',  ( 31.90170717962885405, 8.563261373066637816, -42.87966478670944781 ) ) ;
#48319=EDGE_CURVE ( 'NONE', #14354, #47669, #26401, .T. ) ;
#48320=CARTESIAN_POINT ( 'NONE',  ( -34.74312654625184393, 10.15703162223800504, 57.82354398925224359 ) ) ;
#48321=CARTESIAN_POINT ( 'NONE',  ( 197.4121679705847328, 98.46451029407251099, 61.76465183233728595 ) ) ;
#48323=CARTESIAN_POINT ( 'NONE',  ( 184.0001683447904099, 83.06228184427189376, 56.72983684963124773 ) ) ;
#48324=CARTESIAN_POINT ( 'NONE',  ( -153.7005182577090068, 67.81869626254727734, 71.30039421697708235 ) ) ;
#48325=CARTESIAN_POINT ( 'NONE',  ( 23.03546163277113124, 7.848986635155161373, 12.61657727460462830 ) ) ;
#48326=CARTESIAN_POINT ( 'NONE',  ( 107.0471828278921009, 27.43080724084234845, 17.06850905904248350 ) ) ;
#48328=CARTESIAN_POINT ( 'NONE',  ( -86.10361028793435878, 25.29528064050659708, -43.61713178642852284 ) ) ;
#48329=CARTESIAN_POINT ( 'NONE',  ( 18.66025561752211104, 6.609375019058820300, 57.41805809103978930 ) ) ;
#48331=CARTESIAN_POINT ( 'NONE',  ( 8.480442907658519047, 6.376693431076494889, -68.15865659835031920 ) ) ;
#48333=ORIENTED_EDGE ( 'NONE', *, *, #68219, .T. ) ;
#48337=CARTESIAN_POINT ( 'NONE',  ( 175.3815143714021190, 73.02838262206999786, 41.68673370242148479 ) ) ;
#48338=CARTESIAN_POINT ( 'NONE',  ( -55.05276343752910151, -170.0000000000000000, 45.31732777293115788 ) ) ;
#48339=CARTESIAN_POINT ( 'NONE',  ( 46.84183314611288296, 9.494161546644496852, -68.98510195083733265 ) ) ;
#48340=CARTESIAN_POINT ( 'NONE',  ( 55.51528220483958620, 12.08323518953685216, -69.82681857395122904 ) ) ;
#48345=CARTESIAN_POINT ( 'NONE',  ( 173.8016025329976344, 71.54639721357104065, 88.69313603028011528 ) ) ;
#48349=CARTESIAN_POINT ( 'NONE',  ( 114.6632852039171411, 30.98120524556724931, 57.89195650209787658 ) ) ;
#48353=CARTESIAN_POINT ( 'NONE',  ( 135.0005116824453637, 43.29964618809727028, 56.43905545767402998 ) ) ;
#48356=B_SPLINE_CURVE_WITH_KNOTS ( 'NONE', 3,
 ( #8821, #24653, #46783, #51029, #41169, #67908, #46088, #30271, #52065, #62964, #19357, #29565, #68254, #13398, #67557, #8116, #20059, #2843, #3878, #14439, #24310, #3526, #40813, #25349, #34860, #56297, #9502, #41511, #40467, #29920, #46429, #45751, #67231, #14770, #30964, #19016, #51720, #62267, #61911, #35193, #56648, #19707, #36236, #52410 ),
 .UNSPECIFIED., .F., .F.,
 ( 4, 2, 2, 2, 2, 2, 2, 2, 2, 2, 2, 2, 2, 2, 2, 2, 2, 2, 2, 2, 2, 4 ),
 ( 0.000000000000000000, 0.003518733725596301810, 0.004398417156995386261, 0.005278100588394469411, 0.007037467451192689488, 0.007917150882591761363, 0.008796834313990834972, 0.01055620117678902209, 0.01231556803958721094, 0.01319525147098630537, 0.01407493490238540153, 0.01495461833378449422, 0.01583430176518358865, 0.01671398519658268134, 0.01759366862798177750, 0.01935303549077994900, 0.02111240235357811704, 0.02199208578497717850, 0.02287176921637623650, 0.02463113607917438025, 0.02639050294197252747, 0.02814986980477067122 ),
 .UNSPECIFIED. ) ;
#48359=CARTESIAN_POINT ( 'NONE',  ( -179.9997297618090784, 95.12611598520665268, 94.99999999999866418 ) ) ;
#48360=EDGE_LOOP ( 'NONE', ( #57361, #49180 ) ) ;
#48364=CARTESIAN_POINT ( 'NONE',  ( -143.2587158300142107, 60.34092810886538416, -38.15695033877188536 ) ) ;
#48366=CARTESIAN_POINT ( 'NONE',  ( -165.7140086129056158, 80.68381997492571145, -70.27195394581150367 ) ) ;
#48367=CARTESIAN_POINT ( 'NONE',  ( -142.8450945664715164, 58.72815783657288335, -38.85811206571208487 ) ) ;
#48371=CARTESIAN_POINT ( 'NONE',  ( -190.6985136298601731, 109.1272424661242582, 94.99999999999866418 ) ) ;
#48372=EDGE_CURVE ( 'NONE', #27916, #11578, #3248, .T. ) ;
#48374=CARTESIAN_POINT ( 'NONE',  ( 135.4423125506059193, 42.39015362494583883, -24.01277294691661268 ) ) ;
#48375=CARTESIAN_POINT ( 'NONE',  ( 88.98408042523108463, 20.23787745328938215, -77.29091413920239972 ) ) ;
#48377=CARTESIAN_POINT ( 'NONE',  ( -99.31850058233797540, 31.30166762705810513, 18.06902438764207020 ) ) ;
#48381=VECTOR ( 'NONE', #37609, 1000.000000000000000 ) ;
#48382=CARTESIAN_POINT ( 'NONE',  ( 188.5837490358996433, 86.53279111916960176, -70.88036999316274489 ) ) ;
#48386=CARTESIAN_POINT ( 'NONE',  ( 103.1534365798307959, 26.83148826706845469, -67.76694820224788884 ) ) ;
#48388=CARTESIAN_POINT ( 'NONE',  ( 84.74140601443112075, 18.78541996275573212, 44.47455478255000116 ) ) ;
#48389=CARTESIAN_POINT ( 'NONE',  ( 66.07923263163411320, 14.44036440558002354, -50.07076703234795190 ) ) ;
#48390=CARTESIAN_POINT ( 'NONE',  ( -119.2804658695888236, 43.47213805166353495, 34.57302842571210277 ) ) ;
#48391=CARTESIAN_POINT ( 'NONE',  ( 212.1931396682533091, 117.2245435827728954, 63.86598910989989264 ) ) ;
#48394=CARTESIAN_POINT ( 'NONE',  ( -55.05276343752910151, -170.0000000000000000, -15.87177340799618364 ) ) ;
#48400=CARTESIAN_POINT ( 'NONE',  ( -81.67541167344860753, 23.49044848824860665, 84.73050038251950866 ) ) ;
#48401=CARTESIAN_POINT ( 'NONE',  ( 93.32228019177713918, 22.88890999585038699, 60.66295313681071377 ) ) ;
#48403=DIRECTION ( 'NONE',  ( -0.8118923937861950435, -0.5838071093367415143, 0.000000000000000000 ) ) ;
#48404=CARTESIAN_POINT ( 'NONE',  ( -94.83794676023110526, 30.26879337035744655, -68.29633011496009942 ) ) ;
#48405=ADVANCED_FACE ( 'NONE', ( #39379 ), #17574, .F. ) ;
#48406=CARTESIAN_POINT ( 'NONE',  ( 116.1038088070373675, 32.81248144313010329, -92.41388108080619190 ) ) ;
#48407=VERTEX_POINT ( 'NONE', #60482 ) ;
#48411=CARTESIAN_POINT ( 'NONE',  ( 62.53356220515463093, 13.59349015304565178, 56.65751152968498161 ) ) ;
#48413=CARTESIAN_POINT ( 'NONE',  ( -7.825402957745081878, 7.899365992529268965, 3.271030448983517580 ) ) ;
#48415=CARTESIAN_POINT ( 'NONE',  ( -6.851003965218994018, 6.829052369041588300, 30.16287756619037452 ) ) ;
#48416=CARTESIAN_POINT ( 'NONE',  ( -31.43908319763709969, 10.61114334766715928, 72.06100499665289760 ) ) ;
#48417=CARTESIAN_POINT ( 'NONE',  ( 79.13548761208615190, 18.05107300752372623, 90.44251185706802687 ) ) ;
#48421=CARTESIAN_POINT ( 'NONE',  ( -154.0833774771448645, 69.51012195447351871, 71.02675010485698692 ) ) ;
#48423=ADVANCED_FACE ( 'NONE', ( #8060 ), #13010, .F. ) ;
#48425=CARTESIAN_POINT ( 'NONE',  ( -104.5916564445179802, 35.10571011602406344, 72.01391628937817302 ) ) ;
#48426=CARTESIAN_POINT ( 'NONE',  ( -133.1640943168118554, 52.70734926280007215, -40.55218783485771894 ) ) ;
#48428=DIRECTION ( 'NONE',  ( 0.000000000000000000, 0.000000000000000000, 1.000000000000000000 ) ) ;
#48429=CARTESIAN_POINT ( 'NONE',  ( -2.190131154568196958, 6.589492063460818727, -21.02878240156981349 ) ) ;
#48430=CARTESIAN_POINT ( 'NONE',  ( -155.0443000888154472, 69.02121705336244872, 86.81356557659563578 ) ) ;
#48431=CARTESIAN_POINT ( 'NONE',  ( 140.1999945597798956, 45.38880890490930398, 33.00061941519715702 ) ) ;
#48434=CARTESIAN_POINT ( 'NONE',  ( 80.71682498289320051, 18.54204664833079264, 15.00838200872322759 ) ) ;
#48435=CARTESIAN_POINT ( 'NONE',  ( 157.9121974517528315, 59.27335488206247760, 2.564916881789687242 ) ) ;
#48438=AXIS2_PLACEMENT_3D ( 'NONE', #19499, #57148, #51525 ) ;
#48441=B_SPLINE_CURVE_WITH_KNOTS ( 'NONE', 3,
 ( #27421, #23560, #38684, #60133, #11947, #50289, #66140, #702, #44997, #39730, #33764, #22156, #17577, #49923, #1753, #2111, #27775, #33420, #17929, #6672, #60829, #39042, #43600, #60486, #32709, #55201, #28476, #62577, #35845, #34471, #68204, #41119, #35494, #24943, #3150, #18968, #14394, #45349, #56955, #62216, #40416, #67507, #56597, #55913, #45701, #61186, #29180, #67860, #23902, #57297, #8777, #46381, #2794, #19656, #9110, #19305, #61863, #30562, #50624, #2445, #52013, #46733, #3828, #20012 ),
 .UNSPECIFIED., .F., .F.,
 ( 4, 2, 2, 2, 2, 2, 2, 2, 2, 2, 2, 2, 2, 2, 2, 2, 2, 2, 2, 2, 2, 2, 2, 2, 2, 2, 2, 2, 2, 2, 2, 4 ),
 ( 0.000000000000000000, 0.002176927744816822309, 0.003265391617225233897, 0.004353855489633644618, 0.004898087425837850846, 0.005442319362042056206, 0.006530783234450467795, 0.007619247106858878515, 0.008707710979267289236, 0.009796174851675701692, 0.01088463872408411241, 0.01197310259649252313, 0.01306156646890093559, 0.01415003034130934631, 0.01523849421371775703, 0.01632695808612616775, 0.01741542195853457847, 0.01959234970335132012, 0.02068081357575972043, 0.02176927744816812074, 0.02285774132057652105, 0.02394620519298491790, 0.02612313293780171158, 0.02666736487400589786, 0.02721159681021008414, 0.02830006068261845323, 0.02938852455502682232, 0.03047698842743518793, 0.03156545229984356049, 0.03265391617225192611, 0.03374238004466029867, 0.03483084391706866428 ),
 .UNSPECIFIED. ) ;
#48444=CARTESIAN_POINT ( 'NONE',  ( -109.3432140528234697, 36.51591785955880454, -39.94014320226850856 ) ) ;
#48445=CARTESIAN_POINT ( 'NONE',  ( -7.825402957745087207, -170.0000000000000000, 91.30468222037457338 ) ) ;
#48448=CARTESIAN_POINT ( 'NONE',  ( 164.4728833318992258, 63.30716077995678148, 39.60918866813992878 ) ) ;
#48457=CARTESIAN_POINT ( 'NONE',  ( -165.9986675144416211, 79.53506019208359135, 40.68902089630642394 ) ) ;
#48458=CARTESIAN_POINT ( 'NONE',  ( -33.84080342750782933, 9.997552308299095358, -76.78360896099182753 ) ) ;
#48463=CARTESIAN_POINT ( 'NONE',  ( -47.55517274199435462, 12.79855951204728370, 91.88478847849279418 ) ) ;
#48465=CARTESIAN_POINT ( 'NONE',  ( -153.6931187576189473, 67.81270084382356345, -75.38512700933921451 ) ) ;
#48466=B_SPLINE_CURVE_WITH_KNOTS ( 'NONE', 3,
 ( #47751, #37551, #32286, #9449, #31586, #31941, #58648, #47072, #21373, #69553, #41803, #53026, #4853, #69214, #48094, #21038, #9798, #42817, #63945, #4512, #42488, #36876, #63262, #37202, #5203, #10471, #47405, #42142, #26657, #16094, #64286, #62918, #59000, #68536, #10819, #53718, #36181, #5540, #26994, #48425, #256, #30909, #63606, #14718 ),
 .UNSPECIFIED., .F., .F.,
 ( 4, 2, 2, 2, 2, 2, 2, 2, 2, 2, 2, 2, 2, 2, 2, 2, 2, 2, 2, 2, 2, 4 ),
 ( 0.02477387709520259204, 0.02633314402883780297, 0.02711277749565540671, 0.02789241096247300697, 0.02945167789610821096, 0.03023131136292582510, 0.03101094482974343924, 0.03257021176337864671, 0.03334984523019624003, 0.03412947869701383335, 0.03568874563064902000, 0.03646837909746659945, 0.03724801256428417195, 0.03802764603110174446, 0.03880727949791931697, 0.04036654643155445504, 0.04192581336518959312, 0.04348508029882473813, 0.04504434723245986927, 0.04660361416609501428, 0.04816288109973015236, 0.04972214803336529043 ),
 .UNSPECIFIED. ) ;
#48467=CARTESIAN_POINT ( 'NONE',  ( -107.4812999401992073, 35.50239240081075565, 86.29593079873286854 ) ) ;
#48478=CARTESIAN_POINT ( 'NONE',  ( 206.7099580236349823, 109.1417833474364727, -63.43384006045138790 ) ) ;
#48481=LINE ( 'NONE', #316, #14432 ) ;
#48482=CARTESIAN_POINT ( 'NONE',  ( -125.8938041572051389, 47.69968343338781125, 72.46449846362081360 ) ) ;
#48483=CARTESIAN_POINT ( 'NONE',  ( 16.77480716385437631, 7.540753720029939267, 30.06375086438559308 ) ) ;
#48484=EDGE_CURVE ( 'NONE', #43433, #49905, #11033, .T. ) ;
#48493=CARTESIAN_POINT ( 'NONE',  ( -79.62258606008208517, 22.68765733708494636, 30.46417967397961490 ) ) ;
#48495=CARTESIAN_POINT ( 'NONE',  ( 63.01563776193091826, 12.67277567978498531, -50.72069083216976537 ) ) ;
#48497=AXIS2_PLACEMENT_3D ( 'NONE', #25713, #10195, #15495 ) ;
#48498=CARTESIAN_POINT ( 'NONE',  ( -30.47069031368415537, 9.433993659086574723, 57.10770550136132329 ) ) ;
#48501=VECTOR ( 'NONE', #11186, 1000.000000000000000 ) ;
#48505=EDGE_CURVE ( 'NONE', #168, #38167, #45700, .T. ) ;
#48506=EDGE_CURVE ( 'NONE', #59279, #44163, #40912, .T. ) ;
#48510=CARTESIAN_POINT ( 'NONE',  ( -147.1538409485623333, 63.51600817366542628, 31.09618653746209560 ) ) ;
#48511=CARTESIAN_POINT ( 'NONE',  ( 55.90910788310616653, 11.13585330978403931, 66.60498196571883511 ) ) ;
#48522=CARTESIAN_POINT ( 'NONE',  ( 67.55134213333074911, 13.77030723107741217, 31.31968777660861036 ) ) ;
#48523=CARTESIAN_POINT ( 'NONE',  ( 20.62738791527532101, 7.711277635208470649, 85.46445541659694811 ) ) ;
#48525=CARTESIAN_POINT ( 'NONE',  ( 79.14242532928585661, 17.00090225993928783, 10.87724778048851881 ) ) ;
#48527=CARTESIAN_POINT ( 'NONE',  ( -76.78936026062119424, 21.61552955137052479, 30.65294656790032946 ) ) ;
#48531=CARTESIAN_POINT ( 'NONE',  ( -142.2626321327577728, 58.26997216742665842, -71.11658358797649271 ) ) ;
#48536=LINE ( 'NONE', #59801, #45769 ) ;
#48540=CARTESIAN_POINT ( 'NONE',  ( 152.3102623290679958, 53.74757787434990774, 42.35763419393935436 ) ) ;
#48541=CARTESIAN_POINT ( 'NONE',  ( 68.94948716683069279, 15.16699441119057745, 32.69983809954490539 ) ) ;
#48546=CARTESIAN_POINT ( 'NONE',  ( -145.3246383987845149, 62.00818849034187252, -75.38709678301769657 ) ) ;
#48549=FACE_BOUND ( 'NONE', #22255, .T. ) ;
#48550=CARTESIAN_POINT ( 'NONE',  ( -3.252497086158839590, 6.636017118947989957, -75.72773057492425153 ) ) ;
#48552=CARTESIAN_POINT ( 'NONE',  ( -146.7404675333698378, 63.17262273741977907, -8.493795772565299274 ) ) ;
#48553=CARTESIAN_POINT ( 'NONE',  ( -123.0348077379026677, 45.83489305753316501, -35.47620429563009026 ) ) ;
#48554=CARTESIAN_POINT ( 'NONE',  ( -84.53753601793930272, 25.73343139558516768, 6.379961366978447401 ) ) ;
#48557=EDGE_CURVE ( 'NONE', #52201, #34184, #37206, .T. ) ;
#48560=CARTESIAN_POINT ( 'NONE',  ( 157.9130201331580565, 57.99550255803048060, 2.564916881789690351 ) ) ;
#48561=CARTESIAN_POINT ( 'NONE',  ( 92.52113039222226121, 22.58921125235803018, -11.81011023875010935 ) ) ;
#48563=CARTESIAN_POINT ( 'NONE',  ( -31.93169728792083362, 10.69234447276977562, 18.37190381572552056 ) ) ;
#48564=ORIENTED_EDGE ( 'NONE', *, *, #4218, .T. ) ;
#48568=CARTESIAN_POINT ( 'NONE',  ( 84.26390409839191875, 19.68678207880321551, -63.03273511366791126 ) ) ;
#48569=CARTESIAN_POINT ( 'NONE',  ( 116.3939302320144691, 32.95725513882212709, 86.49556688537334992 ) ) ;
#48570=CARTESIAN_POINT ( 'NONE',  ( -142.3187766126155225, 59.59460822661996815, 62.85579774729529845 ) ) ;
#48571=CARTESIAN_POINT ( 'NONE',  ( 64.94794467308302899, 13.12874966082104322, -9.112897588248744185 ) ) ;
#48572=CARTESIAN_POINT ( 'NONE',  ( -28.13128612339709278, 10.08889185338653327, -36.06824119723449229 ) ) ;
#48574=CARTESIAN_POINT ( 'NONE',  ( -72.70872533823838069, 21.20779489546082885, -91.74330869458320592 ) ) ;
#48578=CARTESIAN_POINT ( 'NONE',  ( 36.98541457540710553, 9.120571655722411464, 71.37510936658638627 ) ) ;
#48579=CARTESIAN_POINT ( 'NONE',  ( -166.7136514167008556, 81.71618216218796249, 61.25921454291933088 ) ) ;
#48583=CARTESIAN_POINT ( 'NONE',  ( 70.26840926437850499, 15.51363403943109631, -95.00000000000133582 ) ) ;
#48587=CARTESIAN_POINT ( 'NONE',  ( 185.7267155939801739, 84.90388481853123892, -22.77551174952004942 ) ) ;
#48588=CARTESIAN_POINT ( 'NONE',  ( 211.3757499519975909, 117.8130818709823444, 13.28818959658699939 ) ) ;
#48591=CARTESIAN_POINT ( 'NONE',  ( 41.09671232177016265, 8.635892912882342287, -23.58539976383162795 ) ) ;
#48595=CARTESIAN_POINT ( 'NONE',  ( 163.5944442552010401, 63.88381951184479846, 68.09088869929966847 ) ) ;
#48599=CARTESIAN_POINT ( 'NONE',  ( 130.3035708464390439, 40.48418876551456691, 16.78814384215078448 ) ) ;
#48602=CARTESIAN_POINT ( 'NONE',  ( -47.79955240516187587, 13.88975739862079628, 62.68960868740774828 ) ) ;
#48605=CARTESIAN_POINT ( 'NONE',  ( -5.275096591305005411, 7.745869104888358336, 84.24396437760638889 ) ) ;
#48606=ORIENTED_EDGE ( 'NONE', *, *, #55107, .F. ) ;
#48607=CARTESIAN_POINT ( 'NONE',  ( 59.08638499266955790, 11.79550614876702141, 4.075424172557957192 ) ) ;
#48608=CARTESIAN_POINT ( 'NONE',  ( -61.39252081892698953, 16.47343302442958546, 60.64715025453807584 ) ) ;
#48611=CARTESIAN_POINT ( 'NONE',  ( 31.89306456119750521, 8.562405279423517257, 90.54126529181490923 ) ) ;
#48613=CARTESIAN_POINT ( 'NONE',  ( 88.98064924903391670, 21.30386569031176691, -63.04019652766769610 ) ) ;
#48615=CARTESIAN_POINT ( 'NONE',  ( -59.94781924509480575, 16.04872117907065032, -63.87327874414468454 ) ) ;
#48616=CARTESIAN_POINT ( 'NONE',  ( 37.70762885381311236, 8.195134395012276585, -8.965104318115102444 ) ) ;
#48617=CARTESIAN_POINT ( 'NONE',  ( 175.8947993867357127, 74.90689716047910451, -49.16091051003656531 ) ) ;
#48618=CARTESIAN_POINT ( 'NONE',  ( -151.2428028786328014, 66.99705074331123456, -76.46685696349274508 ) ) ;
#48622=CARTESIAN_POINT ( 'NONE',  ( -47.55256438668344288, 13.83151366677316219, -42.95852722453810202 ) ) ;
#48626=CARTESIAN_POINT ( 'NONE',  ( 12.68603346975294599, 7.427591953486039955, 44.34740265932830994 ) ) ;
#48627=CARTESIAN_POINT ( 'NONE',  ( 204.6977192012829505, 108.0580384837234931, -78.17048162308530834 ) ) ;
#48629=CARTESIAN_POINT ( 'NONE',  ( -83.98097503028121480, 25.50453459670680800, 86.30605427587425993 ) ) ;
#48630=DIRECTION ( 'NONE',  ( -0.000000000000000000, 1.000000000000000000, -0.000000000000000000 ) ) ;
#48631=ORIENTED_EDGE ( 'NONE', *, *, #39402, .F. ) ;
#48635=CARTESIAN_POINT ( 'NONE',  ( -9.771516655894552983, 7.025139475821121415, -23.33315609593830686 ) ) ;
#48636=CARTESIAN_POINT ( 'NONE',  ( -49.43915770973590895, 13.24768844696974845, 42.81511741946465577 ) ) ;
#48641=CARTESIAN_POINT ( 'NONE',  ( -35.38962320578852427, 11.29584325137384937, 70.94093902761839843 ) ) ;
#48642=CARTESIAN_POINT ( 'NONE',  ( -15.07235766390729026, 8.482541916553470784, -18.02097754923428852 ) ) ;
#48644=CARTESIAN_POINT ( 'NONE',  ( 23.28785143291466397, 6.856621069835718174, -16.67558055457178057 ) ) ;
#48646=VECTOR ( 'NONE', #45164, 1000.000000000000000 ) ;
#48654=AXIS2_PLACEMENT_3D ( 'NONE', #46530, #56751, #41268 ) ;
#48656=CARTESIAN_POINT ( 'NONE',  ( -157.0069571479806996, 72.18154199622281908, 11.07571264450559312 ) ) ;
#48657=CARTESIAN_POINT ( 'NONE',  ( -107.7743374187917595, 35.66028478413599601, 16.30335207078181980 ) ) ;
#48658=CARTESIAN_POINT ( 'NONE',  ( 17.74393407086870056, 6.570779001277778697, 44.77212087285361974 ) ) ;
#48659=CARTESIAN_POINT ( 'NONE',  ( -157.0040855759218630, 72.17887538959165283, 92.33198874388405386 ) ) ;
#48660=ORIENTED_EDGE ( 'NONE', *, *, #32710, .F. ) ;
#48661=ORIENTED_EDGE ( 'NONE', *, *, #38442, .F. ) ;
#48664=CARTESIAN_POINT ( 'NONE',  ( -8.320652113663527416, 6.923290556636832349, 18.27103044898354867 ) ) ;
#48665=CARTESIAN_POINT ( 'NONE',  ( 88.21281915446409982, 21.03303114364613435, -89.66901925827936282 ) ) ;
#48666=CARTESIAN_POINT ( 'NONE',  ( -38.26497993382596263, 10.81185389040528122, 67.67827709005032943 ) ) ;
#48669=CARTESIAN_POINT ( 'NONE',  ( 184.3966782763551748, 83.48172388049827930, 56.90975353678252446 ) ) ;
#48670=CARTESIAN_POINT ( 'NONE',  ( -156.9252506979473196, 70.73559306219777909, 63.92116529121810942 ) ) ;
#48671=CARTESIAN_POINT ( 'NONE',  ( -7.825402957745081878, 7.899365992529270741, -50.41807073194384259 ) ) ;
#48676=EDGE_CURVE ( 'NONE', #67501, #10586, #69557, .T. ) ;
#48678=DIRECTION ( 'NONE',  ( -0.8160245890732938934, -0.5780171883497599028, 0.000000000000000000 ) ) ;
#48683=CARTESIAN_POINT ( 'NONE',  ( 177.7889574972182345, 75.33777460203562271, 30.05619048107344327 ) ) ;
#48684=CARTESIAN_POINT ( 'NONE',  ( -127.6992109187851980, 47.69334801994794049, -49.70753535056091721 ) ) ;
#48686=CARTESIAN_POINT ( 'NONE',  ( 55.99998955208977947, 12.18058389017404686, -67.40205469635807844 ) ) ;
#48691=CARTESIAN_POINT ( 'NONE',  ( -125.8938041572051105, 46.49392987655493670, -88.60280507916129977 ) ) ;
#48693=CARTESIAN_POINT ( 'NONE',  ( 198.2581645178918848, 99.52881771501677122, 13.71845634271636172 ) ) ;
#48695=VERTEX_POINT ( 'NONE', #47408 ) ;
#48696=DIRECTION ( 'NONE',  ( -0.000000000000000000, 1.000000000000000000, -0.000000000000000000 ) ) ;
#48700=CARTESIAN_POINT ( 'NONE',  ( 104.3786071038062033, 27.35811053916146562, -92.41772670280587931 ) ) ;
#48701=CARTESIAN_POINT ( 'NONE',  ( 137.4031600461561027, 44.79620770172218869, 57.24220012813282210 ) ) ;
#48706=CARTESIAN_POINT ( 'NONE',  ( 93.92910382125421620, 22.04227458821877761, -41.58192722603683222 ) ) ;
#48707=ADVANCED_FACE ( 'NONE', ( #32289 ), #5543, .F. ) ;
#48708=DIRECTION ( 'NONE',  ( -0.8160245890732938934, -0.5780171883497599028, 0.000000000000000000 ) ) ;
#48713=EDGE_CURVE ( 'NONE', #3372, #17473, #5880, .T. ) ;
#48716=CARTESIAN_POINT ( 'NONE',  ( -165.6215009671260248, 80.58889799860442338, -68.74239935707777249 ) ) ;
#48717=CARTESIAN_POINT ( 'NONE',  ( -142.1381007084227122, 58.17237452544241449, -43.73358479738932658 ) ) ;
#48719=DIRECTION ( 'NONE',  ( -0.000000000000000000, 1.000000000000000000, -0.000000000000000000 ) ) ;
#48721=EDGE_LOOP ( 'NONE', ( #33984, #41954 ) ) ;
#48722=CARTESIAN_POINT ( 'NONE',  ( -133.1093894320205777, 51.43221067881453479, 36.00316402828616447 ) ) ;
#48723=CARTESIAN_POINT ( 'NONE',  ( -125.8938041572051389, -170.0000000000000000, 11.27539728269340280 ) ) ;
#48725=CARTESIAN_POINT ( 'NONE',  ( 82.95057496836386690, 18.19812356106674400, -9.923320146636031680 ) ) ;
#48726=CARTESIAN_POINT ( 'NONE',  ( 87.58098510096631628, 19.74745174099415479, -77.62095623220717755 ) ) ;
#48729=CARTESIAN_POINT ( 'NONE',  ( -99.10260179032846395, 31.19580119595417500, 17.97233264255025986 ) ) ;
#48730=CARTESIAN_POINT ( 'NONE',  ( -95.50384525802326152, 29.46973564057718420, -66.13451531431674368 ) ) ;
#48736=CARTESIAN_POINT ( 'NONE',  ( 46.41758729921142645, 9.425975226414237795, 34.75085537779860800 ) ) ;
#48743=CARTESIAN_POINT ( 'NONE',  ( -76.79042791651912125, 22.68960395613480330, -62.19449990835644826 ) ) ;
#48746=CARTESIAN_POINT ( 'NONE',  ( 46.12582897016702077, 10.39833982076224572, -39.78811412968926220 ) ) ;
#48750=CARTESIAN_POINT ( 'NONE',  ( -29.51272929882556539, 10.30144624948896670, 18.12442451181507508 ) ) ;
#48752=CARTESIAN_POINT ( 'NONE',  ( -11.78792974237933677, 7.181513757308656487, -49.29051053082125833 ) ) ;
#48754=FACE_OUTER_BOUND ( 'NONE', #50313, .T. ) ;
#48755=CARTESIAN_POINT ( 'NONE',  ( 15.78827728214693416, 6.500811158483328356, -8.674393508222097537 ) ) ;
#48756=CARTESIAN_POINT ( 'NONE',  ( 152.1190604254709910, 53.60705199010330801, -22.04039180145268162 ) ) ;
#48757=CARTESIAN_POINT ( 'NONE',  ( 37.45439421541016145, 9.177432671831375899, 17.82874747546184580 ) ) ;
#48760=CARTESIAN_POINT ( 'NONE',  ( 209.9451731426637480, 113.8261094108102753, 85.02890187354657314 ) ) ;
#48762=ORIENTED_EDGE ( 'NONE', *, *, #6454, .T. ) ;
#48764=CYLINDRICAL_SURFACE ( 'NONE', #28643, 7.500000000000013323 ) ;
#48766=CARTESIAN_POINT ( 'NONE',  ( -7.825402957745087207, 6.891034867348158954, 45.11558103944722120 ) ) ;
#48768=CARTESIAN_POINT ( 'NONE',  ( 86.98327316344760618, 20.60587179896667465, 83.40257220075987732 ) ) ;
#48772=CARTESIAN_POINT ( 'NONE',  ( -151.6797345123119101, 67.37848486615948218, 72.25752099154021835 ) ) ;
#48774=CARTESIAN_POINT ( 'NONE',  ( -167.6524579626394882, 82.69702609844095775, -47.35039770195071895 ) ) ;
#48776=CARTESIAN_POINT ( 'NONE',  ( -132.0870433264403516, 51.94057326482884207, -38.17611669845395284 ) ) ;
#48780=CARTESIAN_POINT ( 'NONE',  ( 198.8752826725510943, 100.3130050945022873, -21.71571402821468766 ) ) ;
#48781=CARTESIAN_POINT ( 'NONE',  ( -150.1435789396691121, 64.71993001749778784, 84.41785612803083438 ) ) ;
#48783=CYLINDRICAL_SURFACE ( 'NONE', #961, 7.500000000000020428 ) ;
#48786=CARTESIAN_POINT ( 'NONE',  ( 79.37778929114109872, 18.12554302172301135, 12.34647733481867604 ) ) ;
#48787=CARTESIAN_POINT ( 'NONE',  ( -149.9471644042847345, 65.87751327280743396, 30.73052297110500319 ) ) ;
#48788=AXIS2_PLACEMENT_3D ( 'NONE', #47919, #69026, #26136 ) ;
#48793=EDGE_CURVE ( 'NONE', #4017, #51087, #34026, .T. ) ;
#48794=VERTEX_POINT ( 'NONE', #34385 ) ;
#48796=B_SPLINE_CURVE_WITH_KNOTS ( 'NONE', 3,
 ( #51023, #60869, #45040, #12694, #66871, #34160, #18670, #55596, #40461, #61905, #24648, #40122, #61579, #13392, #13729, #35188, #67551, #36575, #10512, #46423, #26019, #35883, #24991, #4898, #21087, #19697, #68580, #31303, #57686, #57339, #42532, #20381, #52059, #58024, #15463, #52730, #9496, #4220, #15116, #47801, #25340, #36917, #20052, #41163 ),
 .UNSPECIFIED., .F., .F.,
 ( 4, 2, 2, 2, 2, 2, 2, 2, 2, 2, 2, 2, 2, 2, 2, 2, 2, 2, 2, 2, 2, 4 ),
 ( 1.398578778534940505E-17, 0.004120577325733468244, 0.006180865988600218845, 0.008241154651466969447, 0.01030144331433372092, 0.01133158764576706369, 0.01236173197720040300, 0.01339187630863374404, 0.01442202064006708681, 0.01545216497150042785, 0.01648230930293376889, 0.01699738146865044375, 0.01751245363436711167, 0.01854259796580047526, 0.01957274229723383191, 0.02060288662866719550, 0.02266317529153392962, 0.02472346395440066374, 0.02678375261726739440, 0.02781389694870080309, 0.02884404128013421179, 0.03296461860586794718 ),
 .UNSPECIFIED. ) ;
#48797=CARTESIAN_POINT ( 'NONE',  ( -118.6666422341620688, 41.91578446950640569, -94.04183589441188929 ) ) ;
#48799=DIRECTION ( 'NONE',  ( 0.000000000000000000, 0.000000000000000000, 1.000000000000000000 ) ) ;
#48800=CARTESIAN_POINT ( 'NONE',  ( 151.6178224291901131, 54.48737267587418387, 14.76196231147637050 ) ) ;
#48802=CARTESIAN_POINT ( 'NONE',  ( 164.9559213734324601, 63.71338633026439879, 37.45297374046533889 ) ) ;
#48806=ORIENTED_EDGE ( 'NONE', *, *, #2918, .T. ) ;
#48808=B_SPLINE_CURVE_WITH_KNOTS ( 'NONE', 3,
 ( #16500, #5257, #28091, #63998, #11918, #32680, #26717, #54105, #33029, #54820, #48147, #5930, #22473, #21770, #15810, #48829, #43214, #49535, #21101, #27742, #64339, #16151, #49183, #59057, #67152, #65749, #8392, #33736, #50951, #28808, #17545, #1366, #44629, #2763, #18941, #13325, #6993, #66454, #39354, #34782, #8035, #12623, #2418, #7352 ),
 .UNSPECIFIED., .F., .F.,
 ( 4, 2, 2, 2, 2, 2, 2, 2, 2, 2, 2, 2, 2, 2, 2, 2, 2, 2, 2, 2, 2, 4 ),
 ( 0.02814986980477066428, 0.02995274102020803464, 0.03085417662792673543, 0.03175561223564543623, 0.03355848345108280312, 0.03536135466652017695, 0.03716422588195755772, 0.03896709709739493155, 0.03986853270511362540, 0.04076996831283231926, 0.04167140392055100617, 0.04257283952826969309, 0.04347427513598838000, 0.04437571074370706692, 0.04527714635142575383, 0.04617858195914444075, 0.04798145317458180070, 0.04978432439001916759, 0.05158719560545653449, 0.05339006682089389444, 0.05519293803633125439, 0.05699580925176862128 ),
 .UNSPECIFIED. ) ;
#48809=CARTESIAN_POINT ( 'NONE',  ( -37.79823708645146496, 10.72197716414928692, -19.95651543701835351 ) ) ;
#48810=CARTESIAN_POINT ( 'NONE',  ( -180.4651598106648294, 97.28730001475651079, 39.87329604086140478 ) ) ;
#48811=CARTESIAN_POINT ( 'NONE',  ( -38.26497993382596974, 10.81185389040525280, -66.54447586226808653 ) ) ;
#48818=DIRECTION ( 'NONE',  ( 0.000000000000000000, 0.000000000000000000, 1.000000000000000000 ) ) ;
#48822=CARTESIAN_POINT ( 'NONE',  ( -51.16305185958752588, 14.71032321365092521, 85.08607359302328632 ) ) ;
#48823=CARTESIAN_POINT ( 'NONE',  ( 79.93126905972553686, 17.24332478304276250, 60.67301135421717362 ) ) ;
#48827=VERTEX_POINT ( 'NONE', #60404 ) ;
#48829=CARTESIAN_POINT ( 'NONE',  ( 187.8959968237854241, 85.77553094678181367, 33.65882037824376738 ) ) ;
#48831=CARTESIAN_POINT ( 'NONE',  ( -72.78737098446268305, 20.16853011470087864, 6.389890168941366078 ) ) ;
#48834=CARTESIAN_POINT ( 'NONE',  ( 201.2497471985136315, 101.7319188750771275, 83.71170961202953720 ) ) ;
#48844=CARTESIAN_POINT ( 'NONE',  ( -86.17927978631389863, 25.32700573188344251, 37.93022061236076325 ) ) ;
#48846=CARTESIAN_POINT ( 'NONE',  ( -29.51272929882557250, 10.30144624948894361, -62.40922725957596384 ) ) ;
#48847=CARTESIAN_POINT ( 'NONE',  ( 46.51377856795993182, 10.46037936279324754, 39.84532587672087089 ) ) ;
#48848=CARTESIAN_POINT ( 'NONE',  ( -102.2801239173131194, -170.0000000000000000, -76.85912785543962400 ) ) ;
#48856=CARTESIAN_POINT ( 'NONE',  ( 187.8389847489735018, 87.20903357420549185, -94.12450799417122482 ) ) ;
#48860=CARTESIAN_POINT ( 'NONE',  ( -29.34297344870648061, 10.27495334741685618, -89.30201075326299076 ) ) ;
#48869=CARTESIAN_POINT ( 'NONE',  ( 140.5781926063689014, 45.63383190293702540, -73.70520198257123923 ) ) ;
#48870=CARTESIAN_POINT ( 'NONE',  ( 8.000000000000007105, 249.8719672152120381, 94.99999999999866418 ) ) ;
#48871=ORIENTED_EDGE ( 'NONE', *, *, #60440, .F. ) ;
#48872=EDGE_CURVE ( 'NONE', #55930, #14210, #50209, .T. ) ;
#48873=CARTESIAN_POINT ( 'NONE',  ( 82.95057496836383848, 18.19812356106674400, 16.92123044382763908 ) ) ;
#48876=CARTESIAN_POINT ( 'NONE',  ( -75.43953471071000649, 21.11829282998125734, 31.13110847576471230 ) ) ;
#48880=VERTEX_POINT ( 'NONE', #20861 ) ;
#48881=CARTESIAN_POINT ( 'NONE',  ( -125.4463376280758951, 47.40387005565906975, 3.785361193902134769 ) ) ;
#48883=CARTESIAN_POINT ( 'NONE',  ( 93.92280655489128094, 22.03989931749465470, 8.601539047791877834 ) ) ;
#48889=AXIS2_PLACEMENT_3D ( 'NONE', #29457, #65719, #12950 ) ;
#48890=CARTESIAN_POINT ( 'NONE',  ( 151.3309484205704507, 53.03078371058069251, 41.22472127221216454 ) ) ;
#48891=VECTOR ( 'NONE', #28606, 1000.000000000000000 ) ;
#48892=CARTESIAN_POINT ( 'NONE',  ( -175.1968289912784371, 90.99944698359490758, -34.99253156508922302 ) ) ;
#48896=CARTESIAN_POINT ( 'NONE',  ( 86.62931800182293784, 20.48449268398422163, 71.55663816294304524 ) ) ;
#48900=CARTESIAN_POINT ( 'NONE',  ( -143.2498117110515921, 60.33382252735061968, -73.29988522007047891 ) ) ;
#48904=FACE_BOUND ( 'NONE', #30066, .T. ) ;
#48906=CARTESIAN_POINT ( 'NONE',  ( -4.504169684898453596, 6.697401007565304099, -63.03359714400242098 ) ) ;
#48907=CARTESIAN_POINT ( 'NONE',  ( -175.1968289912784655, 90.99944698359492179, 72.38567079676552396 ) ) ;
#48909=CARTESIAN_POINT ( 'NONE',  ( -119.2949674747224975, 43.48097822533564738, -38.81081628568947650 ) ) ;
#48910=CARTESIAN_POINT ( 'NONE',  ( -79.62207341875658528, 23.76621716825509623, 18.52792914764348353 ) ) ;
#48913=CARTESIAN_POINT ( 'NONE',  ( -71.99036027973076557, 19.88994728656304289, -92.87964317901223410 ) ) ;
#48914=CARTESIAN_POINT ( 'NONE',  ( 70.25990036603479894, 14.47042233282419943, 12.42607342676760496 ) ) ;
#48915=CARTESIAN_POINT ( 'NONE',  ( 162.1014732644455307, 61.34312237409765345, 15.98357356154483533 ) ) ;
#48916=CARTESIAN_POINT ( 'NONE',  ( 94.14197848494937659, 23.19876128416620631, -16.46679285838030893 ) ) ;
#48918=CARTESIAN_POINT ( 'NONE',  ( -32.41898580403142915, 10.77423026598439471, 18.32383438413782528 ) ) ;
#48921=CARTESIAN_POINT ( 'NONE',  ( 84.72546926745363294, 19.84015517905186599, -62.89578937353809351 ) ) ;
#48922=CARTESIAN_POINT ( 'NONE',  ( 102.8837474253813014, 26.71671612110911553, 89.31275824274561614 ) ) ;
#48923=CARTESIAN_POINT ( 'NONE',  ( -144.9417090887490360, 61.69631066549397502, 59.11060452198194781 ) ) ;
#48925=CARTESIAN_POINT ( 'NONE',  ( -24.18270484670773612, 9.527492911955590671, -40.85707012195633325 ) ) ;
#48926=CARTESIAN_POINT ( 'NONE',  ( -48.70883077256302585, 14.10659259062419046, -73.56901164759405276 ) ) ;
#48928=CARTESIAN_POINT ( 'NONE',  ( -118.7011544766493500, 43.11604763363182968, -13.42784816232486733 ) ) ;
#48931=CARTESIAN_POINT ( 'NONE',  ( 38.43102714813442589, 9.298961820315048143, 56.80533550196272330 ) ) ;
#48932=CARTESIAN_POINT ( 'NONE',  ( 176.0745160362857860, 73.68684431790050837, 69.23986300298068386 ) ) ;
#48935=CARTESIAN_POINT ( 'NONE',  ( -166.3231866619663606, 81.31146386205588783, -12.18699256254814500 ) ) ;
#48936=DIRECTION ( 'NONE',  ( -0.000000000000000000, 1.000000000000000000, -0.000000000000000000 ) ) ;
#48939=AXIS2_PLACEMENT_3D ( 'NONE', #18362, #1487, #66571 ) ;
#48940=CARTESIAN_POINT ( 'NONE',  ( 187.8973304652193690, 87.27378997243177139, -20.02744225065407946 ) ) ;
#48941=CARTESIAN_POINT ( 'NONE',  ( 210.6584452238134872, 116.7138338345754249, 5.284484997206956969 ) ) ;
#48942=CARTESIAN_POINT ( 'NONE',  ( -85.33861794503827980, 26.06603235258742401, -92.87200205917845608 ) ) ;
#48943=CARTESIAN_POINT ( 'NONE',  ( -102.2801239173131194, -170.0000000000000000, 72.36362509687883460 ) ) ;
#48947=CARTESIAN_POINT ( 'NONE',  ( -57.65733424639443427, 15.39521790791522982, -35.67890556914403533 ) ) ;
#48952=CYLINDRICAL_SURFACE ( 'NONE', #8801, 7.500000000000020428 ) ;
#48953=DIRECTION ( 'NONE',  ( -0.000000000000000000, 1.000000000000000000, -0.000000000000000000 ) ) ;
#48954=CARTESIAN_POINT ( 'NONE',  ( 86.62931800182293784, -170.0000000000000000, 29.71208757247930521 ) ) ;
#48956=CARTESIAN_POINT ( 'NONE',  ( 80.34841469379381351, -170.0000000000000000, 94.99999999999866418 ) ) ;
#48958=B_SPLINE_CURVE_WITH_KNOTS ( 'NONE', 3,
 ( #23946, #2493, #66875, #7069, #40126, #34517, #28527, #54895, #61582, #66187, #49614, #34164, #13058, #50335, #1807, #23261 ),
 .UNSPECIFIED., .F., .F.,
 ( 4, 2, 2, 2, 2, 2, 2, 4 ),
 ( 0.01012072446094006324, 0.01138741587173669988, 0.01265410728253333825, 0.01392079869332997488, 0.01518749010412661152, 0.01645418151492324815, 0.01772087292571988479, 0.02025425574731319622 ),
 .UNSPECIFIED. ) ;
#48959=ORIENTED_EDGE ( 'NONE', *, *, #61956, .T. ) ;
#48961=EDGE_CURVE ( 'NONE', #8644, #21982, #5710, .T. ) ;
#48962=ADVANCED_FACE ( 'NONE', ( #5708 ), #6415, .T. ) ;
#48969=CARTESIAN_POINT ( 'NONE',  ( 110.2429982417149290, 28.88204397445231209, 29.61121420573730489 ) ) ;
#48970=ORIENTED_EDGE ( 'NONE', *, *, #28421, .T. ) ;
#48972=CARTESIAN_POINT ( 'NONE',  ( -56.72814287166055891, 15.13700122306437379, -62.24644308817313743 ) ) ;
#48975=CARTESIAN_POINT ( 'NONE',  ( 160.9099843287284557, 61.67000084894967671, 30.22885540498834800 ) ) ;
#48976=CARTESIAN_POINT ( 'NONE',  ( 109.3154830994003390, 29.56170298203816316, 2.809493426657196480 ) ) ;
#48979=CARTESIAN_POINT ( 'NONE',  ( -47.61402178322639855, 13.84598486314981614, -43.70512311542479011 ) ) ;
#48982=CARTESIAN_POINT ( 'NONE',  ( 8.767814708128309320, 7.383611927972574485, 34.86454251663690940 ) ) ;
#48983=CARTESIAN_POINT ( 'NONE',  ( 69.71320131704045764, 14.32603187575852921, -93.43281573010639818 ) ) ;
#48984=CARTESIAN_POINT ( 'NONE',  ( 79.12222162355536170, 16.99473220795134054, 90.79787899594637679 ) ) ;
#48989=EDGE_CURVE ( 'NONE', #8166, #31066, #16613, .T. ) ;
#48991=ORIENTED_EDGE ( 'NONE', *, *, #64567, .T. ) ;
#48992=CARTESIAN_POINT ( 'NONE',  ( -12.78015296493258113, 7.264294661536299103, -10.42199259816774060 ) ) ;
#48993=CARTESIAN_POINT ( 'NONE',  ( -51.34325167237330589, 13.71819364263221530, 44.34027758300791078 ) ) ;
#48998=CARTESIAN_POINT ( 'NONE',  ( -60.47589866267036030, 17.25153113855769149, -47.90273905312907488 ) ) ;
#49003=AXIS2_PLACEMENT_3D ( 'NONE', #18688, #49279, #66544 ) ;
#49006=EDGE_LOOP ( 'NONE', ( #56761, #31516, #10212, #39153 ) ) ;
#49009=CARTESIAN_POINT ( 'NONE',  ( -26.69138721373299106, 9.876636144558636587, 85.59062689267271651 ) ) ;
#49010=CARTESIAN_POINT ( 'NONE',  ( -96.78198318406110445, 30.07417864442862410, -47.63888010278168395 ) ) ;
#49011=CARTESIAN_POINT ( 'NONE',  ( -109.7078892845591582, 36.71702188566221281, 12.24582890309084071 ) ) ;
#49012=CARTESIAN_POINT ( 'NONE',  ( 21.73827885904430346, 6.764046335627707407, 32.94214015723378708 ) ) ;
#49013=CARTESIAN_POINT ( 'NONE',  ( 134.3135005523731991, 42.87884033955812413, -24.16835682549730535 ) ) ;
#49019=CARTESIAN_POINT ( 'NONE',  ( 31.90247004928965069, 8.563336936370820496, -43.62320764982623444 ) ) ;
#49020=B_SPLINE_CURVE_WITH_KNOTS ( 'NONE', 3,
 ( #6068, #27530, #1774, #44681, #7399, #28857, #2124, #23577, #66500, #69412, #25316, #45721, #67197, #9127, #29197, #29530, #46056, #13369, #3496, #29888, #52030, #62935, #68222, #18639, #14408, #24966, #24621, #56266, #51000, #2811, #51689, #46397, #20030, #41483, #34492, #35859, #62235, #24274, #67877, #8083, #50643, #7748, #40099, #67527 ),
 .UNSPECIFIED., .F., .F.,
 ( 4, 2, 2, 2, 2, 2, 2, 2, 2, 2, 2, 2, 2, 2, 2, 2, 2, 2, 2, 2, 2, 4 ),
 ( 0.000000000000000000, 0.001487235713946833890, 0.002230853570920231319, 0.002974471427893629616, 0.004461707141840403658, 0.005948942855787178567, 0.007436178569733952609, 0.008179796426707356544, 0.008923414283680760478, 0.01041064999762751457, 0.01189788571157426693, 0.01264150356854762229, 0.01338512142552098112, 0.01487235713946772307, 0.01561597499644110446, 0.01635959285341448410, 0.01784682856736124340, 0.01933406428130800270, 0.02007768213828138235, 0.02082129999525476199, 0.02230853570920153170, 0.02379577142314830140 ),
 .UNSPECIFIED. ) ;
#49021=CARTESIAN_POINT ( 'NONE',  ( -38.93878980550034896, 10.94326053663842124, 65.05816493757461672 ) ) ;
#49022=CARTESIAN_POINT ( 'NONE',  ( 204.6977192012829505, 108.0580384837234931, 56.05227132923312183 ) ) ;
#49023=VERTEX_POINT ( 'NONE', #10990 ) ;
#49025=LINE ( 'NONE', #22318, #65239 ) ;
#49028=CARTESIAN_POINT ( 'NONE',  ( 102.7551177910568470, 25.56939188780863503, 9.769129899803088435 ) ) ;
#49029=CYLINDRICAL_SURFACE ( 'NONE', #16278, 7.500000000000020428 ) ;
#49033=CARTESIAN_POINT ( 'NONE',  ( 13.36262230781614946, 7.441298897118792333, 17.78385849237590222 ) ) ;
#49035=ORIENTED_EDGE ( 'NONE', *, *, #68306, .T. ) ;
#49036=AXIS2_PLACEMENT_3D ( 'NONE', #42474, #62905, #4503 ) ;
#49040=CARTESIAN_POINT ( 'NONE',  ( -133.1527834403230202, 51.46311219732124442, -40.50885773641505239 ) ) ;
#49041=CARTESIAN_POINT ( 'NONE',  ( 39.89571693415783926, 8.473773298340393723, -62.46436805589144114 ) ) ;
#49042=CARTESIAN_POINT ( 'NONE',  ( 59.30258796551118650, 12.87111270082601067, -76.60025956098559163 ) ) ;
#49043=EDGE_LOOP ( 'NONE', ( #47249, #14911, #59774, #5892 ) ) ;
#49045=VECTOR ( 'NONE', #27482, 1000.000000000000000 ) ;
#49046=ORIENTED_EDGE ( 'NONE', *, *, #68617, .F. ) ;
#49050=EDGE_LOOP ( 'NONE', ( #11969, #66313, #33378, #67180 ) ) ;
#49052=VERTEX_POINT ( 'NONE', #42987 ) ;
#49053=CARTESIAN_POINT ( 'NONE',  ( 177.7960900018545374, 75.34533826015463376, -36.98054387538336130 ) ) ;
#49057=CARTESIAN_POINT ( 'NONE',  ( 116.0963032583228198, 32.80867113471309438, 59.24019559371290455 ) ) ;
#49059=CARTESIAN_POINT ( 'NONE',  ( 134.0849965622594198, 42.73957449886185600, 56.35489142945906593 ) ) ;
#49060=CARTESIAN_POINT ( 'NONE',  ( -73.63346300764936814, 20.46798018699518096, -48.18129300630896239 ) ) ;
#49062=CARTESIAN_POINT ( 'NONE',  ( -95.04120270830171080, 29.25306318840326369, 40.04767500533338875 ) ) ;
#49063=CARTESIAN_POINT ( 'NONE',  ( 89.22118407503259618, 20.32164250407898365, -36.27957951410743220 ) ) ;
#49064=CARTESIAN_POINT ( 'NONE',  ( -47.55256438668344998, 13.83151366677316396, -16.11397663407440817 ) ) ;
#49066=CARTESIAN_POINT ( 'NONE',  ( 8.000000000000007105, 249.8719672152120381, 94.99999999999866418 ) ) ;
#49068=CARTESIAN_POINT ( 'NONE',  ( -148.6471085600700235, 64.76880961642447687, -49.77594517346916803 ) ) ;
#49070=CARTESIAN_POINT ( 'NONE',  ( -132.9606448460427828, 51.32627791221455027, 94.40546275677576205 ) ) ;
#49072=CARTESIAN_POINT ( 'NONE',  ( 60.61895554631706773, 13.15982272268127673, 17.59165741550849660 ) ) ;
#49073=ORIENTED_EDGE ( 'NONE', *, *, #18989, .T. ) ;
#49074=CARTESIAN_POINT ( 'NONE',  ( -132.2352756077770835, 50.81350938245623183, 34.10723656463518694 ) ) ;
#49078=ADVANCED_FACE ( 'NONE', ( #43683 ), #48952, .F. ) ;
#49080=CARTESIAN_POINT ( 'NONE',  ( 80.72161230109726660, 17.48902961068030848, -21.12390682281932186 ) ) ;
#49082=CARTESIAN_POINT ( 'NONE',  ( 93.61951000632930686, 21.92572933971849025, -72.89543003249312392 ) ) ;
#49083=CARTESIAN_POINT ( 'NONE',  ( -95.52163045714286227, 29.47808868198297105, 7.913069298181163447 ) ) ;
#49086=VERTEX_POINT ( 'NONE', #33154 ) ;
#49087=VECTOR ( 'NONE', #50447, 1000.000000000000000 ) ;
#49088=CARTESIAN_POINT ( 'NONE',  ( 40.38414441725699788, 8.538832720399534892, 44.86554498887630160 ) ) ;
#49093=DIRECTION ( 'NONE',  ( -1.000000000000000000, 0.000000000000000000, 0.000000000000000000 ) ) ;
#49094=DIRECTION ( 'NONE',  ( -0.000000000000000000, 1.000000000000000000, -0.000000000000000000 ) ) ;
#49095=CARTESIAN_POINT ( 'NONE',  ( 41.80372346091801461, 9.750024116765239057, -36.01055466632809754 ) ) ;
#49096=CARTESIAN_POINT ( 'NONE',  ( 158.3595886390531859, 58.34525996025800509, -77.92900715080654095 ) ) ;
#49097=VERTEX_POINT ( 'NONE', #49654 ) ;
#49100=CARTESIAN_POINT ( 'NONE',  ( -11.57931195747592668, 7.164335452024274353, -36.40669791821974854 ) ) ;
#49103=CARTESIAN_POINT ( 'NONE',  ( -85.53818824935325438, 25.05912739833918934, -93.26644400273796975 ) ) ;
#49104=CARTESIAN_POINT ( 'NONE',  ( 39.40195752203892710, -170.0000000000000000, -43.11981746542777927 ) ) ;
#49105=CARTESIAN_POINT ( 'NONE',  ( 32.09610685027467269, 8.582590950734816815, 8.856186440854040498 ) ) ;
#49107=CARTESIAN_POINT ( 'NONE',  ( 115.8406869673190300, 32.68156040898470138, -92.10329871651862277 ) ) ;
#49114=CARTESIAN_POINT ( 'NONE',  ( -11.78188048797444942, 8.190559674012726887, 4.394732934608507335 ) ) ;
#49119=CARTESIAN_POINT ( 'NONE',  ( -102.7502407665687372, 33.01985383847077316, -61.85912785543960268 ) ) ;
#49120=CARTESIAN_POINT ( 'NONE',  ( 89.81441025544566514, 21.60030303444519717, 84.07925712847533362 ) ) ;
#49122=EDGE_LOOP ( 'NONE', ( #15759, #49930 ) ) ;
#49123=B_SPLINE_CURVE_WITH_KNOTS ( 'NONE', 3,
 ( #36699, #57117, #57799, #52175, #3995, #8930, #63774, #58146, #15586, #30377, #57455, #9963, #68689, #58473, #41621, #4344, #68364, #9267, #46195, #19470, #62740, #25802, #47231, #67675, #40929, #41966, #52846, #9619, #63427, #26135, #37035, #15234, #51828, #10286, #31416, #3638, #41281, #4668, #46545, #25113, #31752, #47569, #68022, #14544, #69025, #25463 ),
 .UNSPECIFIED., .F., .F.,
 ( 4, 2, 2, 2, 2, 2, 2, 2, 2, 2, 2, 2, 2, 2, 2, 2, 2, 2, 2, 2, 2, 2, 4 ),
 ( 0.02404638330965503529, 0.02555608299537562300, 0.02631093283823591686, 0.02706578268109621072, 0.02857548236681676027, 0.02933033220967704024, 0.03008518205253731675, 0.03159488173825786977, 0.03310458142397841586, 0.03385943126683869236, 0.03461428110969896887, 0.03612398079541951496, 0.03687883063827979147, 0.03763368048114007491, 0.03838853032400035142, 0.03914338016686062793, 0.04065307985258120177, 0.04216277953830176173, 0.04367247922402233556, 0.04518217890974290246, 0.04593702875260316509, 0.04669187859546342773, 0.04820157828118395993 ),
 .UNSPECIFIED. ) ;
#49126=CARTESIAN_POINT ( 'NONE',  ( -133.3392045760936639, 51.59583146030204404, 10.22114052722352362 ) ) ;
#49127=CARTESIAN_POINT ( 'NONE',  ( -165.7149569557576001, 80.68479365246973600, -40.99114865466042090 ) ) ;
#49128=CARTESIAN_POINT ( 'NONE',  ( -179.5391134141993348, 94.56797110730775557, 88.11752450009484505 ) ) ;
#49129=ORIENTED_EDGE ( 'NONE', *, *, #63614, .F. ) ;
#49130=CARTESIAN_POINT ( 'NONE',  ( -122.3963566076408398, 44.23346594671849630, -49.06497968827187606 ) ) ;
#49133=CARTESIAN_POINT ( 'NONE',  ( -4.071369321747694947, 7.682719369516284758, -63.25129218461325564 ) ) ;
#49137=ORIENTED_EDGE ( 'NONE', *, *, #17137, .F. ) ;
#49139=CARTESIAN_POINT ( 'NONE',  ( 200.4600337307565781, 100.7087439352121123, -37.62052402236275128 ) ) ;
#49142=CARTESIAN_POINT ( 'NONE',  ( -94.77890319529976182, 30.24118571794803856, 37.51899750598869332 ) ) ;
#49143=LINE ( 'NONE', #47855, #19083 ) ;
#49147=CARTESIAN_POINT ( 'NONE',  ( 175.0634607207819045, 74.11351956991632051, 68.13290361812578055 ) ) ;
#49149=ORIENTED_EDGE ( 'NONE', *, *, #4379, .T. ) ;
#49155=CARTESIAN_POINT ( 'NONE',  ( 164.6406716478537930, 63.44801348349338355, 34.69351737438754668 ) ) ;
#49157=CARTESIAN_POINT ( 'NONE',  ( -77.02112161466365592, 22.77583432622785153, -35.29432619449520558 ) ) ;
#49159=DIRECTION ( 'NONE',  ( -0.000000000000000000, 1.000000000000000000, -0.000000000000000000 ) ) ;
#49160=CARTESIAN_POINT ( 'NONE',  ( -37.79601571721867259, 10.72155118426296383, -11.98514248803286897 ) ) ;
#49161=CARTESIAN_POINT ( 'NONE',  ( 151.2875339161446107, 52.99901520459633986, -93.04759937140129011 ) ) ;
#49162=CARTESIAN_POINT ( 'NONE',  ( -37.07602570886410831, 10.58457435034603122, -74.63365721006658760 ) ) ;
#49163=CARTESIAN_POINT ( 'NONE',  ( 22.89270809252619898, 7.840160460323052583, 66.77530781516593095 ) ) ;
#49166=ORIENTED_EDGE ( 'NONE', *, *, #56528, .F. ) ;
#49173=CARTESIAN_POINT ( 'NONE',  ( -126.3508039230932809, 46.79479538767116509, 72.46449846362081360 ) ) ;
#49174=CARTESIAN_POINT ( 'NONE',  ( -61.26024128027892601, 17.48385755755500170, 87.28489753407048113 ) ) ;
#49176=CARTESIAN_POINT ( 'NONE',  ( 82.13067365723600233, 17.93447087949266816, 58.03607088492858423 ) ) ;
#49180=ORIENTED_EDGE ( 'NONE', *, *, #23983, .T. ) ;
#49183=CARTESIAN_POINT ( 'NONE',  ( 188.5837490358995865, 86.53279111916963018, 36.49783236869197367 ) ) ;
#49184=B_SPLINE_CURVE_WITH_KNOTS ( 'NONE', 3,
 ( #13715, #3172, #8799, #8447, #56276, #30248, #13041, #24633, #40790, #8091, #51699, #3507, #67888, #19681, #66857, #67206, #50315, #14416, #18996, #35869, #57322, #28866, #2133, #23585, #45025, #18299, #39758, #50652, #2474, #23928, #18652, #40108, #61563, #13380, #34841, #4883 ),
 .UNSPECIFIED., .F., .F.,
 ( 4, 2, 2, 2, 2, 2, 2, 2, 2, 2, 2, 2, 2, 2, 2, 2, 2, 4 ),
 ( 0.000000000000000000, 0.001548367318450147691, 0.003096734636900295382, 0.004645101955350443290, 0.006193469273800590764, 0.007741836592250738239, 0.008516020251475821951, 0.009290203910700905662, 0.01083857122915107309, 0.01238693854760123877, 0.01393530586605140620, 0.01548367318450157362, 0.01703204050295174105, 0.01858040782140191194, 0.02012877513985207936, 0.02167714245830224679, 0.02322550977675241074, 0.02477387709520257816 ),
 .UNSPECIFIED. ) ;
#49189=CARTESIAN_POINT ( 'NONE',  ( -50.52927270563903761, 13.51486287463704805, 4.970287360925811804 ) ) ;
#49192=VECTOR ( 'NONE', #12332, 1000.000000000000000 ) ;
#49193=CARTESIAN_POINT ( 'NONE',  ( 160.9099843287284273, 61.67000084894965539, -77.14934695686636701 ) ) ;
#49200=ORIENTED_EDGE ( 'NONE', *, *, #64471, .T. ) ;
#49202=CARTESIAN_POINT ( 'NONE',  ( -24.95029760921699591, 9.631514785009940738, -73.43094535933371958 ) ) ;
#49204=CARTESIAN_POINT ( 'NONE',  ( 43.14669449386823175, 9.942681284149132992, 43.93040857229122764 ) ) ;
#49205=CARTESIAN_POINT ( 'NONE',  ( -25.35398647985413234, 8.671412257862233020, 60.16984811174116032 ) ) ;
#49207=CARTESIAN_POINT ( 'NONE',  ( -190.6985136298601731, 109.1272424661242582, 94.99999999999866418 ) ) ;
#49209=EDGE_LOOP ( 'NONE', ( #62616, #58086, #32298, #52785 ) ) ;
#49211=ORIENTED_EDGE ( 'NONE', *, *, #52096, .T. ) ;
#49212=DIRECTION ( 'NONE',  ( -0.000000000000000000, 1.000000000000000000, -0.000000000000000000 ) ) ;
#49214=CARTESIAN_POINT ( 'NONE',  ( 36.99999522780156980, 9.122638774496639513, -23.38445250925136065 ) ) ;
#49216=CARTESIAN_POINT ( 'NONE',  ( 57.39083379741713742, 11.43779987330584724, 59.17179337101942593 ) ) ;
#49223=ORIENTED_EDGE ( 'NONE', *, *, #66005, .T. ) ;
#49228=CARTESIAN_POINT ( 'NONE',  ( 141.2366329129481244, 46.06278879703611295, -71.73044966183998383 ) ) ;
#49234=CARTESIAN_POINT ( 'NONE',  ( -72.20490592113145567, 19.96451062593609294, 41.75807547809249343 ) ) ;
#49236=DIRECTION ( 'NONE',  ( 0.000000000000000000, -1.000000000000000000, 0.000000000000000000 ) ) ;
#49239=CARTESIAN_POINT ( 'NONE',  ( -145.5261806899006842, 60.87473129144525785, -75.51763515817562222 ) ) ;
#49240=CARTESIAN_POINT ( 'NONE',  ( 92.19920907511537678, 21.39700525884450144, 5.321486460283676223 ) ) ;
#49247=CARTESIAN_POINT ( 'NONE',  ( 36.77024545412684375, 9.095083943590518416, 30.38650154362253630 ) ) ;
#49248=CARTESIAN_POINT ( 'NONE',  ( -173.1211646369891355, 88.63826465341151106, -49.71195716475001092 ) ) ;
#49249=CARTESIAN_POINT ( 'NONE',  ( -132.9409505933031710, 51.31241517713429090, -18.18881852736828364 ) ) ;
#49256=B_SPLINE_CURVE_WITH_KNOTS ( 'NONE', 3,
 ( #65223, #48664, #32177, #44095, #505, #5437, #43746, #38485, #11745, #54656, #6483, #38850, #26890, #64525, #33578, #24058, #17741, #50089, #39535, #39198, #12112, #49719, #19112, #40567, #44817, #45498, #23009, #2259, #18085, #60987, #65943, #29672, #66983, #2950, #44461, #66296, #7179, #60639, #1548, #50438, #18425, #7539, #18775, #24409, #34624 ),
 .UNSPECIFIED., .F., .F.,
 ( 4, 2, 2, 2, 2, 2, 2, 2, 1, 2, 2, 2, 2, 2, 2, 2, 2, 2, 2, 2, 2, 2, 4 ),
 ( 0.000000000000000000, 0.001467747071934219147, 0.002201620607901326552, 0.002935494143868433957, 0.004403241215802653104, 0.005870988287736871383, 0.007338735359671084459, 0.008072608895638188828, 0.008806482431605295799, 0.009540355967572401036, 0.01027422950353950627, 0.01174197657547371675, 0.01247585011144082025, 0.01320972364740792375, 0.01467747071934213769, 0.01541134425530924119, 0.01614521779127634296, 0.01761296486321055343, 0.01908071193514476044, 0.01981458547111187088, 0.02054845900707897785, 0.02201620607901318832, 0.02348395315094740227 ),
 .UNSPECIFIED. ) ;
#49257=FACE_BOUND ( 'NONE', #53287, .T. ) ;
#49258=CARTESIAN_POINT ( 'NONE',  ( -2.866724795119718561, 6.618578306599220085, -64.11449573703076510 ) ) ;
#49260=CARTESIAN_POINT ( 'NONE',  ( -145.9181947914994737, 62.49417193455356312, -8.878911523042834375 ) ) ;
#49261=CARTESIAN_POINT ( 'NONE',  ( -31.43908319763709969, 9.591432048623762086, -62.16174795566551836 ) ) ;
#49264=CARTESIAN_POINT ( 'NONE',  ( 133.8566784816069344, 41.42467568809808398, 2.665790248531674678 ) ) ;
#49265=CARTESIAN_POINT ( 'NONE',  ( -152.5067928559255392, 66.76529500553621688, 4.487733889797546283 ) ) ;
#49266=CARTESIAN_POINT ( 'NONE',  ( -124.9970785861867455, 47.10847819093959998, -76.70786858315703682 ) ) ;
#49268=CARTESIAN_POINT ( 'NONE',  ( 113.8568724296587646, 30.58972477291341008, 3.677294227703742813 ) ) ;
#49269=CARTESIAN_POINT ( 'NONE',  ( 89.65730223173018487, 21.54473673261222899, -23.34280881699134369 ) ) ;
#49272=VERTEX_POINT ( 'NONE', #7476 ) ;
#49274=CARTESIAN_POINT ( 'NONE',  ( 82.34401416830213805, 19.05992892018825202, -76.32612924313528424 ) ) ;
#49276=CARTESIAN_POINT ( 'NONE',  ( -142.0227972901369071, 59.36121938936275200, 64.50888617194736696 ) ) ;
#49278=CARTESIAN_POINT ( 'NONE',  ( -25.07901552294942960, 9.649193085547777216, -38.83467625327824635 ) ) ;
#49279=DIRECTION ( 'NONE',  ( -0.000000000000000000, 1.000000000000000000, -0.000000000000000000 ) ) ;
#49281=CARTESIAN_POINT ( 'NONE',  ( -125.6703656163502529, 47.55170550253213690, -23.06915330777030704 ) ) ;
#49284=CARTESIAN_POINT ( 'NONE',  ( 181.0840389613909736, 80.03940679743415387, 71.15314469597512925 ) ) ;
#49287=CARTESIAN_POINT ( 'NONE',  ( 39.40195752203892710, 8.409560354027387774, -89.30891864635511013 ) ) ;
#49288=CARTESIAN_POINT ( 'NONE',  ( -166.3231866619664174, 81.31146386205591625, 68.34665920884295076 ) ) ;
#49289=CARTESIAN_POINT ( 'NONE',  ( -166.0031475600388831, 80.98114714564765393, -12.98692819457663106 ) ) ;
#49297=CARTESIAN_POINT ( 'NONE',  ( 105.4376736768159049, 27.81988511842609313, -49.18599103925714644 ) ) ;
#49298=CARTESIAN_POINT ( 'NONE',  ( -15.27748264047829352, 7.491388194171919146, 65.44047530913044852 ) ) ;
#49299=CARTESIAN_POINT ( 'NONE',  ( -84.54326985437107567, 24.64760594531648863, -11.08512233598886176 ) ) ;
#49301=CARTESIAN_POINT ( 'NONE',  ( 39.89571693415785347, 8.473773298340395499, -8.775266874964071206 ) ) ;
#49302=CARTESIAN_POINT ( 'NONE',  ( 212.1983751099433846, 117.2326047784727194, -16.84004950763299391 ) ) ;
#49303=FACE_BOUND ( 'NONE', #49918, .T. ) ;
#49304=CARTESIAN_POINT ( 'NONE',  ( -62.49130718206700408, 16.80297926264071151, -43.70676811772677439 ) ) ;
#49308=CARTESIAN_POINT ( 'NONE',  ( 91.49210130311620048, 22.20929244416437598, -37.60641575626819844 ) ) ;
#49310=CARTESIAN_POINT ( 'NONE',  ( -180.6158171975815776, 97.47361786002632300, 11.15276930330031036 ) ) ;
#49311=CARTESIAN_POINT ( 'NONE',  ( 212.1669304543882220, 119.0398299474538675, 62.85156645179986157 ) ) ;
#49314=LINE ( 'NONE', #44036, #14236 ) ;
#49316=CARTESIAN_POINT ( 'NONE',  ( 55.90910788310616653, 11.13585330978404109, 12.91588078479143498 ) ) ;
#49317=CARTESIAN_POINT ( 'NONE',  ( -58.96922974609609014, 15.76655591015168056, 58.26108731115323280 ) ) ;
#49322=CARTESIAN_POINT ( 'NONE',  ( 86.62931800182293784, 20.48449268398422163, -62.66611478937537782 ) ) ;
#49326=CARTESIAN_POINT ( 'NONE',  ( 38.42020198992003799, 8.283430712587438904, -23.72674118770138563 ) ) ;
#49327=CARTESIAN_POINT ( 'NONE',  ( 163.5944442552009548, 63.88381951184481267, 41.24633810883595686 ) ) ;
#49328=CARTESIAN_POINT ( 'NONE',  ( 105.4376736768159191, 27.81988511842610379, 4.503110141670216393 ) ) ;
#49329=CARTESIAN_POINT ( 'NONE',  ( 63.01563776193091826, 13.70579113808095073, 2.968410348757589468 ) ) ;
#49330=CARTESIAN_POINT ( 'NONE',  ( 87.11228333101212229, 19.58587579906928156, 44.71208757247933363 ) ) ;
#49331=CARTESIAN_POINT ( 'NONE',  ( 102.7938674513918471, 26.67851209377773003, -15.56664358664439085 ) ) ;
#49332=CARTESIAN_POINT ( 'NONE',  ( -47.55316895016326839, 13.83165595246916979, 11.47544540822512360 ) ) ;
#49334=CARTESIAN_POINT ( 'NONE',  ( -153.9466444020484062, 69.38783913630635425, -89.95288446847763453 ) ) ;
#49337=CARTESIAN_POINT ( 'NONE',  ( 93.72383014846688809, 21.96492462047006100, 88.44459928000046034 ) ) ;
#49342=CARTESIAN_POINT ( 'NONE',  ( -15.08468253268399906, 7.472949889606721463, -18.02137581700551294 ) ) ;
#49343=CARTESIAN_POINT ( 'NONE',  ( -165.7250372467519810, 80.69514495077957861, 93.26859561057739256 ) ) ;
#49344=CARTESIAN_POINT ( 'NONE',  ( -54.09522495088364735, 14.42642983673692392, -23.32612737743259146 ) ) ;
#49347=CARTESIAN_POINT ( 'NONE',  ( -36.00304714721387001, 11.40794940913595923, 70.53273267370495603 ) ) ;
#49349=CARTESIAN_POINT ( 'NONE',  ( -76.10397364431024414, 21.36211154336729834, -76.51270562591143687 ) ) ;
#49351=EDGE_CURVE ( 'NONE', #58864, #67205, #60573, .T. ) ;
#49352=VERTEX_POINT ( 'NONE', #57728 ) ;
#49355=ORIENTED_EDGE ( 'NONE', *, *, #69516, .F. ) ;
#49356=CARTESIAN_POINT ( 'NONE',  ( -148.6426892915312692, 64.76241938621078020, 18.87627064943540489 ) ) ;
#49357=CARTESIAN_POINT ( 'NONE',  ( -56.74702624633194858, 16.18586554270559219, -89.08696668261721641 ) ) ;
#49358=CARTESIAN_POINT ( 'NONE',  ( -27.47737346315476259, 9.991540138299660256, 85.02917570802463842 ) ) ;
#49360=CARTESIAN_POINT ( 'NONE',  ( -96.02415295709707266, 29.71480036090586196, -46.65887338834314590 ) ) ;
#49368=EDGE_CURVE ( 'NONE', #30571, #47754, #9190, .T. ) ;
#49371=DIRECTION ( 'NONE',  ( 0.000000000000000000, 0.000000000000000000, 1.000000000000000000 ) ) ;
#49372=CARTESIAN_POINT ( 'NONE',  ( 59.72526569420001863, 11.93313563009888689, -9.618805749340053168 ) ) ;
#49376=CARTESIAN_POINT ( 'NONE',  ( -48.33725449172840172, 12.98311179783358682, 34.44141564906372110 ) ) ;
#49378=CARTESIAN_POINT ( 'NONE',  ( 197.1979149960398274, 98.19687999752004259, 63.21691722051551920 ) ) ;
#49380=CARTESIAN_POINT ( 'NONE',  ( 186.6075385349484463, 85.85749512876287781, 58.55496012458434762 ) ) ;
#49381=CARTESIAN_POINT ( 'NONE',  ( -156.6819053601225846, 70.51177710383656461, 67.32408636767608812 ) ) ;
#49382=CARTESIAN_POINT ( 'NONE',  ( -0.5783162822156596716, 7.534184941292926929, -40.97127712057928051 ) ) ;
#49384=CARTESIAN_POINT ( 'NONE',  ( -165.7138623879809529, 79.24467249981147177, 12.69207250051168856 ) ) ;
#49386=FACE_BOUND ( 'NONE', #49122, .T. ) ;
#49388=CARTESIAN_POINT ( 'NONE',  ( 9.057575839850585453, 6.378493414438676901, -66.54567355087297642 ) ) ;
#49390=B_SPLINE_CURVE_WITH_KNOTS ( 'NONE', 3,
 ( #6859, #22689, #38516, #12145, #11422, #49053, #59963, #43780, #66327, #32893, #33606, #890, #55036, #12489, #11780, #33256, #54691, #33951, #34302, #54331, #55747, #28669, #6515, #28309, #27962, #49407, #39570, #1236, #23046, #44493, #65975, #55384, #1951, #23406, #18116, #61021, #57478, #68044, #35333, #61708, #67697, #25481, #13867, #46567 ),
 .UNSPECIFIED., .F., .F.,
 ( 4, 2, 2, 2, 2, 2, 2, 2, 2, 2, 2, 2, 2, 2, 2, 2, 2, 2, 2, 2, 2, 4 ),
 ( 0.000000000000000000, 0.003518733725596278391, 0.004398417156995355903, 0.005278100588394431247, 0.007037467451192647855, 0.007917150882591742281, 0.008796834313990836707, 0.01055620117678906893, 0.01231556803958730288, 0.01319525147098641986, 0.01407493490238553684, 0.01495461833378465208, 0.01583430176518376906, 0.01671398519658288603, 0.01759366862798200301, 0.01935303549078017105, 0.02111240235357833214, 0.02199208578497738667, 0.02287176921637643426, 0.02463113607917451903, 0.02639050294197260033, 0.02814986980477068509 ),
 .UNSPECIFIED. ) ;
#49394=CARTESIAN_POINT ( 'NONE',  ( -126.7989199172159545, 47.09198523267864545, -49.87294221663437099 ) ) ;
#49401=ORIENTED_EDGE ( 'NONE', *, *, #16102, .T. ) ;
#49403=CARTESIAN_POINT ( 'NONE',  ( -129.8649418364887538, 49.16412313266191347, -89.72624065702046892 ) ) ;
#49404=CARTESIAN_POINT ( 'NONE',  ( 187.4809559129425338, 85.32157829635528401, 94.42977490495529480 ) ) ;
#49407=CARTESIAN_POINT ( 'NONE',  ( 173.8575673535406168, 71.59843387604337295, -45.75285605104306086 ) ) ;
#49408=B_SPLINE_CURVE_WITH_KNOTS ( 'NONE', 3,
 ( #39882, #33923, #56067, #23381, #55006, #44820, #55718, #29330, #60297, #18088, #61343, #55360, #65584, #39540, #60994, #50781, #49376, #7542, #49724, #2602, #65948, #1553, #1206, #17745, #39201, #65552, #11720, #1176, #59551, #39173, #480, #48636, #17346, #123, #27907, #48993, #64502, #21579, #11368, #43380, #33193, #21928, #54266 ),
 .UNSPECIFIED., .F., .F.,
 ( 4, 2, 2, 2, 2, 2, 2, 2, 2, 2, 2, 2, 1, 2, 2, 2, 2, 2, 2, 2, 2, 4 ),
 ( 0.02390068823634510300, 0.02538837671117075492, 0.02613222094858358088, 0.02687606518599640684, 0.02836375366082204141, 0.02985144213564767945, 0.03059528637306050194, 0.03133913061047332443, 0.03282681908529898329, 0.03431450756012464909, 0.03580219603495030795, 0.03654604027236314084, 0.03728988450977597374, 0.03803372874718879970, 0.03877757298460163260, 0.04026526145942728452, 0.04175294993425293644, 0.04324063840907858836, 0.04398448264649141431, 0.04472832688390424027, 0.04621601535872986444, 0.04770370383355548860 ),
 .UNSPECIFIED. ) ;
#49409=CARTESIAN_POINT ( 'NONE',  ( 110.2429982417149432, 28.88204397445229432, 17.76666361527367499 ) ) ;
#49413=CARTESIAN_POINT ( 'NONE',  ( -71.96390573417176029, 19.88067451234327621, -39.21214165021154940 ) ) ;
#49416=CARTESIAN_POINT ( 'NONE',  ( -29.74902699556085039, 10.33856194202125778, -8.661514771972045779 ) ) ;
#49417=CARTESIAN_POINT ( 'NONE',  ( -48.23766733091049730, 13.99378332280058679, -12.73082205257937360 ) ) ;
#49419=CARTESIAN_POINT ( 'NONE',  ( 114.6632852039170984, 30.98120524556721023, -49.48624585975684198 ) ) ;
#49421=CARTESIAN_POINT ( 'NONE',  ( -142.0070007485041401, 59.34878529741516928, -42.58233384625039974 ) ) ;
#49423=CARTESIAN_POINT ( 'NONE',  ( -122.1008507185714080, 44.04671359203690884, 85.33186843359860063 ) ) ;
#49425=DIRECTION ( 'NONE',  ( -0.000000000000000000, 1.000000000000000000, -0.000000000000000000 ) ) ;
#49428=CYLINDRICAL_SURFACE ( 'NONE', #59292, 7.500000000000013323 ) ;
#49432=CARTESIAN_POINT ( 'NONE',  ( 84.74140601443112075, 18.78541996275572856, -9.214546398377361669 ) ) ;
#49433=CARTESIAN_POINT ( 'NONE',  ( 41.80869235728136601, 9.750404582811603049, 3.449047885945065062 ) ) ;
#49434=CARTESIAN_POINT ( 'NONE',  ( 86.62931800182293784, 19.42108912189596381, -77.66611478937542756 ) ) ;
#49440=CARTESIAN_POINT ( 'NONE',  ( 45.90128843543705983, 9.343910238294478532, 33.63887583473116649 ) ) ;
#49444=CARTESIAN_POINT ( 'NONE',  ( 207.8407634284391463, 112.5209879629464069, -37.00314380516740442 ) ) ;
#49445=CARTESIAN_POINT ( 'NONE',  ( -76.32456871438913026, 22.51591205926309769, -76.60115264913015665 ) ) ;
#49446=CARTESIAN_POINT ( 'NONE',  ( -105.4556185321791162, 34.42302275449793569, 71.67470424851612165 ) ) ;
#49447=CARTESIAN_POINT ( 'NONE',  ( -31.43908319763709969, 9.591432048623767415, -50.31719736520186359 ) ) ;
#49451=CARTESIAN_POINT ( 'NONE',  ( -24.61094659556678010, 9.585225265507405723, 13.98425489515978271 ) ) ;
#49459=CARTESIAN_POINT ( 'NONE',  ( -179.9997297618090784, 96.71425526203211120, 94.99999999999866418 ) ) ;
#49461=CARTESIAN_POINT ( 'NONE',  ( 115.2641405259299745, 32.39624275045399315, -91.52542046738727777 ) ) ;
#49463=CARTESIAN_POINT ( 'NONE',  ( 205.4975936689702110, 107.4441653241353691, 82.92102392413544010 ) ) ;
#49466=CARTESIAN_POINT ( 'NONE',  ( 56.28782924480456984, 12.23883190161851608, 67.50924629393880139 ) ) ;
#49467=CARTESIAN_POINT ( 'NONE',  ( 13.83281508467570831, 7.452090093180183672, -62.60602632425918301 ) ) ;
#49468=CARTESIAN_POINT ( 'NONE',  ( -78.66644367742111399, -170.0000000000000000, 11.07365054920946079 ) ) ;
#49471=CARTESIAN_POINT ( 'NONE',  ( 89.21443742848369141, 21.38598633305952390, 83.83068150208889335 ) ) ;
#49479=CARTESIAN_POINT ( 'NONE',  ( -132.2286325684322321, 52.04087929935080581, -38.39048859397041724 ) ) ;
#49481=CARTESIAN_POINT ( 'NONE',  ( -119.2682179969168175, 42.28333404791697347, -38.86063178010808628 ) ) ;
#49485=CARTESIAN_POINT ( 'NONE',  ( -142.4136725729621560, 58.38849625135428312, 94.36932141740047086 ) ) ;
#49489=CARTESIAN_POINT ( 'NONE',  ( 197.8436586345020203, 97.39326576892285914, -46.92396185645527140 ) ) ;
#49490=CARTESIAN_POINT ( 'NONE',  ( 164.6046919270428930, 64.73376589608267295, -95.00000000000133582 ) ) ;
#49491=CARTESIAN_POINT ( 'NONE',  ( 16.27765348919936983, 6.516472002017809295, -50.51894409868578606 ) ) ;
#49497=CARTESIAN_POINT ( 'NONE',  ( -120.8703893864066146, 43.27420333016311815, -90.52915191075125279 ) ) ;
#49498=DIRECTION ( 'NONE',  ( 0.000000000000000000, 0.000000000000000000, 1.000000000000000000 ) ) ;
#49499=CARTESIAN_POINT ( 'NONE',  ( -8.320534640989464492, 7.931748412542455995, -62.26262132240751157 ) ) ;
#49501=CARTESIAN_POINT ( 'NONE',  ( 157.9130201331580565, 57.99550255803046639, 29.40946747225336466 ) ) ;
#49512=ADVANCED_FACE ( 'NONE', ( #27083 ), #11956, .F. ) ;
#49514=CARTESIAN_POINT ( 'NONE',  ( -133.3799602664182657, 52.86209125874982107, 11.80555390119608994 ) ) ;
#49520=DIRECTION ( 'NONE',  ( -0.000000000000000000, 1.000000000000000000, -0.000000000000000000 ) ) ;
#49521=CARTESIAN_POINT ( 'NONE',  ( -190.6985136298601731, 109.1272424661242582, 7.126870892829554549 ) ) ;
#49526=CARTESIAN_POINT ( 'NONE',  ( -130.5740389938243027, 49.65308610043481252, 70.84463781538606497 ) ) ;
#49527=CARTESIAN_POINT ( 'NONE',  ( -71.27103490383372275, 20.70545763375146109, -14.49721781705724233 ) ) ;
#49529=CARTESIAN_POINT ( 'NONE',  ( 133.8566784816069628, 41.42467568809806977, 17.66579024853170310 ) ) ;
#49531=CARTESIAN_POINT ( 'NONE',  ( -173.1211646369891639, 87.12891641440852197, -88.40105834567665966 ) ) ;
#49534=ORIENTED_EDGE ( 'NONE', *, *, #45979, .T. ) ;
#49535=CARTESIAN_POINT ( 'NONE',  ( 188.2076037774874635, 86.11782719225436722, 34.44517487742668038 ) ) ;
#49539=CARTESIAN_POINT ( 'NONE',  ( -122.3759299995709711, 45.41285412136513600, 58.32378120899723228 ) ) ;
#49540=LINE ( 'NONE', #61162, #15424 ) ;
#49543=EDGE_LOOP ( 'NONE', ( #39288, #30512 ) ) ;
#49546=ORIENTED_EDGE ( 'NONE', *, *, #3724, .T. ) ;
#49550=CARTESIAN_POINT ( 'NONE',  ( -81.90266786693713641, 23.58030232261292625, 44.70113455631799582 ) ) ;
#49551=CARTESIAN_POINT ( 'NONE',  ( -31.43908319763709969, 10.61114334766716638, -77.16174795566554678 ) ) ;
#49552=CARTESIAN_POINT ( 'NONE',  ( 45.04506994399702080, 10.22854084020123899, 32.44892839504316839 ) ) ;
#49559=CARTESIAN_POINT ( 'NONE',  ( 33.46033188299904992, 8.722678254080102889, -20.85871202478321962 ) ) ;
#49563=CARTESIAN_POINT ( 'NONE',  ( -0.3732240621745017140, 7.527003275829102336, 65.43944316759959179 ) ) ;
#49565=B_SPLINE_CURVE_WITH_KNOTS ( 'NONE', 3,
 ( #26891, #149, #43055, #48665, #32864, #42036, #43405, #16679, #15309, #63843, #47641, #69100, #15650, #37101, #66298, #50778, #7181, #34269 ),
 .UNSPECIFIED., .F., .F.,
 ( 4, 2, 2, 2, 2, 2, 2, 2, 4 ),
 ( 0.01000416104488733443, 0.01126184431380911413, 0.01251952758273089383, 0.01377721085165267527, 0.01503489412057445497, 0.01629257738949623641, 0.01755026065841801611, 0.01880794392733979581, 0.02006562719626157551 ),
 .UNSPECIFIED. ) ;
#49570=AXIS2_PLACEMENT_3D ( 'NONE', #9431, #15049, #53004 ) ;
#49572=CARTESIAN_POINT ( 'NONE',  ( -118.8689810167775960, 42.03922634358559662, -71.89854666037425091 ) ) ;
#49574=ORIENTED_EDGE ( 'NONE', *, *, #41912, .T. ) ;
#49578=CARTESIAN_POINT ( 'NONE',  ( -131.8384800362509282, 51.76463137407609594, -91.50743145908269582 ) ) ;
#49582=DIRECTION ( 'NONE',  ( -0.000000000000000000, 1.000000000000000000, -0.000000000000000000 ) ) ;
#49584=CARTESIAN_POINT ( 'NONE',  ( -71.21970990337018748, 19.62334883444993139, 36.89203884133947042 ) ) ;
#49587=CARTESIAN_POINT ( 'NONE',  ( -144.9439644317224349, 60.40328483334190679, -75.11390089952729454 ) ) ;
#49588=CARTESIAN_POINT ( 'NONE',  ( 91.13361825170456143, 21.00701373666981553, 16.38409351591118934 ) ) ;
#49593=EDGE_CURVE ( 'NONE', #23015, #63135, #24919, .T. ) ;
#49594=CARTESIAN_POINT ( 'NONE',  ( 69.20653952489904270, 15.23397960627465686, 86.75553736170155616 ) ) ;
#49595=CARTESIAN_POINT ( 'NONE',  ( 35.44311777160620380, 8.940232499250166498, 43.78863461845804750 ) ) ;
#49596=CARTESIAN_POINT ( 'NONE',  ( -177.1514380519393512, 93.28180884530866024, -35.87169415068767364 ) ) ;
#49598=CARTESIAN_POINT ( 'NONE',  ( -133.3149301983942507, 51.57857650535022742, -14.45055437769056361 ) ) ;
#49600=CARTESIAN_POINT ( 'NONE',  ( 129.1381264900934696, 38.64720302602604107, -64.51794085108998900 ) ) ;
#49603=CARTESIAN_POINT ( 'NONE',  ( -149.0764453401867797, 65.13297611514538232, -76.65738112195568021 ) ) ;
#49607=CARTESIAN_POINT ( 'NONE',  ( -156.9262190792699414, 72.10659547035874084, -41.17427441558346857 ) ) ;
#49609=CARTESIAN_POINT ( 'NONE',  ( -180.4614954900548582, 97.28277348252829881, 63.59750393255907142 ) ) ;
#49614=CARTESIAN_POINT ( 'NONE',  ( -13.16282047539117173, 7.297462132103659016, -91.32137775416312309 ) ) ;
#49615=CARTESIAN_POINT ( 'NONE',  ( -149.9449619562961402, 64.55090813009799433, 3.876270649435375137 ) ) ;
#49618=CARTESIAN_POINT ( 'NONE',  ( -15.13464256769235661, 8.488509377255647692, 39.31406149208217471 ) ) ;
#49619=CARTESIAN_POINT ( 'NONE',  ( 113.4351684956570381, 30.38657459074491385, 3.463604245180824659 ) ) ;
#49622=CARTESIAN_POINT ( 'NONE',  ( -38.92718193365331558, 11.96647478777219753, 11.36126298385067201 ) ) ;
#49627=CARTESIAN_POINT ( 'NONE',  ( 82.14396250120411480, 18.99560174459420736, -76.18202846519534432 ) ) ;
#49628=CARTESIAN_POINT ( 'NONE',  ( 102.7352309018612573, 26.65364508785401298, 90.71718089035570642 ) ) ;
#49633=FACE_OUTER_BOUND ( 'NONE', #24722, .T. ) ;
#49634=CARTESIAN_POINT ( 'NONE',  ( -71.28077210551055032, 20.70883253687733117, -95.00000000000133582 ) ) ;
#49639=CARTESIAN_POINT ( 'NONE',  ( 178.1903523079566298, 75.72906488635186406, 56.72024832093088520 ) ) ;
#49640=CARTESIAN_POINT ( 'NONE',  ( 40.22957559924974191, 8.518286412483671910, -89.34336208694358561 ) ) ;
#49642=CARTESIAN_POINT ( 'NONE',  ( -165.7690020878297616, 80.74028011998674970, -16.87889564165705281 ) ) ;
#49643=CARTESIAN_POINT ( 'NONE',  ( 157.4703587214989398, -170.0000000000000000, -9.279633708673955539 ) ) ;
#49645=CARTESIAN_POINT ( 'NONE',  ( 106.0228389049370463, 28.07756796303168656, -49.62712291136129039 ) ) ;
#49646=CARTESIAN_POINT ( 'NONE',  ( 16.28382582968306735, 7.523443033994205997, -35.51894409868578606 ) ) ;
#49647=CARTESIAN_POINT ( 'NONE',  ( -79.62258606008205675, 22.68765733708495702, -23.22492150694771240 ) ) ;
#49650=CARTESIAN_POINT ( 'NONE',  ( 211.7451286015360665, 116.5372661580811524, -14.39814270739270974 ) ) ;
#49651=FACE_BOUND ( 'NONE', #7365, .T. ) ;
#49652=CARTESIAN_POINT ( 'NONE',  ( 158.3516718297675823, 59.61984652322052369, 56.29275500237260133 ) ) ;
#49654=CARTESIAN_POINT ( 'NONE',  ( 110.2429982417149290, 28.88204397445231209, 2.766663615273646570 ) ) ;
#49657=CARTESIAN_POINT ( 'NONE',  ( -50.52615126106342558, 14.55080735582893858, 58.66218285867929438 ) ) ;
#49658=CARTESIAN_POINT ( 'NONE',  ( 63.01563776193091826, 13.70579113808095073, -50.72069083216976537 ) ) ;
#49659=CARTESIAN_POINT ( 'NONE',  ( 210.0122310839191755, 115.7355030290287345, 68.86736864163312077 ) ) ;
#49663=EDGE_LOOP ( 'NONE', ( #370, #26895, #35001, #15174, #60561 ) ) ;
#49665=CARTESIAN_POINT ( 'NONE',  ( -56.02358673658414290, 14.94347049174936970, 57.20932295525945221 ) ) ;
#49668=VERTEX_POINT ( 'NONE', #8071 ) ;
#49670=CARTESIAN_POINT ( 'NONE',  ( -61.52761555060401832, 17.56359742150277015, -19.68907097625505997 ) ) ;
#49671=CARTESIAN_POINT ( 'NONE',  ( 102.8458551240039753, 25.60773946375956811, 35.84670615152459305 ) ) ;
#49674=EDGE_LOOP ( 'NONE', ( #50918, #59895, #67593, #1769 ) ) ;
#49676=CARTESIAN_POINT ( 'NONE',  ( 164.4761273435912017, 64.62485394454746768, 34.17979310171889296 ) ) ;
#49677=CARTESIAN_POINT ( 'NONE',  ( -155.1359377029286009, 70.46175948311804405, -64.17498559856824158 ) ) ;
#49678=CARTESIAN_POINT ( 'NONE',  ( 68.94309019697863050, 15.16533147648755531, 15.08993511401731880 ) ) ;
#49680=EDGE_CURVE ( 'NONE', #13609, #64426, #29520, .T. ) ;
#49681=CARTESIAN_POINT ( 'NONE',  ( -50.14440374537738876, 14.45628984983895116, -37.02434562548277341 ) ) ;
#49682=CARTESIAN_POINT ( 'NONE',  ( -48.58279704072702287, 14.07632445131079635, 14.77428691758652768 ) ) ;
#49683=CARTESIAN_POINT ( 'NONE',  ( -127.4644500646575409, 48.74852676951793740, -22.90636119001569071 ) ) ;
#49691=ORIENTED_EDGE ( 'NONE', *, *, #4703, .F. ) ;
#49692=CARTESIAN_POINT ( 'NONE',  ( -9.525868120571905351, 7.007646177566257073, -8.764757431761587725 ) ) ;
#49693=DIRECTION ( 'NONE',  ( -0.000000000000000000, 1.000000000000000000, -0.000000000000000000 ) ) ;
#49694=CARTESIAN_POINT ( 'NONE',  ( -55.05276343752909440, 14.68156374112637330, -8.371773407996169425 ) ) ;
#49695=CARTESIAN_POINT ( 'NONE',  ( 104.7147873368644753, 26.40702926859712463, -11.48552898774475572 ) ) ;
#49696=CARTESIAN_POINT ( 'NONE',  ( -57.89360529881253825, 16.50663720601370699, -35.76264078408507174 ) ) ;
#49699=CARTESIAN_POINT ( 'NONE',  ( -15.15117926080556465, -170.0000000000000000, -95.00000000000133582 ) ) ;
#49707=CARTESIAN_POINT ( 'NONE',  ( -56.11927569309192876, 16.01314504639333336, -88.97860608119357551 ) ) ;
#49708=CARTESIAN_POINT ( 'NONE',  ( -23.93408125862919178, 9.494352577851083552, 91.57808385503631143 ) ) ;
#49710=VECTOR ( 'NONE', #35450, 1000.000000000000000 ) ;
#49714=ORIENTED_EDGE ( 'NONE', *, *, #49368, .F. ) ;
#49716=ORIENTED_EDGE ( 'NONE', *, *, #49945, .F. ) ;
#49717=AXIS2_PLACEMENT_3D ( 'NONE', #42470, #31927, #63931 ) ;
#49719=CARTESIAN_POINT ( 'NONE',  ( -15.32520546926283167, 7.495995523981875408, 11.26390656212526586 ) ) ;
#49720=CARTESIAN_POINT ( 'NONE',  ( 32.14349651933088126, 7.576119504381664704, -71.91552036636386447 ) ) ;
#49722=CARTESIAN_POINT ( 'NONE',  ( 62.04664474957769471, 12.44961624115901522, -8.923359081094497824 ) ) ;
#49724=CARTESIAN_POINT ( 'NONE',  ( -47.80193682758675067, 12.85650137125658077, 35.83676103695687232 ) ) ;
#49727=CARTESIAN_POINT ( 'NONE',  ( 184.9757174666827382, 84.09845285279332927, 57.23800133820973457 ) ) ;
#49728=CARTESIAN_POINT ( 'NONE',  ( 177.5945652320814077, 75.14951358071814980, -63.92694727933915999 ) ) ;
#49730=CARTESIAN_POINT ( 'NONE',  ( -1.096061481932295578, 7.553048580900441067, -46.23872224921927199 ) ) ;
#49732=CARTESIAN_POINT ( 'NONE',  ( -172.7154982671752634, 86.67743928531943709, 3.977144016177345254 ) ) ;
#49734=FACE_BOUND ( 'NONE', #46615, .T. ) ;
#49738=CARTESIAN_POINT ( 'NONE',  ( -129.3963145237380843, 48.84337839101543466, -62.62225689922211558 ) ) ;
#49740=CARTESIAN_POINT ( 'NONE',  ( 43.14356474118744700, 8.925336319666881124, -76.48306521520852641 ) ) ;
#49741=LINE ( 'NONE', #39564, #19807 ) ;
#49743=EDGE_CURVE ( 'NONE', #15400, #23050, #41123, .T. ) ;
#49746=CARTESIAN_POINT ( 'NONE',  ( 187.5458047452486312, 85.39230033703691447, 86.67446375648381718 ) ) ;
#49747=VERTEX_POINT ( 'NONE', #57304 ) ;
#49748=ADVANCED_FACE ( 'NONE', ( #8428 ), #36193, .F. ) ;
#49754=EDGE_LOOP ( 'NONE', ( #20637, #60237 ) ) ;
#49757=CARTESIAN_POINT ( 'NONE',  ( -76.77329340382466683, 21.60914066444071935, -35.34250697107755457 ) ) ;
#49760=CARTESIAN_POINT ( 'NONE',  ( 89.88695630745277754, 20.55793566325391453, -36.54904141640419368 ) ) ;
#49762=CARTESIAN_POINT ( 'NONE',  ( -48.70883077256303295, 14.10659259062419224, -19.87991046666667216 ) ) ;
#49766=VECTOR ( 'NONE', #61528, 1000.000000000000000 ) ;
#49768=CARTESIAN_POINT ( 'NONE',  ( -122.7930600691578178, 44.48546375740914272, -8.724487278797921519 ) ) ;
#49770=CARTESIAN_POINT ( 'NONE',  ( -76.10382222627279702, 22.43453174720078991, 18.12638239063526413 ) ) ;
#49771=CARTESIAN_POINT ( 'NONE',  ( -142.3187766126154941, 59.59460822661996815, -44.52240461455945564 ) ) ;
#49774=CARTESIAN_POINT ( 'NONE',  ( -131.7960692854462081, 50.50475183506788568, 87.17087325982676305 ) ) ;
#49778=EDGE_CURVE ( 'NONE', #56227, #5626, #15686, .T. ) ;
#49781=CARTESIAN_POINT ( 'NONE',  ( 83.37782009939532202, 19.39546426214657515, 43.97496025697474664 ) ) ;
#49783=CARTESIAN_POINT ( 'NONE',  ( 185.5415406465189676, 83.23025870924408309, -22.93060259331669570 ) ) ;
#49784=CARTESIAN_POINT ( 'NONE',  ( 141.2894128405439460, 46.09731134920846785, -15.64124612904248579 ) ) ;
#49786=CARTESIAN_POINT ( 'NONE',  ( 89.22118407503259618, 20.32164250407901207, -63.12413010457111540 ) ) ;
#49788=CARTESIAN_POINT ( 'NONE',  ( -156.8685326950935064, 70.68337020863233988, -94.46790515003011990 ) ) ;
#49789=VERTEX_POINT ( 'NONE', #57991 ) ;
#49792=CARTESIAN_POINT ( 'NONE',  ( 44.34263167748004264, 9.103379693481564061, 31.75007173307530550 ) ) ;
#49799=CARTESIAN_POINT ( 'NONE',  ( 212.1488570093001726, 119.0116247937291547, -44.69745977012216542 ) ) ;
#49800=DIRECTION ( 'NONE',  ( -0.000000000000000000, 1.000000000000000000, -0.000000000000000000 ) ) ;
#49801=DIRECTION ( 'NONE',  ( -0.000000000000000000, 1.000000000000000000, -0.000000000000000000 ) ) ;
#49802=CARTESIAN_POINT ( 'NONE',  ( -27.70562707895080123, 9.007984652865424380, -49.34063250321889882 ) ) ;
#49805=CARTESIAN_POINT ( 'NONE',  ( -25.07901552294942604, 9.649193085547802085, 14.85442492764910583 ) ) ;
#49809=CARTESIAN_POINT ( 'NONE',  ( -86.13912425708386422, 25.31016616653309725, 90.88912426079336626 ) ) ;
#49811=CARTESIAN_POINT ( 'NONE',  ( 126.3554864210862121, 38.22801630372147486, 37.23830996261533954 ) ) ;
#49818=CARTESIAN_POINT ( 'NONE',  ( 212.1225368307689507, 117.1159163218940478, 91.47960818144875361 ) ) ;
#49821=CARTESIAN_POINT ( 'NONE',  ( 12.03162622199373466, 7.415834979634797541, -63.36749908192140879 ) ) ;
#49822=CARTESIAN_POINT ( 'NONE',  ( -8.320534640989469821, 7.931748412542455995, 18.27103044898354511 ) ) ;
#49826=CARTESIAN_POINT ( 'NONE',  ( -95.69827994653627457, 29.56114141562974140, -92.60069445672345978 ) ) ;
#49828=ORIENTED_EDGE ( 'NONE', *, *, #62967, .F. ) ;
#49831=CARTESIAN_POINT ( 'NONE',  ( -37.93983213483219430, 11.77368372188049150, -39.04474621805233880 ) ) ;
#49832=CARTESIAN_POINT ( 'NONE',  ( -168.1811549361197535, 83.25427431521138999, -47.86022128265202724 ) ) ;
#49833=CARTESIAN_POINT ( 'NONE',  ( -168.3771781763924196, 81.99782240093493613, 86.17408653350808834 ) ) ;
#49835=CARTESIAN_POINT ( 'NONE',  ( -121.5921196778231490, 43.72569502503146310, -48.57545037443222924 ) ) ;
#49836=FACE_OUTER_BOUND ( 'NONE', #63653, .T. ) ;
#49837=CARTESIAN_POINT ( 'NONE',  ( 204.6977192012829789, -170.0000000000000000, -24.48138044215792419 ) ) ;
#49838=CARTESIAN_POINT ( 'NONE',  ( -4.731197926646207641, 7.716745361328039898, -76.59901871495883086 ) ) ;
#49844=CARTESIAN_POINT ( 'NONE',  ( 197.3059626281005592, 96.72682679064189415, -42.51509034027653655 ) ) ;
#49846=CARTESIAN_POINT ( 'NONE',  ( 22.30016284075437127, 6.796348835713780012, -39.26592317429871315 ) ) ;
#49855=CARTESIAN_POINT ( 'NONE',  ( -74.79002408692173276, 20.88280597089420709, -9.345738677820531137 ) ) ;
#49857=CARTESIAN_POINT ( 'NONE',  ( -38.69882630632968556, 11.92152976277064624, -94.57351083330412678 ) ) ;
#49861=ORIENTED_EDGE ( 'NONE', *, *, #4841, .F. ) ;
#49862=CARTESIAN_POINT ( 'NONE',  ( 164.6499013411308283, 63.45576988183551492, 39.09533417168172065 ) ) ;
#49865=CARTESIAN_POINT ( 'NONE',  ( 157.4703587214989398, -170.0000000000000000, -97.31328548006501933 ) ) ;
#49868=CARTESIAN_POINT ( 'NONE',  ( -144.5610324426709496, 61.38759170201291226, -90.35978530201006720 ) ) ;
#49871=CARTESIAN_POINT ( 'NONE',  ( -34.74312654625183683, 10.15703162223799794, -22.71010778213880599 ) ) ;
#49872=CARTESIAN_POINT ( 'NONE',  ( -173.9617926765113509, 89.58633395456780590, 45.78627089199527944 ) ) ;
#49874=CARTESIAN_POINT ( 'NONE',  ( -132.9126122820979106, 52.52752252041128145, 8.618821758353476525 ) ) ;
#49875=CARTESIAN_POINT ( 'NONE',  ( 22.28700331106866628, 7.803633676228378668, 68.11117160914710666 ) ) ;
#49877=ORIENTED_EDGE ( 'NONE', *, *, #3701, .F. ) ;
#49880=CARTESIAN_POINT ( 'NONE',  ( 206.0512581537811911, 108.2133605824158025, -90.10690865741280220 ) ) ;
#49881=ADVANCED_FACE ( 'NONE', ( #59696 ), #31951, .T. ) ;
#49883=CARTESIAN_POINT ( 'NONE',  ( -109.7079446832838983, 37.86719386855315861, 10.10418760775352354 ) ) ;
#49884=DIRECTION ( 'NONE',  ( -0.000000000000000000, 1.000000000000000000, -0.000000000000000000 ) ) ;
#49885=CARTESIAN_POINT ( 'NONE',  ( -37.79823708645147207, 10.72197716414928870, -46.80106602748205091 ) ) ;
#49889=CARTESIAN_POINT ( 'NONE',  ( -131.6508182719824163, 50.40277850441008667, 60.13134880733180410 ) ) ;
#49890=CARTESIAN_POINT ( 'NONE',  ( -75.43495400358862923, 22.18831810339352728, -22.54335848465174408 ) ) ;
#49894=CARTESIAN_POINT ( 'NONE',  ( 37.00112095025830428, 8.109340230899356072, 44.52341621389895465 ) ) ;
#49900=CARTESIAN_POINT ( 'NONE',  ( 86.62931800182293784, 19.42108912189597092, 29.71208757247930521 ) ) ;
#49901=CARTESIAN_POINT ( 'NONE',  ( 163.7403496014743780, 64.00600007368873889, -74.59240683662380889 ) ) ;
#49905=VERTEX_POINT ( 'NONE', #22428 ) ;
#49909=ORIENTED_EDGE ( 'NONE', *, *, #27399, .F. ) ;
#49911=CARTESIAN_POINT ( 'NONE',  ( -9.525868120571907127, 7.007646177566256185, -62.45385861268897543 ) ) ;
#49912=CARTESIAN_POINT ( 'NONE',  ( 41.09759788073306908, 9.651672055033841957, 44.72369366750157837 ) ) ;
#49913=CARTESIAN_POINT ( 'NONE',  ( -28.35330809568272414, 9.105138953156460602, 71.40111999495567829 ) ) ;
#49916=ORIENTED_EDGE ( 'NONE', *, *, #21072, .T. ) ;
#49918=EDGE_LOOP ( 'NONE', ( #24246, #4552 ) ) ;
#49919=DIRECTION ( 'NONE',  ( 0.000000000000000000, 0.000000000000000000, 1.000000000000000000 ) ) ;
#49920=CARTESIAN_POINT ( 'NONE',  ( -190.6985136298601731, 109.1272424661242582, 94.99999999999866418 ) ) ;
#49921=AXIS2_PLACEMENT_3D ( 'NONE', #7714, #1737, #29500 ) ;
#49923=CARTESIAN_POINT ( 'NONE',  ( 141.0393956947250729, 47.13639180521968086, 88.51104251071252804 ) ) ;
#49928=VECTOR ( 'NONE', #41311, 1000.000000000000000 ) ;
#49930=ORIENTED_EDGE ( 'NONE', *, *, #27089, .F. ) ;
#49934=CARTESIAN_POINT ( 'NONE',  ( 63.01563776193091826, 12.67277567978498176, 56.65751152968497451 ) ) ;
#49935=CARTESIAN_POINT ( 'NONE',  ( -127.5408520446061118, 48.79957756518083301, -88.77401935478938810 ) ) ;
#49937=ORIENTED_EDGE ( 'NONE', *, *, #42584, .F. ) ;
#49940=CARTESIAN_POINT ( 'NONE',  ( 11.21653854975268949, 6.397128675385705954, 43.48040107386871966 ) ) ;
#49943=ADVANCED_FACE ( 'NONE', ( #48106 ), #69563, .F. ) ;
#49944=B_SPLINE_CURVE_WITH_KNOTS ( 'NONE', 3,
 ( #26446, #43289, #54184, #48553, #11283, #37327, #16222, #42273, #27465, #42943, #65117, #59123, #6005, #43639, #48909, #388, #10944, #15544, #5332, #20814, #58435, #32415, #53145, #59818, #4977, #22201, #63736, #47883, #69347, #36995, #42613, #15880, #58778, #32064, #26787, #53840, #67810, #54893, #44342, #66525, #62171, #1095, #40714, #17978, #3437, #33471 ),
 .UNSPECIFIED., .F., .F.,
 ( 4, 2, 2, 2, 2, 2, 2, 2, 2, 2, 2, 2, 2, 2, 2, 2, 2, 2, 2, 2, 2, 2, 4 ),
 ( 6.938893903907228378E-18, 0.003192770216278285802, 0.003990962770347853891, 0.004789155324417422414, 0.006385540432556558593, 0.007183732986626134055, 0.007981925540695709517, 0.009578310648834860441, 0.01037650320290445585, 0.01117469575697405126, 0.01197288831104364668, 0.01277108086511324209, 0.01436746597325243117, 0.01596385108139162373, 0.01676204363546120527, 0.01756023618953079027, 0.01835842874360037527, 0.01915662129766995680, 0.02075300640580914763, 0.02234939151394833845, 0.02394577662208752927, 0.02474396917615712468, 0.02554216173022672010 ),
 .UNSPECIFIED. ) ;
#49945=EDGE_CURVE ( 'NONE', #54901, #5523, #13942, .T. ) ;
#49946=VERTEX_POINT ( 'NONE', #7299 ) ;
#49947=CARTESIAN_POINT ( 'NONE',  ( -143.2471548081022945, 59.04577938365765988, -73.31919755755201606 ) ) ;
#49953=CARTESIAN_POINT ( 'NONE',  ( 63.36355093506870872, 13.78687103992073304, 83.50303152118553385 ) ) ;
#49954=CARTESIAN_POINT ( 'NONE',  ( 35.66087318222939473, 8.964867769223229033, 30.89476568492769459 ) ) ;
#49955=CIRCLE ( 'NONE', #11743, 243.4957430088094839 ) ;
#49956=CARTESIAN_POINT ( 'NONE',  ( 63.01563776193091826, 13.70579113808094895, 29.81296093922127710 ) ) ;
#49957=CARTESIAN_POINT ( 'NONE',  ( -130.1964689553233256, 49.39217932424205060, -9.408478371563832710 ) ) ;
#49958=CARTESIAN_POINT ( 'NONE',  ( 157.4703587214989113, 57.65129005721576050, 71.25401806271709404 ) ) ;
#49959=CARTESIAN_POINT ( 'NONE',  ( 15.78827728214693416, -170.0000000000000000, 64.35925826316893961 ) ) ;
#49960=ORIENTED_EDGE ( 'NONE', *, *, #15434, .T. ) ;
#49962=CARTESIAN_POINT ( 'NONE',  ( -142.9756886485677683, 60.11539876121631210, -72.85257420866612676 ) ) ;
#49965=CARTESIAN_POINT ( 'NONE',  ( -150.3831389294225573, 66.25266777263976792, -49.76475080778571680 ) ) ;
#49966=CARTESIAN_POINT ( 'NONE',  ( 110.2429982417149574, -170.0000000000000000, -16.57788697519001175 ) ) ;
#49969=CARTESIAN_POINT ( 'NONE',  ( -37.52119286077852678, 11.69341290629620467, 33.32117128371067594 ) ) ;
#49976=CARTESIAN_POINT ( 'NONE',  ( -47.80896875121164413, 12.85816703949531181, -67.60146438707388938 ) ) ;
#49977=CARTESIAN_POINT ( 'NONE',  ( 204.6977192012829789, 108.0580384837235073, 44.20772073876944575 ) ) ;
#49980=CARTESIAN_POINT ( 'NONE',  ( 116.9200705848630548, 32.09536795999726166, 13.72062155485845381 ) ) ;
#49981=CARTESIAN_POINT ( 'NONE',  ( 46.44475613279522008, 10.44930307940658309, -94.19703056843508193 ) ) ;
#49983=CARTESIAN_POINT ( 'NONE',  ( -101.3502439362134595, 33.43728945125133123, -49.97127150509140847 ) ) ;
#49987=CARTESIAN_POINT ( 'NONE',  ( 79.37778929114109872, 18.12554302172301846, -68.18717443657236288 ) ) ;
#49990=DIRECTION ( 'NONE',  ( -0.000000000000000000, 1.000000000000000000, -0.000000000000000000 ) ) ;
#49993=CARTESIAN_POINT ( 'NONE',  ( -121.1841775822198031, 44.65790002524553159, -21.42663191464236760 ) ) ;
#49997=CARTESIAN_POINT ( 'NONE',  ( 176.6258282025054029, 74.21441092921632787, 57.61756429977015159 ) ) ;
#49999=CARTESIAN_POINT ( 'NONE',  ( -165.9154624515710452, 80.89088623112733956, 67.26787457162097894 ) ) ;
#50000=CARTESIAN_POINT ( 'NONE',  ( -165.9121868482146454, 80.88751546905567125, -17.45774927130959142 ) ) ;
#50002=ORIENTED_EDGE ( 'NONE', *, *, #64880, .F. ) ;
#50003=CARTESIAN_POINT ( 'NONE',  ( 103.4725384926516938, 26.96797537091726937, -46.65885272433202147 ) ) ;
#50005=PLANE ( 'NONE',  #9899 ) ;
#50006=CARTESIAN_POINT ( 'NONE',  ( -80.55742067659895156, 23.05042616197511407, -23.04419711036395313 ) ) ;
#50008=CARTESIAN_POINT ( 'NONE',  ( 208.9781236209185806, 112.4006213943319636, -10.80618506829177505 ) ) ;
#50009=FACE_BOUND ( 'NONE', #46012, .T. ) ;
#50011=CARTESIAN_POINT ( 'NONE',  ( 163.1370549780983481, 63.50181104276883559, 58.81513812535254715 ) ) ;
#50015=VERTEX_POINT ( 'NONE', #2717 ) ;
#50020=EDGE_CURVE ( 'NONE', #34701, #39310, #13212, .T. ) ;
#50021=CARTESIAN_POINT ( 'NONE',  ( -49.13048465129991627, 14.20828170588043626, 69.29014951661490329 ) ) ;
#50022=CARTESIAN_POINT ( 'NONE',  ( -173.9526029538035914, 89.57590038685106038, 4.011525743166236779 ) ) ;
#50023=CARTESIAN_POINT ( 'NONE',  ( 207.8407634284391747, 112.5209879629464211, 70.37505855668734966 ) ) ;
#50024=CARTESIAN_POINT ( 'NONE',  ( 84.97343609940686804, 18.86260005312945864, -62.84732350933633427 ) ) ;
#50028=CARTESIAN_POINT ( 'NONE',  ( 58.09436971064712907, 11.58462396079456447, 16.14920760772560726 ) ) ;
#50030=CARTESIAN_POINT ( 'NONE',  ( -62.45356936877015386, 16.79156452995241011, 63.42059391416657377 ) ) ;
#50038=EDGE_CURVE ( 'NONE', #6692, #27030, #20269, .T. ) ;
#50043=CARTESIAN_POINT ( 'NONE',  ( 44.34689728705970424, 10.12166135033765357, 69.91849532475755780 ) ) ;
#50046=CARTESIAN_POINT ( 'NONE',  ( 66.30230369578302430, 14.49551544185122154, 3.722485516513172499 ) ) ;
#50049=B_SPLINE_CURVE_WITH_KNOTS ( 'NONE', 3,
 ( #65641, #17434, #24476, #45915, #3012, #68077, #40626, #56462, #13901, #14932, #25513, #57851, #41672, #40293, #46951, #67384, #63131, #51547, #8289, #62789, #36399, #46247, #9672, #35017, #31133, #29735, #68414, #51199, #67047, #19173, #56826, #20216, #4390, #3690, #19879, #8640, #62084, #52567, #35364, #25854, #30091, #18838, #3352, #61736, #51878, #24812 ),
 .UNSPECIFIED., .F., .F.,
 ( 4, 2, 2, 2, 2, 2, 2, 2, 2, 2, 2, 2, 2, 2, 2, 2, 2, 2, 2, 2, 2, 2, 4 ),
 ( 0.02420077021543439941, 0.02572112563160192794, 0.02648130333968567313, 0.02724148104776941831, 0.02876183646393687746, 0.02952201417202060876, 0.03028219188010434007, 0.03180254729627183391, 0.03332290271243931734, 0.03408308042052305559, 0.03484325812860678689, 0.03636361354477424951, 0.03712379125285798775, 0.03788396896094171212, 0.03864414666902545037, 0.03940432437710918168, 0.04092467979327663041, 0.04244503520944408609, 0.04396539062561154176, 0.04548574604177899744, 0.04624592374986270793, 0.04700610145794641842, 0.04852645687411387410 ),
 .UNSPECIFIED. ) ;
#50051=CARTESIAN_POINT ( 'NONE',  ( -14.35185884954381308, 7.404296649871966451, 94.99999999999866418 ) ) ;
#50052=CARTESIAN_POINT ( 'NONE',  ( -128.9843070188472609, 49.78011598923034597, -22.41800723653680905 ) ) ;
#50055=CARTESIAN_POINT ( 'NONE',  ( 86.34144820818993082, 19.32281591521217834, 83.39973882909016822 ) ) ;
#50058=ORIENTED_EDGE ( 'NONE', *, *, #2276, .F. ) ;
#50060=CARTESIAN_POINT ( 'NONE',  ( 46.42281973867198275, 9.426811321855158354, 13.21852725678505536 ) ) ;
#50061=CARTESIAN_POINT ( 'NONE',  ( -177.9905692847866590, 94.28020182061023036, 86.29945827821053683 ) ) ;
#50062=CARTESIAN_POINT ( 'NONE',  ( -51.78153763344961646, 13.82841714689605084, -22.63801217197542925 ) ) ;
#50063=CARTESIAN_POINT ( 'NONE',  ( 109.7774723066848566, 28.66666416591279187, -24.07788697519002596 ) ) ;
#50064=DIRECTION ( 'NONE',  ( -0.000000000000000000, 1.000000000000000000, -0.000000000000000000 ) ) ;
#50065=CARTESIAN_POINT ( 'NONE',  ( -60.66101049381765620, 17.30588917955502026, -37.71267411079076481 ) ) ;
#50066=LINE ( 'NONE', #39859, #7417 ) ;
#50068=CARTESIAN_POINT ( 'NONE',  ( -15.27748264047829529, 7.491388194171919146, 38.59592471866675112 ) ) ;
#50069=ORIENTED_EDGE ( 'NONE', *, *, #25667, .T. ) ;
#50071=DIRECTION ( 'NONE',  ( -0.000000000000000000, 1.000000000000000000, -0.000000000000000000 ) ) ;
#50074=CARTESIAN_POINT ( 'NONE',  ( -149.5074843970971017, 65.50121172469319220, 18.87627064943540134 ) ) ;
#50076=B_SPLINE_CURVE_WITH_KNOTS ( 'NONE', 3,
 ( #53981, #53645, #64562, #542, #16710, #37474, #47676, #47332, #184, #11087, #5469, #43439, #21640, #43094, #68790, #32550, #64916, #38168, #43783, #61025, #39231, #12493, #55040, #6153, #66668, #49057, #44846, #38520, #60328, #27614, #44129, #18468, #6519, #33955, #39916, #6863 ),
 .UNSPECIFIED., .F., .F.,
 ( 4, 2, 2, 2, 2, 2, 2, 2, 2, 2, 2, 2, 2, 2, 2, 2, 2, 4 ),
 ( 1.551583845779545699E-17, 0.001545474820159036195, 0.003090949640318056777, 0.004636424460477077576, 0.006181899280636097942, 0.007727374100795117440, 0.008500111510874630225, 0.009272848920954141275, 0.01081832374111319807, 0.01236379856127225660, 0.01390927338143131166, 0.01545474820159034937, 0.01700022302174938535, 0.01854569784190842133, 0.02009117266206745731, 0.02163664748222649675, 0.02318212230238552579, 0.02472759712254455136 ),
 .UNSPECIFIED. ) ;
#50077=CARTESIAN_POINT ( 'NONE',  ( -35.41028269237559556, 11.29952379634140769, 85.03514065792309395 ) ) ;
#50078=CARTESIAN_POINT ( 'NONE',  ( 114.6797682035589361, 32.10876583290006892, -22.64371918772569003 ) ) ;
#50082=FACE_OUTER_BOUND ( 'NONE', #43682, .T. ) ;
#50083=LINE ( 'NONE', #1912, #45324 ) ;
#50089=CARTESIAN_POINT ( 'NONE',  ( -14.92903005859421128, 7.458185427130748835, 13.18945556359724591 ) ) ;
#50091=DIRECTION ( 'NONE',  ( -0.9115451497320358198, 0.4112000000000002875, -0.000000000000000000 ) ) ;
#50092=B_SPLINE_CURVE_WITH_KNOTS ( 'NONE', 3,
 ( #66451, #27384, #23178, #1017, #39697, #38649, #12974, #1715, #23525, #12618, #60453, #22819, #43563, #33388, #1363, #7346, #17895, #38294, #54455, #6286, #44623, #65389, #60793, #55518, #12269, #27737, #54814, #17177, #44261, #48823, #39350, #28086, #6988, #28803, #28441, #49176, #50250, #2072, #22467, #34440, #44966, #65742, #55880, #43907, #60090 ),
 .UNSPECIFIED., .F., .F.,
 ( 4, 2, 2, 2, 2, 2, 2, 2, 2, 2, 2, 1, 2, 2, 2, 2, 2, 2, 2, 2, 2, 2, 4 ),
 ( 1.430489624538199204E-17, 0.001502898956853342561, 0.002254348435280008420, 0.003005797913706674280, 0.004508696870560044596, 0.005260146348986746885, 0.006011595827413450041, 0.007514494784266913599, 0.009017393741120378892, 0.01052029269797384245, 0.01127174217640059158, 0.01202319165482733897, 0.01277464113325408636, 0.01352609061168083202, 0.01502898956853428863, 0.01578043904696102562, 0.01653188852538776260, 0.01803478748224124004, 0.01953768643909471747, 0.02028913591752145099, 0.02104058539594818450, 0.02254348435280161683, 0.02404638330965504917 ),
 .UNSPECIFIED. ) ;
#50095=CARTESIAN_POINT ( 'NONE',  ( 197.9843579228224542, 99.18296459057401648, 66.90814327346225809 ) ) ;
#50096=ORIENTED_EDGE ( 'NONE', *, *, #36999, .F. ) ;
#50098=CARTESIAN_POINT ( 'NONE',  ( 197.8588046850312878, 99.02485934465606476, -67.57714079882474323 ) ) ;
#50100=CARTESIAN_POINT ( 'NONE',  ( -0.3732240621745021580, 7.527003275829101447, -41.93875919425514098 ) ) ;
#50101=CARTESIAN_POINT ( 'NONE',  ( -167.3055661520540696, 80.87982228118417538, -91.14224052605258919 ) ) ;
#50103=FACE_BOUND ( 'NONE', #64472, .T. ) ;
#50104=CARTESIAN_POINT ( 'NONE',  ( -189.3388110241866116, 107.2270502731164612, 90.85541177745594155 ) ) ;
#50105=EDGE_CURVE ( 'NONE', #41204, #52964, #8969, .T. ) ;
#50111=CARTESIAN_POINT ( 'NONE',  ( -131.1078488676298832, 50.02394948559179255, -63.86183002538741960 ) ) ;
#50112=CARTESIAN_POINT ( 'NONE',  ( -105.8683518445188412, 35.77995342500076958, -75.96225039305235782 ) ) ;
#50117=DIRECTION ( 'NONE',  ( -0.8160245890732938934, -0.5780171883497599028, 0.000000000000000000 ) ) ;
#50118=CARTESIAN_POINT ( 'NONE',  ( 181.8074882258020466, 79.33812234480652137, 83.01091592049938583 ) ) ;
#50119=ORIENTED_EDGE ( 'NONE', *, *, #48506, .T. ) ;
#50120=AXIS2_PLACEMENT_3D ( 'NONE', #48294, #65554, #66607 ) ;
#50123=CARTESIAN_POINT ( 'NONE',  ( 151.1700480242206766, 54.15904440870137648, 40.98678080714243066 ) ) ;
#50128=CIRCLE ( 'NONE', #29943, 243.4957430088094839 ) ;
#50129=CARTESIAN_POINT ( 'NONE',  ( -178.2427210808089342, 93.01567669683338124, 5.992848471648135167 ) ) ;
#50130=CARTESIAN_POINT ( 'NONE',  ( -75.43953471070999228, 21.11829282998124313, -49.40254329562629465 ) ) ;
#50134=CARTESIAN_POINT ( 'NONE',  ( -31.43908319763710679, 10.61114334766716283, -8.472646774738153752 ) ) ;
#50135=CARTESIAN_POINT ( 'NONE',  ( -48.23389383802710739, 13.99288361739331776, -19.00461935341500208 ) ) ;
#50139=CARTESIAN_POINT ( 'NONE',  ( -74.18622060908363380, 21.73430079572372975, 5.039450213261992495 ) ) ;
#50142=DIRECTION ( 'NONE',  ( -0.000000000000000000, 1.000000000000000000, -0.000000000000000000 ) ) ;
#50144=CARTESIAN_POINT ( 'NONE',  ( 83.60262962804350195, 18.41036205028015971, -50.18795455408093176 ) ) ;
#50146=CARTESIAN_POINT ( 'NONE',  ( -145.5261806899007127, 60.87473129144529338, 58.70511779414287190 ) ) ;
#50147=CARTESIAN_POINT ( 'NONE',  ( 84.74089592029041285, 19.84571403269344714, 29.94973715047667540 ) ) ;
#50148=CARTESIAN_POINT ( 'NONE',  ( -78.66644367742109978, 22.32174330031319442, 30.41820113967310490 ) ) ;
#50150=CARTESIAN_POINT ( 'NONE',  ( -119.5576859660651223, 42.46117483543970650, 60.94340854921288297 ) ) ;
#50152=CARTESIAN_POINT ( 'NONE',  ( -174.7903139851460139, 90.53182997092832807, -8.043439406538249514 ) ) ;
#50154=ORIENTED_EDGE ( 'NONE', *, *, #36771, .F. ) ;
#50155=ORIENTED_EDGE ( 'NONE', *, *, #12502, .T. ) ;
#50156=CARTESIAN_POINT ( 'NONE',  ( 45.49006904354233427, 9.279592366778889101, 33.02688758334598873 ) ) ;
#50157=CARTESIAN_POINT ( 'NONE',  ( 197.3054165770395514, 96.72615186924552688, -18.28925989677753350 ) ) ;
#50160=CARTESIAN_POINT ( 'NONE',  ( 210.9631450001600967, 117.1791136960929833, -47.98552383177344183 ) ) ;
#50162=CARTESIAN_POINT ( 'NONE',  ( -71.27103490383373696, 20.70545763375144688, -68.18631899798461404 ) ) ;
#50163=CARTESIAN_POINT ( 'NONE',  ( -104.1342612728951877, 33.73231160250195160, 57.58144852683274451 ) ) ;
#50164=CARTESIAN_POINT ( 'NONE',  ( -30.94753041835914686, 9.510749728915504519, -35.31719736520183517 ) ) ;
#50165=CARTESIAN_POINT ( 'NONE',  ( 164.7167608259061637, 63.51199216609074227, -72.42214042571447408 ) ) ;
#50167=ORIENTED_EDGE ( 'NONE', *, *, #22642, .T. ) ;
#50171=FACE_OUTER_BOUND ( 'NONE', #11614, .T. ) ;
#50173=CARTESIAN_POINT ( 'NONE',  ( 126.8114659053432263, 38.48351437375815465, 34.38739146146416203 ) ) ;
#50177=CARTESIAN_POINT ( 'NONE',  ( -97.88021438939448160, 31.71889184683104190, -9.577608110017886034 ) ) ;
#50179=CARTESIAN_POINT ( 'NONE',  ( 58.47885130911550533, 12.69429933094348684, 31.32040142421980278 ) ) ;
#50183=CARTESIAN_POINT ( 'NONE',  ( 55.77012379229940109, 12.13428856597101024, 66.11046144963563620 ) ) ;
#50187=CARTESIAN_POINT ( 'NONE',  ( 203.1420903260746229, 104.2307086582027438, 70.93374687166461001 ) ) ;
#50189=CARTESIAN_POINT ( 'NONE',  ( -96.89229402469325692, 30.12691466369447468, -90.96714292758291265 ) ) ;
#50194=CARTESIAN_POINT ( 'NONE',  ( -189.2739965869454011, 107.1373753350176656, -16.14596922345551278 ) ) ;
#50195=CARTESIAN_POINT ( 'NONE',  ( -38.92718193365330848, 11.96647478777219753, -42.32783819707668016 ) ) ;
#50196=CARTESIAN_POINT ( 'NONE',  ( -165.6404838346739155, 80.60836113891892296, -41.59413812189578863 ) ) ;
#50198=CARTESIAN_POINT ( 'NONE',  ( -166.7504005514883829, 80.30621656552872878, 88.03983344583103587 ) ) ;
#50199=VERTEX_POINT ( 'NONE', #10392 ) ;
#50200=CARTESIAN_POINT ( 'NONE',  ( -118.7011677090247161, 41.93687969120208692, -44.55502681419259403 ) ) ;
#50202=CARTESIAN_POINT ( 'NONE',  ( -142.3393481102175429, 58.33014244976923379, -17.69161782318237996 ) ) ;
#50203=CARTESIAN_POINT ( 'NONE',  ( -2.177337698256110787, 7.595833446947581002, -64.80389893477351393 ) ) ;
#50207=CARTESIAN_POINT ( 'NONE',  ( 161.9743715636469119, 62.54005768132974197, -91.30411002385437769 ) ) ;
#50208=CARTESIAN_POINT ( 'NONE',  ( 199.7278513351970446, 99.76879341361768638, -38.18984482819509196 ) ) ;
#50209=B_SPLINE_CURVE_WITH_KNOTS ( 'NONE', 3,
 ( #33687, #45262, #27689, #38600, #60042, #39646, #50548, #55117, #49130, #49835, #60748, #11861, #973, #1661, #33339, #2367, #23125, #7650, #22420, #50200, #44575, #66052, #17847, #29101, #12568, #54408, #61104, #54764, #1314, #55469, #28041, #49481, #7292, #12927, #55830, #66748, #18539, #39991, #61450, #31762, #69030, #67097, #53194, #26143, #5022, #24172 ),
 .UNSPECIFIED., .F., .F.,
 ( 4, 2, 2, 2, 2, 2, 2, 2, 2, 2, 2, 2, 2, 2, 2, 2, 2, 2, 2, 2, 2, 2, 4 ),
 ( 0.02584318557310393699, 0.02743529570732771566, 0.02823135077443958418, 0.02902740584155144923, 0.03061951597577517933, 0.03221162610999891290, 0.03380373624422264300, 0.03459979131133449071, 0.03539584637844634535, 0.03619190144555819305, 0.03698795651267004075, 0.03858006664689374310, 0.03937612171400560468, 0.04017217678111746626, 0.04096823184822932784, 0.04176428691534118942, 0.04335639704956491258, 0.04494850718378863574, 0.04654061731801235891, 0.04813272745223608207, 0.04892878251934794365, 0.04972483758645979829, 0.05131694772068349369 ),
 .UNSPECIFIED. ) ;
#50211=EDGE_CURVE ( 'NONE', #3111, #68404, #50076, .T. ) ;
#50214=CARTESIAN_POINT ( 'NONE',  ( 22.53041628628730209, 6.810083298012985509, -39.69690971090911802 ) ) ;
#50215=CARTESIAN_POINT ( 'NONE',  ( 113.8626313173126334, 31.71036178495294067, 16.85260883570550661 ) ) ;
#50217=CARTESIAN_POINT ( 'NONE',  ( 62.53328835682437159, 12.56090025569837287, 29.81296093922127710 ) ) ;
#50220=AXIS2_PLACEMENT_3D ( 'NONE', #59406, #680, #54466 ) ;
#50221=CARTESIAN_POINT ( 'NONE',  ( 177.7964363391244547, 76.75162026635251777, 30.05250232064427252 ) ) ;
#50222=CARTESIAN_POINT ( 'NONE',  ( -38.26251837371328435, 11.83628080764031409, -93.36397248376952973 ) ) ;
#50224=FACE_OUTER_BOUND ( 'NONE', #16702, .T. ) ;
#50227=CARTESIAN_POINT ( 'NONE',  ( -24.18270484670773968, 9.527492911955594224, 39.67658164943471633 ) ) ;
#50228=CARTESIAN_POINT ( 'NONE',  ( -73.63128929564828695, 21.53548093502884342, -37.05148811347594773 ) ) ;
#50230=ORIENTED_EDGE ( 'NONE', *, *, #42026, .T. ) ;
#50232=CARTESIAN_POINT ( 'NONE',  ( 177.6874527215932176, 76.64335277577062300, -90.68412946948107844 ) ) ;
#50233=AXIS2_PLACEMENT_3D ( 'NONE', #5414, #65553, #22282 ) ;
#50234=LINE ( 'NONE', #34057, #6116 ) ;
#50235=CARTESIAN_POINT ( 'NONE',  ( -177.5288247523078553, 93.72924674643513754, 44.40754021158874565 ) ) ;
#50238=ORIENTED_EDGE ( 'NONE', *, *, #42258, .F. ) ;
#50239=ORIENTED_EDGE ( 'NONE', *, *, #4379, .F. ) ;
#50241=CARTESIAN_POINT ( 'NONE',  ( 63.01563776193091826, -170.0000000000000000, -23.87614024170608218 ) ) ;
#50243=CARTESIAN_POINT ( 'NONE',  ( -38.26497993382595553, 10.81185389040525635, -39.69992527180441755 ) ) ;
#50244=ADVANCED_FACE ( 'NONE', ( #34306 ), #11783, .F. ) ;
#50245=CARTESIAN_POINT ( 'NONE',  ( -94.87314045600119528, 29.17466428498257969, 90.48494885821429534 ) ) ;
#50246=CARTESIAN_POINT ( 'NONE',  ( -149.0782809666403637, 63.81577337591401289, 30.72082123989905256 ) ) ;
#50248=CARTESIAN_POINT ( 'NONE',  ( -76.32456871438913026, 22.51591205926310124, -22.91205146820279026 ) ) ;
#50250=CARTESIAN_POINT ( 'NONE',  ( 82.74007713545063325, 18.13042311233563098, 57.63927396060999797 ) ) ;
#50251=ORIENTED_EDGE ( 'NONE', *, *, #67425, .T. ) ;
#50253=CARTESIAN_POINT ( 'NONE',  ( 35.44781468922822398, 7.928097401423699786, 31.03618968133934430 ) ) ;
#50254=DIRECTION ( 'NONE',  ( -0.000000000000000000, 1.000000000000000000, -0.000000000000000000 ) ) ;
#50260=CARTESIAN_POINT ( 'NONE',  ( -47.80896875121164413, 12.85816703949531536, 12.93218738431712289 ) ) ;
#50263=ORIENTED_EDGE ( 'NONE', *, *, #65270, .T. ) ;
#50269=CARTESIAN_POINT ( 'NONE',  ( 63.01563776193090405, 13.70579113808098271, -35.72069083216973695 ) ) ;
#50270=FACE_OUTER_BOUND ( 'NONE', #2436, .T. ) ;
#50274=CARTESIAN_POINT ( 'NONE',  ( 152.1153500913667642, 54.85403770686892955, -65.21174665958072580 ) ) ;
#50275=CARTESIAN_POINT ( 'NONE',  ( -38.26497993382596263, 10.81185389040525635, 40.83372649958661782 ) ) ;
#50278=CARTESIAN_POINT ( 'NONE',  ( 141.2894128405439176, 46.09731134920846074, -42.48579671950618319 ) ) ;
#50279=APPLICATION_CONTEXT ( 'automotive_design' ) ;
#50285=VERTEX_POINT ( 'NONE', #27966 ) ;
#50289=CARTESIAN_POINT ( 'NONE',  ( 141.2920930135741173, 47.30245445423356898, 91.74529553920554292 ) ) ;
#50295=CARTESIAN_POINT ( 'NONE',  ( 164.7167608259061922, 63.51199216609071385, -18.73303924478714677 ) ) ;
#50298=CARTESIAN_POINT ( 'NONE',  ( 141.0804878838241336, 45.96076546397620177, -68.28228989354154521 ) ) ;
#50301=ADVANCED_FACE ( 'NONE', ( #34662 ), #1955, .F. ) ;
#50304=CARTESIAN_POINT ( 'NONE',  ( 161.7006237583813970, 62.31514460450500792, -22.98982369199385900 ) ) ;
#50305=CARTESIAN_POINT ( 'NONE',  ( 13.84937401517046851, 6.446378549072247388, 44.76393167428260256 ) ) ;
#50306=ORIENTED_EDGE ( 'NONE', *, *, #47260, .F. ) ;
#50307=CARTESIAN_POINT ( 'NONE',  ( -61.86403937395562025, 16.61416349803656090, -66.41162500208781694 ) ) ;
#50310=CARTESIAN_POINT ( 'NONE',  ( 163.7379901688713062, 64.00402364591248272, -39.49700036984320661 ) ) ;
#50311=CARTESIAN_POINT ( 'NONE',  ( 93.63037639125411715, 21.92981100938040484, 13.06913551750571756 ) ) ;
#50312=CARTESIAN_POINT ( 'NONE',  ( 164.4728833318992542, 63.30716077995680990, -40.92446310325109948 ) ) ;
#50313=EDGE_LOOP ( 'NONE', ( #9503, #23705, #24097, #18561 ) ) ;
#50314=AXIS2_PLACEMENT_3D ( 'NONE', #22081, #27346, #31599 ) ;
#50315=CARTESIAN_POINT ( 'NONE',  ( -95.05323930133207000, 30.36974142673411947, 13.24519497187949391 ) ) ;
#50319=CARTESIAN_POINT ( 'NONE',  ( 32.90051628396145844, 8.664124555952449569, 33.64247275619753452 ) ) ;
#50320=CARTESIAN_POINT ( 'NONE',  ( -178.2448732545371115, 94.58403736950705820, -36.71535872372318465 ) ) ;
#50321=CARTESIAN_POINT ( 'NONE',  ( -179.3508319071551966, 95.92102653685060432, -91.71737262036411664 ) ) ;
#50322=CARTESIAN_POINT ( 'NONE',  ( 153.2384531768735769, 54.43344429203621360, 69.96338799158385768 ) ) ;
#50323=CARTESIAN_POINT ( 'NONE',  ( 127.2202105166096402, 37.55913282978156076, -73.87116003439983558 ) ) ;
#50325=CARTESIAN_POINT ( 'NONE',  ( 141.0517870458593563, 47.14452711594498879, -68.23502628271137382 ) ) ;
#50327=CARTESIAN_POINT ( 'NONE',  ( -11.78188048797445475, 8.190559674012726887, 58.08383411553590037 ) ) ;
#50329=CARTESIAN_POINT ( 'NONE',  ( -156.0204364459165163, 71.27041535366187475, -38.58461829599199433 ) ) ;
#50330=VECTOR ( 'NONE', #56628, 1000.000000000000000 ) ;
#50332=CARTESIAN_POINT ( 'NONE',  ( -38.68632430131781774, 11.91908191268690942, 39.66289844268187892 ) ) ;
#50334=CARTESIAN_POINT ( 'NONE',  ( -2.177337698256109455, 7.595833446947581002, 42.57430342708116910 ) ) ;
#50335=CARTESIAN_POINT ( 'NONE',  ( -14.65035343718723482, 7.431577370124334614, -93.38227200523709826 ) ) ;
#50337=CARTESIAN_POINT ( 'NONE',  ( -3.862560291631539133, 7.672660553664873540, -22.44576929375073604 ) ) ;
#50338=CARTESIAN_POINT ( 'NONE',  ( -9.779603649692299783, 8.034615131607074190, 44.87335778418307086 ) ) ;
#50339=CARTESIAN_POINT ( 'NONE',  ( 113.4493678088378203, 30.39339414805072792, 17.06312677987657622 ) ) ;
#50346=CARTESIAN_POINT ( 'NONE',  ( 102.7551177910568327, 25.56939188780866345, -70.76452187158794516 ) ) ;
#50347=CARTESIAN_POINT ( 'NONE',  ( 45.35621884287174765, 10.27694987765648449, -20.86182146456972930 ) ) ;
#50348=CARTESIAN_POINT ( 'NONE',  ( 46.50704915687940399, 9.440294391580033917, 66.67262751023041289 ) ) ;
#50352=CARTESIAN_POINT ( 'NONE',  ( -78.66644367742111399, 22.32174330031318377, 57.26275173013680586 ) ) ;
#50358=CARTESIAN_POINT ( 'NONE',  ( 175.3815143714021758, 73.02838262207001208, 68.53128429288518930 ) ) ;
#50360=CARTESIAN_POINT ( 'NONE',  ( 109.7732660198864494, 29.77277639096405792, 71.45576479620105204 ) ) ;
#50361=EDGE_CURVE ( 'NONE', #28307, #49946, #45191, .T. ) ;
#50362=CARTESIAN_POINT ( 'NONE',  ( -165.6208371326873703, 80.58821715390998008, -15.66524306475966455 ) ) ;
#50365=DIRECTION ( 'NONE',  ( 0.000000000000000000, 0.000000000000000000, 1.000000000000000000 ) ) ;
#50367=EDGE_CURVE ( 'NONE', #44993, #50858, #41308, .T. ) ;
#50368=CARTESIAN_POINT ( 'NONE',  ( 90.51709546286271291, 21.85407654229980423, 3.949318351511905689 ) ) ;
#50369=FACE_OUTER_BOUND ( 'NONE', #42955, .T. ) ;
#50370=CARTESIAN_POINT ( 'NONE',  ( 181.0840389613909736, 78.60582251573005408, -51.22505766587963905 ) ) ;
#50371=CYLINDRICAL_SURFACE ( 'NONE', #21786, 7.500000000000013323 ) ;
#50373=FACE_BOUND ( 'NONE', #41239, .T. ) ;
#50380=CARTESIAN_POINT ( 'NONE',  ( -179.2128128997734393, 95.75254520622991095, 7.073590364011439924 ) ) ;
#50382=CARTESIAN_POINT ( 'NONE',  ( 85.67452303415197434, 19.09699411916384904, -62.71192339984101238 ) ) ;
#50386=FACE_OUTER_BOUND ( 'NONE', #50961, .T. ) ;
#50387=CARTESIAN_POINT ( 'NONE',  ( 199.3764470687682149, 100.9548044849098716, -38.53510737021463228 ) ) ;
#50388=EDGE_LOOP ( 'NONE', ( #25847, #69079, #29728, #32288 ) ) ;
#50390=VERTEX_POINT ( 'NONE', #13871 ) ;
#50393=CARTESIAN_POINT ( 'NONE',  ( 94.11595392909974578, 23.18887043179184815, -69.65182159334985101 ) ) ;
#50394=EDGE_LOOP ( 'NONE', ( #7285, #55495 ) ) ;
#50395=ORIENTED_EDGE ( 'NONE', *, *, #47480, .T. ) ;
#50396=CARTESIAN_POINT ( 'NONE',  ( 40.38132770291768736, 9.553709436640062336, 71.71008232015611839 ) ) ;
#50397=CARTESIAN_POINT ( 'NONE',  ( -173.1211646369891355, 88.63826465341151106, 57.66624519710472185 ) ) ;
#50400=ORIENTED_EDGE ( 'NONE', *, *, #61538, .F. ) ;
#50402=CARTESIAN_POINT ( 'NONE',  ( -51.77431913897918747, 14.86466849149170955, 17.73581465740154428 ) ) ;
#50403=CARTESIAN_POINT ( 'NONE',  ( -133.2787743207940707, 52.78950725740543248, -14.23327279590464833 ) ) ;
#50404=CARTESIAN_POINT ( 'NONE',  ( -156.7429055738855936, 71.93655028710443844, -93.96263355926134864 ) ) ;
#50405=CARTESIAN_POINT ( 'NONE',  ( 111.8699272271189358, 29.64190505307780654, -23.90307673515284037 ) ) ;
#50406=CARTESIAN_POINT ( 'NONE',  ( 87.31198329270952740, 19.65488789718978069, 83.42517577981676880 ) ) ;
#50414=CARTESIAN_POINT ( 'NONE',  ( 107.0477776024378898, 27.43148174916616355, -23.36746922899289558 ) ) ;
#50415=CARTESIAN_POINT ( 'NONE',  ( 140.8935642633566943, 45.83887848292358314, -94.58095331458939370 ) ) ;
#50416=CARTESIAN_POINT ( 'NONE',  ( 204.7199663062789057, 108.0881780334054838, 82.89220380942870747 ) ) ;
#50419=CARTESIAN_POINT ( 'NONE',  ( -71.56718866013692093, 19.74312628447965068, -66.98874544750654536 ) ) ;
#50423=CARTESIAN_POINT ( 'NONE',  ( 15.29305096970402289, 7.491604910111008486, -8.674393508222093985 ) ) ;
#50426=AXIS2_PLACEMENT_3D ( 'NONE', #15682, #37130, #58576 ) ;
#50427=CARTESIAN_POINT ( 'NONE',  ( 64.94098077424391136, 14.16208887966257457, -23.64097255858331792 ) ) ;
#50428=CARTESIAN_POINT ( 'NONE',  ( 181.5079096844946491, 80.47139261082469375, -78.06960825634331513 ) ) ;
#50429=CARTESIAN_POINT ( 'NONE',  ( -165.6397095829521788, 80.60756690931943069, 37.71251476309661399 ) ) ;
#50430=CARTESIAN_POINT ( 'NONE',  ( 111.1865443042262456, 30.43181341527238715, -24.03313457428269473 ) ) ;
#50431=VECTOR ( 'NONE', #1316, 1000.000000000000000 ) ;
#50432=CARTESIAN_POINT ( 'NONE',  ( -108.6909373351217312, 36.15835109565439609, 7.250169111965115931 ) ) ;
#50433=DIRECTION ( 'NONE',  ( -0.000000000000000000, 1.000000000000000000, -0.000000000000000000 ) ) ;
#50434=CARTESIAN_POINT ( 'NONE',  ( 139.6326990672751265, 46.22017155708127234, -21.46926057526128417 ) ) ;
#50435=ORIENTED_EDGE ( 'NONE', *, *, #67045, .T. ) ;
#50437=CARTESIAN_POINT ( 'NONE',  ( -7.825402957745087207, -170.0000000000000000, -96.60717191287118055 ) ) ;
#50438=CARTESIAN_POINT ( 'NONE',  ( -10.91976120871577827, 7.112268444252504374, 3.934707406933564133 ) ) ;
#50440=CARTESIAN_POINT ( 'NONE',  ( 56.66438910147189034, 11.28870326331392526, -20.37264592891143522 ) ) ;
#50442=B_SPLINE_CURVE_WITH_KNOTS ( 'NONE', 3,
 ( #67638, #40893, #62353, #47528, #21171, #10255, #58109, #20465, #41250, #31040, #47198, #4981, #63740, #14507, #52140, #62706, #20817, #41928, #57419, #35965, #4307, #25424, #52484, #14845 ),
 .UNSPECIFIED., .F., .F.,
 ( 4, 2, 2, 2, 2, 2, 2, 2, 2, 2, 2, 4 ),
 ( 0.009967446706431848380, 0.01121006802826941991, 0.01245268935010699143, 0.01307400001102577806, 0.01369531067194456470, 0.01493793199378213796, 0.01555924265470091244, 0.01618055331561968346, 0.01742317463745724979, 0.01804448529837605550, 0.01866579595929486121, 0.01990841728113247958 ),
 .UNSPECIFIED. ) ;
#50444=CARTESIAN_POINT ( 'NONE',  ( -190.6985136298602015, 109.1272424661243434, 42.87371446347281534 ) ) ;
#50445=CARTESIAN_POINT ( 'NONE',  ( 198.4059165548112276, 99.71594270191991427, 67.64306774733000793 ) ) ;
#50447=DIRECTION ( 'NONE',  ( -0.000000000000000000, 1.000000000000000000, -0.000000000000000000 ) ) ;
#50448=CARTESIAN_POINT ( 'NONE',  ( -62.41727141396690115, 17.83188754031768042, -68.07784404646591270 ) ) ;
#50449=CARTESIAN_POINT ( 'NONE',  ( 197.3756653044962945, 98.41886189307120958, -72.30260639311568127 ) ) ;
#50453=CARTESIAN_POINT ( 'NONE',  ( -171.5864836273286755, 85.43596863096360039, -88.54944863603246574 ) ) ;
#50455=FACE_BOUND ( 'NONE', #58663, .T. ) ;
#50457=CARTESIAN_POINT ( 'NONE',  ( -1.083610669212419664, 6.545642299653469109, 67.78290952672001879 ) ) ;
#50460=CARTESIAN_POINT ( 'NONE',  ( 150.0278556977734183, 53.32860603304214209, 64.83238834058245459 ) ) ;
#50462=AXIS2_PLACEMENT_3D ( 'NONE', #61138, #54801, #12960 ) ;
#50466=CARTESIAN_POINT ( 'NONE',  ( -188.6739852773920347, 108.2139733222100517, 9.872393598427303019 ) ) ;
#50467=CARTESIAN_POINT ( 'NONE',  ( 15.78827728214693416, 6.500811158483284835, 3.170157082241545687 ) ) ;
#50468=ORIENTED_EDGE ( 'NONE', *, *, #19048, .F. ) ;
#50471=CARTESIAN_POINT ( 'NONE',  ( 153.2208437558771834, 55.67531116261155688, 43.10704344242034836 ) ) ;
#50476=CARTESIAN_POINT ( 'NONE',  ( -178.7458319892713803, 93.61502008198023361, 16.44468136262722524 ) ) ;
#50477=CARTESIAN_POINT ( 'NONE',  ( -3.252497086158848916, 6.636017118948021931, 4.805921196466799827 ) ) ;
#50481=CARTESIAN_POINT ( 'NONE',  ( -190.6985136298601731, 109.1272424661242582, 33.97142148329322708 ) ) ;
#50483=CARTESIAN_POINT ( 'NONE',  ( 114.6890011751076202, 30.99337387307412683, -37.36302526878641572 ) ) ;
#50484=CARTESIAN_POINT ( 'NONE',  ( 8.000000000000007105, 249.8719672152120381, 94.99999999999866418 ) ) ;
#50486=CARTESIAN_POINT ( 'NONE',  ( -169.1122507277982834, 84.24359299875008844, -75.41064519614697303 ) ) ;
#50487=CARTESIAN_POINT ( 'NONE',  ( -131.1785597586340941, 50.07314260389248517, 86.47842268959267642 ) ) ;
#50493=CARTESIAN_POINT ( 'NONE',  ( -142.4991775570125299, 58.45550857435405590, 67.79001987503191629 ) ) ;
#50494=CARTESIAN_POINT ( 'NONE',  ( 82.14396250120408638, 18.99560174459421802, 31.19617389665937779 ) ) ;
#50500=CARTESIAN_POINT ( 'NONE',  ( -180.2188652555596207, 96.98354576637423463, -17.80801388957663534 ) ) ;
#50506=CARTESIAN_POINT ( 'NONE',  ( 110.2429982417149290, 28.88204397445231209, 56.45576479620100940 ) ) ;
#50510=CARTESIAN_POINT ( 'NONE',  ( 63.98009977735161158, 12.89803120691695604, -23.82977458817669358 ) ) ;
#50511=CARTESIAN_POINT ( 'NONE',  ( -71.86568654225716557, 20.91200104397924875, -72.63218713565318296 ) ) ;
#50512=CARTESIAN_POINT ( 'NONE',  ( -108.9136445001390143, 36.28030794288190464, 68.37215121731419742 ) ) ;
#50513=CARTESIAN_POINT ( 'NONE',  ( -23.98903001682803193, 8.486614814224632042, -43.81140712853910202 ) ) ;
#50517=ORIENTED_EDGE ( 'NONE', *, *, #63378, .F. ) ;
#50519=CARTESIAN_POINT ( 'NONE',  ( -71.48316049915626991, 19.71415776932100528, 93.78843686400733759 ) ) ;
#50520=LINE ( 'NONE', #29076, #8265 ) ;
#50522=CARTESIAN_POINT ( 'NONE',  ( 128.4157044224113804, 39.39296260757094359, 31.82551368169737316 ) ) ;
#50526=CARTESIAN_POINT ( 'NONE',  ( -149.5074843970971017, 64.17983161892348676, 57.56537183036274996 ) ) ;
#50528=CARTESIAN_POINT ( 'NONE',  ( 55.51528220483959331, 12.08323518953685216, 37.55138378790348241 ) ) ;
#50529=CARTESIAN_POINT ( 'NONE',  ( 38.75182793578637330, 8.325674960048864648, 83.62384145260158164 ) ) ;
#50530=CARTESIAN_POINT ( 'NONE',  ( 0.000000000000000000, 0.000000000000000000, 0.000000000000000000 ) ) ;
#50532=CARTESIAN_POINT ( 'NONE',  ( -0.8055628312658242862, 6.535476276302842003, -45.56989120479929767 ) ) ;
#50534=CARTESIAN_POINT ( 'NONE',  ( -15.32495246574475267, 8.506829480038508251, 10.26907141737711804 ) ) ;
#50535=CARTESIAN_POINT ( 'NONE',  ( -147.7845268487069745, 62.73119438705056439, 18.68858363414569723 ) ) ;
#50536=DIRECTION ( 'NONE',  ( 0.000000000000000000, -1.000000000000000000, 0.000000000000000000 ) ) ;
#50537=CARTESIAN_POINT ( 'NONE',  ( 197.2200752504831485, 96.62072041958364821, 64.21650735878895944 ) ) ;
#50538=CARTESIAN_POINT ( 'NONE',  ( -95.59001106299177764, 29.51022327712105664, -92.80581223319890682 ) ) ;
#50541=VECTOR ( 'NONE', #9233, 1000.000000000000000 ) ;
#50548=CARTESIAN_POINT ( 'NONE',  ( -123.4531143159639157, 44.90777521523904880, -49.50914397245080778 ) ) ;
#50549=CARTESIAN_POINT ( 'NONE',  ( -144.3945994505580757, 59.96115386701887218, -20.96066555231037754 ) ) ;
#50550=CARTESIAN_POINT ( 'NONE',  ( -6.125624616441579740, 7.794071945221086040, -62.45369946781575266 ) ) ;
#50552=CARTESIAN_POINT ( 'NONE',  ( 164.9007491581839417, 64.98457710411663868, 91.68427848334972907 ) ) ;
#50554=CARTESIAN_POINT ( 'NONE',  ( 158.9247692837400052, 60.07442151987904566, -89.94665146420680912 ) ) ;
#50555=CARTESIAN_POINT ( 'NONE',  ( 198.3926538463959162, 98.07933330386030946, -39.72515298445662779 ) ) ;
#50556=CARTESIAN_POINT ( 'NONE',  ( -156.0204364459164594, 71.27041535366186054, 41.94903347539903393 ) ) ;
#50558=CARTESIAN_POINT ( 'NONE',  ( 20.74852474914889910, 6.709938988646747760, -37.37222025436115302 ) ) ;
#50559=CARTESIAN_POINT ( 'NONE',  ( 117.3145357257065768, 33.41973663092564806, 12.81680853675090503 ) ) ;
#50561=EDGE_CURVE ( 'NONE', #52688, #9201, #45066, .T. ) ;
#50562=CARTESIAN_POINT ( 'NONE',  ( 59.95259601283825646, 11.98300577492411634, 30.46261997733679650 ) ) ;
#50565=CARTESIAN_POINT ( 'NONE',  ( 180.2494929075577943, 79.18888319146950039, 44.30859410551142474 ) ) ;
#50566=CARTESIAN_POINT ( 'NONE',  ( 22.89634831467701304, 6.832298124325686395, -67.45812584797086231 ) ) ;
#50567=CARTESIAN_POINT ( 'NONE',  ( -15.13464256769235838, 8.488509377255649468, -68.06414086977258648 ) ) ;
#50570=LINE ( 'NONE', #9654, #19502 ) ;
#50572=CARTESIAN_POINT ( 'NONE',  ( -74.79539698934961223, 21.95498232236883496, -49.04378561426771910 ) ) ;
#50574=CARTESIAN_POINT ( 'NONE',  ( 205.5049354810107900, 109.1776577097391225, -78.17048162308532255 ) ) ;
#50577=CARTESIAN_POINT ( 'NONE',  ( 110.7117404013331452, 30.20916032354563185, 29.61121420573731555 ) ) ;
#50578=CARTESIAN_POINT ( 'NONE',  ( 127.4669243510812890, 38.85312661085429653, 67.81406123581646739 ) ) ;
#50579=CARTESIAN_POINT ( 'NONE',  ( 20.74561700410411191, 7.717362891868938313, 70.00851792305307697 ) ) ;
#50580=ORIENTED_EDGE ( 'NONE', *, *, #61214, .T. ) ;
#50582=VERTEX_POINT ( 'NONE', #641 ) ;
#50585=CARTESIAN_POINT ( 'NONE',  ( 15.78827728214693416, 7.507518794609588042, -23.67439350822212774 ) ) ;
#50587=CARTESIAN_POINT ( 'NONE',  ( -37.92542950990691963, 10.74638084523341952, -46.59059523367306355 ) ) ;
#50588=CARTESIAN_POINT ( 'NONE',  ( 218.0000000000000000, 128.6235316737731296, 94.99999999999866418 ) ) ;
#50590=CARTESIAN_POINT ( 'NONE',  ( -132.0958200534848004, 50.71531800824802616, 60.73979307723551102 ) ) ;
#50591=CARTESIAN_POINT ( 'NONE',  ( -173.1211646369891355, 87.12891641440857882, -76.55650775521370122 ) ) ;
#50594=ORIENTED_EDGE ( 'NONE', *, *, #68084, .T. ) ;
#50595=CARTESIAN_POINT ( 'NONE',  ( 34.83825437341840114, 7.859462995505743343, 31.44215116196434678 ) ) ;
#50596=CARTESIAN_POINT ( 'NONE',  ( 86.62931800182293784, 20.48449268398423229, 56.55663816294300261 ) ) ;
#50598=EDGE_CURVE ( 'NONE', #5626, #25055, #38979, .T. ) ;
#50601=CARTESIAN_POINT ( 'NONE',  ( -124.7710763417278201, 46.96042092553521741, 57.54553104023176502 ) ) ;
#50602=CARTESIAN_POINT ( 'NONE',  ( -10.69547582519244600, 8.103864215011986616, -49.86004041143019805 ) ) ;
#50605=CARTESIAN_POINT ( 'NONE',  ( 155.7277429502854034, 56.30804678861341728, -50.93229212615000989 ) ) ;
#50606=EDGE_LOOP ( 'NONE', ( #60128, #41513, #8136, #45795 ) ) ;
#50608=CARTESIAN_POINT ( 'NONE',  ( -157.0069704378501854, 70.81086990254190994, -14.88609962755286986 ) ) ;
#50615=CARTESIAN_POINT ( 'NONE',  ( 151.1700480242206197, 54.15904440870131964, -66.39142155471229501 ) ) ;
#50616=CARTESIAN_POINT ( 'NONE',  ( -38.54881010929334906, 10.86689971295294654, 40.15423812736370479 ) ) ;
#50617=CARTESIAN_POINT ( 'NONE',  ( 141.2811136745703209, 46.09188267874204570, -44.61855967972866210 ) ) ;
#50620=CARTESIAN_POINT ( 'NONE',  ( -125.4481990864046139, 46.20056605584955634, 30.61994787315706645 ) ) ;
#50622=CARTESIAN_POINT ( 'NONE',  ( 37.45439421541014724, 9.177432671831377675, -9.015803115001828516 ) ) ;
#50624=CARTESIAN_POINT ( 'NONE',  ( 126.6387625275754374, 38.38663782932677293, 92.76825455630849149 ) ) ;
#50625=CYLINDRICAL_SURFACE ( 'NONE', #63927, 7.500000000000020428 ) ;
#50627=CARTESIAN_POINT ( 'NONE',  ( -125.0023254877051784, 45.90912477771776423, -76.71887141435124136 ) ) ;
#50629=CARTESIAN_POINT ( 'NONE',  ( 164.3577270662354124, 63.21061577643037310, -19.76033467163099644 ) ) ;
#50631=CARTESIAN_POINT ( 'NONE',  ( 68.61679388097593346, 14.04192738700837317, 59.16375057879944421 ) ) ;
#50632=CARTESIAN_POINT ( 'NONE',  ( 134.7770330630252715, 41.98246829846535633, -62.91025920626427848 ) ) ;
#50637=ADVANCED_FACE ( 'NONE', ( #32646 ), #54078, .F. ) ;
#50638=CARTESIAN_POINT ( 'NONE',  ( -31.43908319763710679, -170.0000000000000000, 45.21645440618919309 ) ) ;
#50643=CARTESIAN_POINT ( 'NONE',  ( 64.94098077424391136, 14.16208887966257279, 56.89267921280773521 ) ) ;
#50646=CARTESIAN_POINT ( 'NONE',  ( 164.4760519199595308, 64.62478832434435105, -40.89396928478465298 ) ) ;
#50652=CARTESIAN_POINT ( 'NONE',  ( -97.48179118242299523, 31.52606332398820399, 5.389128531495072316 ) ) ;
#50655=CARTESIAN_POINT ( 'NONE',  ( 69.99712624136184047, 15.44163584096631325, 93.82355723117841251 ) ) ;
#50656=CARTESIAN_POINT ( 'NONE',  ( 155.7277429502854034, 56.30804678861341017, 29.60135964524100061 ) ) ;
#50657=CARTESIAN_POINT ( 'NONE',  ( 86.15454111412294935, 20.32174891186169319, -23.97701360844805762 ) ) ;
#50658=CARTESIAN_POINT ( 'NONE',  ( -132.2352756077771119, 50.81350938245625315, -19.58186461629218655 ) ) ;
#50659=CARTESIAN_POINT ( 'NONE',  ( -145.6099850599923968, 60.94286946341170363, -89.59051459497440817 ) ) ;
#50661=ADVANCED_FACE ( 'NONE', ( #38619 ), #54790, .F. ) ;
#50662=ORIENTED_EDGE ( 'NONE', *, *, #42060, .T. ) ;
#50663=CARTESIAN_POINT ( 'NONE',  ( -94.83091526606384036, 30.26550147229323073, 63.84764049538445363 ) ) ;
#50664=CARTESIAN_POINT ( 'NONE',  ( -15.07235766390729026, 8.482541916553474337, 62.51267422215675396 ) ) ;
#50667=FACE_OUTER_BOUND ( 'NONE', #7127, .T. ) ;
#50670=CARTESIAN_POINT ( 'NONE',  ( -1.866625526081663544, 7.583073082893620587, 42.19666861288822446 ) ) ;
#50671=CARTESIAN_POINT ( 'NONE',  ( 133.8566784816069344, -170.0000000000000000, -16.67876034193198365 ) ) ;
#50673=CARTESIAN_POINT ( 'NONE',  ( -0.9897066053608923886, 7.549089325901772618, -19.16927265933078317 ) ) ;
#50674=CARTESIAN_POINT ( 'NONE',  ( -8.810383862755511331, 7.965311326754782151, 45.06702628433764346 ) ) ;
#50675=CARTESIAN_POINT ( 'NONE',  ( -62.45176220516622578, 16.79101814080732424, 12.22500217833821878 ) ) ;
#50677=CARTESIAN_POINT ( 'NONE',  ( -96.76336539645315327, 31.18045094643427717, -47.61949373948618813 ) ) ;
#50681=CARTESIAN_POINT ( 'NONE',  ( 44.34362023773823580, 10.12115849931652711, -21.93874443874187108 ) ) ;
#50682=CARTESIAN_POINT ( 'NONE',  ( 46.13856685535755986, 9.381502944822521783, 67.59186432702131242 ) ) ;
#50686=EDGE_CURVE ( 'NONE', #18800, #36151, #21394, .T. ) ;
#50687=ADVANCED_FACE ( 'NONE', ( #24547 ), #35434, .F. ) ;
#50688=EDGE_CURVE ( 'NONE', #32880, #35021, #60904, .T. ) ;
#50692=CARTESIAN_POINT ( 'NONE',  ( -168.7187482717113198, 82.35796501763485367, 59.07591196666088962 ) ) ;
#50694=VERTEX_POINT ( 'NONE', #18559 ) ;
#50699=VECTOR ( 'NONE', #66295, 1000.000000000000000 ) ;
#50701=CARTESIAN_POINT ( 'NONE',  ( 157.4703587214989113, 57.65129005721575339, -24.27963370867398396 ) ) ;
#50703=CARTESIAN_POINT ( 'NONE',  ( 58.08938767906776235, 12.61185010801508888, -10.69966040140734620 ) ) ;
#50705=CARTESIAN_POINT ( 'NONE',  ( 107.9213359589209063, 28.92595015506875100, -36.27514522574465161 ) ) ;
#50706=CARTESIAN_POINT ( 'NONE',  ( 21.74799039132243550, 7.772294950329605712, -38.43909590461863957 ) ) ;
#50708=DIRECTION ( 'NONE',  ( -0.000000000000000000, 1.000000000000000000, -0.000000000000000000 ) ) ;
#50709=CARTESIAN_POINT ( 'NONE',  ( 211.0967808702091588, 115.5516932918877018, -20.90306055675851482 ) ) ;
#50710=FACE_BOUND ( 'NONE', #42745, .T. ) ;
#50714=CARTESIAN_POINT ( 'NONE',  ( 32.37980458033285913, 8.611076697115699119, -67.31855367964614345 ) ) ;
#50716=CARTESIAN_POINT ( 'NONE',  ( 157.0336341255056141, 57.31169401067818114, 2.564916881789689462 ) ) ;
#50720=CARTESIAN_POINT ( 'NONE',  ( 198.2581645178918563, 99.52881771501682806, -39.97064483821105085 ) ) ;
#50725=CARTESIAN_POINT ( 'NONE',  ( -86.17927978631391284, 25.32700573188346738, -69.44798174949396241 ) ) ;
#50726=CARTESIAN_POINT ( 'NONE',  ( -62.49137879463568623, 17.85440472148627933, -14.88192700454524520 ) ) ;
#50731=CARTESIAN_POINT ( 'NONE',  ( 45.04506994399700659, 10.22854084020123899, 59.29347898550686580 ) ) ;
#50733=CARTESIAN_POINT ( 'NONE',  ( 23.09541709302172308, 6.844586979481588784, 8.962678893484639531 ) ) ;
#50735=VERTEX_POINT ( 'NONE', #26938 ) ;
#50741=CARTESIAN_POINT ( 'NONE',  ( -47.94536219817735656, 13.92422159065987586, 8.527031293414781388 ) ) ;
#50742=CARTESIAN_POINT ( 'NONE',  ( -132.4776673493542489, 52.21763813822158085, -19.17034394188376112 ) ) ;
#50748=ORIENTED_EDGE ( 'NONE', *, *, #53154, .F. ) ;
#50751=CARTESIAN_POINT ( 'NONE',  ( 39.88971011078923823, 8.472992116645418292, 3.069283715499572907 ) ) ;
#50753=CARTESIAN_POINT ( 'NONE',  ( -49.14234466229833487, 13.17605306081208560, -20.49537269497533032 ) ) ;
#50754=CARTESIAN_POINT ( 'NONE',  ( 107.0471828278920583, 27.43080724084233069, -9.776041531421187258 ) ) ;
#50755=CARTESIAN_POINT ( 'NONE',  ( 203.9276061909314706, 105.2889220654478777, 2.363170148305746565 ) ) ;
#50756=CARTESIAN_POINT ( 'NONE',  ( 211.5020032503682330, 118.0078774122368515, 87.23615886703346689 ) ) ;
#50757=CYLINDRICAL_SURFACE ( 'NONE', #36638, 7.500000000000020428 ) ;
#50758=CARTESIAN_POINT ( 'NONE',  ( -85.64924756730677302, 26.19583280090850153, 62.01450634387265382 ) ) ;
#50759=CARTESIAN_POINT ( 'NONE',  ( -15.13254930056756464, 7.477527548005403979, 39.32343163489576199 ) ) ;
#50761=CARTESIAN_POINT ( 'NONE',  ( 10.83521140779424030, 7.398743030771586682, -21.82737784355149557 ) ) ;
#50763=ORIENTED_EDGE ( 'NONE', *, *, #10010, .T. ) ;
#50764=CARTESIAN_POINT ( 'NONE',  ( -144.9417090887490644, 61.69631066549396792, 5.421503341054570768 ) ) ;
#50766=CARTESIAN_POINT ( 'NONE',  ( -37.11830583849306464, 11.61671896815851390, 86.49628856077504224 ) ) ;
#50768=EDGE_CURVE ( 'NONE', #62204, #68773, #19801, .T. ) ;
#50770=FACE_OUTER_BOUND ( 'NONE', #4610, .T. ) ;
#50771=EDGE_CURVE ( 'NONE', #988, #40831, #50817, .T. ) ;
#50778=CARTESIAN_POINT ( 'NONE',  ( 93.59491193977102341, 22.99153521538281453, -94.19891465754322724 ) ) ;
#50781=CARTESIAN_POINT ( 'NONE',  ( -48.57297291660698590, 13.03920345822338334, 34.00833018951762909 ) ) ;
#50782=CARTESIAN_POINT ( 'NONE',  ( 70.26840926437850499, -170.0000000000000000, -95.00000000000133582 ) ) ;
#50784=LINE ( 'NONE', #45156, #58097 ) ;
#50785=CARTESIAN_POINT ( 'NONE',  ( -56.02289203441036847, 15.98631679403370320, -62.10799750277473663 ) ) ;
#50786=CARTESIAN_POINT ( 'NONE',  ( 197.2847860006354779, 98.30530166401516112, -71.82171173343019177 ) ) ;
#50788=B_SPLINE_CURVE_WITH_KNOTS ( 'NONE', 3,
 ( #68561, #26346, #58007, #25320, #53053, #63635, #15781, #21070, #5227, #30588, #9478, #10154, #31967, #15448, #16123, #26004, #52036, #3855, #52382, #63288, #61379, #68886, #57668, #58337, #10496, #9826, #53393, #31284, #30938, #69241, #42516, #4202, #46754, #68226, #36899, #41488, #52711, #4539, #21397, #47432, #31617, #42842, #20716, #64313, #64664, #65013 ),
 .UNSPECIFIED., .F., .F.,
 ( 4, 2, 2, 2, 2, 2, 2, 2, 2, 2, 2, 2, 2, 2, 2, 2, 2, 2, 2, 2, 2, 2, 4 ),
 ( 0.000000000000000000, 0.003736383952885418379, 0.005604575929328127135, 0.007472767905770836758, 0.008406863893992191569, 0.009340959882213546381, 0.01120915185865624039, 0.01214324784687757092, 0.01307734383509889971, 0.01401143982332023023, 0.01494553581154155902, 0.01587963179976289302, 0.01681372778798422354, 0.01774782377620555407, 0.01868191976442688459, 0.01961601575264821859, 0.02055011174086954912, 0.02148420772909087964, 0.02241830371731221017, 0.02428649569375488856, 0.02615468767019756696, 0.02802287964664024883, 0.02989107162308292723 ),
 .UNSPECIFIED. ) ;
#50790=CARTESIAN_POINT ( 'NONE',  ( 102.8458551240039185, 25.60773946375956811, 9.002155561060931177 ) ) ;
#50791=CARTESIAN_POINT ( 'NONE',  ( -167.6386155194958576, 81.22597462185139250, 16.62036470824096313 ) ) ;
#50797=CARTESIAN_POINT ( 'NONE',  ( -7.825402957745087207, 6.891034867348159842, 71.96013162991091860 ) ) ;
#50801=CARTESIAN_POINT ( 'NONE',  ( 150.9013375937531123, 53.96275732797612079, 67.38256602799636141 ) ) ;
#50812=CARTESIAN_POINT ( 'NONE',  ( 63.01563776193090405, 12.67277567978497643, 71.65751152968501003 ) ) ;
#50813=CARTESIAN_POINT ( 'NONE',  ( -180.0179082103088035, 95.14811732286295864, -66.09535773320961027 ) ) ;
#50817=B_SPLINE_CURVE_WITH_KNOTS ( 'NONE', 3,
 ( #21313, #47019, #53659, #5484, #14661, #68477, #36123, #36467, #57923, #37842, #38182, #54704, #22357, #32908, #48364, #5818, #32566, #22703, #54346, #33624, #53993, #49421, #6873, #11793, #17417, #49771, #39244, #38533, #64576, #12506, #1251, #60340, #6168, #28325, #27275, #43107, #33964, #27630, #44514, #7230, #44144, #64929, #17788, #49068, #11436, #60688 ),
 .UNSPECIFIED., .F., .F.,
 ( 4, 2, 2, 2, 2, 2, 2, 2, 2, 2, 2, 2, 2, 2, 2, 2, 2, 2, 2, 2, 2, 2, 4 ),
 ( 3.179800655392250756E-17, 0.003373244802897452585, 0.004216556003621778001, 0.005059867204346101682, 0.006746489605794751647, 0.007589800806519077063, 0.008433112007243401612, 0.009276423207967727028, 0.01011973440869205071, 0.01180635681014071195, 0.01349297921158937492, 0.01433629041231369167, 0.01517960161303801361, 0.01686622401448661587, 0.01770953521521088925, 0.01855284641593516609, 0.02023946881738373713, 0.02108278001810798621, 0.02192609121883223183, 0.02361271362028073695, 0.02445602482100496175, 0.02529933602172918655, 0.02698595842317763269 ),
 .UNSPECIFIED. ) ;
#50818=CARTESIAN_POINT ( 'NONE',  ( -175.9970298498767249, 90.38640259140137800, 4.537318838786393194 ) ) ;
#50819=CARTESIAN_POINT ( 'NONE',  ( -2.174378755909794236, 6.588636630831475216, 15.72640502805996654 ) ) ;
#50820=CARTESIAN_POINT ( 'NONE',  ( 58.09877917144280701, 12.61383386832654452, -48.90516037375699909 ) ) ;
#50821=CARTESIAN_POINT ( 'NONE',  ( -86.10360257264194672, 26.38663017581291115, 38.92037401638386029 ) ) ;
#50823=CARTESIAN_POINT ( 'NONE',  ( 139.3067271572849677, 44.81402783181198402, 15.32414253876127930 ) ) ;
#50827=CARTESIAN_POINT ( 'NONE',  ( 116.6734749296699079, 31.97209464358268605, -39.53049973554296770 ) ) ;
#50828=CARTESIAN_POINT ( 'NONE',  ( -75.00452312211128003, 22.03104735285382532, 4.523913399809351255 ) ) ;
#50830=CARTESIAN_POINT ( 'NONE',  ( 42.71504753277076105, 8.863481902720385719, -36.38681058640105448 ) ) ;
#50831=EDGE_CURVE ( 'NONE', #60761, #41997, #67649, .T. ) ;
#50835=CARTESIAN_POINT ( 'NONE',  ( 79.38020582286198135, 17.07365509555549110, -45.31021711467555235 ) ) ;
#50836=AXIS2_PLACEMENT_3D ( 'NONE', #10061, #26586, #42416 ) ;
#50839=CARTESIAN_POINT ( 'NONE',  ( 86.62931800182293784, 20.48449268398423229, 44.71208757247933363 ) ) ;
#50842=VECTOR ( 'NONE', #47547, 1000.000000000000000 ) ;
#50843=CARTESIAN_POINT ( 'NONE',  ( -125.4481990864045855, 46.20056605584957765, 57.46449846362079228 ) ) ;
#50845=CARTESIAN_POINT ( 'NONE',  ( 21.08384185994383841, 7.735488641401683907, -91.38067577833801636 ) ) ;
#50846=CARTESIAN_POINT ( 'NONE',  ( -47.65155309726505806, 13.85482731128119838, 36.57865308283418670 ) ) ;
#50847=ORIENTED_EDGE ( 'NONE', *, *, #9397, .F. ) ;
#50849=CARTESIAN_POINT ( 'NONE',  ( 104.7147873368645179, 26.40702926859711042, 69.04812278364634892 ) ) ;
#50852=CARTESIAN_POINT ( 'NONE',  ( -189.2442476610617916, 107.0963225822736433, 65.70228303047002782 ) ) ;
#50855=CARTESIAN_POINT ( 'NONE',  ( -26.87327614295023892, 8.886070347947290671, -36.84684950165980410 ) ) ;
#50858=VERTEX_POINT ( 'NONE', #19509 ) ;
#50861=CARTESIAN_POINT ( 'NONE',  ( -10.91976120871578537, 7.112268444252506150, -49.75439377399378316 ) ) ;
#50862=CARTESIAN_POINT ( 'NONE',  ( -72.54743664134970516, 20.08440888238853717, 87.25848529910209095 ) ) ;
#50865=DIRECTION ( 'NONE',  ( -0.8160245890732938934, -0.5780171883497599028, 0.000000000000000000 ) ) ;
#50866=CARTESIAN_POINT ( 'NONE',  ( -56.72676045871359207, 16.18052435693490310, 30.50251775650468744 ) ) ;
#50868=CARTESIAN_POINT ( 'NONE',  ( 55.64941047419414843, 12.11006143146460978, 38.78652927538340123 ) ) ;
#50869=CARTESIAN_POINT ( 'NONE',  ( 31.99225359986736095, 7.561112794910904711, 89.89537387559623483 ) ) ;
#50872=CARTESIAN_POINT ( 'NONE',  ( -3.857727530059809062, 6.665032499723453796, -36.54875858820001611 ) ) ;
#50874=CARTESIAN_POINT ( 'NONE',  ( -14.33576511807126153, 8.413127487936186810, 14.52671630318449303 ) ) ;
#50877=CARTESIAN_POINT ( 'NONE',  ( -109.5025362253418706, 36.60371748273998094, -67.27247425872458564 ) ) ;
#50878=CARTESIAN_POINT ( 'NONE',  ( 130.7457207912711112, 40.74300766298685517, -23.51872159297877829 ) ) ;
#50882=CARTESIAN_POINT ( 'NONE',  ( 129.1052153257903683, 39.78893484542956571, -37.69982810349421243 ) ) ;
#50883=CARTESIAN_POINT ( 'NONE',  ( -126.3458714439411068, 46.79154809309480356, 3.775397282693374823 ) ) ;
#50884=DIRECTION ( 'NONE',  ( -0.000000000000000000, 1.000000000000000000, -0.000000000000000000 ) ) ;
#50887=FACE_OUTER_BOUND ( 'NONE', #43224, .T. ) ;
#50890=EDGE_CURVE ( 'NONE', #21908, #66303, #13888, .T. ) ;
#50898=CARTESIAN_POINT ( 'NONE',  ( 150.4653148198808879, 53.64543865262506017, 87.89445436269947720 ) ) ;
#50901=CARTESIAN_POINT ( 'NONE',  ( 130.3245512970360664, 39.33195360491887271, 43.64341809288409735 ) ) ;
#50904=CARTESIAN_POINT ( 'NONE',  ( -156.3734885497381129, 71.59531449004283843, 35.19087983619847648 ) ) ;
#50907=CARTESIAN_POINT ( 'NONE',  ( 79.38020582286199556, 17.07365509555549110, 8.378884066251806928 ) ) ;
#50910=CARTESIAN_POINT ( 'NONE',  ( 59.72526569420001152, 11.93313563009888867, 44.07029543158733276 ) ) ;
#50913=CARTESIAN_POINT ( 'NONE',  ( 175.0696098417091378, 74.11936424544845181, 32.32058490622820557 ) ) ;
#50914=EDGE_CURVE ( 'NONE', #25055, #52276, #29034, .T. ) ;
#50915=CARTESIAN_POINT ( 'NONE',  ( -31.43908319763710679, 10.61114334766713796, -89.00629854612920155 ) ) ;
#50917=CARTESIAN_POINT ( 'NONE',  ( -15.32584732649904247, 8.506915958926390076, -69.27421579052196421 ) ) ;
#50918=ORIENTED_EDGE ( 'NONE', *, *, #63202, .F. ) ;
#50919=CARTESIAN_POINT ( 'NONE',  ( -95.00922893699316774, 30.34910376528943132, 89.83886361574879231 ) ) ;
#50920=CARTESIAN_POINT ( 'NONE',  ( -23.99957301099516727, 9.503061049698466434, 36.73396631618189900 ) ) ;
#50921=CARTESIAN_POINT ( 'NONE',  ( -71.86568654225716557, 20.91200104397924875, -45.78763654518949267 ) ) ;
#50923=B_SPLINE_CURVE_WITH_KNOTS ( 'NONE', 3,
 ( #39517, #1898, #65924, #39860, #6464, #27912, #49349, #12790, #1183, #16997, #44075, #66611, #7522, #18404, #2239, #838, #28973, #65559, #61316, #12090, #59906, #38826, #60275, #6802, #54984, #28254, #17719, #12437, #50419, #33896, #34248, #13479, #67307, #9237, #14849, #14169, #24733, #24389, #45831, #25077, #67991, #51463, #57424, #40897 ),
 .UNSPECIFIED., .F., .F.,
 ( 4, 2, 2, 2, 2, 2, 2, 2, 2, 2, 2, 2, 2, 2, 2, 2, 2, 2, 2, 2, 2, 4 ),
 ( 0.02432640572110343277, 0.02583721026359366707, 0.02659261253483879983, 0.02734801480608393259, 0.02885881934857420852, 0.02961422161981933088, 0.03036962389106444976, 0.03188042843355469447, 0.03339123297604493917, 0.03414663524729004418, 0.03490203751853514919, 0.03641284206102534532, 0.03716824433227044339, 0.03792364660351554145, 0.03943445114600568902, 0.04094525568849584352, 0.04245606023098599802, 0.04396686477347614558, 0.04472226704472121589, 0.04547766931596629314, 0.04698847385845641295, 0.04849927840094653275 ),
 .UNSPECIFIED. ) ;
#50924=CARTESIAN_POINT ( 'NONE',  ( 210.6584452238134588, 116.7138338345753681, -75.24916677418407573 ) ) ;
#50925=CARTESIAN_POINT ( 'NONE',  ( 139.7883986595928434, 46.32091287009617986, 32.41387198680679660 ) ) ;
#50926=CARTESIAN_POINT ( 'NONE',  ( 218.0000000000000000, 126.6235316737731296, 94.99999999999866418 ) ) ;
#50927=CARTESIAN_POINT ( 'NONE',  ( -127.4644500646574556, 48.74852676951797292, 3.938189400447978716 ) ) ;
#50928=CARTESIAN_POINT ( 'NONE',  ( 63.01563776193091826, 13.70579113808094718, -77.56524142263344856 ) ) ;
#50929=B_SPLINE_CURVE_WITH_KNOTS ( 'NONE', 3,
 ( #5541, #69555, #15758, #64287, #16097, #26996, #21717, #59001, #10820, #43165, #32973, #64639, #54406, #6231, #37903, #27687, #49128, #971, #28386, #24170, #13266, #23818, #18883, #3060, #2023, #45613, #60746, #18192, #44573, #55115, #7982, #7648, #40333, #51246, #61780, #29434, #17481, #49833, #34382, #65692, #44207, #50198, #66050, #8336, #12925, #13603, #6936, #23480, #29780, #12219, #33685, #35060, #1659, #29099, #67095, #66402, #55467, #2365 ),
 .UNSPECIFIED., .F., .F.,
 ( 4, 2, 2, 2, 2, 2, 2, 2, 2, 2, 2, 2, 2, 2, 2, 2, 2, 2, 2, 2, 2, 2, 2, 2, 2, 2, 2, 2, 4 ),
 ( 0.000000000000000000, 0.001128500949314689087, 0.002257001898629378174, 0.003385502847944066827, 0.003949753322601412021, 0.004514003797258757215, 0.005642504746573493574, 0.006771005695888229065, 0.007899506645202964555, 0.009028007594517700046, 0.01128500949314724215, 0.01354201139177678079, 0.01579901329040632116, 0.01805601518903586153, 0.01918451613835061437, 0.02031301708766536721, 0.02257001898629487982, 0.02369851993560962919, 0.02482702088492437509, 0.02708402278355386689, 0.02821252373286863707, 0.02934102468218340726, 0.03046952563149817397, 0.03159802658081294069, 0.03216227705547035354, 0.03272652753012775945, 0.03385502847944261984, 0.03498352942875748023, 0.03611203037807233368 ),
 .UNSPECIFIED. ) ;
#50941=CARTESIAN_POINT ( 'NONE',  ( -125.8938041572051105, 46.49392987655492959, 57.46449846362076386 ) ) ;
#50945=DIRECTION ( 'NONE',  ( 0.000000000000000000, 0.000000000000000000, 1.000000000000000000 ) ) ;
#50947=CARTESIAN_POINT ( 'NONE',  ( -94.96454763573188984, 30.32814623986933000, -94.53419202597292781 ) ) ;
#50949=CARTESIAN_POINT ( 'NONE',  ( 84.27937148876358719, 19.69225537006224158, 56.93023493300005100 ) ) ;
#50951=CARTESIAN_POINT ( 'NONE',  ( 188.2133404574781537, 86.12414067617872604, 39.15481199342811891 ) ) ;
#50954=CARTESIAN_POINT ( 'NONE',  ( 39.40195752203892710, 8.409560354027389550, 18.06928371549960133 ) ) ;
#50959=CARTESIAN_POINT ( 'NONE',  ( -108.2330097037575598, 35.90915053323784178, -91.63594520124935627 ) ) ;
#50960=CARTESIAN_POINT ( 'NONE',  ( 173.9832054143776077, 73.09312616907610050, -95.00000000000133582 ) ) ;
#50961=EDGE_LOOP ( 'NONE', ( #2279, #34138, #11425, #524 ) ) ;
#50963=CARTESIAN_POINT ( 'NONE',  ( -62.15063206372443005, 17.75106610013994057, 62.18892694254114417 ) ) ;
#50967=CARTESIAN_POINT ( 'NONE',  ( 150.4542242713869484, 53.63744268572192198, -67.80470997374955289 ) ) ;
#50968=CARTESIAN_POINT ( 'NONE',  ( -31.43908319763710679, 9.591432048623758533, 45.21645440618919309 ) ) ;
#50969=( BOUNDED_CURVE ( )  B_SPLINE_CURVE ( 3, ( #36310, #57765, #13808, #4305 ),
 .UNSPECIFIED., .F., .F. ) 
 B_SPLINE_CURVE_WITH_KNOTS ( ( 4, 4 ),
 ( 2.506209174768084136, 3.776976132411494103 ),
 .UNSPECIFIED. ) 
 CURVE ( )  GEOMETRIC_REPRESENTATION_ITEM ( )  RATIONAL_B_SPLINE_CURVE ( ( 1.000000000000000000, 0.8698961108463048042, 0.8698961108463048042, 1.000000000000000000 ) ) 
 REPRESENTATION_ITEM ( '' )  );
#50970=CARTESIAN_POINT ( 'NONE',  ( 137.4117721579688123, 43.61242559081433257, -36.90228539602491509 ) ) ;
#50972=SHAPE_REPRESENTATION_RELATIONSHIP ( 'NONE' , 'NONE' ,  #45199, #63416 ) ;
#50975=ORIENTED_EDGE ( 'NONE', *, *, #59522, .F. ) ;
#50977=CARTESIAN_POINT ( 'NONE',  ( 188.5837490358996433, 86.53279111916964439, 9.653281778228306464 ) ) ;
#50978=CARTESIAN_POINT ( 'NONE',  ( 92.51858280840788495, 21.51505926344914243, 59.38593706081789492 ) ) ;
#50984=CARTESIAN_POINT ( 'NONE',  ( -121.1775535805057444, 43.46577565517554831, -63.40630286045660569 ) ) ;
#50989=CARTESIAN_POINT ( 'NONE',  ( 69.73342236697678231, 14.33173522011652068, 60.78623098035528471 ) ) ;
#50990=CARTESIAN_POINT ( 'NONE',  ( 135.0005116824453921, 43.29964618809725607, 2.749954276746684023 ) ) ;
#50998=FACE_OUTER_BOUND ( 'NONE', #34777, .T. ) ;
#50999=ORIENTED_EDGE ( 'NONE', *, *, #20170, .F. ) ;
#51000=CARTESIAN_POINT ( 'NONE',  ( 69.72789637502502558, 15.37065610545702121, 60.80231955136558497 ) ) ;
#51001=CARTESIAN_POINT ( 'NONE',  ( 126.4177291868981428, 37.11054216252123439, 91.72012540680618997 ) ) ;
#51005=CARTESIAN_POINT ( 'NONE',  ( 160.9097745014957184, 61.67033591969549633, -36.95542617067341240 ) ) ;
#51009=B_SPLINE_CURVE_WITH_KNOTS ( 'NONE', 3,
 ( #25799, #26131, #47566, #51824, #69022, #20849, #37032, #58470, #10282, #3634, #14541, #11320, #38060, #59161, #43326, #16257, #16944, #1131, #42649, #37713, #48248, #11673, #10978, #27155, #78, #22582, #32446, #64448, #44022, #64105, #48940, #64802, #32788, #427, #65500, #21877, #53875, #48587, #31747, #60215, #5364, #15916, #59504, #58817, #17299, #54220, #42976, #69379 ),
 .UNSPECIFIED., .F., .F.,
 ( 4, 2, 2, 2, 2, 2, 2, 2, 2, 2, 2, 2, 2, 2, 2, 2, 2, 2, 2, 2, 2, 2, 2, 4 ),
 ( 1.734723475976807094E-18, 0.003619254076116414955, 0.004524067595145476843, 0.005428881114174538731, 0.007238508152232685060, 0.008143321671261782510, 0.009048135190290882562, 0.01085776222834906012, 0.01176257574737815496, 0.01266738926640724981, 0.01357220278543634640, 0.01447701630446544124, 0.01538182982349453609, 0.01628664334252363094, 0.01719145686155273273, 0.01809627038058182757, 0.01900108389961092242, 0.01990589741864001727, 0.02171552445669828330, 0.02262033797572741978, 0.02352515149475655626, 0.02533477853281483616, 0.02714440557087311606, 0.02895403260893138903 ),
 .UNSPECIFIED. ) ;
#51012=CARTESIAN_POINT ( 'NONE',  ( 57.46055693957354293, 12.48011040142442241, 85.95216039237527639 ) ) ;
#51014=CARTESIAN_POINT ( 'NONE',  ( 81.04027388895738682, 18.64386073872847760, -11.45175216555015041 ) ) ;
#51015=CARTESIAN_POINT ( 'NONE',  ( -174.6851410627011774, 90.41141687855389364, -88.55546965300769102 ) ) ;
#51017=CARTESIAN_POINT ( 'NONE',  ( 126.4754729582248132, 37.14269484129876275, -69.01268951799154650 ) ) ;
#51019=CARTESIAN_POINT ( 'NONE',  ( -99.10904156412046007, 32.31949011661291138, 71.67685420465566892 ) ) ;
#51020=CARTESIAN_POINT ( 'NONE',  ( -14.33576511807126685, 8.413127487936190363, 68.21581748411188073 ) ) ;
#51021=ORIENTED_EDGE ( 'NONE', *, *, #66117, .T. ) ;
#51022=CARTESIAN_POINT ( 'NONE',  ( -152.9008427825210958, 68.45483453645053373, -49.00505458194412256 ) ) ;
#51023=CARTESIAN_POINT ( 'NONE',  ( 204.6977192012829789, 108.0580384837234931, -9.481380442157895772 ) ) ;
#51024=CARTESIAN_POINT ( 'NONE',  ( -36.89224332184167565, 11.57404295377976311, 32.56159292348578305 ) ) ;
#51027=CARTESIAN_POINT ( 'NONE',  ( -47.56463531432802228, 12.80077789972090407, -69.07071056560511124 ) ) ;
#51028=CARTESIAN_POINT ( 'NONE',  ( 205.0999694062794276, 106.8955893716605203, -51.32593103262163226 ) ) ;
#51029=CARTESIAN_POINT ( 'NONE',  ( 178.4027079424739100, 75.93756746109791322, 16.97168195328412210 ) ) ;
#51030=CARTESIAN_POINT ( 'NONE',  ( -56.72814287166056602, 15.13700122306437379, 18.28720868321791571 ) ) ;
#51036=CARTESIAN_POINT ( 'NONE',  ( 43.96062659677687634, 10.06332325923986204, -10.29970569430655303 ) ) ;
#51038=CARTESIAN_POINT ( 'NONE',  ( 46.13320811200729565, 9.380653113584040526, 60.91438470745498535 ) ) ;
#51041=CARTESIAN_POINT ( 'NONE',  ( -102.7494334820056849, 34.14986869751099618, -8.170026674512229192 ) ) ;
#51045=CARTESIAN_POINT ( 'NONE',  ( -167.6386155194957723, 81.22597462185137829, 70.30946588916833662 ) ) ;
#51047=VERTEX_POINT ( 'NONE', #65543 ) ;
#51048=AXIS2_PLACEMENT_3D ( 'NONE', #2984, #56431, #40600 ) ;
#51051=CARTESIAN_POINT ( 'NONE',  ( 173.5837434292113812, 71.34409607026157119, -17.16855947548079442 ) ) ;
#51053=CARTESIAN_POINT ( 'NONE',  ( 106.0228389049370605, 28.07756796303168301, 57.75107945049343527 ) ) ;
#51056=CARTESIAN_POINT ( 'NONE',  ( 55.57634120535661992, 12.09544293553729943, -15.39196884852826841 ) ) ;
#51059=CARTESIAN_POINT ( 'NONE',  ( 18.19858669090299585, 7.596860100017451600, -35.91253959148980357 ) ) ;
#51062=FACE_BOUND ( 'NONE', #16255, .T. ) ;
#51068=DIRECTION ( 'NONE',  ( -0.000000000000000000, 1.000000000000000000, -0.000000000000000000 ) ) ;
#51070=FACE_OUTER_BOUND ( 'NONE', #18906, .T. ) ;
#51076=DIRECTION ( 'NONE',  ( -0.000000000000000000, 1.000000000000000000, -0.000000000000000000 ) ) ;
#51078=EDGE_LOOP ( 'NONE', ( #1070, #10896 ) ) ;
#51080=EDGE_LOOP ( 'NONE', ( #38960, #68220 ) ) ;
#51082=CARTESIAN_POINT ( 'NONE',  ( -86.10361028793437299, 25.29528064050657221, -70.46168237689222735 ) ) ;
#51085=EDGE_CURVE ( 'NONE', #7668, #54444, #16425, .T. ) ;
#51087=VERTEX_POINT ( 'NONE', #48627 ) ;
#51088=CARTESIAN_POINT ( 'NONE',  ( 42.71247067544612719, 9.879726907348446829, 57.52408926830288038 ) ) ;
#51090=CARTESIAN_POINT ( 'NONE',  ( -102.6996017731805750, 34.12480707976105521, -88.71245073017188076 ) ) ;
#51093=EDGE_LOOP ( 'NONE', ( #47074, #41203 ) ) ;
#51097=CARTESIAN_POINT ( 'NONE',  ( 173.7263186949344345, 72.85225335320953377, -72.05203316818773374 ) ) ;
#51101=CARTESIAN_POINT ( 'NONE',  ( 79.91920957766411959, 18.29292522273510357, -39.93360915899626207 ) ) ;
#51102=CARTESIAN_POINT ( 'NONE',  ( -102.2801239173131194, -170.0000000000000000, -96.20367844590329298 ) ) ;
#51104=ORIENTED_EDGE ( 'NONE', *, *, #65947, .T. ) ;
#51105=ORIENTED_EDGE ( 'NONE', *, *, #7722, .F. ) ;
#51106=CARTESIAN_POINT ( 'NONE',  ( 41.80536115778103579, 8.734184316430665618, 3.460590674310346504 ) ) ;
#51107=LINE ( 'NONE', #8194, #9133 ) ;
#51108=CARTESIAN_POINT ( 'NONE',  ( -47.95468448182518983, 12.89252559348045679, -13.43679395526418396 ) ) ;
#51109=CARTESIAN_POINT ( 'NONE',  ( 103.1567541746301657, 25.73937982110324896, -19.08631000368835373 ) ) ;
#51112=CARTESIAN_POINT ( 'NONE',  ( 205.5119110209522830, 109.1913085791014453, 82.92244948186888109 ) ) ;
#51113=CARTESIAN_POINT ( 'NONE',  ( 204.6977192012829505, 108.0580384837234931, 29.20772073876942088 ) ) ;
#51114=FACE_OUTER_BOUND ( 'NONE', #19741, .T. ) ;
#51115=CARTESIAN_POINT ( 'NONE',  ( -8.811275908848678284, 6.956777180392053950, 30.16455914700392427 ) ) ;
#51116=ORIENTED_EDGE ( 'NONE', *, *, #66168, .F. ) ;
#51121=CARTESIAN_POINT ( 'NONE',  ( 188.4918087359956473, 87.93403732562657638, -71.78073924401245165 ) ) ;
#51122=CARTESIAN_POINT ( 'NONE',  ( -165.7149569557575717, 80.68479365246975021, 39.54250311673061447 ) ) ;
#51123=CARTESIAN_POINT ( 'NONE',  ( 209.4789161463551750, 113.1367444519304257, -76.45320715356564278 ) ) ;
#51124=CARTESIAN_POINT ( 'NONE',  ( -26.49928411671542960, 9.848831533840664676, 16.53656075554865623 ) ) ;
#51127=DIRECTION ( 'NONE',  ( -0.000000000000000000, 1.000000000000000000, -0.000000000000000000 ) ) ;
#51128=CARTESIAN_POINT ( 'NONE',  ( 126.4324872316703079, 37.11876756822024959, -42.42733774312184636 ) ) ;
#51130=ORIENTED_EDGE ( 'NONE', *, *, #36455, .F. ) ;
#51133=CARTESIAN_POINT ( 'NONE',  ( 188.4735550466079417, 87.91368577883815760, 89.15183869550180873 ) ) ;
#51135=CARTESIAN_POINT ( 'NONE',  ( 217.9999999999999716, 126.6235316737731580, -95.00000000000133582 ) ) ;
#51136=CARTESIAN_POINT ( 'NONE',  ( -29.02794087136070900, 9.207646203414357799, -62.54324267984874552 ) ) ;
#51139=VERTEX_POINT ( 'NONE', #26859 ) ;
#51140=CARTESIAN_POINT ( 'NONE',  ( 39.40195752203892710, 9.424259417798133143, -77.46436805589148378 ) ) ;
#51142=B_SPLINE_CURVE_WITH_KNOTS ( 'NONE', 3,
 ( #18339, #33832, #39802, #66901, #34880, #34190, #56319, #8139, #44733, #49640, #1468, #49287 ),
 .UNSPECIFIED., .F., .F.,
 ( 4, 2, 2, 2, 2, 4 ),
 ( 0.000000000000000000, 0.002491861676607965564, 0.004983723353215931129, 0.007475585029823895826, 0.008721515868127872537, 0.009967446706431848380 ),
 .UNSPECIFIED. ) ;
#51143=CARTESIAN_POINT ( 'NONE',  ( -60.47589866267035319, 17.25153113855768439, -74.74728964359273675 ) ) ;
#51144=CARTESIAN_POINT ( 'NONE',  ( 197.5344433744249386, 98.61756151884685551, -68.42576040693960238 ) ) ;
#51151=CARTESIAN_POINT ( 'NONE',  ( -47.61380558691494969, 12.81230778489787347, 65.64890909038182087 ) ) ;
#51155=CARTESIAN_POINT ( 'NONE',  ( -4.081377963939787357, 6.676029627840589065, 57.95687600658722971 ) ) ;
#51156=EDGE_CURVE ( 'NONE', #18323, #37531, #47429, .T. ) ;
#51159=CARTESIAN_POINT ( 'NONE',  ( 152.6804161981488619, 55.27286404993338920, 57.97779815228713574 ) ) ;
#51173=CARTESIAN_POINT ( 'NONE',  ( -175.9852529046322616, 90.37283472601129120, 18.42162745504879595 ) ) ;
#51174=CARTESIAN_POINT ( 'NONE',  ( -0.7174461528505752250, 6.532311451815527192, 13.17673894021459446 ) ) ;
#51179=CARTESIAN_POINT ( 'NONE',  ( 153.4645101005155539, 54.60099007857102293, 84.22599575989748644 ) ) ;
#51180=CARTESIAN_POINT ( 'NONE',  ( 138.1919700334460970, 44.10401742531043823, 4.027875862906625137 ) ) ;
#51185=CARTESIAN_POINT ( 'NONE',  ( -71.26746920569851795, 20.70422440535243425, 9.820768664776275969 ) ) ;
#51188=CARTESIAN_POINT ( 'NONE',  ( -118.9648984637947819, 42.09776532027431273, 94.69885810538663407 ) ) ;
#51190=CARTESIAN_POINT ( 'NONE',  ( 79.14242532928585661, 17.00090225993928428, -42.81185340043884224 ) ) ;
#51198=CARTESIAN_POINT ( 'NONE',  ( -121.2008155373973750, 43.48033530165982796, 59.09401072938392474 ) ) ;
#51199=CARTESIAN_POINT ( 'NONE',  ( -85.96384504792887071, 26.32782846176033331, -14.02102585345735974 ) ) ;
#51200=CARTESIAN_POINT ( 'NONE',  ( -180.3114074031035727, 97.09758726817784691, -17.52189378749824300 ) ) ;
#51202=CARTESIAN_POINT ( 'NONE',  ( -51.34562532494748410, 14.75613283840036871, 44.35518551528009112 ) ) ;
#51203=ORIENTED_EDGE ( 'NONE', *, *, #51156, .F. ) ;
#51206=CARTESIAN_POINT ( 'NONE',  ( -109.5157885508426432, 37.76058765671429995, 13.21563288999418617 ) ) ;
#51208=CARTESIAN_POINT ( 'NONE',  ( 161.7048274740120632, 61.01946783654761219, 57.54637987710646030 ) ) ;
#51209=CYLINDRICAL_SURFACE ( 'NONE', #21698, 7.500000000000020428 ) ;
#51210=CARTESIAN_POINT ( 'NONE',  ( 182.5617509987553149, 80.11195108039724744, -51.08114882856880712 ) ) ;
#51211=CARTESIAN_POINT ( 'NONE',  ( 15.78827728214693416, 6.500811158483284835, 30.01470767270522089 ) ) ;
#51212=CARTESIAN_POINT ( 'NONE',  ( 160.5141379054754225, 60.05651755415393467, -63.59944546789614606 ) ) ;
#51218=CARTESIAN_POINT ( 'NONE',  ( -71.43680309721476362, 19.69815736714263466, 89.58515710192457959 ) ) ;
#51219=CARTESIAN_POINT ( 'NONE',  ( 177.6913206243945638, 75.24308051341677128, -90.71550574208795581 ) ) ;
#51220=CARTESIAN_POINT ( 'NONE',  ( 70.51484748609223630, 14.53801151001411895, -43.73266891657371502 ) ) ;
#51222=CARTESIAN_POINT ( 'NONE',  ( -62.29496909743952671, 17.79481128341707930, 39.78269874340612944 ) ) ;
#51224=CARTESIAN_POINT ( 'NONE',  ( 58.08938767906775524, 12.61185010801510131, 42.98944077952003084 ) ) ;
#51225=CARTESIAN_POINT ( 'NONE',  ( 40.71722863567654827, 8.584032429807034958, 83.71188065785378285 ) ) ;
#51228=CYLINDRICAL_SURFACE ( 'NONE', #67724, 7.500000000000020428 ) ;
#51230=CARTESIAN_POINT ( 'NONE',  ( -190.6985136298602015, 109.1272424661243434, -37.65993730791821292 ) ) ;
#51234=CARTESIAN_POINT ( 'NONE',  ( 19.11382977197791888, 7.636807742668410448, -9.434045545063515448 ) ) ;
#51235=CARTESIAN_POINT ( 'NONE',  ( 198.3926538463958593, 98.07933330386025261, 67.65304937739811919 ) ) ;
#51239=EDGE_LOOP ( 'NONE', ( #54567, #55589 ) ) ;
#51242=DIRECTION ( 'NONE',  ( -0.000000000000000000, 1.000000000000000000, -0.000000000000000000 ) ) ;
#51243=CARTESIAN_POINT ( 'NONE',  ( -125.8938041572051105, 46.49392987655492959, 3.775397282693376599 ) ) ;
#51245=EDGE_CURVE ( 'NONE', #38218, #5375, #40712, .T. ) ;
#51246=CARTESIAN_POINT ( 'NONE',  ( -170.0422773253271203, 83.76581591185905040, 85.16679510493294458 ) ) ;
#51248=VECTOR ( 'NONE', #65234, 1000.000000000000000 ) ;
#51250=VECTOR ( 'NONE', #62410, 1000.000000000000000 ) ;
#51258=CARTESIAN_POINT ( 'NONE',  ( 160.7775378522616450, 61.56282986428943360, 83.85992522728291476 ) ) ;
#51262=CARTESIAN_POINT ( 'NONE',  ( -151.6797345123118532, 67.37848486615945376, 45.41297040107649252 ) ) ;
#51265=CARTESIAN_POINT ( 'NONE',  ( 204.6977192012829789, 106.3443248447423457, 44.20772073876944575 ) ) ;
#51268=CARTESIAN_POINT ( 'NONE',  ( 56.19513604272051310, 11.19349063094192687, 40.44209435148105314 ) ) ;
#51269=ORIENTED_EDGE ( 'NONE', *, *, #37012, .T. ) ;
#51270=ORIENTED_EDGE ( 'NONE', *, *, #1113, .F. ) ;
#51271=CARTESIAN_POINT ( 'NONE',  ( -165.9154624515710168, 80.89088623112733956, 13.57877339069360900 ) ) ;
#51272=CARTESIAN_POINT ( 'NONE',  ( 21.73827885904430701, 6.764046335627709183, -74.43606220462095280 ) ) ;
#51273=CARTESIAN_POINT ( 'NONE',  ( -128.7724923851857852, 49.63576597317773320, 71.89386820983963844 ) ) ;
#51274=VERTEX_POINT ( 'NONE', #47874 ) ;
#51275=CARTESIAN_POINT ( 'NONE',  ( -97.82962700614261564, 31.69462283565845695, 85.66353045367125674 ) ) ;
#51276=CARTESIAN_POINT ( 'NONE',  ( -75.00452312211128003, 22.03104735285380400, -49.16518778111800714 ) ) ;
#51278=B_SPLINE_CURVE_WITH_KNOTS ( 'NONE', 3,
 ( #43902, #17889, #66445, #22812, #18232, #39003, #65383, #7339, #23169, #33725, #60447, #55874, #44616, #54450, #55157, #16827, #50243, #6632, #39344, #27732, #28795, #28080, #22461, #65736, #29136, #6279, #17171, #38643, #39687, #50587, #49885, #60084, #60787, #12610, #11906, #33383, #34071, #54809, #2408, #55512, #61145, #12968, #23863, #45305 ),
 .UNSPECIFIED., .F., .F.,
 ( 4, 2, 2, 2, 2, 2, 2, 2, 2, 2, 2, 2, 2, 2, 2, 2, 2, 2, 2, 2, 2, 4 ),
 ( 7.152448122690996019E-18, 0.001476829494128853752, 0.002215244241193284423, 0.002953658988257715744, 0.004430488482386571447, 0.005907317976515427151, 0.007384147470644282854, 0.008122562217708703333, 0.008860976964773122078, 0.01033780645890195089, 0.01181463595303078144, 0.01255305070009518631, 0.01329146544715958944, 0.01476829494128840091, 0.01550670968835280925, 0.01624512443541721585, 0.01772195392954603946, 0.01919878342367485960, 0.01993719817073927661, 0.02067561291780369362, 0.02215244241193250682, 0.02362927190606132002 ),
 .UNSPECIFIED. ) ;
#51279=CARTESIAN_POINT ( 'NONE',  ( 209.6642862813004626, 115.2127693334913658, -76.30817762714391961 ) ) ;
#51282=LINE ( 'NONE', #50926, #53821 ) ;
#51283=CARTESIAN_POINT ( 'NONE',  ( -132.4896623150434323, 52.22616402022728721, 14.85463847962715356 ) ) ;
#51284=CARTESIAN_POINT ( 'NONE',  ( 63.01563776193090405, 13.70579113808097382, -62.56524142263340593 ) ) ;
#51285=ORIENTED_EDGE ( 'NONE', *, *, #53580, .F. ) ;
#51288=CARTESIAN_POINT ( 'NONE',  ( -142.1332311300252798, 59.44822332309654911, -16.86392425921542682 ) ) ;
#51292=CARTESIAN_POINT ( 'NONE',  ( -49.09658814250866499, 13.16488830565666390, -91.82710492038845018 ) ) ;
#51294=B_SPLINE_CURVE_WITH_KNOTS ( 'NONE', 3,
 ( #47057, #36162, #47732, #8751, #4496, #46710, #69195, #19990, #42466, #31240, #4832, #63584, #15053, #68514, #46355, #9434, #30889, #51652, #68186, #41442, #42125, #14366, #20322, #52336, #15397, #36856, #36506, #57958, #9779, #52670, #25956, #3461, #47387, #68844, #58296, #67837, #31572, #53007, #26304, #19634, #21021, #63926, #62556 ),
 .UNSPECIFIED., .F., .F.,
 ( 4, 2, 2, 2, 2, 2, 2, 2, 2, 2, 2, 2, 1, 2, 2, 2, 2, 2, 2, 2, 2, 4 ),
 ( 0.02358007599568756954, 0.02505677178601661836, 0.02579511968118113757, 0.02653346757634565331, 0.02801016336667470560, 0.02948685915700375443, 0.03022520705216828404, 0.03096355494733281366, 0.03244025073766187289, 0.03391694652799093213, 0.03539364231831998442, 0.03613199021348451057, 0.03687033810864902977, 0.03760868600381355592, 0.03834703389897807513, 0.03982372968930711354, 0.04130042547963615196, 0.04277712126996519038, 0.04351546916512971652, 0.04425381706029422879, 0.04573051285062329496, 0.04720720864095235419 ),
 .UNSPECIFIED. ) ;
#51296=ADVANCED_FACE ( 'NONE', ( #25755 ), #36649, .F. ) ;
#51298=CARTESIAN_POINT ( 'NONE',  ( 206.2980740120524104, 108.5619562183279925, 56.21387322886499049 ) ) ;
#51300=ORIENTED_EDGE ( 'NONE', *, *, #54829, .T. ) ;
#51301=CARTESIAN_POINT ( 'NONE',  ( -109.7686203588201153, 37.90089348911613598, 38.51078262366649341 ) ) ;
#51303=CARTESIAN_POINT ( 'NONE',  ( -179.9818533554779094, 95.10411966562014641, -92.82201583766619990 ) ) ;
#51305=EDGE_CURVE ( 'NONE', #62204, #62313, #37668, .T. ) ;
#51306=CARTESIAN_POINT ( 'NONE',  ( 82.14396250120410059, 18.99560174459420736, 58.04072448712305743 ) ) ;
#51307=ORIENTED_EDGE ( 'NONE', *, *, #48, .F. ) ;
#51310=FACE_OUTER_BOUND ( 'NONE', #1233, .T. ) ;
#51312=CARTESIAN_POINT ( 'NONE',  ( 33.03621582719335237, 7.666716336587112046, 6.595962476436807442 ) ) ;
#51313=DIRECTION ( 'NONE',  ( -0.000000000000000000, 1.000000000000000000, -0.000000000000000000 ) ) ;
#51314=CARTESIAN_POINT ( 'NONE',  ( 150.5550643769628323, 52.46819381604269239, -46.53967426915813377 ) ) ;
#51319=CARTESIAN_POINT ( 'NONE',  ( -62.55184817504200367, 17.87278652436700099, 64.14626842136314622 ) ) ;
#51327=ADVANCED_FACE ( 'NONE', ( #22190 ), #69337, .F. ) ;
#51330=CARTESIAN_POINT ( 'NONE',  ( -118.3960663196801306, 41.75130200162920602, 37.55200035001683290 ) ) ;
#51333=CARTESIAN_POINT ( 'NONE',  ( -177.1381400275772080, 93.26609858452818003, -75.40501691932175277 ) ) ;
#51334=CARTESIAN_POINT ( 'NONE',  ( 90.30166390191402570, 20.70652093100730440, 57.49911369470580524 ) ) ;
#51336=CARTESIAN_POINT ( 'NONE',  ( 199.7286177451876199, 101.4075663537892069, -22.61804941524460233 ) ) ;
#51340=CARTESIAN_POINT ( 'NONE',  ( 200.8410151090926661, 101.2014854111317419, 43.15449351457530014 ) ) ;
#51343=CARTESIAN_POINT ( 'NONE',  ( 70.51484748609223630, 14.53801151001409409, 63.64553344528102485 ) ) ;
#51344=CARTESIAN_POINT ( 'NONE',  ( 184.5165707593032209, 82.14321753839030293, -90.70306685600688468 ) ) ;
#51348=B_SPLINE_CURVE_WITH_KNOTS ( 'NONE', 3,
 ( #65570, #60975, #23698, #45140, #34258, #66620, #18416, #54647, #27921, #49010, #847, #49360, #22299, #43737, #1194, #17359, #38838, #60286, #12099, #33569, #30015, #2936, #4567, #58367, #35291, #8212, #42206, #26031, #26376, #56746, #51475, #13152, #14181, #45488, #13489, #52741, #3285, #8564, #2588, #29319, #19104, #40221, #67318, #63667 ),
 .UNSPECIFIED., .F., .F.,
 ( 4, 2, 2, 2, 2, 2, 2, 2, 2, 2, 2, 2, 2, 2, 2, 2, 2, 2, 2, 2, 2, 4 ),
 ( 0.02495775893651561508, 0.02650251144344301438, 0.02804726395037041367, 0.02959201645729781296, 0.03113676896422521226, 0.03268152147115261502, 0.03345389772461631467, 0.03422627397808002125, 0.03577102648500744136, 0.03654340273847116183, 0.03731577899193488229, 0.03808815524539860276, 0.03886053149886233016, 0.04040528400578975721, 0.04117766025925346379, 0.04195003651271717038, 0.04349478901964456967, 0.04503954152657196897, 0.04581191778003566861, 0.04658429403349936826, 0.04812904654042682306, 0.04967379904735427093 ),
 .UNSPECIFIED. ) ;
#51349=CARTESIAN_POINT ( 'NONE',  ( 163.5944442552010401, 63.88381951184481267, -12.44276307209138821 ) ) ;
#51353=CARTESIAN_POINT ( 'NONE',  ( 133.6177090015579267, 41.28025736076558161, 83.19673575245394659 ) ) ;
#51356=CARTESIAN_POINT ( 'NONE',  ( -148.6409722988650515, 63.44808865916662199, -61.70444773994812238 ) ) ;
#51358=CARTESIAN_POINT ( 'NONE',  ( 164.0158927577712689, 62.92463143894070043, -47.32386914606765771 ) ) ;
#51364=CARTESIAN_POINT ( 'NONE',  ( -178.7653014892675571, 95.21116012989124044, -90.95673312123581411 ) ) ;
#51365=CARTESIAN_POINT ( 'NONE',  ( -144.2204146883836415, 59.82124005924111998, -90.66219284191375039 ) ) ;
#51366=CARTESIAN_POINT ( 'NONE',  ( 94.06699947028484132, 23.17027898120150908, 36.21459868573237628 ) ) ;
#51367=ORIENTED_EDGE ( 'NONE', *, *, #8041, .F. ) ;
#51369=FACE_OUTER_BOUND ( 'NONE', #25836, .T. ) ;
#51370=ORIENTED_EDGE ( 'NONE', *, *, #52765, .T. ) ;
#51371=CARTESIAN_POINT ( 'NONE',  ( 154.4435090467314069, 56.59612921827835663, -9.913691618128661176 ) ) ;
#51374=CARTESIAN_POINT ( 'NONE',  ( -37.93983213483221562, 11.77368372188049683, 41.48890555333869656 ) ) ;
#51375=CARTESIAN_POINT ( 'NONE',  ( -157.0069704378502138, 70.81086990254192415, -68.57520080848023269 ) ) ;
#51377=CARTESIAN_POINT ( 'NONE',  ( 55.52382973330894345, 11.05893590846274499, 90.51414599712177278 ) ) ;
#51378=CARTESIAN_POINT ( 'NONE',  ( -51.35181696773308602, 13.72007042346227834, -76.10265169357263915 ) ) ;
#51383=ORIENTED_EDGE ( 'NONE', *, *, #42878, .T. ) ;
#51388=CARTESIAN_POINT ( 'NONE',  ( 102.7571040248400749, 25.57023079238895491, -69.73951755044804202 ) ) ;
#51391=CARTESIAN_POINT ( 'NONE',  ( 41.33692564073609077, 8.668977654195472837, 57.00815978476482115 ) ) ;
#51394=CARTESIAN_POINT ( 'NONE',  ( -3.819748713895199099, 6.663105659409133352, 84.95562319304882237 ) ) ;
#51396=CARTESIAN_POINT ( 'NONE',  ( -108.6622665321723247, 37.28993738537008795, -19.61751752820619643 ) ) ;
#51400=CARTESIAN_POINT ( 'NONE',  ( -168.7150276173048269, 82.35404041280330034, 71.25389808330632491 ) ) ;
#51405=CARTESIAN_POINT ( 'NONE',  ( 174.1364721914477229, 71.85829564941442982, -19.71991761371826968 ) ) ;
#51406=CARTESIAN_POINT ( 'NONE',  ( 103.4725384926517222, 26.96797537091728003, 60.71934963752268999 ) ) ;
#51407=CARTESIAN_POINT ( 'NONE',  ( 157.4703587214989398, -170.0000000000000000, -36.12418429913763163 ) ) ;
#51409=CARTESIAN_POINT ( 'NONE',  ( 61.09977118998601497, 13.26754120022606465, -23.63138592492630252 ) ) ;
#51410=VERTEX_POINT ( 'NONE', #48896 ) ;
#51414=CARTESIAN_POINT ( 'NONE',  ( 19.10949903373832370, 7.636938177523842519, -49.74798475061973591 ) ) ;
#51415=CARTESIAN_POINT ( 'NONE',  ( 9.045716588192245666, 7.384596431530731309, 67.68043104435533053 ) ) ;
#51417=FACE_BOUND ( 'NONE', #3186, .T. ) ;
#51419=ORIENTED_EDGE ( 'NONE', *, *, #33436, .F. ) ;
#51422=CARTESIAN_POINT ( 'NONE',  ( 33.93974911725172205, 8.773765372885563352, -75.10966096496471778 ) ) ;
#51423=CARTESIAN_POINT ( 'NONE',  ( -173.9617926765112941, 89.58633395456783433, 18.94172030153162112 ) ) ;
#51424=CARTESIAN_POINT ( 'NONE',  ( 15.46104383007058658, 6.490338125820253268, 83.70377566018196092 ) ) ;
#51425=CARTESIAN_POINT ( 'NONE',  ( 22.84562496400137022, 7.837215652665284082, 93.82577997359511812 ) ) ;
#51429=CARTESIAN_POINT ( 'NONE',  ( 198.7123879174244507, 100.1053816708572413, -48.35335775156385552 ) ) ;
#51434=CARTESIAN_POINT ( 'NONE',  ( -86.06016868996614733, 25.27707703029501474, -68.17648637259551947 ) ) ;
#51437=VECTOR ( 'NONE', #49212, 1000.000000000000000 ) ;
#51439=CARTESIAN_POINT ( 'NONE',  ( 9.416656162223558724, 6.380306691996770141, -39.05494724020170594 ) ) ;
#51444=ADVANCED_FACE ( 'NONE', ( #21160 ), #5996, .T. ) ;
#51447=CARTESIAN_POINT ( 'NONE',  ( 181.0840389613909736, 80.03940679743416808, -78.06960825634331513 ) ) ;
#51450=CARTESIAN_POINT ( 'NONE',  ( 63.01563776193091826, -170.0000000000000000, 71.65751152968501003 ) ) ;
#51454=CARTESIAN_POINT ( 'NONE',  ( 44.35071890818839790, 9.104600422692259443, 16.22605661256570997 ) ) ;
#51455=CARTESIAN_POINT ( 'NONE',  ( 180.6713229637342693, 79.61878926895391828, 2.464043515047720678 ) ) ;
#51458=CARTESIAN_POINT ( 'NONE',  ( 134.6141278563448225, 41.88200982625879476, -89.71241211332302612 ) ) ;
#51460=CARTESIAN_POINT ( 'NONE',  ( 209.9330698459270366, 115.6170919607588985, 85.01721959398543049 ) ) ;
#51462=DIRECTION ( 'NONE',  ( -0.000000000000000000, 1.000000000000000000, -0.000000000000000000 ) ) ;
#51463=CARTESIAN_POINT ( 'NONE',  ( -77.71448999903256549, 21.96089801565737787, -62.00523686349998798 ) ) ;
#51464=CARTESIAN_POINT ( 'NONE',  ( -11.14880195267006613, 7.129907723790827490, 44.35696964094925221 ) ) ;
#51466=B_SPLINE_CURVE_WITH_KNOTS ( 'NONE', 3,
 ( #8431, #29882, #46049, #46741, #24615, #18978, #14730, #68214, #25655, #46390, #67869, #51344, #35853, #3159, #67519, #36196, #19666, #57307 ),
 .UNSPECIFIED., .F., .F.,
 ( 4, 2, 2, 2, 2, 2, 2, 2, 4 ),
 ( 0.000000000000000000, 0.001501532864490863093, 0.002252299296736294532, 0.003003065728981726187, 0.004504598593472635033, 0.006006131457963544314, 0.009009197186945320374, 0.01051073005143618455, 0.01201226291592704873 ),
 .UNSPECIFIED. ) ;
#51472=CARTESIAN_POINT ( 'NONE',  ( 186.6075385349484179, 85.85749512876284939, -75.66779282773408966 ) ) ;
#51473=CARTESIAN_POINT ( 'NONE',  ( -166.3231866619663606, 81.31146386205591625, 41.50210861837916809 ) ) ;
#51475=CARTESIAN_POINT ( 'NONE',  ( -96.00016893459648770, 29.70347032303887858, -38.40669615010640570 ) ) ;
#51476=CARTESIAN_POINT ( 'NONE',  ( -27.70185240367226953, 10.02491413133430775, 4.364727659495228451 ) ) ;
#51477=DIRECTION ( 'NONE',  ( 0.000000000000000000, 0.000000000000000000, 1.000000000000000000 ) ) ;
#51478=DIRECTION ( 'NONE',  ( 0.000000000000000000, 0.000000000000000000, 1.000000000000000000 ) ) ;
#51479=CARTESIAN_POINT ( 'NONE',  ( 127.2397149628677369, 37.56999625068102233, -39.95516007037436879 ) ) ;
#51480=ORIENTED_EDGE ( 'NONE', *, *, #3578, .F. ) ;
#51484=CARTESIAN_POINT ( 'NONE',  ( 188.2262945779355903, 87.63857788125626769, 88.20066469376320129 ) ) ;
#51486=CARTESIAN_POINT ( 'NONE',  ( -29.04258984626623530, 9.210213971636683539, -76.77276363795868974 ) ) ;
#51493=EDGE_LOOP ( 'NONE', ( #17600, #52570, #4956, #60934 ) ) ;
#51497=CARTESIAN_POINT ( 'NONE',  ( 207.8407634284391179, 112.5209879629463785, 16.68595737575994420 ) ) ;
#51500=CARTESIAN_POINT ( 'NONE',  ( -25.07735481787161191, 9.648965052008787069, 60.58124441867286691 ) ) ;
#51502=CARTESIAN_POINT ( 'NONE',  ( -47.80193682758677909, 12.85650137125658787, 62.68131162742057683 ) ) ;
#51504=CARTESIAN_POINT ( 'NONE',  ( -2.874437057892792691, 6.618922960888053986, 58.80530662568687461 ) ) ;
#51508=DIRECTION ( 'NONE',  ( -0.000000000000000000, 1.000000000000000000, -0.000000000000000000 ) ) ;
#51509=CARTESIAN_POINT ( 'NONE',  ( -54.56693200831794144, 14.55131601960338905, -35.21632399845986328 ) ) ;
#51511=FACE_OUTER_BOUND ( 'NONE', #55861, .T. ) ;
#51514=ORIENTED_EDGE ( 'NONE', *, *, #35205, .F. ) ;
#51515=ORIENTED_EDGE ( 'NONE', *, *, #56639, .F. ) ;
#51517=CARTESIAN_POINT ( 'NONE',  ( -180.6213815675305341, 95.88446356933846459, -69.36606367677470075 ) ) ;
#51521=CARTESIAN_POINT ( 'NONE',  ( -180.4643341113398094, 95.69224917234936356, 13.03253127180882309 ) ) ;
#51522=CARTESIAN_POINT ( 'NONE',  ( -1.728570918131775880, 6.570609986804680780, 6.396230257614674564 ) ) ;
#51523=CARTESIAN_POINT ( 'NONE',  ( 63.01563776193091826, 13.70579113808095073, -50.72069083216976537 ) ) ;
#51524=CARTESIAN_POINT ( 'NONE',  ( -83.53167274806554587, 25.32068190668983831, 43.64689675707840877 ) ) ;
#51525=DIRECTION ( 'NONE',  ( -0.8160245890732938934, -0.5780171883497599028, 0.000000000000000000 ) ) ;
#51526=CARTESIAN_POINT ( 'NONE',  ( 140.2332932573541200, 45.41010019581509027, 14.14583329522551125 ) ) ;
#51528=ORIENTED_EDGE ( 'NONE', *, *, #16588, .F. ) ;
#51530=ADVANCED_FACE ( 'NONE', ( #35178 ), #40115, .F. ) ;
#51532=CARTESIAN_POINT ( 'NONE',  ( 46.50207827473963107, 9.439498081273457686, -45.54875031526387374 ) ) ;
#51534=CARTESIAN_POINT ( 'NONE',  ( -119.1064753703575718, 42.18441154001784099, 94.99999999999866418 ) ) ;
#51536=CARTESIAN_POINT ( 'NONE',  ( 67.54641595172913071, 14.80690682047551121, 43.30947815275538915 ) ) ;
#51540=CARTESIAN_POINT ( 'NONE',  ( -142.9730935922299579, 58.82921737386682537, 68.75594806298462913 ) ) ;
#51544=CARTESIAN_POINT ( 'NONE',  ( 181.0840389613909736, 78.60582251573003987, -9.380507075415925655 ) ) ;
#51546=CARTESIAN_POINT ( 'NONE',  ( -118.3927673406137160, 41.74929850983306068, 65.20241849948250490 ) ) ;
#51547=CARTESIAN_POINT ( 'NONE',  ( -85.64924756730680144, 26.19583280090849442, -18.51914542751836734 ) ) ;
#51548=CARTESIAN_POINT ( 'NONE',  ( 16.21073205782802162, 7.521094197081421129, -89.20804527961311692 ) ) ;
#51549=CARTESIAN_POINT ( 'NONE',  ( -152.5046761101291963, 66.76407727525179325, -35.43405179214044409 ) ) ;
#51551=ORIENTED_EDGE ( 'NONE', *, *, #18110, .T. ) ;
#51552=EDGE_CURVE ( 'NONE', #25068, #42723, #57407, .T. ) ;
#51553=CARTESIAN_POINT ( 'NONE',  ( -104.1393288135077455, 34.86912007524089319, 18.45559023715674840 ) ) ;
#51559=DIRECTION ( 'NONE',  ( -0.000000000000000000, 0.000000000000000000, -1.000000000000000000 ) ) ;
#51560=CARTESIAN_POINT ( 'NONE',  ( -143.2582950235167800, 60.34055023774276094, 87.75006652546248631 ) ) ;
#51562=VERTEX_POINT ( 'NONE', #3513 ) ;
#51564=CARTESIAN_POINT ( 'NONE',  ( -151.6648563624119390, 67.36546864992756412, -22.66487162737027461 ) ) ;
#51566=CARTESIAN_POINT ( 'NONE',  ( 63.98971758354223027, 12.90030016320051232, -35.76819646162389432 ) ) ;
#51567=CARTESIAN_POINT ( 'NONE',  ( 106.1738623902246275, 27.04424563638256629, -90.79883557465640820 ) ) ;
#51569=CARTESIAN_POINT ( 'NONE',  ( -62.55320287144887459, 17.87319849854530318, 38.05489813362841289 ) ) ;
#51570=CARTESIAN_POINT ( 'NONE',  ( -102.2801239173131194, -170.0000000000000000, -23.17002667451225406 ) ) ;
#51571=EDGE_CURVE ( 'NONE', #48198, #275, #46770, .T. ) ;
#51573=CARTESIAN_POINT ( 'NONE',  ( 55.51637278631174865, 12.08345311280959677, 36.80331343779680253 ) ) ;
#51576=CARTESIAN_POINT ( 'NONE',  ( -0.8011128725815479523, 6.535315321814157308, -40.27799443517058364 ) ) ;
#51578=CARTESIAN_POINT ( 'NONE',  ( -121.1775535805057160, 43.46577565517550568, 17.12734891093444034 ) ) ;
#51580=CARTESIAN_POINT ( 'NONE',  ( 127.6144785300460711, 37.78099129859915450, -20.84396720244194512 ) ) ;
#51581=CARTESIAN_POINT ( 'NONE',  ( 15.78827728214693060, 7.507518794609574719, -8.674393508222097537 ) ) ;
#51582=CARTESIAN_POINT ( 'NONE',  ( 197.9847015768255574, 97.56951352050454318, 66.90867592435427014 ) ) ;
#51591=CARTESIAN_POINT ( 'NONE',  ( 8.485361335568063268, 6.376707943524878353, -95.00000000000133582 ) ) ;
#51593=EDGE_LOOP ( 'NONE', ( #59619, #63902, #60227, #36741 ) ) ;
#51594=CARTESIAN_POINT ( 'NONE',  ( -146.5268141329886760, 61.69196909035590437, -8.582240967115531305 ) ) ;
#51595=CARTESIAN_POINT ( 'NONE',  ( 198.7123879174243939, 100.1053816708572555, 5.335743429363529522 ) ) ;
#51596=ORIENTED_EDGE ( 'NONE', *, *, #65922, .F. ) ;
#51597=CARTESIAN_POINT ( 'NONE',  ( 149.9883001095526822, 53.30008207809360954, 91.24430364700101848 ) ) ;
#51598=ORIENTED_EDGE ( 'NONE', *, *, #18406, .T. ) ;
#51600=CARTESIAN_POINT ( 'NONE',  ( 126.8237978310704790, 37.33705012421152958, 39.62906459034504536 ) ) ;
#51606=CARTESIAN_POINT ( 'NONE',  ( -2.793168949963659387, 7.622505585224017999, -91.02962397824867935 ) ) ;
#51609=CARTESIAN_POINT ( 'NONE',  ( -165.6397095829521788, 80.60756690931941648, 10.86796417263294856 ) ) ;
#51612=CARTESIAN_POINT ( 'NONE',  ( 23.28785143291466397, 6.856621069835716398, -70.36468173549914695 ) ) ;
#51613=CARTESIAN_POINT ( 'NONE',  ( -126.3453033442920628, 47.99870040347951061, 57.46449846362077807 ) ) ;
#51615=CARTESIAN_POINT ( 'NONE',  ( -99.42452458507153779, 32.47480804767672424, 84.74605913991881323 ) ) ;
#51619=CARTESIAN_POINT ( 'NONE',  ( 208.9585401441655961, 114.1617785893844257, -64.48185821820443664 ) ) ;
#51620=EDGE_CURVE ( 'NONE', #45282, #29274, #15110, .T. ) ;
#51621=CARTESIAN_POINT ( 'NONE',  ( 141.1220430186942565, 47.19066702031172866, 38.89026279445103285 ) ) ;
#51625=CARTESIAN_POINT ( 'NONE',  ( 69.35866309798979046, 15.27376159675660539, -66.05564973924086303 ) ) ;
#51630=CARTESIAN_POINT ( 'NONE',  ( 9.001060725719206346, 7.384057747890103940, -93.40660889270941425 ) ) ;
#51631=CARTESIAN_POINT ( 'NONE',  ( -172.3057147739577033, 86.22480007276998037, -49.67904019660583259 ) ) ;
#51634=CARTESIAN_POINT ( 'NONE',  ( -50.64797127373722674, 13.54441475554784979, -90.31972401984275223 ) ) ;
#51637=CARTESIAN_POINT ( 'NONE',  ( -147.3614567344829140, 62.37986555269942812, 45.42098636282473478 ) ) ;
#51639=CARTESIAN_POINT ( 'NONE',  ( -169.1041038606267648, 82.76530082651281361, -75.40566809599023657 ) ) ;
#51641=CARTESIAN_POINT ( 'NONE',  ( -108.0902552660050446, 36.97681740369922920, 33.25039213534302007 ) ) ;
#51643=CARTESIAN_POINT ( 'NONE',  ( -37.07086358537073068, 10.58360809068249964, 15.84908622039232817 ) ) ;
#51650=CARTESIAN_POINT ( 'NONE',  ( 32.09567473596477782, 7.571373529017940029, 12.28090692073144119 ) ) ;
#51651=CARTESIAN_POINT ( 'NONE',  ( -15.07235766390728671, 8.482541916553477890, -44.86552813969799303 ) ) ;
#51652=CARTESIAN_POINT ( 'NONE',  ( -38.54712373114178092, 11.89174538567467465, -18.41568109954191002 ) ) ;
#51654=VERTEX_POINT ( 'NONE', #14068 ) ;
#51656=ORIENTED_EDGE ( 'NONE', *, *, #1578, .F. ) ;
#51657=CARTESIAN_POINT ( 'NONE',  ( -55.05276343752909440, 14.68156374112638751, 30.31732777293113301 ) ) ;
#51658=CARTESIAN_POINT ( 'NONE',  ( -58.33157376762796531, 16.63098604184964913, 71.41156564722952282 ) ) ;
#51659=CARTESIAN_POINT ( 'NONE',  ( -28.13852122803039890, 9.072484007196644384, 4.119663645332994228 ) ) ;
#51663=CARTESIAN_POINT ( 'NONE',  ( -60.12777185093246146, 16.10091404267868498, -90.86635757588598494 ) ) ;
#51664=CARTESIAN_POINT ( 'NONE',  ( -38.89042640463647871, 10.93374343663409221, 38.70441581485059146 ) ) ;
#51669=CARTESIAN_POINT ( 'NONE',  ( -156.9232798886536671, 72.10386843399172108, 63.90848877142625639 ) ) ;
#51670=CARTESIAN_POINT ( 'NONE',  ( -125.0023254877051784, 45.90912477771774292, 30.65933094750346299 ) ) ;
#51673=CARTESIAN_POINT ( 'NONE',  ( -180.5200658187031877, 97.35517482626556784, -70.32344830815547709 ) ) ;
#51675=CARTESIAN_POINT ( 'NONE',  ( 112.7784411285248751, 30.07270878825233851, 30.04885473467402335 ) ) ;
#51681=CARTESIAN_POINT ( 'NONE',  ( 184.0001683447903531, 83.06228184427187955, 29.88528625916754322 ) ) ;
#51682=CARTESIAN_POINT ( 'NONE',  ( 139.6326990672750696, 46.22017155708125102, 5.375290015202373262 ) ) ;
#51686=EDGE_CURVE ( 'NONE', #68538, #41004, #7081, .T. ) ;
#51687=CARTESIAN_POINT ( 'NONE',  ( 163.7403496014744633, 64.00600007368879574, -20.90330565569645316 ) ) ;
#51689=CARTESIAN_POINT ( 'NONE',  ( 69.36287815987333261, 15.27486453472190142, 60.15464916579820454 ) ) ;
#51691=CARTESIAN_POINT ( 'NONE',  ( 126.6810562747852345, 37.25730572548798136, 88.48790994800812371 ) ) ;
#51694=CARTESIAN_POINT ( 'NONE',  ( -147.3614567344829709, 62.37986555269942812, -61.95721599902998378 ) ) ;
#51697=CARTESIAN_POINT ( 'NONE',  ( 163.1495034066983862, 62.20479872133081045, -38.69930229318859460 ) ) ;
#51699=CARTESIAN_POINT ( 'NONE',  ( -96.45303203827904781, 31.03218867996499242, 15.92233808110716708 ) ) ;
#51703=DIRECTION ( 'NONE',  ( 1.000000000000000000, 0.000000000000000000, -0.000000000000000000 ) ) ;
#51704=CARTESIAN_POINT ( 'NONE',  ( -168.7187482717113483, 82.35796501763486788, 32.23136137619717090 ) ) ;
#51705=CARTESIAN_POINT ( 'NONE',  ( 157.4703587214989113, 57.65129005721575339, 56.25401806271706562 ) ) ;
#51707=CARTESIAN_POINT ( 'NONE',  ( 94.11595392909971736, 23.18887043179185525, 37.72638076850486044 ) ) ;
#51709=CARTESIAN_POINT ( 'NONE',  ( -101.3502439362134595, 33.43728945125135255, 57.40693085676335983 ) ) ;
#51710=CARTESIAN_POINT ( 'NONE',  ( -9.765753193741730342, 8.033970690975920093, 57.21132304879623121 ) ) ;
#51713=CARTESIAN_POINT ( 'NONE',  ( 157.0316110297313799, 58.58403635656377162, -9.279633708673957315 ) ) ;
#51715=CARTESIAN_POINT ( 'NONE',  ( 105.7953515382196485, 27.97683113100024244, 43.16950470399848427 ) ) ;
#51718=CARTESIAN_POINT ( 'NONE',  ( 188.0094179620990928, 87.39792407168452826, 7.070946854141474169 ) ) ;
#51719=CARTESIAN_POINT ( 'NONE',  ( 210.1633650091869185, 114.1507944623967035, -48.96769043267524069 ) ) ;
#51720=CARTESIAN_POINT ( 'NONE',  ( 177.2011275744679040, 74.76848439756736298, 3.543480587856852715 ) ) ;
#51721=CARTESIAN_POINT ( 'NONE',  ( -61.86403937395562025, 16.61416349803656090, 14.12202676930323086 ) ) ;
#51724=ORIENTED_EDGE ( 'NONE', *, *, #11405, .T. ) ;
#51726=CARTESIAN_POINT ( 'NONE',  ( 46.65974587859240330, 10.48396258569370332, -18.22915301820460598 ) ) ;
#51729=CARTESIAN_POINT ( 'NONE',  ( -12.11585256177172276, 7.208421262014329756, 85.14452039693073004 ) ) ;
#51731=CARTESIAN_POINT ( 'NONE',  ( -104.7956873821848802, 35.21322275870669216, -22.73943902020269903 ) ) ;
#51733=CARTESIAN_POINT ( 'NONE',  ( -76.31381168750411348, 21.43908608416556305, 71.90022727437172989 ) ) ;
#51734=LINE ( 'NONE', #14451, #16137 ) ;
#51738=CARTESIAN_POINT ( 'NONE',  ( -156.9406434201983984, 70.74968524571478667, 39.37071447540302671 ) ) ;
#51740=CARTESIAN_POINT ( 'NONE',  ( 178.1999009735082211, 75.73911533785329198, -9.953687985995264498 ) ) ;
#51741=CARTESIAN_POINT ( 'NONE',  ( -169.8885678771097787, 85.07765565657315676, 58.38415322356205905 ) ) ;
#51744=CARTESIAN_POINT ( 'NONE',  ( 57.39233401791016576, 12.46575990788835320, -11.38927566978218664 ) ) ;
#51745=ORIENTED_EDGE ( 'NONE', *, *, #60924, .F. ) ;
#51748=CARTESIAN_POINT ( 'NONE',  ( 211.5066273949820186, 116.1727691518062215, 6.669578147803371770 ) ) ;
#51749=LINE ( 'NONE', #57719, #30501 ) ;
#51750=CARTESIAN_POINT ( 'NONE',  ( 212.1962110267000696, 117.2292732107321740, 36.33105866627646918 ) ) ;
#51751=FACE_BOUND ( 'NONE', #41536, .T. ) ;
#51755=DIRECTION ( 'NONE',  ( -0.000000000000000000, 1.000000000000000000, -0.000000000000000000 ) ) ;
#51758=LINE ( 'NONE', #13775, #29847 ) ;
#51759=CARTESIAN_POINT ( 'NONE',  ( 20.10458824423762891, 6.677140564692391145, 85.06154812080229988 ) ) ;
#51764=CARTESIAN_POINT ( 'NONE',  ( -78.66644367742111399, -170.0000000000000000, 64.76275173013681297 ) ) ;
#51765=EDGE_CURVE ( 'NONE', #53693, #51871, #69102, .T. ) ;
#51766=CARTESIAN_POINT ( 'NONE',  ( 202.7540649946182896, 105.3989460363904698, -51.08106962100063697 ) ) ;
#51769=CARTESIAN_POINT ( 'NONE',  ( -84.22570405563701001, 24.51726571826275247, 16.13179647595237043 ) ) ;
#51770=VERTEX_POINT ( 'NONE', #25164 ) ;
#51771=CARTESIAN_POINT ( 'NONE',  ( -80.31691774066409550, 22.95709084517031684, -62.14002771806871550 ) ) ;
#51775=EDGE_CURVE ( 'NONE', #60761, #53864, #8287, .T. ) ;
#51776=ORIENTED_EDGE ( 'NONE', *, *, #32799, .F. ) ;
#51777=CARTESIAN_POINT ( 'NONE',  ( 11.21653854975268949, 6.397128675385706842, -37.05325069752230860 ) ) ;
#51779=CARTESIAN_POINT ( 'NONE',  ( 20.74093720376649230, 6.709541214524347374, 5.016829158437670522 ) ) ;
#51782=CARTESIAN_POINT ( 'NONE',  ( 173.9457771591584958, 73.05793967547531054, -72.88831180620124428 ) ) ;
#51785=CARTESIAN_POINT ( 'NONE',  ( 107.9362503323352769, 27.82881837607801856, -36.27000779090448646 ) ) ;
#51786=CARTESIAN_POINT ( 'NONE',  ( 83.38619203015947789, 19.39783821526630447, -50.10106600002546173 ) ) ;
#51787=CARTESIAN_POINT ( 'NONE',  ( -165.8925458123985948, 80.86730909018719160, -93.88204572899961420 ) ) ;
#51790=ORIENTED_EDGE ( 'NONE', *, *, #42590, .T. ) ;
#51796=CARTESIAN_POINT ( 'NONE',  ( 139.6324999503821118, 45.02288024089203589, -92.41009172426876717 ) ) ;
#51798=CARTESIAN_POINT ( 'NONE',  ( -122.8202784017355498, 45.69728649588466851, -62.41294849004252399 ) ) ;
#51800=CARTESIAN_POINT ( 'NONE',  ( 204.6977192012829505, 108.0580384837234931, -24.48138044215792419 ) ) ;
#51801=CARTESIAN_POINT ( 'NONE',  ( -78.66644367742109978, 23.39876645725289706, 57.26275173013680586 ) ) ;
#51804=CARTESIAN_POINT ( 'NONE',  ( 10.13563904803030979, 7.391572367417535538, -11.22086992224583923 ) ) ;
#51805=EDGE_LOOP ( 'NONE', ( #68754, #34655 ) ) ;
#51809=CARTESIAN_POINT ( 'NONE',  ( 186.2680729609085120, 85.48839327635664631, -76.01000320357321982 ) ) ;
#51810=CARTESIAN_POINT ( 'NONE',  ( -143.2587158300141539, 60.34092810886536995, 69.22125202308285452 ) ) ;
#51814=CARTESIAN_POINT ( 'NONE',  ( -104.1342612728951593, 33.73231160250196581, 3.892347345905328382 ) ) ;
#51815=CARTESIAN_POINT ( 'NONE',  ( 10.82760985890677752, 7.398654328676808944, -37.37257414635145381 ) ) ;
#51819=CARTESIAN_POINT ( 'NONE',  ( 186.5193936449931869, 85.76190592813432545, 85.31929775637671298 ) ) ;
#51821=FACE_OUTER_BOUND ( 'NONE', #3, .T. ) ;
#51822=CARTESIAN_POINT ( 'NONE',  ( 12.69192874957004769, 6.421326776602847453, 3.834725903590704643 ) ) ;
#51823=CARTESIAN_POINT ( 'NONE',  ( 42.48820792780864508, 9.847387255477764612, -76.80433085855322872 ) ) ;
#51824=CARTESIAN_POINT ( 'NONE',  ( 183.7875981612220073, 82.83906702837187197, -9.881439232383749882 ) ) ;
#51825=CARTESIAN_POINT ( 'NONE',  ( 204.6977192012829789, 108.0580384837234931, 17.36317014830577321 ) ) ;
#51827=CARTESIAN_POINT ( 'NONE',  ( -178.5790738944854184, 93.41591512785082330, -37.06229826213597534 ) ) ;
#51828=CARTESIAN_POINT ( 'NONE',  ( 93.09528872995976201, 21.72934119836187605, -12.64476263866717431 ) ) ;
#51829=CARTESIAN_POINT ( 'NONE',  ( -26.88635117726412815, 9.904687797303049379, 70.54110651337641968 ) ) ;
#51831=B_SPLINE_CURVE_WITH_KNOTS ( 'NONE', 3,
 ( #11473, #32261, #48069, #21345, #43829, #32940, #53694, #63916, #49100, #16419, #58285, #64260, #26635, #54382, #5514, #10106, #231, #69186, #10440, #21688, #6207, #43139, #31563, #37877, #37522, #4821, #26291, #21013, #59323, #31913, #53342, #69526, #11135, #32599, #5853, #27308, #48752, #22041, #43486, #50861, #1288, #60719, #39617, #65666, #2677 ),
 .UNSPECIFIED., .F., .F.,
 ( 4, 2, 2, 2, 2, 2, 2, 2, 1, 2, 2, 2, 2, 2, 2, 2, 2, 2, 2, 2, 2, 2, 4 ),
 ( 1.734723475976807094E-18, 0.001467747071934254058, 0.002201620607901382930, 0.002935494143868511586, 0.004403241215802774534, 0.005870988287737037049, 0.007338735359671300432, 0.008072608895638421281, 0.008806482431605545599, 0.009540355967572666449, 0.01027422950353978903, 0.01174197657547401165, 0.01247585011144112556, 0.01320972364740823773, 0.01467747071934244474, 0.01541134425530953436, 0.01614521779127663093, 0.01761296486321079630, 0.01908071193514496861, 0.01981458547111204088, 0.02054845900707912010, 0.02201620607901325771, 0.02348395315094739533 ),
 .UNSPECIFIED. ) ;
#51832=CARTESIAN_POINT ( 'NONE',  ( -54.56693200831792723, 14.55131601960339260, 72.16187836339486239 ) ) ;
#51833=CARTESIAN_POINT ( 'NONE',  ( -0.8011128725815451768, 6.535315321814157308, 67.10020792668412071 ) ) ;
#51836=CARTESIAN_POINT ( 'NONE',  ( 156.5993887774280040, 58.24868799840904643, 56.30154359095186578 ) ) ;
#51837=DIRECTION ( 'NONE',  ( -0.8118923937861950435, -0.5838071093367415143, 0.000000000000000000 ) ) ;
#51838=CARTESIAN_POINT ( 'NONE',  ( -51.78153763344963068, 13.82841714689605794, -49.48256276243913021 ) ) ;
#51840=CARTESIAN_POINT ( 'NONE',  ( -0.9745223251005035170, 7.548327269165426401, 94.42701984305149665 ) ) ;
#51847=AXIS2_PLACEMENT_3D ( 'NONE', #49959, #44331, #66175 ) ;
#51860=CARTESIAN_POINT ( 'NONE',  ( 149.9762816496916003, 52.05155590316277880, 90.11743903550856771 ) ) ;
#51861=CARTESIAN_POINT ( 'NONE',  ( 134.3172730033263349, 41.70277427218490374, 17.66579024853170665 ) ) ;
#51864=CARTESIAN_POINT ( 'NONE',  ( 9.057575839850576571, 6.378493414438676901, 67.67707940144546797 ) ) ;
#51871=VERTEX_POINT ( 'NONE', #19171 ) ;
#51872=ORIENTED_EDGE ( 'NONE', *, *, #3418, .T. ) ;
#51876=CARTESIAN_POINT ( 'NONE',  ( 186.2722199822850655, 84.01218714714251234, -11.44440540467959799 ) ) ;
#51877=CARTESIAN_POINT ( 'NONE',  ( -118.9649285217355583, 42.09781191014329949, 62.08225238709908922 ) ) ;
#51878=CARTESIAN_POINT ( 'NONE',  ( -79.14638003838379632, 23.58242782405879012, -8.270900041254195756 ) ) ;
#51879=CARTESIAN_POINT ( 'NONE',  ( 16.76400266940279593, 6.533513613209220416, -23.62695608403941705 ) ) ;
#51880=CARTESIAN_POINT ( 'NONE',  ( -50.53243683205840142, 14.55237037207940531, 43.82175149422371163 ) ) ;
#51883=CARTESIAN_POINT ( 'NONE',  ( -105.4642082819535887, 35.56541171990214423, 17.98124511787474589 ) ) ;
#51885=LINE ( 'NONE', #35371, #45071 ) ;
#51886=CARTESIAN_POINT ( 'NONE',  ( 102.7351271102982224, 25.56094931096820488, 90.72548476243952109 ) ) ;
#51888=VECTOR ( 'NONE', #29538, 1000.000000000000000 ) ;
#51891=CARTESIAN_POINT ( 'NONE',  ( -144.4759242270947937, 61.31787838020377279, 86.31655861621851500 ) ) ;
#51898=CARTESIAN_POINT ( 'NONE',  ( -86.06489347855101357, 25.27905598459106784, 63.50647088109550964 ) ) ;
#51900=CARTESIAN_POINT ( 'NONE',  ( 103.9024360978282999, 26.05738592538718379, -93.08474446646899025 ) ) ;
#51905=CARTESIAN_POINT ( 'NONE',  ( 187.5246323291926842, 86.86207184872515086, 67.53503301494710342 ) ) ;
#51906=CARTESIAN_POINT ( 'NONE',  ( 8.288104306525688969, 6.376394648992967262, -16.66097189769440945 ) ) ;
#51909=VERTEX_POINT ( 'NONE', #14256 ) ;
#51910=CARTESIAN_POINT ( 'NONE',  ( -1.088326810997878091, 6.545818265928951440, -46.25019226022950392 ) ) ;
#51912=CARTESIAN_POINT ( 'NONE',  ( -124.3331814159187161, 45.47486189329070072, 3.936062064721631337 ) ) ;
#51915=CARTESIAN_POINT ( 'NONE',  ( 23.23965501943000334, 7.861749956303023978, -17.15812566989634291 ) ) ;
#51916=CARTESIAN_POINT ( 'NONE',  ( 8.763528846667105299, 7.383598436776578566, 13.30899920650040080 ) ) ;
#51920=CARTESIAN_POINT ( 'NONE',  ( 126.8114659053431694, 38.48351437375816175, -46.14626030992690175 ) ) ;
#51922=CARTESIAN_POINT ( 'NONE',  ( -109.6657532478350845, 37.84376708859253569, -43.84539487966294757 ) ) ;
#51923=CARTESIAN_POINT ( 'NONE',  ( 188.2091813586561670, 87.61952156613881471, -41.36644826682314857 ) ) ;
#51927=CARTESIAN_POINT ( 'NONE',  ( -28.13852122803041311, 9.072484007196637279, -22.72488694513067031 ) ) ;
#51930=ORIENTED_EDGE ( 'NONE', *, *, #3318, .F. ) ;
#51931=CARTESIAN_POINT ( 'NONE',  ( 164.9053016786531316, 64.98846293739913449, 89.59488780726475454 ) ) ;
#51933=CARTESIAN_POINT ( 'NONE',  ( -59.58556642339446086, 16.99097764963621060, 16.96804118674567974 ) ) ;
#51935=CARTESIAN_POINT ( 'NONE',  ( -155.1359377029286009, 70.46175948311804405, 43.20321676328643434 ) ) ;
#51937=EDGE_CURVE ( 'NONE', #16320, #53253, #52564, .T. ) ;
#51950=CARTESIAN_POINT ( 'NONE',  ( -34.34470740021929913, 11.10817648171062366, -89.58872634471485696 ) ) ;
#51951=DIRECTION ( 'NONE',  ( 0.000000000000000000, 0.000000000000000000, 1.000000000000000000 ) ) ;
#51952=ORIENTED_EDGE ( 'NONE', *, *, #1578, .T. ) ;
#51953=CARTESIAN_POINT ( 'NONE',  ( 133.8566784816069344, -170.0000000000000000, -43.52331093239567394 ) ) ;
#51954=ADVANCED_FACE ( 'NONE', ( #41334 ), #58188, .F. ) ;
#51958=VERTEX_POINT ( 'NONE', #20907 ) ;
#51959=CARTESIAN_POINT ( 'NONE',  ( -56.02027488966933078, 14.94257193099085868, -8.418912259423796840 ) ) ;
#51960=CARTESIAN_POINT ( 'NONE',  ( -128.1282195935087884, 49.19720162550164844, -76.42132434122385121 ) ) ;
#51961=CARTESIAN_POINT ( 'NONE',  ( 117.4711568421289627, 33.49899443629671936, 39.17702909593091931 ) ) ;
#51962=CARTESIAN_POINT ( 'NONE',  ( -126.3495878770406193, 48.00153794568855403, 18.77539728269342234 ) ) ;
#51963=CARTESIAN_POINT ( 'NONE',  ( 70.26639875985989647, 15.51307715494296069, -68.08326665301770220 ) ) ;
#51967=CARTESIAN_POINT ( 'NONE',  ( -171.4814970982680222, 85.32124710276291069, -34.88158325180384622 ) ) ;
#51972=CARTESIAN_POINT ( 'NONE',  ( -144.9287131874381771, 60.39056348581543432, 44.18048465558430848 ) ) ;
#51974=CARTESIAN_POINT ( 'NONE',  ( 209.9944361927104808, 113.8994774711241007, 58.23723418828768672 ) ) ;
#51975=ORIENTED_EDGE ( 'NONE', *, *, #12159, .F. ) ;
#51976=CARTESIAN_POINT ( 'NONE',  ( -109.5157885508426574, 37.76058765671428574, 40.06018348045786581 ) ) ;
#51979=CARTESIAN_POINT ( 'NONE',  ( 86.62931800182292363, 20.48449268398425716, -89.51066537983906812 ) ) ;
#51980=CARTESIAN_POINT ( 'NONE',  ( 79.52639011421921111, 18.17129627604991171, 66.51676211103118419 ) ) ;
#51982=CARTESIAN_POINT ( 'NONE',  ( -83.23830101421552286, 24.11594324015501201, -90.35514600372840732 ) ) ;
#51986=CARTESIAN_POINT ( 'NONE',  ( 33.76124497394584267, 7.742545529019360551, 15.53639134207576511 ) ) ;
#51987=CARTESIAN_POINT ( 'NONE',  ( -10.92576759990585167, 8.121994053275063408, -36.08453108487010752 ) ) ;
#51989=CARTESIAN_POINT ( 'NONE',  ( -125.8938041572051389, -170.0000000000000000, -88.60280507916129977 ) ) ;
#51992=CARTESIAN_POINT ( 'NONE',  ( -121.9323109100150191, 45.13109664935808496, -89.73066178333888843 ) ) ;
#51994=CARTESIAN_POINT ( 'NONE',  ( -59.95707852844800101, 16.05120821151903954, 32.12152303550877264 ) ) ;
#51996=CARTESIAN_POINT ( 'NONE',  ( -190.4966031023458584, 108.8421921967458843, 15.75534704198573088 ) ) ;
#51998=CARTESIAN_POINT ( 'NONE',  ( -61.25157674566710853, 16.43158121994553511, -92.17786549963551579 ) ) ;
#51999=CARTESIAN_POINT ( 'NONE',  ( -95.61819996182573789, 29.52346081122277255, -12.21564220075769391 ) ) ;
#52004=VERTEX_POINT ( 'NONE', #52899 ) ;
#52007=CARTESIAN_POINT ( 'NONE',  ( -156.0209085498132140, 71.27066046086517304, 61.30830681328009035 ) ) ;
#52009=CARTESIAN_POINT ( 'NONE',  ( -121.5921196778232058, 43.72569502503144179, 31.95820139695877771 ) ) ;
#52010=CYLINDRICAL_SURFACE ( 'NONE', #52385, 7.500000000000020428 ) ;
#52011=VERTEX_POINT ( 'NONE', #31130 ) ;
#52012=CARTESIAN_POINT ( 'NONE',  ( -180.5234362879039622, 97.35934147644944403, -67.80900013366066048 ) ) ;
#52013=CARTESIAN_POINT ( 'NONE',  ( 127.0069430753658395, 38.59356149538464109, 93.77475522799868202 ) ) ;
#52014=EDGE_CURVE ( 'NONE', #44986, #29362, #18791, .T. ) ;
#52015=CARTESIAN_POINT ( 'NONE',  ( 113.8568724296587504, 30.58972477291342784, 30.52184481816738781 ) ) ;
#52016=EDGE_CURVE ( 'NONE', #52425, #21098, #3711, .T. ) ;
#52020=EDGE_CURVE ( 'NONE', #29274, #67595, #16291, .T. ) ;
#52023=CARTESIAN_POINT ( 'NONE',  ( 116.6457744947906860, 31.95847117670279403, -74.18078547863080985 ) ) ;
#52024=CARTESIAN_POINT ( 'NONE',  ( 186.6075385349484463, 85.85749512876287781, 31.71040953412066088 ) ) ;
#52025=CARTESIAN_POINT ( 'NONE',  ( 141.3586046882815310, 47.34625111366352712, 9.656894089140847015 ) ) ;
#52027=EDGE_LOOP ( 'NONE', ( #33669, #16968, #41083, #38105 ) ) ;
#52029=ORIENTED_EDGE ( 'NONE', *, *, #34901, .T. ) ;
#52030=CARTESIAN_POINT ( 'NONE',  ( 70.51522979775972999, 15.57935281015687146, 64.65971896463177870 ) ) ;
#52031=CARTESIAN_POINT ( 'NONE',  ( 132.6840581302284079, 40.72084251088482176, 83.28510945087752759 ) ) ;
#52032=VECTOR ( 'NONE', #6655, 1000.000000000000000 ) ;
#52033=AXIS2_PLACEMENT_3D ( 'NONE', #13821, #53160, #58790 ) ;
#52035=VERTEX_POINT ( 'NONE', #14508 ) ;
#52036=CARTESIAN_POINT ( 'NONE',  ( -180.3153482337535252, 95.51031295027644319, 40.46297689070883763 ) ) ;
#52040=CARTESIAN_POINT ( 'NONE',  ( 115.7731501832035832, 32.64791439093733061, -48.51258337113941366 ) ) ;
#52046=CARTESIAN_POINT ( 'NONE',  ( -132.4819073909166320, 50.98736898418872698, 41.74248034566528531 ) ) ;
#52048=CARTESIAN_POINT ( 'NONE',  ( 79.14113188808478583, 18.05280674635442040, -15.98610417696640695 ) ) ;
#52049=CARTESIAN_POINT ( 'NONE',  ( -175.8203575500379259, 91.72143465022357134, -88.89240186285151424 ) ) ;
#52052=CARTESIAN_POINT ( 'NONE',  ( 86.62931800182293784, 20.48449268398423229, 44.71208757247933363 ) ) ;
#52058=CARTESIAN_POINT ( 'NONE',  ( 152.1153500913667358, 54.85403770686897218, -11.52264547865338429 ) ) ;
#52059=CARTESIAN_POINT ( 'NONE',  ( 210.6584452238134872, 116.7138338345753965, -21.56006559325671645 ) ) ;
#52060=CARTESIAN_POINT ( 'NONE',  ( 106.0228389049370463, 28.07756796303168656, 30.90652886002973077 ) ) ;
#52061=CARTESIAN_POINT ( 'NONE',  ( -0.7076388175553600668, 7.538734751903869657, 35.20121844452963700 ) ) ;
#52062=CARTESIAN_POINT ( 'NONE',  ( -173.1211646369891355, -170.0000000000000000, 30.82169460664101734 ) ) ;
#52063=CARTESIAN_POINT ( 'NONE',  ( 186.6075385349484463, 85.85749512876287781, 4.865858943656973246 ) ) ;
#52064=CARTESIAN_POINT ( 'NONE',  ( 211.1200456646897123, 115.5868795682034005, -39.94236214982109345 ) ) ;
#52065=CARTESIAN_POINT ( 'NONE',  ( 176.6214367443247681, 74.20967084876664899, 16.01070763406217523 ) ) ;
#52066=EDGE_LOOP ( 'NONE', ( #57377, #16403 ) ) ;
#52069=CARTESIAN_POINT ( 'NONE',  ( -73.81801970646056077, 21.60231032711190835, 70.49010474810707194 ) ) ;
#52072=CARTESIAN_POINT ( 'NONE',  ( -8.487474335736092002, 6.934846266162439044, 83.82687023565640061 ) ) ;
#52073=CARTESIAN_POINT ( 'NONE',  ( -108.1180879163843116, 36.99199941971029659, -10.93529391401303386 ) ) ;
#52075=CARTESIAN_POINT ( 'NONE',  ( -74.19961951691010427, 20.67022044985852602, 58.73306680916620337 ) ) ;
#52076=CARTESIAN_POINT ( 'NONE',  ( 202.1083097594007256, 102.8573673850798542, -90.44468564295731028 ) ) ;
#52079=CARTESIAN_POINT ( 'NONE',  ( -156.3790798118593273, 70.23422112803315542, 35.20372313786793228 ) ) ;
#52081=CARTESIAN_POINT ( 'NONE',  ( 175.3815143714021190, 73.02838262206998365, -12.00236747850586916 ) ) ;
#52085=CARTESIAN_POINT ( 'NONE',  ( 133.8566784816069060, 42.60093787723652525, -9.178760341931967659 ) ) ;
#52089=CARTESIAN_POINT ( 'NONE',  ( 207.4696221732442041, 110.2206209205162253, 2.882253511827710835 ) ) ;
#52090=CARTESIAN_POINT ( 'NONE',  ( 9.050324533885198974, 7.384616180193985358, 61.02893197393973423 ) ) ;
#52092=FACE_BOUND ( 'NONE', #34102, .T. ) ;
#52096=EDGE_CURVE ( 'NONE', #29274, #29060, #15937, .T. ) ;
#52098=EDGE_CURVE ( 'NONE', #18617, #24506, #10426, .T. ) ;
#52099=ORIENTED_EDGE ( 'NONE', *, *, #34734, .F. ) ;
#52101=CARTESIAN_POINT ( 'NONE',  ( -118.5222689009585935, 43.00653498780619088, 90.38654037676664643 ) ) ;
#52103=CARTESIAN_POINT ( 'NONE',  ( -165.7138623879809529, 79.24467249981145756, -14.15247808995200174 ) ) ;
#52104=CARTESIAN_POINT ( 'NONE',  ( -179.8989115484066872, 96.59045402602909292, 14.70008741146901343 ) ) ;
#52105=CARTESIAN_POINT ( 'NONE',  ( 8.313220962251200774, 6.376421556596937990, 91.89783802061894846 ) ) ;
#52106=CARTESIAN_POINT ( 'NONE',  ( -7.825402957745083654, 6.891034867348166060, 3.271030448983516692 ) ) ;
#52109=CARTESIAN_POINT ( 'NONE',  ( -96.78198318406116130, 30.07417864442863120, 59.73932225907307014 ) ) ;
#52110=ORIENTED_EDGE ( 'NONE', *, *, #63682, .F. ) ;
#52111=CARTESIAN_POINT ( 'NONE',  ( -79.61931371420119774, 22.68640080971621842, 18.52793425929278825 ) ) ;
#52113=CARTESIAN_POINT ( 'NONE',  ( -61.53550548562875377, 17.56596194025585334, -12.06819366122919845 ) ) ;
#52117=CARTESIAN_POINT ( 'NONE',  ( 10.13846145460683346, 6.385368868491632988, -38.06222546885739888 ) ) ;
#52118=CARTESIAN_POINT ( 'NONE',  ( -107.3393890951915068, 36.56899896043363185, -90.64997796909688077 ) ) ;
#52119=CARTESIAN_POINT ( 'NONE',  ( 109.7732660198864210, 29.77277639096405792, 17.76666361527367144 ) ) ;
#52120=ORIENTED_EDGE ( 'NONE', *, *, #7147, .T. ) ;
#52122=CARTESIAN_POINT ( 'NONE',  ( -38.44802608776349473, 10.84733462796151215, 88.71676382914708370 ) ) ;
#52123=CARTESIAN_POINT ( 'NONE',  ( 175.5429257635130682, 74.57009623370768736, -65.48940413290104345 ) ) ;
#52126=CARTESIAN_POINT ( 'NONE',  ( 105.4375968828853587, 26.72149058755205786, -37.65901433614699556 ) ) ;
#52127=CARTESIAN_POINT ( 'NONE',  ( 86.62931800182293784, 20.48449268398422873, -50.82156419891174437 ) ) ;
#52128=LINE ( 'NONE', #45117, #68074 ) ;
#52134=CARTESIAN_POINT ( 'NONE',  ( -83.15209219203883606, 25.16621997697721014, -63.42963256430944341 ) ) ;
#52135=CARTESIAN_POINT ( 'NONE',  ( -6.972640973861005342, 6.835494286893509575, -89.10717191287116634 ) ) ;
#52138=CARTESIAN_POINT ( 'NONE',  ( 129.5193594945038740, 38.86618897895341718, 16.30267058858694895 ) ) ;
#52140=CARTESIAN_POINT ( 'NONE',  ( 34.01806748219127741, 7.770218348519284390, -91.58336029640328491 ) ) ;
#52141=CARTESIAN_POINT ( 'NONE',  ( -118.3918229753714826, 42.92682904595257298, -69.76788943947511257 ) ) ;
#52143=CARTESIAN_POINT ( 'NONE',  ( -189.8133172329396814, -170.0000000000000000, 94.99999999999866418 ) ) ;
#52145=CARTESIAN_POINT ( 'NONE',  ( -102.2801239173131194, 32.78103895658057354, 45.51907450641513009 ) ) ;
#52148=CARTESIAN_POINT ( 'NONE',  ( -59.23442743245837505, 16.88959283244545162, 85.27218783227613130 ) ) ;
#52152=DIRECTION ( 'NONE',  ( 0.000000000000000000, 0.000000000000000000, 1.000000000000000000 ) ) ;
#52154=FACE_OUTER_BOUND ( 'NONE', #49674, .T. ) ;
#52156=CARTESIAN_POINT ( 'NONE',  ( 138.1901928158493149, 45.29454828899442731, -37.38403742761511950 ) ) ;
#52157=CARTESIAN_POINT ( 'NONE',  ( 34.84173759613680943, 7.859847277726513148, -37.14537742033876100 ) ) ;
#52158=CARTESIAN_POINT ( 'NONE',  ( 198.7765072002625288, 98.56267746775340299, 94.99999999999866418 ) ) ;
#52159=CARTESIAN_POINT ( 'NONE',  ( 8.336237313193160858, 7.382629160459401874, -42.04131975006048094 ) ) ;
#52160=CARTESIAN_POINT ( 'NONE',  ( 127.4953815656694758, 37.71366486045444333, -39.51891617239016341 ) ) ;
#52165=CARTESIAN_POINT ( 'NONE',  ( 173.5849338432005879, 72.72001811100811608, 90.26313734863605021 ) ) ;
#52168=DIRECTION ( 'NONE',  ( -0.000000000000000000, 0.000000000000000000, -1.000000000000000000 ) ) ;
#52169=UNCERTAINTY_MEASURE_WITH_UNIT (LENGTH_MEASURE( 1.000000000000000082E-05 ), #7025, 'distance_accuracy_value', 'NONE');
#52170=CARTESIAN_POINT ( 'NONE',  ( 15.29293866748103881, 6.484959508098435244, 18.17015708224156967 ) ) ;
#52173=CARTESIAN_POINT ( 'NONE',  ( 174.2469308602415197, 71.96142024047684060, -73.66458895490379177 ) ) ;
#52175=CARTESIAN_POINT ( 'NONE',  ( 88.28780346671264567, 19.99350429399659035, -23.79527902889355673 ) ) ;
#52176=CARTESIAN_POINT ( 'NONE',  ( -24.61094659556677655, 9.585225265507402170, 67.67335607608715975 ) ) ;
#52178=CARTESIAN_POINT ( 'NONE',  ( -48.99162761293258228, 13.13973062091724131, 60.23760786283060753 ) ) ;
#52179=VECTOR ( 'NONE', #25921, 1000.000000000000000 ) ;
#52180=EDGE_CURVE ( 'NONE', #52822, #21908, #66652, .T. ) ;
#52182=EDGE_CURVE ( 'NONE', #45785, #5837, #6194, .T. ) ;
#52184=DIRECTION ( 'NONE',  ( 0.000000000000000000, 0.000000000000000000, 1.000000000000000000 ) ) ;
#52185=CARTESIAN_POINT ( 'NONE',  ( -107.0809603157386505, 36.42942792191063006, -63.57645921949710299 ) ) ;
#52186=CARTESIAN_POINT ( 'NONE',  ( -47.61380558691494258, 12.81230778489787880, -41.72929327147289058 ) ) ;
#52193=CARTESIAN_POINT ( 'NONE',  ( -57.65733424639441296, 15.39521790791522804, 71.69929679271069745 ) ) ;
#52196=B_SPLINE_CURVE_WITH_KNOTS ( 'NONE', 3,
 ( #10941, #38370, #1092, #54181, #32412, #6002, #22544, #59471, #28522, #65465, #48550, #1802, #65113, #385, #53837, #16910, #17257, #43636, #59815, #27461, #5656, #33800, #27116, #11630, #33468, #60173, #21840, #22894, #1441, #43286, #54540, #6367, #27821, #44337, #49258, #11281, #65824, #38728, #48906, #43985, #39089, #42940, #11994, #54890, #6713 ),
 .UNSPECIFIED., .F., .F.,
 ( 4, 2, 2, 1, 2, 2, 2, 2, 2, 2, 2, 2, 2, 2, 2, 2, 2, 2, 2, 2, 2, 2, 4 ),
 ( 0.02348395315094737798, 0.02495010856601295041, 0.02568318627354573488, 0.02641626398107851936, 0.02714934168861130731, 0.02788241939614409179, 0.02934857481120968503, 0.03008165251874248339, 0.03081473022627528174, 0.03228088564134087846, 0.03301396334887367334, 0.03374704105640646823, 0.03521319647147206494, 0.03667935188653766165, 0.03741242959407043572, 0.03814550730160321673, 0.03961166271666881344, 0.04107781813173440322, 0.04254397354679999299, 0.04327705125433278094, 0.04401012896186556889, 0.04547628437693113784, 0.04694243979199670680 ),
 .UNSPECIFIED. ) ;
#52199=FACE_OUTER_BOUND ( 'NONE', #53640, .T. ) ;
#52200=CARTESIAN_POINT ( 'NONE',  ( -102.2801239173131052, 32.78103895658057354, 57.36362509687880618 ) ) ;
#52201=VERTEX_POINT ( 'NONE', #19356 ) ;
#52204=CARTESIAN_POINT ( 'NONE',  ( 56.52885800925552928, 12.28784885070978561, -47.01758796310792832 ) ) ;
#52205=CARTESIAN_POINT ( 'NONE',  ( -86.16710354151693707, 26.41338104675946497, 38.15269484146957524 ) ) ;
#52206=CARTESIAN_POINT ( 'NONE',  ( -24.71645982722742119, 9.599558729461499240, -12.63840101433433993 ) ) ;
#52207=CARTESIAN_POINT ( 'NONE',  ( 89.87518614971251907, 20.55373388674513180, 30.43397069802014698 ) ) ;
#52210=CARTESIAN_POINT ( 'NONE',  ( 13.37820144534468092, 6.435512790162279728, 71.46574325679264916 ) ) ;
#52211=LINE ( 'NONE', #36039, #34074 ) ;
#52212=CARTESIAN_POINT ( 'NONE',  ( 197.3119541548906568, 98.33923235143194574, 35.39365102528960705 ) ) ;
#52213=CARTESIAN_POINT ( 'NONE',  ( -71.16355647947769114, 20.66831286809284762, 91.86052901098470613 ) ) ;
#52214=DIRECTION ( 'NONE',  ( 0.000000000000000000, -1.000000000000000000, 0.000000000000000000 ) ) ;
#52216=CARTESIAN_POINT ( 'NONE',  ( 66.30636076182547356, 14.49616748423541779, 44.07007479522269477 ) ) ;
#52218=ORIENTED_EDGE ( 'NONE', *, *, #15902, .F. ) ;
#52219=CARTESIAN_POINT ( 'NONE',  ( 110.2429982417149574, 29.99119854320845846, -77.76698815611739235 ) ) ;
#52221=CARTESIAN_POINT ( 'NONE',  ( 200.8410151090926377, 101.2014854111317561, -64.22370884727946816 ) ) ;
#52225=CARTESIAN_POINT ( 'NONE',  ( 15.78827728214693416, 6.500811158483284835, -23.67439350822212774 ) ) ;
#52227=CARTESIAN_POINT ( 'NONE',  ( -49.44484229820456278, 14.28460989390479519, 42.82150934049000313 ) ) ;
#52228=ORIENTED_EDGE ( 'NONE', *, *, #46685, .T. ) ;
#52229=ORIENTED_EDGE ( 'NONE', *, *, #42110, .T. ) ;
#52230=CARTESIAN_POINT ( 'NONE',  ( -109.6657532478350987, 37.84376708859254990, 9.843706301264420588 ) ) ;
#52233=CARTESIAN_POINT ( 'NONE',  ( 103.5744911984874221, 25.91722113382955683, 87.35084054165872658 ) ) ;
#52235=AXIS2_PLACEMENT_3D ( 'NONE', #68333, #3961, #45478 ) ;
#52237=CARTESIAN_POINT ( 'NONE',  ( 186.6118452967671999, 84.37814701615437230, -38.63095407981293761 ) ) ;
#52244=ORIENTED_EDGE ( 'NONE', *, *, #39014, .F. ) ;
#52245=CARTESIAN_POINT ( 'NONE',  ( -149.9471644042847345, 65.87751327280743396, -22.95857820982234543 ) ) ;
#52248=CARTESIAN_POINT ( 'NONE',  ( 64.93495251696903381, 13.12601614965099373, -50.47501578450074078 ) ) ;
#52249=CARTESIAN_POINT ( 'NONE',  ( 103.6901687706621118, 25.96661075370345984, -93.43913290534256078 ) ) ;
#52251=CARTESIAN_POINT ( 'NONE',  ( -35.99414836699285303, 11.40630460607620833, -75.64038296020707719 ) ) ;
#52252=CARTESIAN_POINT ( 'NONE',  ( -156.3790798118593273, 70.23422112803315542, -18.48537804305940924 ) ) ;
#52254=CARTESIAN_POINT ( 'NONE',  ( 8.288451200428832877, 6.376395059685424194, -15.68249724139179158 ) ) ;
#52256=CARTESIAN_POINT ( 'NONE',  ( 22.28700331106867694, 7.803633676228380445, 14.42207042821974561 ) ) ;
#52257=CARTESIAN_POINT ( 'NONE',  ( 188.5662303205147055, 86.51341602961785782, 64.25165609669510047 ) ) ;
#52258=CARTESIAN_POINT ( 'NONE',  ( -118.8504142000305706, 42.02789424825282083, 13.86596505667573709 ) ) ;
#52259=CARTESIAN_POINT ( 'NONE',  ( 63.50528314073024205, 12.78634332146812547, -62.56524142263340593 ) ) ;
#52261=CARTESIAN_POINT ( 'NONE',  ( 15.78827728214693416, 7.507518794609588042, -23.67439350822212774 ) ) ;
#52262=CARTESIAN_POINT ( 'NONE',  ( 199.3671895066314903, 99.30947926630331324, 58.25206002476129896 ) ) ;
#52264=EDGE_LOOP ( 'NONE', ( #24963, #49223, #65007, #31853 ) ) ;
#52274=CARTESIAN_POINT ( 'NONE',  ( -30.95355748062275936, 9.511738996772313826, -23.47264677473818395 ) ) ;
#52276=VERTEX_POINT ( 'NONE', #49977 ) ;
#52278=CARTESIAN_POINT ( 'NONE',  ( 151.1900544856616762, 54.17358268150817224, 94.71353523477451120 ) ) ;
#52281=CARTESIAN_POINT ( 'NONE',  ( 127.2397149628677369, 37.56999625068102233, 40.57849170101663816 ) ) ;
#52284=CARTESIAN_POINT ( 'NONE',  ( -94.78109144324893975, 29.13179392050637162, 37.73384696942510885 ) ) ;
#52294=CARTESIAN_POINT ( 'NONE',  ( -123.6699087229882110, 45.04696784753415528, -22.73548513474139909 ) ) ;
#52296=CARTESIAN_POINT ( 'NONE',  ( -173.9548930713590948, 88.06040582145364226, -22.83265499627751893 ) ) ;
#52298=CARTESIAN_POINT ( 'NONE',  ( -131.6253556217204732, 51.61436399519948282, 60.10113730160578172 ) ) ;
#52300=CARTESIAN_POINT ( 'NONE',  ( -109.7479544825926183, 37.88941408414071077, 92.47845238461742667 ) ) ;
#52303=EDGE_CURVE ( 'NONE', #16320, #32410, #56534, .T. ) ;
#52304=CARTESIAN_POINT ( 'NONE',  ( -58.10608953386397957, 15.52134062643864532, -22.72640478715415568 ) ) ;
#52305=CARTESIAN_POINT ( 'NONE',  ( -132.6092625803567842, 52.31125232006265691, -65.90852614572540347 ) ) ;
#52307=CARTESIAN_POINT ( 'NONE',  ( -128.9863978264385196, 49.78205252558956317, 18.11205277819082227 ) ) ;
#52308=CARTESIAN_POINT ( 'NONE',  ( 66.94365390260637128, 14.65531706601758977, -76.45896609455289195 ) ) ;
#52311=CARTESIAN_POINT ( 'NONE',  ( -142.3187766126154656, 59.59460822661994683, -17.67785402409575468 ) ) ;
#52312=CARTESIAN_POINT ( 'NONE',  ( -166.3175803736862122, 79.86140754556167565, -39.04379056814254767 ) ) ;
#52313=DIRECTION ( 'NONE',  ( 0.000000000000000000, 0.000000000000000000, 1.000000000000000000 ) ) ;
#52315=CARTESIAN_POINT ( 'NONE',  ( -71.42546113164833343, 20.75891408601218302, 39.93699313454726507 ) ) ;
#52316=CYLINDRICAL_SURFACE ( 'NONE', #58453, 7.500000000000013323 ) ;
#52319=DIRECTION ( 'NONE',  ( -0.000000000000000000, 1.000000000000000000, -0.000000000000000000 ) ) ;
#52320=CARTESIAN_POINT ( 'NONE',  ( -166.3188283541502415, 79.86268666707381669, -72.22739220925680570 ) ) ;
#52321=EDGE_LOOP ( 'NONE', ( #9676, #22652, #44609, #57990 ) ) ;
#52322=CARTESIAN_POINT ( 'NONE',  ( -106.6940984894958007, 35.07986071359380986, -21.75232707253212538 ) ) ;
#52324=EDGE_LOOP ( 'NONE', ( #4359, #24857 ) ) ;
#52326=CARTESIAN_POINT ( 'NONE',  ( -38.26497993382596263, 10.81185389040528300, 13.98917590912293996 ) ) ;
#52327=CARTESIAN_POINT ( 'NONE',  ( 81.74250361646211616, 18.86685472882137660, 69.76712954530790967 ) ) ;
#52328=CARTESIAN_POINT ( 'NONE',  ( -84.62094424603726850, 24.67969995822045348, -91.73912349652042053 ) ) ;
#52330=CARTESIAN_POINT ( 'NONE',  ( 33.31166872005965729, 8.707041209322239794, 6.185351823203305344 ) ) ;
#52336=CARTESIAN_POINT ( 'NONE',  ( -38.87871322265799279, 11.95691939779334234, -14.99132105584396513 ) ) ;
#52343=CARTESIAN_POINT ( 'NONE',  ( 8.679939806240511757, 7.383357464882124077, -67.45892186114495814 ) ) ;
#52344=CARTESIAN_POINT ( 'NONE',  ( -189.2826425734428994, 107.1493800926106132, 12.45157081075467609 ) ) ;
#52346=AXIS2_PLACEMENT_3D ( 'NONE', #19005, #24644, #35182 ) ;
#52349=CARTESIAN_POINT ( 'NONE',  ( 150.5538013146980347, 53.70974888488128585, -40.71184894097334706 ) ) ;
#52354=CARTESIAN_POINT ( 'NONE',  ( -156.8728827992623849, 72.05711009495561825, 63.62291505455890217 ) ) ;
#52355=CARTESIAN_POINT ( 'NONE',  ( 181.0840389613909451, 80.03940679743416808, -9.380507075415923879 ) ) ;
#52359=CARTESIAN_POINT ( 'NONE',  ( -125.8938041572051389, 47.69968343338778283, -49.91370389823397602 ) ) ;
#52360=VERTEX_POINT ( 'NONE', #5585 ) ;
#52361=CARTESIAN_POINT ( 'NONE',  ( -176.3856149167965555, 92.38076834121982017, -62.29001654799212417 ) ) ;
#52362=CARTESIAN_POINT ( 'NONE',  ( 93.71772995179816235, 21.96265635001558536, 66.51989931170464843 ) ) ;
#52363=CARTESIAN_POINT ( 'NONE',  ( 203.9228889538744625, 106.9879579748728418, -24.45170175305141314 ) ) ;
#52364=CARTESIAN_POINT ( 'NONE',  ( 110.2429982417149290, 28.88204397445231209, -24.07788697519002596 ) ) ;
#52365=CARTESIAN_POINT ( 'NONE',  ( -119.5267374018686724, 42.44190186039716650, -65.26197758995584763 ) ) ;
#52367=CARTESIAN_POINT ( 'NONE',  ( 200.8298320869470501, 101.1869877914233484, 30.26769475748699989 ) ) ;
#52368=CARTESIAN_POINT ( 'NONE',  ( 112.7784411285248751, 30.07270878825233851, -77.32934762718066679 ) ) ;
#52369=CARTESIAN_POINT ( 'NONE',  ( 186.2575601542430661, 85.47765906955505955, 42.24398978463538157 ) ) ;
#52370=CARTESIAN_POINT ( 'NONE',  ( 157.4703587214989398, 58.92748579479258808, 17.56491688178971700 ) ) ;
#52376=CARTESIAN_POINT ( 'NONE',  ( -107.7743374187916885, 35.66028478413599601, -37.38574911014553948 ) ) ;
#52381=ORIENTED_EDGE ( 'NONE', *, *, #47480, .F. ) ;
#52382=CARTESIAN_POINT ( 'NONE',  ( -180.5231752320737257, 95.76423526868921954, 39.56937748859167669 ) ) ;
#52384=CARTESIAN_POINT ( 'NONE',  ( 116.9197133427646804, 33.22079464767577406, -46.87639412244661941 ) ) ;
#52385=AXIS2_PLACEMENT_3D ( 'NONE', #30910, #10131, #52687 ) ;
#52388=CARTESIAN_POINT ( 'NONE',  ( 126.8114659053431694, 38.48351437375816886, 61.23194205192785944 ) ) ;
#52395=CARTESIAN_POINT ( 'NONE',  ( -173.1211646369891355, 87.12891641440857882, 30.82169460664101734 ) ) ;
#52396=CARTESIAN_POINT ( 'NONE',  ( -33.36721086971961370, 9.915747831546608992, -62.40970415560823170 ) ) ;
#52397=CARTESIAN_POINT ( 'NONE',  ( 90.30732934992394689, 21.77797012484621320, 43.76604365556254095 ) ) ;
#52401=CARTESIAN_POINT ( 'NONE',  ( 152.8672128926848188, 55.41186463791522954, -22.70565529590070497 ) ) ;
#52402=CARTESIAN_POINT ( 'NONE',  ( -62.13370439300283721, 16.69510293645669563, 89.01348188984179899 ) ) ;
#52403=CARTESIAN_POINT ( 'NONE',  ( 105.4376736768159475, 27.81988511842610023, 31.34766073213387472 ) ) ;
#52404=B_SPLINE_CURVE_WITH_KNOTS ( 'NONE', 3,
 ( #16559, #46942, #3679, #25157, #59112, #38015, #68067, #52216, #59460, #51536, #68403, #20207, #62433, #5647, #19870, #3342, #14584, #36044, #42931, #57500, #41663, #37665, #30771, #57843, #4034, #53487, #27, #21482, #10929, #32402, #27106, #48541, #376, #43278, #6703, #44693, #23590, #33791, #45028, #60517, #55230, #65100, #60859, #49956 ),
 .UNSPECIFIED., .F., .F.,
 ( 4, 2, 2, 2, 2, 2, 2, 2, 2, 2, 2, 2, 2, 2, 2, 2, 2, 2, 2, 2, 2, 4 ),
 ( 0.000000000000000000, 0.001487235713946824349, 0.002230853570920217441, 0.002974471427893610534, 0.004461707141840360290, 0.005948942855787110046, 0.007436178569733859801, 0.008179796426707235113, 0.008923414283680609557, 0.01041064999762737579, 0.01189788571157414203, 0.01264150356854752515, 0.01338512142552090653, 0.01487235713946766583, 0.01561597499644105068, 0.01635959285341443553, 0.01784682856736120871, 0.01933406428130798535, 0.02007768213828137194, 0.02082129999525475159, 0.02230853570920152129, 0.02379577142314828753 ),
 .UNSPECIFIED. ) ;
#52405=CARTESIAN_POINT ( 'NONE',  ( -1.862553927312063040, 7.582910205528084369, 33.04026090934276993 ) ) ;
#52406=LINE ( 'NONE', #52062, #12376 ) ;
#52407=CARTESIAN_POINT ( 'NONE',  ( 184.5867277229703802, 83.68414666546580349, 16.59965183973755387 ) ) ;
#52409=CARTESIAN_POINT ( 'NONE',  ( 212.1700216741373310, 117.1889356120870929, -44.55361903701415116 ) ) ;
#52410=CARTESIAN_POINT ( 'NONE',  ( 181.0840389613909736, 78.60582251573003987, 2.464043515047718458 ) ) ;
#52414=VERTEX_POINT ( 'NONE', #11206 ) ;
#52415=CARTESIAN_POINT ( 'NONE',  ( -72.35078170365748917, 21.08176362823952843, 60.71011165796286235 ) ) ;
#52417=CARTESIAN_POINT ( 'NONE',  ( 55.90536342106781120, 11.13510150712953184, -72.50233492501236299 ) ) ;
#52420=CARTESIAN_POINT ( 'NONE',  ( 19.54452863209719382, 7.657034792877146501, 44.02475270524415407 ) ) ;
#52425=VERTEX_POINT ( 'NONE', #43207 ) ;
#52427=CARTESIAN_POINT ( 'NONE',  ( -151.2410113808308552, 65.66338888995507261, 30.91080334718760980 ) ) ;
#52428=CARTESIAN_POINT ( 'NONE',  ( 62.04664474957770182, 12.44961624115901877, -35.76790967155817924 ) ) ;
#52437=CARTESIAN_POINT ( 'NONE',  ( -126.3453033442920344, 47.99870040347946087, 30.61994787315706645 ) ) ;
#52438=VERTEX_POINT ( 'NONE', #37596 ) ;
#52439=CARTESIAN_POINT ( 'NONE',  ( 210.5178985598939505, 114.6803933586780317, 14.59982085240562988 ) ) ;
#52440=CARTESIAN_POINT ( 'NONE',  ( 9.819093282782489496, 7.389085782749408970, 68.92638477701862598 ) ) ;
#52441=CARTESIAN_POINT ( 'NONE',  ( 210.6741002223296846, 114.9147155784838077, 41.24653036116778537 ) ) ;
#52448=CARTESIAN_POINT ( 'NONE',  ( -122.1036342099435501, 45.23906970976855746, 85.31054657959678877 ) ) ;
#52449=CARTESIAN_POINT ( 'NONE',  ( -168.7187482717113767, 82.35796501763486788, -21.45773980473016351 ) ) ;
#52451=CARTESIAN_POINT ( 'NONE',  ( 63.01563776193091826, 12.67277567978498176, 29.81296093922127710 ) ) ;
#52455=CARTESIAN_POINT ( 'NONE',  ( -101.3602137809054540, 32.31558061113913283, 57.40576275019232355 ) ) ;
#52457=CARTESIAN_POINT ( 'NONE',  ( -84.97622048504842951, 24.82614411847757907, 7.011873618776862216 ) ) ;
#52462=CARTESIAN_POINT ( 'NONE',  ( -120.6739978760426197, 44.33795494230366785, 16.66634037272415014 ) ) ;
#52463=CARTESIAN_POINT ( 'NONE',  ( -178.5790738944854468, 93.41591512785086593, 70.31590409971879296 ) ) ;
#52464=CARTESIAN_POINT ( 'NONE',  ( 126.6395826915640299, 37.23416510613626684, 61.79751572699002793 ) ) ;
#52467=CARTESIAN_POINT ( 'NONE',  ( -38.55722845454012315, 10.86859975449739402, 89.02085468374171739 ) ) ;
#52470=CARTESIAN_POINT ( 'NONE',  ( 174.6242782760050147, 73.69713439533578025, -66.74970077171313676 ) ) ;
#52471=LINE ( 'NONE', #67625, #24676 ) ;
#52473=CARTESIAN_POINT ( 'NONE',  ( 79.18180043629686793, 18.06526831600445959, -44.34015328538779954 ) ) ;
#52477=CARTESIAN_POINT ( 'NONE',  ( 39.89571693415785347, 8.473773298340393723, 18.06928371549960133 ) ) ;
#52478=CARTESIAN_POINT ( 'NONE',  ( 177.0027897064244655, 75.97676392242546228, 16.27253295564755931 ) ) ;
#52479=B_SPLINE_CURVE_WITH_KNOTS ( 'NONE', 3,
 ( #49322, #60241, #28221, #44408, #101, #48613, #1153, #33864, #44049, #21557, #453, #43002, #16288, #37740, #59183, #21907, #808, #8525, #39481, #45451, #8170, #50393, #24004, #7490, #13789, #18725, #18033, #55306, #61290, #60937, #44767, #13112, #40183, #34577, #45099, #28942, #34912, #56018, #23659, #61967, #7126, #56350, #12757, #45804, #24360 ),
 .UNSPECIFIED., .F., .F.,
 ( 4, 2, 2, 2, 2, 2, 2, 2, 2, 2, 2, 1, 2, 2, 2, 2, 2, 2, 2, 2, 2, 2, 4 ),
 ( 0.000000000000000000, 0.001510509505235982548, 0.002265764257853956475, 0.003021019010471930402, 0.004531528515707878256, 0.005286783268325870831, 0.006042038020943863406, 0.007552547526179844220, 0.009063057031415825901, 0.01057356653665180758, 0.01132882128926979842, 0.01208407604188778753, 0.01283933079450577837, 0.01359458554712377094, 0.01510509505235972140, 0.01586034980497767755, 0.01661560455759563543, 0.01812611406283149221, 0.01963662356806735246, 0.02039187832068526524, 0.02114713307330317801, 0.02265764257853904520, 0.02416815208377490545 ),
 .UNSPECIFIED. ) ;
#52483=CARTESIAN_POINT ( 'NONE',  ( 129.1137093889808511, 38.63348691920623423, 4.350904459445209760 ) ) ;
#52484=CARTESIAN_POINT ( 'NONE',  ( 32.22469126021599095, 7.584221829288119388, -94.59231775885801596 ) ) ;
#52486=CARTESIAN_POINT ( 'NONE',  ( -120.1650841064594033, 44.02024060322520427, -64.41117799840883151 ) ) ;
#52487=CARTESIAN_POINT ( 'NONE',  ( 211.7318474105134385, 118.3631723164074145, 34.08830694803145178 ) ) ;
#52488=CARTESIAN_POINT ( 'NONE',  ( -102.2801239173131052, 33.91021738430207222, 18.67452391595144334 ) ) ;
#52489=CARTESIAN_POINT ( 'NONE',  ( -107.7743374187916885, 35.66028478413599601, 43.14790266124550300 ) ) ;
#52492=CARTESIAN_POINT ( 'NONE',  ( -47.70992047900629274, 13.86859651505968039, 89.94426166759667751 ) ) ;
#52493=VERTEX_POINT ( 'NONE', #59047 ) ;
#52494=EDGE_CURVE ( 'NONE', #31358, #54401, #1983, .T. ) ;
#52498=CARTESIAN_POINT ( 'NONE',  ( 19.11382977197791533, 7.636807742668409560, -63.12314672599089960 ) ) ;
#52500=CARTESIAN_POINT ( 'NONE',  ( -146.7404675333698663, 63.17262273741978618, 72.03985599882574320 ) ) ;
#52502=CARTESIAN_POINT ( 'NONE',  ( 134.0849965622593913, 42.73957449886184889, -51.02331093239570947 ) ) ;
#52503=CARTESIAN_POINT ( 'NONE',  ( -30.95341298663140961, 10.53108683215056196, 3.371903815725489473 ) ) ;
#52508=ORIENTED_EDGE ( 'NONE', *, *, #10795, .F. ) ;
#52509=CARTESIAN_POINT ( 'NONE',  ( 184.8109923074100607, 83.92257297578457553, 83.98258588058325813 ) ) ;
#52510=CARTESIAN_POINT ( 'NONE',  ( 129.2375969008351717, 39.86537432630840527, -91.29033810975268182 ) ) ;
#52511=CARTESIAN_POINT ( 'NONE',  ( 67.23580198090078852, 14.72857320832442696, -90.69627056048217639 ) ) ;
#52513=CARTESIAN_POINT ( 'NONE',  ( 46.23304607317102466, 10.41544405387738514, -73.07032476065955962 ) ) ;
#52515=CARTESIAN_POINT ( 'NONE',  ( 208.9585401441656529, 114.1617785893844399, 16.05179355318660583 ) ) ;
#52517=CARTESIAN_POINT ( 'NONE',  ( 181.0840389613909736, 78.60582251573003987, -24.38050707541595230 ) ) ;
#52519=CARTESIAN_POINT ( 'NONE',  ( -172.7116702014379541, 86.67317892691256986, 18.97714401617737323 ) ) ;
#52526=CARTESIAN_POINT ( 'NONE',  ( 128.4157044224114088, 39.39296260757092227, 4.980963091233736151 ) ) ;
#52528=CARTESIAN_POINT ( 'NONE',  ( -54.08816720029308556, 15.46531105893042302, 72.11509934368264396 ) ) ;
#52529=DIRECTION ( 'NONE',  ( 0.000000000000000000, 0.000000000000000000, 1.000000000000000000 ) ) ;
#52530=CARTESIAN_POINT ( 'NONE',  ( -48.56549579811110817, 13.03742088415616074, -38.92047726962127996 ) ) ;
#52533=CARTESIAN_POINT ( 'NONE',  ( 15.78827728214693416, -170.0000000000000000, -16.17439350822211352 ) ) ;
#52534=CARTESIAN_POINT ( 'NONE',  ( -59.56523643198713813, 15.93788386494078146, 70.65753556899086618 ) ) ;
#52535=ORIENTED_EDGE ( 'NONE', *, *, #25969, .T. ) ;
#52538=CARTESIAN_POINT ( 'NONE',  ( 41.99370981210045528, 9.776766948428255333, 84.05726211029711692 ) ) ;
#52539=CARTESIAN_POINT ( 'NONE',  ( -176.3896317155480347, 90.84057090619018027, -75.82101722059705651 ) ) ;
#52544=CARTESIAN_POINT ( 'NONE',  ( -0.5658006089934857208, 7.533733779014708531, 8.824489085581655345 ) ) ;
#52545=CARTESIAN_POINT ( 'NONE',  ( 157.4703587214989113, 58.92748579479260229, 44.40946747225338953 ) ) ;
#52546=CARTESIAN_POINT ( 'NONE',  ( 162.3437785836964053, 61.54175036639340135, 84.88835865730561636 ) ) ;
#52547=CARTESIAN_POINT ( 'NONE',  ( 94.02921784728459897, 22.08005910033065788, 38.45896049467276612 ) ) ;
#52549=VERTEX_POINT ( 'NONE', #33728 ) ;
#52553=CARTESIAN_POINT ( 'NONE',  ( -29.04400972079232801, 10.22852224114065400, 44.82796049359348700 ) ) ;
#52554=CARTESIAN_POINT ( 'NONE',  ( 197.8598785550297521, 99.02620879292953759, 33.61171724563484986 ) ) ;
#52555=CARTESIAN_POINT ( 'NONE',  ( -75.70982523951138887, 22.28913922295978267, 84.70770602012026984 ) ) ;
#52563=CARTESIAN_POINT ( 'NONE',  ( 201.9869293910475676, 102.6997661182767274, -63.66579325029184133 ) ) ;
#52564=LINE ( 'NONE', #4388, #43994 ) ;
#52565=CARTESIAN_POINT ( 'NONE',  ( -118.6157340058429668, 41.88485941274767299, 66.79490357616732865 ) ) ;
#52567=CARTESIAN_POINT ( 'NONE',  ( -82.33596576276354995, 24.83688096733768447, -9.211860750952368448 ) ) ;
#52569=CARTESIAN_POINT ( 'NONE',  ( -156.3790798118593273, 70.23422112803314121, -45.32992863352309598 ) ) ;
#52570=ORIENTED_EDGE ( 'NONE', *, *, #20170, .T. ) ;
#52572=ORIENTED_EDGE ( 'NONE', *, *, #43023, .T. ) ;
#52578=CARTESIAN_POINT ( 'NONE',  ( 111.5744020652610118, 29.50263541599086992, 83.41251877751304278 ) ) ;
#52579=CARTESIAN_POINT ( 'NONE',  ( 115.0485321076020568, 32.28990710985443968, -10.79877544804474354 ) ) ;
#52584=VERTEX_POINT ( 'NONE', #7692 ) ;
#52590=CARTESIAN_POINT ( 'NONE',  ( -38.54237244144231056, 11.89088379031760567, -67.24215503103580716 ) ) ;
#52592=CARTESIAN_POINT ( 'NONE',  ( 32.29989959354726636, 7.591763852038296179, 66.68145312022730309 ) ) ;
#52593=CARTESIAN_POINT ( 'NONE',  ( 45.58404625205363203, 9.294209029025518376, 86.84349537472557756 ) ) ;
#52594=CARTESIAN_POINT ( 'NONE',  ( 17.48988570800758424, 7.568061572928497682, 17.97865980060091928 ) ) ;
#52596=CARTESIAN_POINT ( 'NONE',  ( -118.4553071845214447, 41.78724769484929880, 10.17744028903938336 ) ) ;
#52599=CARTESIAN_POINT ( 'NONE',  ( 22.15943197741200166, 7.796127622097904109, -20.13900179068516394 ) ) ;
#52600=CARTESIAN_POINT ( 'NONE',  ( 157.4703587214989113, 57.65129005721575339, -36.12418429913763163 ) ) ;
#52601=ORIENTED_EDGE ( 'NONE', *, *, #31760, .F. ) ;
#52602=CARTESIAN_POINT ( 'NONE',  ( 157.4703587214989113, 58.92748579479260229, -36.12418429913763163 ) ) ;
#52606=CARTESIAN_POINT ( 'NONE',  ( 42.70988075781782811, 8.862408058333494765, -76.71303559248512727 ) ) ;
#52611=CARTESIAN_POINT ( 'NONE',  ( -25.35398647985413234, 8.671412257862231243, -20.36380365964988570 ) ) ;
#52612=CARTESIAN_POINT ( 'NONE',  ( 197.6329787101073805, 98.74106466892200729, 7.327278958723961289 ) ) ;
#52616=ORIENTED_EDGE ( 'NONE', *, *, #16464, .T. ) ;
#52617=CARTESIAN_POINT ( 'NONE',  ( 132.9557829392755366, 42.05591979570418459, -77.82755400474042062 ) ) ;
#52621=CARTESIAN_POINT ( 'NONE',  ( -99.11448999425219597, 31.20120877265620507, 31.20370467994214891 ) ) ;
#52630=ORIENTED_EDGE ( 'NONE', *, *, #64505, .F. ) ;
#52631=CARTESIAN_POINT ( 'NONE',  ( -118.9649285217355867, 42.09781191014327817, -18.45139938429198168 ) ) ;
#52634=CARTESIAN_POINT ( 'NONE',  ( -178.5835577246388368, 93.42126246260829703, -20.51231665930944459 ) ) ;
#52635=CARTESIAN_POINT ( 'NONE',  ( -133.3923804760465543, 52.87100816290224969, 64.39721494377326394 ) ) ;
#52637=CARTESIAN_POINT ( 'NONE',  ( 59.30258796551118650, 12.87111270082601244, 3.933392210405418865 ) ) ;
#52642=CARTESIAN_POINT ( 'NONE',  ( -57.65733424639444138, 15.39521790791522982, -8.834354978680334369 ) ) ;
#52643=CARTESIAN_POINT ( 'NONE',  ( -131.3096895243911035, 51.39228038925229924, -64.04718217629171306 ) ) ;
#52646=CARTESIAN_POINT ( 'NONE',  ( -150.3157714147627360, 64.86772057656135360, -88.53461949308422163 ) ) ;
#52650=CARTESIAN_POINT ( 'NONE',  ( 185.1647878987787124, 82.82967084668432278, -76.87782371961525030 ) ) ;
#52652=CARTESIAN_POINT ( 'NONE',  ( 8.000000000000007105, 249.8719672152120381, -95.00000000000133582 ) ) ;
#52653=DIRECTION ( 'NONE',  ( -0.000000000000000000, 1.000000000000000000, -0.000000000000000000 ) ) ;
#52654=CARTESIAN_POINT ( 'NONE',  ( -73.63128929564828695, 21.53548093502884342, 43.48216365791507343 ) ) ;
#52655=CARTESIAN_POINT ( 'NONE',  ( 84.73231936899557581, 18.78199960571076943, 29.94021395482606707 ) ) ;
#52656=CARTESIAN_POINT ( 'NONE',  ( -149.0732005398558044, 63.81212100765655748, 45.71137907923015575 ) ) ;
#52657=CARTESIAN_POINT ( 'NONE',  ( -118.9668643994983483, 43.27909474462861539, 41.00722457807798804 ) ) ;
#52658=CARTESIAN_POINT ( 'NONE',  ( -165.6210506643949145, 79.15024150453837137, -68.75523839542780991 ) ) ;
#52659=VERTEX_POINT ( 'NONE', #4142 ) ;
#52660=CARTESIAN_POINT ( 'NONE',  ( -108.9452487746634404, 36.29752968355630571, -19.14672792289445624 ) ) ;
#52666=CARTESIAN_POINT ( 'NONE',  ( 35.66087318222938762, 8.964867769223229033, 4.050215094464022059 ) ) ;
#52669=CARTESIAN_POINT ( 'NONE',  ( -97.49665543375860466, 31.53324358035375496, -63.56147199533193515 ) ) ;
#52670=CARTESIAN_POINT ( 'NONE',  ( -37.93983213483220851, 11.77368372188049506, -12.20019562758866627 ) ) ;
#52673=CARTESIAN_POINT ( 'NONE',  ( -125.4861769891490439, 47.42972183831692234, -88.60280507916131398 ) ) ;
#52676=CARTESIAN_POINT ( 'NONE',  ( 8.336237313193162635, 7.382629160459400985, -68.88587034052414992 ) ) ;
#52677=CARTESIAN_POINT ( 'NONE',  ( -23.93880457192868860, 8.479983864459176957, 11.11157786848920637 ) ) ;
#52681=CARTESIAN_POINT ( 'NONE',  ( 150.2805372522807374, 53.51147386362155345, -41.47252479654510893 ) ) ;
#52684=CARTESIAN_POINT ( 'NONE',  ( -151.2511071212632032, 67.00426547928870491, 72.37311975729836888 ) ) ;
#52685=CARTESIAN_POINT ( 'NONE',  ( 173.7263186949343776, 72.85225335320953377, -18.36293198726037801 ) ) ;
#52687=DIRECTION ( 'NONE',  ( 0.000000000000000000, 0.000000000000000000, 1.000000000000000000 ) ) ;
#52688=VERTEX_POINT ( 'NONE', #9419 ) ;
#52691=CARTESIAN_POINT ( 'NONE',  ( 94.12811352634518869, 22.11743943276049507, 63.53265709158580421 ) ) ;
#52692=CARTESIAN_POINT ( 'NONE',  ( 117.7447573007802930, 32.50990724960317380, 37.60142151178813918 ) ) ;
#52693=CARTESIAN_POINT ( 'NONE',  ( -147.4626691880993690, 62.46326773148431499, 84.67342306922898842 ) ) ;
#52694=CARTESIAN_POINT ( 'NONE',  ( 136.9798231265810671, 43.34196232604180921, 30.17573291222522869 ) ) ;
#52696=CARTESIAN_POINT ( 'NONE',  ( 197.2200752504831485, 96.62072041958357715, 37.37195676832524782 ) ) ;
#52698=CARTESIAN_POINT ( 'NONE',  ( 187.8973304652193406, 87.27378997243177139, 33.66165893027326916 ) ) ;
#52699=CARTESIAN_POINT ( 'NONE',  ( 156.3797504404255960, 58.07856685387021400, 29.48589258846897465 ) ) ;
#52702=CARTESIAN_POINT ( 'NONE',  ( 175.8947993867357411, 74.90689716047909030, 58.21729185181819588 ) ) ;
#52705=CARTESIAN_POINT ( 'NONE',  ( -108.6634958860518338, 36.14357436892402831, -38.56921122755016995 ) ) ;
#52706=CARTESIAN_POINT ( 'NONE',  ( 68.93219921887761359, 14.12322281954860692, -74.68096442457768092 ) ) ;
#52707=CARTESIAN_POINT ( 'NONE',  ( -61.86845765289633192, 16.61548683002700955, 34.67755665058201942 ) ) ;
#52709=CARTESIAN_POINT ( 'NONE',  ( 150.2193536046551685, 53.46717047532149536, 8.129190380543040106 ) ) ;
#52711=CARTESIAN_POINT ( 'NONE',  ( -178.0658882571760842, 92.80593104957425510, 32.67775869025225433 ) ) ;
#52712=EDGE_CURVE ( 'NONE', #51562, #66812, #9764, .T. ) ;
#52719=CARTESIAN_POINT ( 'NONE',  ( 139.7928618793172859, 45.12615179300591706, 68.44561210618307712 ) ) ;
#52720=CARTESIAN_POINT ( 'NONE',  ( -165.9111709580270997, 79.44576090485632847, 40.40830571265144755 ) ) ;
#52721=CARTESIAN_POINT ( 'NONE',  ( 150.9184679586218749, 52.73111408630722252, 67.41327876333463109 ) ) ;
#52725=CARTESIAN_POINT ( 'NONE',  ( 46.90208227351340753, 10.52324439420451085, 10.32737426675875625 ) ) ;
#52728=EDGE_CURVE ( 'NONE', #34501, #52414, #14683, .T. ) ;
#52729=CARTESIAN_POINT ( 'NONE',  ( 150.0516754638056227, 53.34587188591233797, -17.91502814048503112 ) ) ;
#52730=CARTESIAN_POINT ( 'NONE',  ( 208.9583973663598329, 114.1615900753670871, -23.16983956928563160 ) ) ;
#52731=CARTESIAN_POINT ( 'NONE',  ( 103.5589117581614715, 27.00490790413959985, 40.55142818294542906 ) ) ;
#52741=CARTESIAN_POINT ( 'NONE',  ( -98.46684543088107944, 30.88557736720388647, -36.05183115025165819 ) ) ;
#52742=CARTESIAN_POINT ( 'NONE',  ( 57.07734607129820148, 11.37318329671159844, -74.67266595444631605 ) ) ;
#52745=CARTESIAN_POINT ( 'NONE',  ( -11.28398375431312317, 7.140872483779192592, 84.64184783976759263 ) ) ;
#52747=CARTESIAN_POINT ( 'NONE',  ( 164.8914542114683854, 64.97670918603527923, -71.58997600903566649 ) ) ;
#52748=ORIENTED_EDGE ( 'NONE', *, *, #8440, .F. ) ;
#52750=DIRECTION ( 'NONE',  ( -0.8118923937861950435, -0.5838071093367415143, 0.000000000000000000 ) ) ;
#52757=CIRCLE ( 'NONE', #38149, 243.4957430088094839 ) ;
#52760=CARTESIAN_POINT ( 'NONE',  ( -126.8016613879753578, 48.30316697011515004, 45.57846390221672550 ) ) ;
#52761=VERTEX_POINT ( 'NONE', #3446 ) ;
#52762=CARTESIAN_POINT ( 'NONE',  ( 209.4789161463552034, 113.1367444519304399, 4.080444617825434328 ) ) ;
#52763=CARTESIAN_POINT ( 'NONE',  ( -144.2155061717026285, 61.10843690942982676, 43.54120042493494225 ) ) ;
#52764=CARTESIAN_POINT ( 'NONE',  ( 207.4696221732442609, 110.2206209205162395, 29.72680410229139270 ) ) ;
#52765=EDGE_CURVE ( 'NONE', #35021, #51770, #36149, .T. ) ;
#52766=CYLINDRICAL_SURFACE ( 'NONE', #58754, 7.500000000000020428 ) ;
#52767=EDGE_CURVE ( 'NONE', #62345, #4217, #32983, .T. ) ;
#52768=EDGE_LOOP ( 'NONE', ( #15862, #29719, #5756, #27956 ) ) ;
#52769=ORIENTED_EDGE ( 'NONE', *, *, #28339, .F. ) ;
#52772=CARTESIAN_POINT ( 'NONE',  ( -165.9111709580270997, 79.44576090485637110, -13.28079546827590107 ) ) ;
#52773=CARTESIAN_POINT ( 'NONE',  ( 140.8984307802396359, 45.84194788389004316, -73.00036953962161590 ) ) ;
#52774=CARTESIAN_POINT ( 'NONE',  ( 68.45098769362923008, 13.99935947269946546, 32.13933842162290233 ) ) ;
#52776=CARTESIAN_POINT ( 'NONE',  ( 9.152181272685988134, 7.385093848481300682, 94.71409728783903859 ) ) ;
#52779=EDGE_CURVE ( 'NONE', #64948, #53864, #27112, .T. ) ;
#52780=CARTESIAN_POINT ( 'NONE',  ( -94.85061234775062644, 29.16417548023186868, 63.80561842459411537 ) ) ;
#52782=EDGE_CURVE ( 'NONE', #30284, #59205, #4459, .T. ) ;
#52784=CARTESIAN_POINT ( 'NONE',  ( -81.01337222286372253, 23.22902179892322394, 3.934242872625056453 ) ) ;
#52785=ORIENTED_EDGE ( 'NONE', *, *, #61099, .T. ) ;
#52787=ADVANCED_FACE ( 'NONE', ( #28356 ), #34352, .F. ) ;
#52788=ORIENTED_EDGE ( 'NONE', *, *, #61745, .T. ) ;
#52789=CARTESIAN_POINT ( 'NONE',  ( 15.29899606819416569, 6.485153354884285015, -50.51894409868581448 ) ) ;
#52790=ADVANCED_FACE ( 'NONE', ( #23449 ), #55792, .F. ) ;
#52792=CARTESIAN_POINT ( 'NONE',  ( -179.9014775667592971, 95.00669833041665413, 61.94859390510309538 ) ) ;
#52793=CARTESIAN_POINT ( 'NONE',  ( 133.8566784816069344, 41.42467568809808398, 71.35489142945907304 ) ) ;
#52795=B_SPLINE_CURVE_WITH_KNOTS ( 'NONE', 3,
 ( #55369, #1216, #12125, #61690, #17384, #44475, #18096, #7551, #50101, #22669, #13514, #6495, #2610, #1931, #38863, #23389, #50453, #66997, #65591, #61002 ),
 .UNSPECIFIED., .F., .F.,
 ( 4, 2, 2, 2, 2, 2, 2, 2, 2, 4 ),
 ( 0.000000000000000000, 0.001710655815380748542, 0.002565983723071116416, 0.003421311630761484073, 0.005131967446142231097, 0.006842623261522978555, 0.008553279076903725145, 0.01026393489228447087, 0.01197459070766521833, 0.01368524652304596405 ),
 .UNSPECIFIED. ) ;
#52796=CARTESIAN_POINT ( 'NONE',  ( -24.41584901541038377, 8.543511933900191480, 88.69366999283610653 ) ) ;
#52797=CARTESIAN_POINT ( 'NONE',  ( 152.8430172091323413, 54.14068524174422237, 31.00228809141104236 ) ) ;
#52801=CARTESIAN_POINT ( 'NONE',  ( -26.49516976694651049, 8.831756547364859600, 43.37753662398635157 ) ) ;
#52802=CARTESIAN_POINT ( 'NONE',  ( -142.0070007485041117, 59.34878529741516218, -69.42688443671409004 ) ) ;
#52806=AXIS2_PLACEMENT_3D ( 'NONE', #59533, #47945, #31442 ) ;
#52809=CARTESIAN_POINT ( 'NONE',  ( -81.90760111942957167, 24.66532273091450378, -62.67973089774071838 ) ) ;
#52810=CARTESIAN_POINT ( 'NONE',  ( 177.7886308167536527, 76.74396398590873503, 16.71637049643586082 ) ) ;
#52812=DIRECTION ( 'NONE',  ( -0.000000000000000000, 1.000000000000000000, -0.000000000000000000 ) ) ;
#52813=CARTESIAN_POINT ( 'NONE',  ( 128.3856248084844651, 38.21741401878865929, 5.012217174567255462 ) ) ;
#52814=CARTESIAN_POINT ( 'NONE',  ( -153.7005182577089499, 67.81869626254724892, 17.61129303604968754 ) ) ;
#52815=CARTESIAN_POINT ( 'NONE',  ( 197.2059918558470031, 98.20695231513643364, 90.81591397967092405 ) ) ;
#52816=CARTESIAN_POINT ( 'NONE',  ( 63.50528314073022784, 12.78634332146811836, 17.96841034875761167 ) ) ;
#52817=CARTESIAN_POINT ( 'NONE',  ( 164.6406716478538783, 63.44801348349344039, 7.848966783923891910 ) ) ;
#52818=LINE ( 'NONE', #68996, #41034 ) ;
#52821=CARTESIAN_POINT ( 'NONE',  ( -54.44781833988737674, 15.56115186513848414, 84.02420198347161318 ) ) ;
#52822=VERTEX_POINT ( 'NONE', #53167 ) ;
#52825=CARTESIAN_POINT ( 'NONE',  ( 16.28382582968307446, 7.523443033994206885, -62.36349468914945504 ) ) ;
#52826=LINE ( 'NONE', #58794, #22628 ) ;
#52830=CARTESIAN_POINT ( 'NONE',  ( 141.0517870458593848, 47.14452711594499590, -41.39047569224774037 ) ) ;
#52831=CARTESIAN_POINT ( 'NONE',  ( 36.76746179515744473, 8.081433644308900099, -36.09346771175318480 ) ) ;
#52836=ORIENTED_EDGE ( 'NONE', *, *, #22290, .T. ) ;
#52837=CARTESIAN_POINT ( 'NONE',  ( 173.6087636303235513, 72.74229495189189265, 89.85593697944948133 ) ) ;
#52838=CARTESIAN_POINT ( 'NONE',  ( -167.6566265204789374, 82.70140535081088728, -10.22451876400831772 ) ) ;
#52844=CARTESIAN_POINT ( 'NONE',  ( 180.2572128312847610, 77.77323980479698662, -78.03573907910868002 ) ) ;
#52845=CARTESIAN_POINT ( 'NONE',  ( -180.2244609727085560, 95.39945930389649220, -44.63604071467989343 ) ) ;
#52846=CARTESIAN_POINT ( 'NONE',  ( 94.02921784728461319, 22.08005910033071117, -15.23014068625460027 ) ) ;
#52852=CARTESIAN_POINT ( 'NONE',  ( 128.0540543950622236, 39.18660671946770435, 14.94423530046998572 ) ) ;
#52854=CARTESIAN_POINT ( 'NONE',  ( 157.4703587214989398, -170.0000000000000000, -43.62418429913764584 ) ) ;
#52855=CARTESIAN_POINT ( 'NONE',  ( -78.66644367742111399, -170.0000000000000000, -69.46000122218158879 ) ) ;
#52856=CARTESIAN_POINT ( 'NONE',  ( 150.0501577908835884, 52.10460126680129633, 11.19079014285864204 ) ) ;
#52857=FACE_OUTER_BOUND ( 'NONE', #17453, .T. ) ;
#52858=EDGE_LOOP ( 'NONE', ( #21653, #68474, #58943, #51952 ) ) ;
#52860=EDGE_CURVE ( 'NONE', #36237, #11965, #21185, .T. ) ;
#52864=EDGE_CURVE ( 'NONE', #25590, #59450, #64001, .T. ) ;
#52865=EDGE_LOOP ( 'NONE', ( #25745, #60772 ) ) ;
#52866=CARTESIAN_POINT ( 'NONE',  ( 32.32377689436478363, 8.605407956458130059, 88.60103337961240300 ) ) ;
#52867=CARTESIAN_POINT ( 'NONE',  ( -179.9014775667593256, 95.00669833041665413, -72.27415904721529216 ) ) ;
#52868=B_SPLINE_CURVE_WITH_KNOTS ( 'NONE', 3,
 ( #45529, #67009, #45880, #3656, #25476, #46213, #46562, #46915, #25129, #18459 ),
 .UNSPECIFIED., .F., .F.,
 ( 4, 2, 2, 2, 4 ),
 ( 0.000000000000000000, 0.001117128179507491988, 0.002234256359014983977, 0.003351384538522475965, 0.004468512718029967953 ),
 .UNSPECIFIED. ) ;
#52869=FACE_OUTER_BOUND ( 'NONE', #35557, .T. ) ;
#52875=CARTESIAN_POINT ( 'NONE',  ( -0.3732240621745017695, 7.527003275829100559, 11.75034198667222718 ) ) ;
#52876=CARTESIAN_POINT ( 'NONE',  ( 174.4912080999798718, 73.57140295268875718, -40.13899342073425913 ) ) ;
#52877=CARTESIAN_POINT ( 'NONE',  ( 159.9380463867843503, 59.59435412114020636, 83.49017641889444974 ) ) ;
#52879=VECTOR ( 'NONE', #68206, 1000.000000000000000 ) ;
#52884=CARTESIAN_POINT ( 'NONE',  ( 13.37366753069832903, 6.435102282077983737, 57.24155959848373243 ) ) ;
#52885=CARTESIAN_POINT ( 'NONE',  ( 14.81290967676422277, 7.477658233646010899, 30.06210274491325407 ) ) ;
#52886=CARTESIAN_POINT ( 'NONE',  ( 204.6977192012829789, 108.0580384837235073, 44.20772073876944575 ) ) ;
#52888=CARTESIAN_POINT ( 'NONE',  ( -86.13811263329068879, 26.40116547045850837, 90.87883607248001283 ) ) ;
#52889=DIRECTION ( 'NONE',  ( -0.000000000000000000, 1.000000000000000000, -0.000000000000000000 ) ) ;
#52893=EDGE_CURVE ( 'NONE', #889, #59217, #37959, .T. ) ;
#52895=CARTESIAN_POINT ( 'NONE',  ( 116.0963032583228483, 32.80867113471310148, -74.98255735860550431 ) ) ;
#52896=DIRECTION ( 'NONE',  ( 0.000000000000000000, 0.000000000000000000, 1.000000000000000000 ) ) ;
#52897=CARTESIAN_POINT ( 'NONE',  ( 204.6977192012829789, 106.3443248447423457, -63.17048162308526571 ) ) ;
#52899=CARTESIAN_POINT ( 'NONE',  ( -55.05276343752909440, 14.68156374112638929, -23.37177340799619785 ) ) ;
#52900=LINE ( 'NONE', #4721, #53378 ) ;
#52901=CARTESIAN_POINT ( 'NONE',  ( 152.2940756559019064, 53.73566983921583784, -75.90150279893470042 ) ) ;
#52903=CARTESIAN_POINT ( 'NONE',  ( -152.9119739516381173, 67.12135129037710612, -49.01105990250665911 ) ) ;
#52905=VERTEX_POINT ( 'NONE', #21735 ) ;
#52906=CARTESIAN_POINT ( 'NONE',  ( 69.72564955710448942, 15.37006465677308675, -13.01647048107183124 ) ) ;
#52907=CARTESIAN_POINT ( 'NONE',  ( -85.64924756730678723, 26.19583280090850153, -45.36369601798204343 ) ) ;
#52908=CARTESIAN_POINT ( 'NONE',  ( 159.2389084450349515, 59.03884018680375334, 71.05616836873035425 ) ) ;
#52909=CARTESIAN_POINT ( 'NONE',  ( 117.3145357257065484, 33.41973663092564095, -14.02774205371277638 ) ) ;
#52910=CARTESIAN_POINT ( 'NONE',  ( 204.6977192012829789, 106.3443248447423173, -9.481380442157895772 ) ) ;
#52912=CARTESIAN_POINT ( 'NONE',  ( 133.8566784816069060, 42.60093787723652525, -9.178760341931967659 ) ) ;
#52913=VERTEX_POINT ( 'NONE', #27016 ) ;
#52917=CARTESIAN_POINT ( 'NONE',  ( 37.46876540261052924, 9.179568636624026112, -50.37052167088771881 ) ) ;
#52921=CARTESIAN_POINT ( 'NONE',  ( 197.3119541548906568, 98.33923235143190311, 62.23820161575331866 ) ) ;
#52922=ORIENTED_EDGE ( 'NONE', *, *, #16382, .T. ) ;
#52924=CARTESIAN_POINT ( 'NONE',  ( 15.78827728214693416, 6.500811158483328356, -8.674393508222097537 ) ) ;
#52926=CARTESIAN_POINT ( 'NONE',  ( 23.28845814680232351, 7.864847136539610872, 10.18352427007710759 ) ) ;
#52927=CARTESIAN_POINT ( 'NONE',  ( 187.2354698746857196, 85.05376776489248414, 59.33325302814636615 ) ) ;
#52933=CARTESIAN_POINT ( 'NONE',  ( 9.689943677145723910, 7.388265075009363692, 6.297457479611937359 ) ) ;
#52937=CARTESIAN_POINT ( 'NONE',  ( 188.4359598230020367, 86.36951380984524462, 8.452180733291799086 ) ) ;
#52940=CARTESIAN_POINT ( 'NONE',  ( 174.2469308602415197, 71.96142024047685481, 33.71361340695089126 ) ) ;
#52942=CARTESIAN_POINT ( 'NONE',  ( -109.7643866341847314, 37.89854104106755983, -43.06589634579863457 ) ) ;
#52943=CARTESIAN_POINT ( 'NONE',  ( 188.0094179620990928, 87.39792407168452826, -46.61815432678586291 ) ) ;
#52945=B_SPLINE_CURVE_WITH_KNOTS ( 'NONE', 3,
 ( #32024, #27418, #22153, #16529, #59080, #43598, #26058, #15504, #37984, #54137, #5283, #42898, #36954, #48856, #33061, #47837 ),
 .UNSPECIFIED., .F., .F.,
 ( 4, 2, 2, 2, 2, 2, 2, 4 ),
 ( 0.01170309506547633979, 0.01321020703997516713, 0.01471731901447399446, 0.01773154296347164566, 0.01923865493797047993, 0.02074576691246931073, 0.02225287888696814154, 0.02375999086146697581 ),
 .UNSPECIFIED. ) ;
#52949=CARTESIAN_POINT ( 'NONE',  ( 204.3091227790962705, 107.5190503136782638, 17.36317014830577676 ) ) ;
#52952=CARTESIAN_POINT ( 'NONE',  ( 112.1164716692773879, 29.75790342121401366, 71.23340654744586686 ) ) ;
#52956=ADVANCED_FACE ( 'NONE', ( #31614 ), #4536, .F. ) ;
#52963=ORIENTED_EDGE ( 'NONE', *, *, #21924, .F. ) ;
#52964=VERTEX_POINT ( 'NONE', #26685 ) ;
#52965=CARTESIAN_POINT ( 'NONE',  ( -167.1619226259399511, 82.18315278115417755, 6.916214303503440242 ) ) ;
#52969=CARTESIAN_POINT ( 'NONE',  ( -147.3614567344829709, 62.37986555269943523, -35.11266540856631480 ) ) ;
#52971=CARTESIAN_POINT ( 'NONE',  ( -107.0277617056979551, 36.40097422522767090, 85.89409362202775355 ) ) ;
#52974=AXIS2_PLACEMENT_3D ( 'NONE', #46309, #30156, #19941 ) ;
#52979=CARTESIAN_POINT ( 'NONE',  ( -133.0835080491124813, 52.64966140620843049, -71.40981646950953632 ) ) ;
#52982=CARTESIAN_POINT ( 'NONE',  ( -95.88718821240198054, 29.65015105908824822, -73.28914486612443113 ) ) ;
#52983=ORIENTED_EDGE ( 'NONE', *, *, #16814, .F. ) ;
#52991=CARTESIAN_POINT ( 'NONE',  ( -71.57025115638937507, 20.80908992785612810, 35.43902869127500566 ) ) ;
#52992=CARTESIAN_POINT ( 'NONE',  ( 82.34195123877069022, 18.00239921638039320, 43.37057751023843366 ) ) ;
#52993=CARTESIAN_POINT ( 'NONE',  ( 69.83260694998126894, 15.39825517924929521, -40.08384761986350497 ) ) ;
#52994=CARTESIAN_POINT ( 'NONE',  ( -120.6420427933462207, 44.31795133507804252, 32.75998872186478650 ) ) ;
#52995=CARTESIAN_POINT ( 'NONE',  ( 210.9747454890631673, 115.3673079504855963, 67.66528286333071662 ) ) ;
#52996=ORIENTED_EDGE ( 'NONE', *, *, #51571, .T. ) ;
#52997=FACE_OUTER_BOUND ( 'NONE', #39961, .T. ) ;
#53002=CARTESIAN_POINT ( 'NONE',  ( 154.4429418375332546, 55.33424769452791026, -23.65634912063520545 ) ) ;
#53004=DIRECTION ( 'NONE',  ( -0.8160245890732938934, -0.5780171883497599028, 0.000000000000000000 ) ) ;
#53005=CARTESIAN_POINT ( 'NONE',  ( 32.09567473596477072, 7.571373529017936477, -68.25274485065961017 ) ) ;
#53007=CARTESIAN_POINT ( 'NONE',  ( -34.52542994698664813, 11.14027065218092361, -9.132801045176456967 ) ) ;
#53009=CARTESIAN_POINT ( 'NONE',  ( -124.2594596607281119, 46.62660695211089745, -88.78007805360886096 ) ) ;
#53013=DIRECTION ( 'NONE',  ( -1.000000000000000000, 0.000000000000000000, 0.000000000000000000 ) ) ;
#53014=LINE ( 'NONE', #68193, #68212 ) ;
#53015=CARTESIAN_POINT ( 'NONE',  ( -0.5183605925911985990, 6.525266619725956119, 35.90767484529200004 ) ) ;
#53017=CARTESIAN_POINT ( 'NONE',  ( -94.78109144324895396, 29.13179392050636451, -15.95525421150224155 ) ) ;
#53018=CARTESIAN_POINT ( 'NONE',  ( 151.1700480242206197, 54.15904440870136227, -39.54687096424860471 ) ) ;
#53019=EDGE_CURVE ( 'NONE', #45299, #66935, #12814, .T. ) ;
#53025=CARTESIAN_POINT ( 'NONE',  ( 174.1422537179815322, 73.24254491731257133, -19.73406368843727066 ) ) ;
#53026=CARTESIAN_POINT ( 'NONE',  ( -107.0544991134679265, 36.41543129049374272, 59.07449925621195774 ) ) ;
#53032=CARTESIAN_POINT ( 'NONE',  ( -7.336760511143403107, 6.859209474528208617, -23.57352014148015584 ) ) ;
#53033=CARTESIAN_POINT ( 'NONE',  ( 203.1414537950835779, 105.9225671689748225, -9.634034691959321606 ) ) ;
#53035=CARTESIAN_POINT ( 'NONE',  ( -142.1225587277077409, 58.16021019177119200, 90.55535391989825200 ) ) ;
#53037=CARTESIAN_POINT ( 'NONE',  ( 136.9934874058118055, 43.35050367224292245, 43.83853296350712014 ) ) ;
#53042=EDGE_CURVE ( 'NONE', #11991, #66081, #24591, .T. ) ;
#53043=CARTESIAN_POINT ( 'NONE',  ( 153.2523375521184335, 55.69936538551847605, 30.70342358034734787 ) ) ;
#53044=DIRECTION ( 'NONE',  ( -0.000000000000000000, 1.000000000000000000, -0.000000000000000000 ) ) ;
#53049=CARTESIAN_POINT ( 'NONE',  ( 63.49940197359692462, 12.78497925206076502, -77.56524142263349120 ) ) ;
#53051=CARTESIAN_POINT ( 'NONE',  ( 150.7770046255792522, 53.87214803240242844, 13.45895202400941848 ) ) ;
#53052=ORIENTED_EDGE ( 'NONE', *, *, #45896, .T. ) ;
#53053=CARTESIAN_POINT ( 'NONE',  ( -176.3791001330698975, 90.82833141237287577, 45.09165477967572855 ) ) ;
#53057=DIRECTION ( 'NONE',  ( -0.000000000000000000, 1.000000000000000000, -0.000000000000000000 ) ) ;
#53059=CARTESIAN_POINT ( 'NONE',  ( -175.9864315813574933, 91.91454246454364352, 31.37775927267171738 ) ) ;
#53060=CARTESIAN_POINT ( 'NONE',  ( -37.92542950990690542, 10.74638084523341774, -73.43514582413676806 ) ) ;
#53061=CARTESIAN_POINT ( 'NONE',  ( 186.2651679807462699, 84.00458780104314371, -22.32374867702027998 ) ) ;
#53063=CARTESIAN_POINT ( 'NONE',  ( 46.23113030541875901, 10.41513832761375902, 13.67933782382501917 ) ) ;
#53064=ORIENTED_EDGE ( 'NONE', *, *, #34550, .T. ) ;
#53067=CARTESIAN_POINT ( 'NONE',  ( -52.00013736311785806, 13.88364424352426774, 84.62652642927972124 ) ) ;
#53068=CARTESIAN_POINT ( 'NONE',  ( 105.4134760436918583, 27.80903124201758203, 42.87025001487361209 ) ) ;
#53072=CARTESIAN_POINT ( 'NONE',  ( 182.7745872728868051, 81.77554423487157464, 17.32141904578063318 ) ) ;
#53073=CARTESIAN_POINT ( 'NONE',  ( 212.0850679406003678, 117.0583048437722340, -42.48649401792513203 ) ) ;
#53076=ORIENTED_EDGE ( 'NONE', *, *, #32234, .T. ) ;
#53078=EDGE_LOOP ( 'NONE', ( #9726, #34098, #35281, #2946 ) ) ;
#53081=DIRECTION ( 'NONE',  ( -0.000000000000000000, 1.000000000000000000, -0.000000000000000000 ) ) ;
#53082=CARTESIAN_POINT ( 'NONE',  ( 55.76066037845577483, 11.10616952318092032, -72.03042357651290217 ) ) ;
#53088=ORIENTED_EDGE ( 'NONE', *, *, #13251, .F. ) ;
#53089=CARTESIAN_POINT ( 'NONE',  ( -74.79002408692174697, 20.88280597089420709, 71.18791309357050068 ) ) ;
#53090=CARTESIAN_POINT ( 'NONE',  ( 198.3695851305816973, 98.05090906089078828, -93.48290386845097544 ) ) ;
#53093=CARTESIAN_POINT ( 'NONE',  ( -155.2912910578197057, 69.24479901948498650, 43.00208789238233464 ) ) ;
#53095=CARTESIAN_POINT ( 'NONE',  ( 55.51597771111714508, 11.05737652677076177, -42.72098034633929586 ) ) ;
#53098=CARTESIAN_POINT ( 'NONE',  ( -55.05276343752910151, -170.0000000000000000, -88.90542517938720835 ) ) ;
#53103=CARTESIAN_POINT ( 'NONE',  ( -132.0738857626834033, 51.93126104279146205, 33.86320823520932066 ) ) ;
#53105=DIRECTION ( 'NONE',  ( -0.000000000000000000, 0.000000000000000000, -1.000000000000000000 ) ) ;
#53106=CARTESIAN_POINT ( 'NONE',  ( -144.9417090887490929, 61.69631066549397502, 32.26605393151823620 ) ) ;
#53107=CARTESIAN_POINT ( 'NONE',  ( 56.30171512200996631, 11.21502580416396100, 67.50933623815409135 ) ) ;
#53110=LINE ( 'NONE', #26406, #47264 ) ;
#53116=CARTESIAN_POINT ( 'NONE',  ( -169.8842709557925161, 83.59602878049477681, -22.14760816498463214 ) ) ;
#53118=DIRECTION ( 'NONE',  ( -0.8160245890732938934, -0.5780171883497599028, 0.000000000000000000 ) ) ;
#53119=CARTESIAN_POINT ( 'NONE',  ( 22.46018177512842584, 7.813889158582806083, 87.76227202242357350 ) ) ;
#53126=CARTESIAN_POINT ( 'NONE',  ( -85.75947274862031122, 25.15128705015480648, 8.585276764537949745 ) ) ;
#53131=CARTESIAN_POINT ( 'NONE',  ( 13.84120792123769128, 6.445822122644895735, -50.27834514783636166 ) ) ;
#53132=CARTESIAN_POINT ( 'NONE',  ( -173.9656771507955000, 88.06879734510549440, 72.66624519710475738 ) ) ;
#53133=CARTESIAN_POINT ( 'NONE',  ( 126.3580543567275640, 37.07735301062819389, 64.15879660461148148 ) ) ;
#53135=CARTESIAN_POINT ( 'NONE',  ( -38.33502649974140297, 10.82522693986058471, 94.42607965810407222 ) ) ;
#53138=CARTESIAN_POINT ( 'NONE',  ( 102.7551177910568612, 25.56939188780864924, -43.91997128112426196 ) ) ;
#53139=CARTESIAN_POINT ( 'NONE',  ( -29.02794087136069834, 9.207646203414352470, 44.83495968200595172 ) ) ;
#53144=CARTESIAN_POINT ( 'NONE',  ( -3.792733964105130084, 6.661044795567934607, -90.22612808589047972 ) ) ;
#53145=CARTESIAN_POINT ( 'NONE',  ( -118.3948752128398922, 42.92869324237091888, -42.11633704353932472 ) ) ;
#53147=DIRECTION ( 'NONE',  ( -0.8160245890732938934, -0.5780171883497599028, 0.000000000000000000 ) ) ;
#53149=CARTESIAN_POINT ( 'NONE',  ( -155.1355020251929488, 69.10372769512068203, 6.393537426473839602 ) ) ;
#53150=CARTESIAN_POINT ( 'NONE',  ( 197.5084910509550298, 98.58493024928847603, 92.57377601736234851 ) ) ;
#53151=CARTESIAN_POINT ( 'NONE',  ( 68.95451040317568925, 14.12887482153123742, 15.07515996775212841 ) ) ;
#53153=CARTESIAN_POINT ( 'NONE',  ( 90.30840373526895348, 21.77864858272153725, -23.01712743521610349 ) ) ;
#53154=EDGE_CURVE ( 'NONE', #56804, #26121, #35477, .T. ) ;
#53155=ORIENTED_EDGE ( 'NONE', *, *, #17966, .T. ) ;
#53158=CARTESIAN_POINT ( 'NONE',  ( -50.13240733217616452, 14.45347886670807647, 85.83683214817698115 ) ) ;
#53159=ORIENTED_EDGE ( 'NONE', *, *, #17946, .F. ) ;
#53160=DIRECTION ( 'NONE',  ( -0.000000000000000000, 1.000000000000000000, -0.000000000000000000 ) ) ;
#53162=CARTESIAN_POINT ( 'NONE',  ( 21.44191228441539110, 7.755009954762316582, -74.81642095281917193 ) ) ;
#53165=CARTESIAN_POINT ( 'NONE',  ( -142.0729208125266325, 59.40063722436775606, 66.20298747330664924 ) ) ;
#53166=CARTESIAN_POINT ( 'NONE',  ( 69.08240197259641491, 14.16210831900843736, -20.79263225278958771 ) ) ;
#53167=CARTESIAN_POINT ( 'NONE',  ( -71.28077210551055032, 19.64439276383075850, -95.00000000000133582 ) ) ;
#53168=CARTESIAN_POINT ( 'NONE',  ( -47.55256438668344998, 13.83151366677316751, -69.80307781500179942 ) ) ;
#53177=CARTESIAN_POINT ( 'NONE',  ( 178.9724693410834391, 77.91338280736979982, 83.29495941411636295 ) ) ;
#53182=CARTESIAN_POINT ( 'NONE',  ( 70.02150084181303669, 15.44810330738962634, -94.20035217677271078 ) ) ;
#53184=CARTESIAN_POINT ( 'NONE',  ( -9.525868120571908904, 7.007646177566257073, 71.76889433962945475 ) ) ;
#53185=CARTESIAN_POINT ( 'NONE',  ( -81.23297981660235223, 23.31577157498398378, -8.719607575958333356 ) ) ;
#53188=CARTESIAN_POINT ( 'NONE',  ( 86.62931800182293784, -170.0000000000000000, -89.51066537983906812 ) ) ;
#53190=CARTESIAN_POINT ( 'NONE',  ( 160.2883311361770211, 61.16711613734478448, 70.70813550747246268 ) ) ;
#53191=( BOUNDED_CURVE ( )  B_SPLINE_CURVE ( 3, ( #59601, #7570, #50466, #2287 ),
 .UNSPECIFIED., .F., .F. ) 
 B_SPLINE_CURVE_WITH_KNOTS ( ( 4, 4 ),
 ( 2.506209174768084580, 3.776976132411493658 ),
 .UNSPECIFIED. ) 
 CURVE ( )  GEOMETRIC_REPRESENTATION_ITEM ( )  RATIONAL_B_SPLINE_CURVE ( ( 1.000000000000000000, 0.8698961108463049152, 0.8698961108463049152, 1.000000000000000000 ) ) 
 REPRESENTATION_ITEM ( '' )  );
#53193=ORIENTED_EDGE ( 'NONE', *, *, #15624, .T. ) ;
#53194=CARTESIAN_POINT ( 'NONE',  ( -124.3250225421925848, 45.46958056770282752, -35.07612196727420439 ) ) ;
#53197=DIRECTION ( 'NONE',  ( -0.000000000000000000, 1.000000000000000000, -0.000000000000000000 ) ) ;
#53198=CARTESIAN_POINT ( 'NONE',  ( 150.4550062612853765, 52.39582885725847206, 12.76969944096150478 ) ) ;
#53212=CARTESIAN_POINT ( 'NONE',  ( -60.66241560458682613, 16.25736033771447708, -74.56350396580954509 ) ) ;
#53215=CARTESIAN_POINT ( 'NONE',  ( 34.83825437341838693, 7.859462995505738014, -22.24695001896300539 ) ) ;
#53216=CARTESIAN_POINT ( 'NONE',  ( 179.4074606910091632, 78.34362448405029511, -36.36429642586875843 ) ) ;
#53225=DIRECTION ( 'NONE',  ( -0.8160245890732938934, -0.5780171883497599028, 0.000000000000000000 ) ) ;
#53226=CARTESIAN_POINT ( 'NONE',  ( 14.08810621383467065, 7.458732232275139928, 30.20580324848959464 ) ) ;
#53227=CARTESIAN_POINT ( 'NONE',  ( 198.4045886930829568, 99.71425793793709147, 32.61891997574733182 ) ) ;
#53238=CARTESIAN_POINT ( 'NONE',  ( -33.83721310978699393, 11.01869210665941523, 57.45054862161848774 ) ) ;
#53239=CARTESIAN_POINT ( 'NONE',  ( -13.79190010541702982, 8.363435739308560102, -11.50286335269423788 ) ) ;
#53240=CARTESIAN_POINT ( 'NONE',  ( 155.7277429502854318, 56.30804678861343149, -77.77684271661371440 ) ) ;
#53243=LINE ( 'NONE', #5068, #25054 ) ;
#53246=CARTESIAN_POINT ( 'NONE',  ( 70.12389542974196388, 15.47520081968154848, -18.81922647478308619 ) ) ;
#53247=CARTESIAN_POINT ( 'NONE',  ( -80.31482177285907653, 24.03632224640839254, -49.93594921041977130 ) ) ;
#53248=CARTESIAN_POINT ( 'NONE',  ( 158.3604774538084428, 58.34594647925809596, 71.21437032374478804 ) ) ;
#53249=CARTESIAN_POINT ( 'NONE',  ( -156.4966862384868307, 71.70877417666511633, 14.14904641178471323 ) ) ;
#53250=CARTESIAN_POINT ( 'NONE',  ( 182.7789203043889756, 80.33475476315295793, -36.40670569473370222 ) ) ;
#53251=CARTESIAN_POINT ( 'NONE',  ( 23.28869764673362397, 6.856674305776598644, 38.00306743024603406 ) ) ;
#53252=CARTESIAN_POINT ( 'NONE',  ( -156.1162923254352961, 71.35845171916716367, 88.34953077652313880 ) ) ;
#53253=VERTEX_POINT ( 'NONE', #58301 ) ;
#53259=CARTESIAN_POINT ( 'NONE',  ( 32.38493285958205092, 8.611594965040671568, -45.77910956698918454 ) ) ;
#53260=CARTESIAN_POINT ( 'NONE',  ( 179.0096185093687779, 76.53352131383246615, 56.43267003127355963 ) ) ;
#53263=CARTESIAN_POINT ( 'NONE',  ( -37.79823708645147917, 10.72197716414928870, 60.57713633437269607 ) ) ;
#53264=CARTESIAN_POINT ( 'NONE',  ( -152.9119739516381458, 67.12135129037709191, -22.16650931204297237 ) ) ;
#53267=CARTESIAN_POINT ( 'NONE',  ( 186.2575601542430377, 85.47765906955505955, 69.08854037509910029 ) ) ;
#53268=CARTESIAN_POINT ( 'NONE',  ( 45.80999061969644970, 9.329701754959341287, 94.99999999999866418 ) ) ;
#53270=CARTESIAN_POINT ( 'NONE',  ( 15.78827728214693060, 7.507518794609573831, 18.17015708224157322 ) ) ;
#53271=CARTESIAN_POINT ( 'NONE',  ( 186.2722199822849518, 84.01218714714249813, 69.08924636671144981 ) ) ;
#53273=CARTESIAN_POINT ( 'NONE',  ( -85.34215807311494473, 24.97769003780924635, -39.18790712996867853 ) ) ;
#53275=CARTESIAN_POINT ( 'NONE',  ( 19.53470118933705280, 6.649487981843461348, 57.85738236312793248 ) ) ;
#53277=CARTESIAN_POINT ( 'NONE',  ( 200.8298320869470217, 101.1869877914233626, 57.11224534795069729 ) ) ;
#53279=CARTESIAN_POINT ( 'NONE',  ( 183.1910712700538397, 80.76073941711163684, 17.17481853169963912 ) ) ;
#53280=CARTESIAN_POINT ( 'NONE',  ( 173.7246046907418986, 71.47482343504563573, 38.28278645884536502 ) ) ;
#53281=CARTESIAN_POINT ( 'NONE',  ( -133.1093894320205777, 51.43221067881454189, -44.53048774310489932 ) ) ;
#53283=CARTESIAN_POINT ( 'NONE',  ( -102.2801239173131194, 33.91021738430207222, -35.01457726497591239 ) ) ;
#53284=ADVANCED_FACE ( 'NONE', ( #58636 ), #9783, .F. ) ;
#53285=CARTESIAN_POINT ( 'NONE',  ( 57.57684776206772170, 12.50442334002048561, -75.23527395922451433 ) ) ;
#53287=EDGE_LOOP ( 'NONE', ( #53607, #65012 ) ) ;
#53288=EDGE_CURVE ( 'NONE', #14559, #12765, #963, .T. ) ;
#53291=CARTESIAN_POINT ( 'NONE',  ( 173.5758067325220395, 71.33673452833791373, 90.29149762729994677 ) ) ;
#53296=CARTESIAN_POINT ( 'NONE',  ( 129.6961120139403647, 38.96846414226718736, 30.76564539126953335 ) ) ;
#53299=CARTESIAN_POINT ( 'NONE',  ( 93.61951000632932107, 21.92572933971849380, -46.05087944202944072 ) ) ;
#53301=ORIENTED_EDGE ( 'NONE', *, *, #23229, .F. ) ;
#53304=CARTESIAN_POINT ( 'NONE',  ( -118.8689810167775676, 42.03922634358558952, -18.20944547944688452 ) ) ;
#53307=DIRECTION ( 'NONE',  ( 0.000000000000000000, 0.000000000000000000, 1.000000000000000000 ) ) ;
#53309=CARTESIAN_POINT ( 'NONE',  ( -146.5341851369306028, 61.69744206542952014, -49.21242434289558076 ) ) ;
#53311=CARTESIAN_POINT ( 'NONE',  ( 61.33840119549016379, 13.32121602003046945, 3.154318263180942772 ) ) ;
#53313=AXIS2_PLACEMENT_3D ( 'NONE', #4163, #14708, #53013 ) ;
#53315=CARTESIAN_POINT ( 'NONE',  ( -133.3926783185152090, 51.63401075114364858, 38.42124472836754023 ) ) ;
#53316=CARTESIAN_POINT ( 'NONE',  ( -58.33245019990695113, 15.58496056636070293, -9.109388937163927835 ) ) ;
#53320=CARTESIAN_POINT ( 'NONE',  ( 135.0005116824453921, 43.29964618809725607, 29.59450486721033258 ) ) ;
#53322=CARTESIAN_POINT ( 'NONE',  ( -190.6985136298601731, 109.1272424661242582, -95.00000000000133582 ) ) ;
#53324=CARTESIAN_POINT ( 'NONE',  ( -95.63568360745007624, 29.53168204475775838, 7.686534007699536097 ) ) ;
#53325=CARTESIAN_POINT ( 'NONE',  ( -153.4231522284453320, 67.57115137896495582, -89.54656928398240723 ) ) ;
#53327=ORIENTED_EDGE ( 'NONE', *, *, #36274, .T. ) ;
#53328=CARTESIAN_POINT ( 'NONE',  ( 188.5645326065591405, 86.51153908883290455, -71.18896735030770628 ) ) ;
#53332=CARTESIAN_POINT ( 'NONE',  ( 102.7938674513918897, 26.67851209377773003, -69.25574476757175546 ) ) ;
#53333=CARTESIAN_POINT ( 'NONE',  ( -78.66644367742109978, 23.39876645725290061, 45.41820113967312977 ) ) ;
#53334=CARTESIAN_POINT ( 'NONE',  ( 85.67452303415194592, 19.09699411916382061, 44.66627896201372749 ) ) ;
#53335=CARTESIAN_POINT ( 'NONE',  ( 63.01563776193091826, 13.70579113808095073, -50.72069083216976537 ) ) ;
#53336=CARTESIAN_POINT ( 'NONE',  ( 43.96421756700841144, 10.06386361114660133, -49.09255290175231323 ) ) ;
#53337=CARTESIAN_POINT ( 'NONE',  ( 210.1954643503415525, 114.1986276268024056, 68.65963326422985347 ) ) ;
#53340=DIRECTION ( 'NONE',  ( 0.000000000000000000, 0.000000000000000000, 1.000000000000000000 ) ) ;
#53342=CARTESIAN_POINT ( 'NONE',  ( -14.32120159453989494, 7.401444311907543039, -46.67511467244946033 ) ) ;
#53343=CARTESIAN_POINT ( 'NONE',  ( 80.71682498289318630, 18.54204664833076066, 68.69748318965059752 ) ) ;
#53345=CARTESIAN_POINT ( 'NONE',  ( 91.49210130311621469, 22.20929244416437598, 69.77178660558656986 ) ) ;
#53347=DIRECTION ( 'NONE',  ( 0.000000000000000000, 0.000000000000000000, 1.000000000000000000 ) ) ;
#53349=CARTESIAN_POINT ( 'NONE',  ( 33.03722315490662709, 7.666819786578624729, -65.98931375990046888 ) ) ;
#53355=CARTESIAN_POINT ( 'NONE',  ( 61.33840119549017089, 13.32121602003047478, 56.84341944410832781 ) ) ;
#53356=CARTESIAN_POINT ( 'NONE',  ( 9.050324533885209632, 7.384616180193988022, -73.19382097837868173 ) ) ;
#53357=FACE_OUTER_BOUND ( 'NONE', #18680, .T. ) ;
#53358=CARTESIAN_POINT ( 'NONE',  ( 39.40195752203892710, 9.424259417798131366, 56.75838489642694640 ) ) ;
#53359=CARTESIAN_POINT ( 'NONE',  ( -0.8055628312658249524, 6.535476276302842003, 34.96376056659171638 ) ) ;
#53360=CARTESIAN_POINT ( 'NONE',  ( -94.77925136849377452, 29.13093715379786275, -15.43817801418533797 ) ) ;
#53361=CARTESIAN_POINT ( 'NONE',  ( 79.12226143468465978, 18.04701779285957741, 90.79126889306922976 ) ) ;
#53367=CARTESIAN_POINT ( 'NONE',  ( 173.9405361758638264, 73.05302209498819366, -14.57814776013407965 ) ) ;
#53370=CARTESIAN_POINT ( 'NONE',  ( -132.4776673493542773, 52.21763813822158085, -46.01489453234746207 ) ) ;
#53373=CARTESIAN_POINT ( 'NONE',  ( -0.7174461528505726715, 6.532311451815525416, -13.66781165024909228 ) ) ;
#53375=CARTESIAN_POINT ( 'NONE',  ( 202.7506655727288774, 105.3943386412348957, -9.726947921299894162 ) ) ;
#53377=CARTESIAN_POINT ( 'NONE',  ( -142.0374482299984891, 58.09359183931726278, 92.66567792160763872 ) ) ;
#53378=VECTOR ( 'NONE', #64507, 1000.000000000000000 ) ;
#53379=CARTESIAN_POINT ( 'NONE',  ( 138.5721691894144101, 44.34516164557649631, 31.15771391547428948 ) ) ;
#53383=CARTESIAN_POINT ( 'NONE',  ( 159.6614743841974473, 60.66237087206236112, 2.878128257468113738 ) ) ;
#53386=CARTESIAN_POINT ( 'NONE',  ( 174.2468109002382448, 73.34092405459590225, 66.74791253496901788 ) ) ;
#53388=CARTESIAN_POINT ( 'NONE',  ( -105.4589068214114178, 34.42476264325678414, -49.32389774318545506 ) ) ;
#53390=CARTESIAN_POINT ( 'NONE',  ( -61.75629144857964548, 16.58190704077737720, 41.18998502750409330 ) ) ;
#53392=ORIENTED_EDGE ( 'NONE', *, *, #50768, .F. ) ;
#53393=CARTESIAN_POINT ( 'NONE',  ( -180.2244609727085560, 95.39945930389649220, 35.89761105671116326 ) ) ;
#53394=CARTESIAN_POINT ( 'NONE',  ( 15.78827728214693416, -170.0000000000000000, 56.85925826316891829 ) ) ;
#53396=VERTEX_POINT ( 'NONE', #61085 ) ;
#53400=CARTESIAN_POINT ( 'NONE',  ( 140.4586216751744985, 45.55624550472995793, 60.28699697572574223 ) ) ;
#53402=CARTESIAN_POINT ( 'NONE',  ( -177.5100621450480105, 93.70693725195826573, 32.22205096411517644 ) ) ;
#53403=CARTESIAN_POINT ( 'NONE',  ( 127.2358066117906787, 38.72257733469226082, 60.29414159756798597 ) ) ;
#53404=ORIENTED_EDGE ( 'NONE', *, *, #7555, .F. ) ;
#53405=CARTESIAN_POINT ( 'NONE',  ( 42.03719354205839664, 9.783015072457470040, 17.59534908508582518 ) ) ;
#53410=CARTESIAN_POINT ( 'NONE',  ( -47.71021106038689652, 12.83493994394914672, 89.94366651930251066 ) ) ;
#53413=FACE_OUTER_BOUND ( 'NONE', #41128, .T. ) ;
#53414=CARTESIAN_POINT ( 'NONE',  ( -109.7470238012287496, 36.73863861880653303, 92.48605150114060791 ) ) ;
#53423=ORIENTED_EDGE ( 'NONE', *, *, #42026, .F. ) ;
#53427=CARTESIAN_POINT ( 'NONE',  ( 210.9506883977752523, 115.3310071214937125, -74.81997715654915737 ) ) ;
#53430=CARTESIAN_POINT ( 'NONE',  ( -71.26675986148647723, 19.63956187826083877, 12.32191659035411391 ) ) ;
#53431=CARTESIAN_POINT ( 'NONE',  ( -120.0051930351106790, 43.92079660368834482, 69.61615127784293122 ) ) ;
#53432=CARTESIAN_POINT ( 'NONE',  ( 22.28700331106867338, 7.803633676228379557, 41.26662101868341637 ) ) ;
#53433=CARTESIAN_POINT ( 'NONE',  ( 199.7240524537553483, 99.76461913835838402, 84.77326177708235377 ) ) ;
#53434=CARTESIAN_POINT ( 'NONE',  ( 159.2325040199866919, 60.31699144791973310, -63.12323753459439502 ) ) ;
#53440=CARTESIAN_POINT ( 'NONE',  ( -23.93933407965396398, 9.495050561681678047, -69.16614878619023443 ) ) ;
#53442=B_SPLINE_CURVE_WITH_KNOTS ( 'NONE', 3,
 ( #68946, #43244, #21457, #58066, #16178, #9885, #26060, #64720, #16531, #20770, #63691, #15506, #58394, #10206, #66480, #12654, #5962, #54848, #28121, #18276, #49563, #1395, #22849, #7382, #16868, #11584, #1052, #12301, #34113, #65420, #54494, #39382, #43940, #17210, #65069, #38326, #54139, #28834, #59770, #6320, #44665, #23214, #11241 ),
 .UNSPECIFIED., .F., .F.,
 ( 4, 2, 2, 2, 2, 2, 2, 2, 1, 2, 2, 2, 2, 2, 2, 2, 2, 2, 2, 2, 2, 4 ),
 ( 0.000000000000000000, 0.001466540241398126216, 0.002199810362097189432, 0.002933080482796252431, 0.004399620724194360649, 0.005866160965592469301, 0.007332701206990578820, 0.008065971327689634013, 0.008799241448388690073, 0.009532511569087746134, 0.01026578168978680046, 0.01173232193118494901, 0.01319886217258310103, 0.01466540241398124958, 0.01539867253468032472, 0.01613194265537939986, 0.01759848289677755015, 0.01906502313817570043, 0.01979829325887477384, 0.02053156337957384725, 0.02199810362097200794, 0.02346464386237016517 ),
 .UNSPECIFIED. ) ;
#53445=CARTESIAN_POINT ( 'NONE',  ( -143.8794621588508846, 59.54894433207191184, 6.412744670210712705 ) ) ;
#53451=CARTESIAN_POINT ( 'NONE',  ( -144.2038301586456157, 61.09856042007388766, 32.89561146611724496 ) ) ;
#53452=CARTESIAN_POINT ( 'NONE',  ( 62.04664474957769471, 12.44961624115900634, 71.61029269029653221 ) ) ;
#53462=VECTOR ( 'NONE', #16761, 1000.000000000000000 ) ;
#53463=DIRECTION ( 'NONE',  ( -0.000000000000000000, 1.000000000000000000, -0.000000000000000000 ) ) ;
#53464=DIRECTION ( 'NONE',  ( -0.000000000000000000, 1.000000000000000000, -0.000000000000000000 ) ) ;
#53465=CARTESIAN_POINT ( 'NONE',  ( 67.56108154898467433, 13.77276756375644595, 43.29870974333168476 ) ) ;
#53466=CARTESIAN_POINT ( 'NONE',  ( 16.45324200325260122, 7.529580975261485065, 83.72611423296160638 ) ) ;
#53471=CARTESIAN_POINT ( 'NONE',  ( -95.50384525802327573, 29.46973564057716644, 68.08823763800167228 ) ) ;
#53472=ORIENTED_EDGE ( 'NONE', *, *, #52303, .F. ) ;
#53473=CARTESIAN_POINT ( 'NONE',  ( -71.16584859396995455, 19.60484997908767824, 38.15316589600989516 ) ) ;
#53476=B_SPLINE_CURVE_WITH_KNOTS ( 'NONE', 3,
 ( #44944, #12953, #18220, #46936, #67123, #52553, #42003, #12596, #68397, #36385, #28777, #18915, #29120, #14915, #9300, #41658, #34753, #13297, #50227, #30766, #61125, #55856, #2390, #50920, #2734, #18563, #41320, #40016, #56189, #20202, #61478, #14579, #8006, #57495, #25500, #63116, #5052, #47954, #27542, #43370, #58858, #59541, #69421, #37068 ),
 .UNSPECIFIED., .F., .F.,
 ( 4, 2, 2, 2, 2, 2, 2, 2, 2, 2, 2, 2, 2, 2, 2, 2, 2, 2, 2, 2, 2, 4 ),
 ( 0.000000000000000000, 0.001473754749730452713, 0.002210632124595686334, 0.002947509499460920172, 0.004421264249191396087, 0.005895018998921872436, 0.007368773748652348785, 0.008105651123517581755, 0.008842528498382814725, 0.01031628324811327893, 0.01179003799784374487, 0.01252691537270897611, 0.01326379274757420734, 0.01473754749730467328, 0.01547442487216991840, 0.01621130224703516004, 0.01768505699676564333, 0.01915881174649612662, 0.01989568912136136999, 0.02063256649622660990, 0.02210632124595708972, 0.02358007599568756954 ),
 .UNSPECIFIED. ) ;
#53478=CARTESIAN_POINT ( 'NONE',  ( -125.8938041572051389, 47.69968343338780414, 18.77539728269342945 ) ) ;
#53479=CARTESIAN_POINT ( 'NONE',  ( -174.7869898116916545, 88.99756909636811031, 72.52766040328414476 ) ) ;
#53480=B_SPLINE_CURVE_WITH_KNOTS ( 'NONE', 3,
 ( #16996, #64855, #53927, #16314, #37770, #21249, #59905, #11726, #32496, #21933, #42360, #38465, #10680, #15969, #32157, #837, #59555, #63819, #33198, #54636, #48642, #27207, #42698, #15631, #485, #11372, #47621, #64155, #22286, #59214, #43385, #5750, #53239, #129, #43033, #16656, #43725, #47967, #65201, #26185, #69072, #37081, #20908, #58523, #38111 ),
 .UNSPECIFIED., .F., .F.,
 ( 4, 2, 2, 1, 2, 2, 2, 2, 2, 2, 2, 2, 2, 2, 2, 2, 2, 2, 2, 2, 2, 2, 4 ),
 ( 0.02346464386237014782, 0.02493212228186625357, 0.02566586149161430644, 0.02639960070136235584, 0.02713333991111040872, 0.02786707912085845812, 0.02933455754035455346, 0.03006829675010259939, 0.03080203595985064879, 0.03226951437934675454, 0.03300325358909480394, 0.03373699279884285335, 0.03520447121833895909, 0.03667194963783507178, 0.03740568884758313506, 0.03813942805733119140, 0.03960690647682731103, 0.04107438489632342371, 0.04254186331581955027, 0.04327560252556761355, 0.04400934173531566990, 0.04547682015481180340, 0.04694429857430792302 ),
 .UNSPECIFIED. ) ;
#53482=CARTESIAN_POINT ( 'NONE',  ( 21.75684465274323998, 6.764994602232764720, 15.23809131227820046 ) ) ;
#53484=ADVANCED_FACE ( 'NONE', ( #61764 ), #51228, .F. ) ;
#53487=CARTESIAN_POINT ( 'NONE',  ( 70.26936813788618963, 15.51386666370915535, 35.34273349493187766 ) ) ;
#53491=DIRECTION ( 'NONE',  ( -0.000000000000000000, 1.000000000000000000, -0.000000000000000000 ) ) ;
#53492=CARTESIAN_POINT ( 'NONE',  ( 140.7888851157410102, 46.97220912571251006, -67.49339367180394333 ) ) ;
#53493=CARTESIAN_POINT ( 'NONE',  ( -145.3233446620409666, 62.00659513626050767, -62.91606084811092359 ) ) ;
#53494=ORIENTED_EDGE ( 'NONE', *, *, #48484, .T. ) ;
#53496=FACE_BOUND ( 'NONE', #26521, .T. ) ;
#53503=CARTESIAN_POINT ( 'NONE',  ( -155.1302201283145337, 69.09929365814129198, 16.34568025258033330 ) ) ;
#53504=CARTESIAN_POINT ( 'NONE',  ( -122.8011284400168392, 45.68452922414297035, -76.10641211455910593 ) ) ;
#53507=CARTESIAN_POINT ( 'NONE',  ( 45.45802413036135903, 10.29289344693338393, -92.36508079978824526 ) ) ;
#53510=CARTESIAN_POINT ( 'NONE',  ( -38.87871322265799279, 11.95691939779334412, 11.85322953461970741 ) ) ;
#53511=ORIENTED_EDGE ( 'NONE', *, *, #34494, .F. ) ;
#53515=DIRECTION ( 'NONE',  ( -0.000000000000000000, 1.000000000000000000, -0.000000000000000000 ) ) ;
#53517=LINE ( 'NONE', #38750, #29014 ) ;
#53518=CARTESIAN_POINT ( 'NONE',  ( 63.98971758354224448, 12.90030016320050876, -8.923645871160223564 ) ) ;
#53519=CARTESIAN_POINT ( 'NONE',  ( 141.0792860804899362, 47.16255757051796138, -45.61442408848115093 ) ) ;
#53521=CARTESIAN_POINT ( 'NONE',  ( -51.34562532494748410, 14.75613283840036871, -63.02301684657460612 ) ) ;
#53522=FACE_OUTER_BOUND ( 'NONE', #41228, .T. ) ;
#53525=ORIENTED_EDGE ( 'NONE', *, *, #6413, .T. ) ;
#53529=CARTESIAN_POINT ( 'NONE',  ( 175.7684093698864558, 74.78503214758480055, 85.16604023312240201 ) ) ;
#53536=CARTESIAN_POINT ( 'NONE',  ( -15.32550079334879456, 7.496023944924842475, 64.21821511530063731 ) ) ;
#53537=CARTESIAN_POINT ( 'NONE',  ( 211.8382652195006699, 118.5282575235989952, 12.17967590094709074 ) ) ;
#53540=CARTESIAN_POINT ( 'NONE',  ( 207.8484262634767958, 110.7633525054914543, -23.80039066132988523 ) ) ;
#53542=B_SPLINE_CURVE_WITH_KNOTS ( 'NONE', 3,
 ( #47071, #41113, #68535, #5202, #69213, #58311, #31585, #63261, #31258, #15067, #21037, #20338, #66911, #41463, #36524, #15415, #53025, #10129, #3823, #52685, #36873, #25291, #62916, #4852, #9795, #68860, #57980, #14388, #53367, #35840, #31940, #4511, #46728, #25974, #26318, #45431, #57292, #47404, #42486, #9105, #14717, #36180, #9448, #52355 ),
 .UNSPECIFIED., .F., .F.,
 ( 4, 2, 2, 2, 2, 2, 2, 2, 2, 2, 2, 2, 2, 2, 2, 2, 2, 2, 2, 2, 2, 4 ),
 ( 0.02895403260893138903, 0.03071603688922224656, 0.03247804116951310410, 0.03424004544980396164, 0.03600204973009481918, 0.03776405401038567672, 0.03864505615053111937, 0.03952605829067656201, 0.04040706043082200466, 0.04128806257096744731, 0.04216906471111288995, 0.04305006685125833260, 0.04393106899140377525, 0.04481207113154921096, 0.04569307327169465360, 0.04657407541184009625, 0.04745507755198553890, 0.04833607969213098154, 0.05009808397242186684, 0.05186008825271275213, 0.05362209253300363743, 0.05714610109358543577 ),
 .UNSPECIFIED. ) ;
#53543=CARTESIAN_POINT ( 'NONE',  ( 164.8914542114683570, 64.97670918603526502, 62.63277694328278500 ) ) ;
#53545=CARTESIAN_POINT ( 'NONE',  ( 63.01563776193091826, -170.0000000000000000, -96.90979201309711755 ) ) ;
#53549=CARTESIAN_POINT ( 'NONE',  ( 154.6667526376337491, 55.50347409140648836, 17.02485824898109001 ) ) ;
#53551=EDGE_CURVE ( 'NONE', #47781, #52360, #22757, .T. ) ;
#53558=CARTESIAN_POINT ( 'NONE',  ( 32.71619935235103327, 8.645270090896708837, 87.68833691130073760 ) ) ;
#53564=CARTESIAN_POINT ( 'NONE',  ( -4.506365319453811580, 7.705038994660874607, 4.040912142253615613 ) ) ;
#53565=CARTESIAN_POINT ( 'NONE',  ( 174.1422537179814753, 73.24254491731255712, -46.57861427890096451 ) ) ;
#53567=CARTESIAN_POINT ( 'NONE',  ( 163.0608430180613198, 62.13093644261793003, 85.55641011433075960 ) ) ;
#53572=CARTESIAN_POINT ( 'NONE',  ( -53.14657859411973817, 15.21831473227210552, -35.45855742538594768 ) ) ;
#53575=CARTESIAN_POINT ( 'NONE',  ( 12.47451846520756646, 7.423604437114564192, 30.78201781477134702 ) ) ;
#53580=EDGE_CURVE ( 'NONE', #35602, #17986, #4336, .T. ) ;
#53582=CARTESIAN_POINT ( 'NONE',  ( 113.8724110608469147, 31.71510301790680941, -76.84776400044430034 ) ) ;
#53583=CARTESIAN_POINT ( 'NONE',  ( -165.9827517816028717, 80.96014358007563771, 94.34005317371386923 ) ) ;
#53584=CYLINDRICAL_SURFACE ( 'NONE', #50233, 7.500000000000013323 ) ;
#53585=FACE_OUTER_BOUND ( 'NONE', #38513, .T. ) ;
#53589=CARTESIAN_POINT ( 'NONE',  ( 22.80839748737789208, 6.826915557457465589, -18.82546783934041201 ) ) ;
#53592=EDGE_LOOP ( 'NONE', ( #35971, #41903 ) ) ;
#53593=ORIENTED_EDGE ( 'NONE', *, *, #18453, .F. ) ;
#53595=CARTESIAN_POINT ( 'NONE',  ( 66.73467315386238852, 14.60276727483218906, -9.845064874592072357 ) ) ;
#53596=CARTESIAN_POINT ( 'NONE',  ( -83.15209219203883606, 25.16621997697722790, -36.58508197384574601 ) ) ;
#53598=CARTESIAN_POINT ( 'NONE',  ( -156.0204364459165163, 71.27041535366187475, 15.10448288493537738 ) ) ;
#53600=EDGE_CURVE ( 'NONE', #34095, #3682, #58876, .T. ) ;
#53604=CARTESIAN_POINT ( 'NONE',  ( 20.37135563017390893, 6.690359945346062709, 43.47186685453966959 ) ) ;
#53605=CARTESIAN_POINT ( 'NONE',  ( -150.9451284960939006, 66.73881725783795105, 84.54405725442943265 ) ) ;
#53607=ORIENTED_EDGE ( 'NONE', *, *, #54911, .F. ) ;
#53608=ORIENTED_EDGE ( 'NONE', *, *, #46121, .F. ) ;
#53610=CARTESIAN_POINT ( 'NONE',  ( -155.5977325361977819, 70.88311713755696530, -11.08395381880265518 ) ) ;
#53611=CARTESIAN_POINT ( 'NONE',  ( 38.42095780754793566, 9.297684251045554404, -35.66794142809995805 ) ) ;
#53613=CARTESIAN_POINT ( 'NONE',  ( -38.26732153931116898, 10.81230693396213205, 61.44875431616114270 ) ) ;
#53614=CARTESIAN_POINT ( 'NONE',  ( 197.6329787101074089, 98.74106466892202150, 61.01638013965135343 ) ) ;
#53615=ORIENTED_EDGE ( 'NONE', *, *, #13111, .T. ) ;
#53617=CARTESIAN_POINT ( 'NONE',  ( 188.0103583326377930, 87.39896620268127947, 66.54395642386660370 ) ) ;
#53618=CARTESIAN_POINT ( 'NONE',  ( -154.0775378574014098, 68.15437918458557931, 71.03131665102951331 ) ) ;
#53620=CARTESIAN_POINT ( 'NONE',  ( 19.54452863209719737, 7.657034792877148277, 17.18020211478049220 ) ) ;
#53623=CARTESIAN_POINT ( 'NONE',  ( -86.15275984831843914, 25.31588180512565600, -42.09545882965587538 ) ) ;
#53624=CARTESIAN_POINT ( 'NONE',  ( 22.30016284075436772, 6.796348835713780012, 68.11227918755604094 ) ) ;
#53625=CARTESIAN_POINT ( 'NONE',  ( -149.5074843970971017, 64.17983161892347255, -7.968279941028269420 ) ) ;
#53626=CARTESIAN_POINT ( 'NONE',  ( 10.13846145460683523, 6.385368868491637429, -64.90677605932107497 ) ) ;
#53627=AXIS2_PLACEMENT_3D ( 'NONE', #44705, #62532, #39092 ) ;
#53631=CARTESIAN_POINT ( 'NONE',  ( -31.43908319763710679, -170.0000000000000000, 72.06100499665289760 ) ) ;
#53633=CARTESIAN_POINT ( 'NONE',  ( 46.90141780929663895, 9.503798448769781970, -70.46900398398989296 ) ) ;
#53634=CARTESIAN_POINT ( 'NONE',  ( 61.33840119549014958, 13.32121602003046235, -77.37933350821008105 ) ) ;
#53640=EDGE_LOOP ( 'NONE', ( #35400, #4025, #60885, #7393 ) ) ;
#53642=ORIENTED_EDGE ( 'NONE', *, *, #48557, .T. ) ;
#53643=CYLINDRICAL_SURFACE ( 'NONE', #50426, 7.500000000000013323 ) ;
#53644=ORIENTED_EDGE ( 'NONE', *, *, #62368, .T. ) ;
#53645=CARTESIAN_POINT ( 'NONE',  ( 110.7167338301703836, 30.21148223254618159, 71.45576479620105204 ) ) ;
#53647=CARTESIAN_POINT ( 'NONE',  ( 136.1037846510192821, 43.98155406734452555, 71.02523018034077040 ) ) ;
#53649=CARTESIAN_POINT ( 'NONE',  ( 81.37856278600284554, 17.69577192910746888, -91.65141974325806018 ) ) ;
#53651=DIRECTION ( 'NONE',  ( 0.000000000000000000, 0.000000000000000000, 1.000000000000000000 ) ) ;
#53652=AXIS2_PLACEMENT_3D ( 'NONE', #17853, #29106, #66061 ) ;
#53657=CARTESIAN_POINT ( 'NONE',  ( -125.8938041572051105, 46.49392987655492959, -23.06915330777029638 ) ) ;
#53659=CARTESIAN_POINT ( 'NONE',  ( -147.7895256390024485, 64.04409735547010030, -34.95785904615254225 ) ) ;
#53662=CARTESIAN_POINT ( 'NONE',  ( -165.6404838346738870, 80.60836113891890875, -68.43868871235946472 ) ) ;
#53663=CARTESIAN_POINT ( 'NONE',  ( -142.2626321327577728, 58.26997216742664421, -44.27203299751281662 ) ) ;
#53665=CARTESIAN_POINT ( 'NONE',  ( 57.07246224906425169, 12.39953617563782906, 15.06960304992271560 ) ) ;
#53668=ORIENTED_EDGE ( 'NONE', *, *, #26828, .F. ) ;
#53669=CARTESIAN_POINT ( 'NONE',  ( 55.50974873964668888, 12.08212941291357012, 90.84068197934951172 ) ) ;
#53671=CARTESIAN_POINT ( 'NONE',  ( 134.7697261969508986, 41.97802808873667146, -24.13692694190012489 ) ) ;
#53673=CARTESIAN_POINT ( 'NONE',  ( 91.49345572560149265, 21.13836538408681065, -75.88006259688719979 ) ) ;
#53674=CARTESIAN_POINT ( 'NONE',  ( 58.14386731224344373, 11.59506827749133429, -91.19280277787788691 ) ) ;
#53676=CARTESIAN_POINT ( 'NONE',  ( -94.79166046756729713, 29.13671350128077364, -68.86817510426273259 ) ) ;
#53678=EDGE_LOOP ( 'NONE', ( #16792, #42665 ) ) ;
#53680=CARTESIAN_POINT ( 'NONE',  ( 188.4904153916305063, 86.42965364612517476, -71.78902575509843587 ) ) ;
#53683=DIRECTION ( 'NONE',  ( -0.000000000000000000, 1.000000000000000000, -0.000000000000000000 ) ) ;
#53684=EDGE_CURVE ( 'NONE', #31812, #68783, #24534, .T. ) ;
#53686=CARTESIAN_POINT ( 'NONE',  ( 107.0555969502564011, 28.53646637607230119, -77.07238525624649128 ) ) ;
#53687=CARTESIAN_POINT ( 'NONE',  ( 79.11678589158262298, 16.99307320450158443, 37.22067676483509757 ) ) ;
#53689=CARTESIAN_POINT ( 'NONE',  ( 45.89268866913129585, 10.36133864615982958, -39.35403686315040517 ) ) ;
#53690=CARTESIAN_POINT ( 'NONE',  ( 205.5105258529713410, 107.4632495673648549, 71.01916293991351381 ) ) ;
#53692=CARTESIAN_POINT ( 'NONE',  ( -105.8768181937898873, 34.64545164169049229, -9.071693415820034190 ) ) ;
#53693=VERTEX_POINT ( 'NONE', #52517 ) ;
#53694=CARTESIAN_POINT ( 'NONE',  ( -10.46803069297986077, 7.077485182625207649, -35.89476353789692809 ) ) ;
#53695=CARTESIAN_POINT ( 'NONE',  ( -85.30133330826032534, 24.96073847331896189, 88.09538619317125097 ) ) ;
#53696=CARTESIAN_POINT ( 'NONE',  ( 92.52113039222220436, 22.58921125235802307, 68.72354153264095089 ) ) ;
#53697=CARTESIAN_POINT ( 'NONE',  ( 154.4550750032602195, 55.34393534448155805, -9.908619237073862607 ) ) ;
#53698=CARTESIAN_POINT ( 'NONE',  ( 32.30062460741316244, 8.603096374765344834, 8.143925628932546346 ) ) ;
#53699=CARTESIAN_POINT ( 'NONE',  ( -95.88693721180811735, 30.76307528361165922, -65.42962194985348390 ) ) ;
#53702=CARTESIAN_POINT ( 'NONE',  ( 211.0199171616895342, 115.4353716546810205, 94.44800888915801806 ) ) ;
#53708=CARTESIAN_POINT ( 'NONE',  ( 46.90208227351340753, 10.52324439420451441, -70.20627750463229688 ) ) ;
#53710=CARTESIAN_POINT ( 'NONE',  ( -104.1244073710069671, 33.72720758483609416, -62.07464707146255023 ) ) ;
#53712=CARTESIAN_POINT ( 'NONE',  ( 86.01230605172118260, 20.27366317264618800, 83.41941906375110705 ) ) ;
#53717=CARTESIAN_POINT ( 'NONE',  ( -130.2196570250629009, 49.40815211106349381, 5.130512497953152895 ) ) ;
#53718=CARTESIAN_POINT ( 'NONE',  ( -107.0809603157386505, 36.42942792191063717, 70.64629373282132008 ) ) ;
#53721=CARTESIAN_POINT ( 'NONE',  ( -126.8016613879753294, 48.30316697011514293, -34.95518786917430987 ) ) ;
#53722=ORIENTED_EDGE ( 'NONE', *, *, #22475, .T. ) ;
#53724=CARTESIAN_POINT ( 'NONE',  ( 89.88695630745282017, 20.55793566325393940, 70.82916094545055330 ) ) ;
#53725=CARTESIAN_POINT ( 'NONE',  ( -145.1840176520338161, 60.59722987250436432, 85.77424136295870483 ) ) ;
#53727=CARTESIAN_POINT ( 'NONE',  ( 141.2894128405439176, 46.09731134920846074, 38.04785505188484507 ) ) ;
#53728=ORIENTED_EDGE ( 'NONE', *, *, #50914, .F. ) ;
#53730=CARTESIAN_POINT ( 'NONE',  ( 81.74250361646204510, 18.86685472882136949, 16.07802836438051486 ) ) ;
#53731=CARTESIAN_POINT ( 'NONE',  ( 160.9099843287284557, 61.67000084894968381, 3.384304814524660365 ) ) ;
#53732=DIRECTION ( 'NONE',  ( -0.000000000000000000, 1.000000000000000000, -0.000000000000000000 ) ) ;
#53737=CARTESIAN_POINT ( 'NONE',  ( -73.10694748374054086, 20.28107308417882493, -20.82856601646535566 ) ) ;
#53738=CARTESIAN_POINT ( 'NONE',  ( 70.46452034227868921, 14.52462608639674535, -71.07036406642562554 ) ) ;
#53741=CARTESIAN_POINT ( 'NONE',  ( 153.8224167330182297, 56.12711234192240539, 16.62213432411530789 ) ) ;
#53742=VERTEX_POINT ( 'NONE', #4343 ) ;
#53743=CARTESIAN_POINT ( 'NONE',  ( 164.0298848570287191, 62.93631132702878972, 40.58462181814118708 ) ) ;
#53744=CARTESIAN_POINT ( 'NONE',  ( 32.12337157895397866, 8.585320123189577046, -95.00000000000133582 ) ) ;
#53748=CARTESIAN_POINT ( 'NONE',  ( 174.1361937581588677, 73.23677172949255976, -94.55001106689485368 ) ) ;
#53749=CARTESIAN_POINT ( 'NONE',  ( 139.1353280997809350, 44.70436000187870462, 69.18824476712693183 ) ) ;
#53751=CARTESIAN_POINT ( 'NONE',  ( 132.0563630623056497, 41.51825634609594573, 56.57050957695005877 ) ) ;
#53752=EDGE_LOOP ( 'NONE', ( #65273, #51105 ) ) ;
#53758=CARTESIAN_POINT ( 'NONE',  ( -107.2385267828037456, 36.51474259889399576, 5.542223241171852166 ) ) ;
#53761=CARTESIAN_POINT ( 'NONE',  ( -109.7362175185300543, 36.73266838575884208, 90.83257743108923421 ) ) ;
#53765=DIRECTION ( 'NONE',  ( -0.000000000000000000, 1.000000000000000000, -0.000000000000000000 ) ) ;
#53770=CARTESIAN_POINT ( 'NONE',  ( 210.6741002223296846, 114.9147155784838503, -66.13167200068693319 ) ) ;
#53773=CARTESIAN_POINT ( 'NONE',  ( -33.74415167774779434, 9.981065646265545155, -89.36609339537675112 ) ) ;
#53774=CARTESIAN_POINT ( 'NONE',  ( 18.20314211955701822, 7.596739727129572906, 30.39710523511859108 ) ) ;
#53775=CARTESIAN_POINT ( 'NONE',  ( 197.2367704513663966, 96.64129968056330711, 91.28287337347603625 ) ) ;
#53776=CYLINDRICAL_SURFACE ( 'NONE', #69209, 7.500000000000013323 ) ;
#53778=DIRECTION ( 'NONE',  ( -0.000000000000000000, 1.000000000000000000, -0.000000000000000000 ) ) ;
#53782=CARTESIAN_POINT ( 'NONE',  ( -30.95341298663138829, 10.53108683215057795, -77.16174795566554678 ) ) ;
#53783=CARTESIAN_POINT ( 'NONE',  ( 57.39083379741710900, 11.43779987330584369, -48.20640899083532105 ) ) ;
#53784=LINE ( 'NONE', #48848, #64236 ) ;
#53785=CARTESIAN_POINT ( 'NONE',  ( -146.5341851369306596, 61.69744206542952014, 4.476676838031795391 ) ) ;
#53792=CARTESIAN_POINT ( 'NONE',  ( 38.91512155099543691, 9.360679678889624711, -23.77526687496408897 ) ) ;
#53795=FACE_OUTER_BOUND ( 'NONE', #20774, .T. ) ;
#53799=EDGE_CURVE ( 'NONE', #65633, #66303, #13550, .T. ) ;
#53804=CARTESIAN_POINT ( 'NONE',  ( -156.3413281584584809, -170.0000000000000000, 94.99999999999866418 ) ) ;
#53807=CARTESIAN_POINT ( 'NONE',  ( 69.74037587279242700, 14.33355757956376131, 40.67087411745646364 ) ) ;
#53808=CARTESIAN_POINT ( 'NONE',  ( 9.120338347441469651, 7.384947993289908474, 87.75479786978895902 ) ) ;
#53810=B_SPLINE_CURVE_WITH_KNOTS ( 'NONE', 3,
 ( #11383, #39190, #55346, #17007, #7172, #28627, #23364, #38840, #39527, #48657, #43397, #16671, #32853, #33215, #6475, #54288, #6110, #27569, #49011, #849, #22301, #43738, #1195, #45142, #62012, #28986, #50432, #3288, #67654, #30362, #35645, #14185, #8912, #18769, #51814, #46181, #66975, #66621 ),
 .UNSPECIFIED., .F., .F.,
 ( 4, 2, 2, 2, 2, 2, 2, 2, 2, 2, 2, 2, 2, 2, 2, 2, 2, 2, 4 ),
 ( 1.589900327696125378E-17, 0.001559859933532243290, 0.003119719867064470967, 0.004679579800596697994, 0.006239439734128925455, 0.007799299667661153783, 0.008579229634427268381, 0.009359159601193383846, 0.01091901953472561304, 0.01169894950149172504, 0.01247887946825783877, 0.01403873940179006276, 0.01559859933532228848, 0.01715845926885451248, 0.01871831920238673300, 0.02027817913591895352, 0.02183803906945117751, 0.02339789900298339803, 0.02495775893651561855 ),
 .UNSPECIFIED. ) ;
#53811=ORIENTED_EDGE ( 'NONE', *, *, #52782, .F. ) ;
#53813=CARTESIAN_POINT ( 'NONE',  ( -78.66644367742111399, -170.0000000000000000, -96.30455181264525777 ) ) ;
#53815=CARTESIAN_POINT ( 'NONE',  ( -75.01314391403411719, 20.96328762434824711, 31.35011065199344671 ) ) ;
#53820=CARTESIAN_POINT ( 'NONE',  ( -122.3759299995709426, 45.41285412136510047, 4.634680028069846358 ) ) ;
#53821=VECTOR ( 'NONE', #56904, 1000.000000000000000 ) ;
#53822=CARTESIAN_POINT ( 'NONE',  ( -173.1211646369891071, 87.12891641440857882, 57.66624519710472185 ) ) ;
#53823=CARTESIAN_POINT ( 'NONE',  ( 126.8947007444828614, 37.37669340849690514, 61.05352645786824439 ) ) ;
#53826=CARTESIAN_POINT ( 'NONE',  ( 150.8925291903903769, 52.71218673668931842, 33.26698628395256918 ) ) ;
#53827=DIRECTION ( 'NONE',  ( -0.000000000000000000, 1.000000000000000000, -0.000000000000000000 ) ) ;
#53832=CARTESIAN_POINT ( 'NONE',  ( -24.93568128341083678, 8.613819379861711312, 41.48431949557672027 ) ) ;
#53836=FACE_BOUND ( 'NONE', #26177, .T. ) ;
#53837=CARTESIAN_POINT ( 'NONE',  ( -1.876547441458565668, 6.576559737910140591, -74.33668192632359251 ) ) ;
#53838=CARTESIAN_POINT ( 'NONE',  ( -180.3114074031035727, 97.09758726817783270, 63.01175798389278526 ) ) ;
#53840=CARTESIAN_POINT ( 'NONE',  ( -121.1841775822197604, 44.65790002524552449, -48.27118250510603303 ) ) ;
#53843=ADVANCED_FACE ( 'NONE', ( #33146 ), #42979, .F. ) ;
#53847=CARTESIAN_POINT ( 'NONE',  ( -84.55783695959762269, 25.74181993349143838, 69.43046075343895041 ) ) ;
#53848=CARTESIAN_POINT ( 'NONE',  ( 87.58754341703161117, 20.81465688423122984, -9.023248056753891078 ) ) ;
#53850=CARTESIAN_POINT ( 'NONE',  ( -35.17718245314463132, 11.25729435722178629, 17.37854247445588740 ) ) ;
#53855=CARTESIAN_POINT ( 'NONE',  ( 17.73567516211396367, 7.577454475141604640, -77.12280871073899391 ) ) ;
#53856=CARTESIAN_POINT ( 'NONE',  ( 102.7603480884046405, 26.66430664428465036, 91.41953138856987948 ) ) ;
#53857=CARTESIAN_POINT ( 'NONE',  ( -149.5074843970971017, 65.50121172469319220, 57.56537183036274286 ) ) ;
#53858=CARTESIAN_POINT ( 'NONE',  ( 68.61679388097593346, 14.04192738700837495, -21.36990119259161958 ) ) ;
#53860=CARTESIAN_POINT ( 'NONE',  ( -25.79929641484369540, 9.749255553662436569, -47.78593713492852402 ) ) ;
#53861=CARTESIAN_POINT ( 'NONE',  ( -47.79955240516189008, 13.88975739862079806, -71.53314426491067479 ) ) ;
#53862=CARTESIAN_POINT ( 'NONE',  ( -71.36019764570897905, 20.73631042140123171, -94.55033525794866023 ) ) ;
#53864=VERTEX_POINT ( 'NONE', #16260 ) ;
#53867=CARTESIAN_POINT ( 'NONE',  ( -168.7314919967218145, 83.83749564070832605, 71.26571717153785812 ) ) ;
#53868=CARTESIAN_POINT ( 'NONE',  ( 126.9799862522376372, 38.57834705404714271, -94.18946796078350303 ) ) ;
#53875=CARTESIAN_POINT ( 'NONE',  ( 186.2680729609084551, 85.48839327635670315, -22.32090202264587120 ) ) ;
#53876=CARTESIAN_POINT ( 'NONE',  ( 207.4566510040494336, 111.9649643341356438, 2.885941162796656911 ) ) ;
#53878=CARTESIAN_POINT ( 'NONE',  ( 43.14712943604300222, 8.926114770663666320, -9.772680129153844319 ) ) ;
#53879=DIRECTION ( 'NONE',  ( 0.000000000000000000, 0.000000000000000000, 1.000000000000000000 ) ) ;
#53886=CARTESIAN_POINT ( 'NONE',  ( 93.43270425363542131, 22.93046121381056679, -46.48805702006733753 ) ) ;
#53890=CARTESIAN_POINT ( 'NONE',  ( 153.2384531768736338, 54.43344429203622781, 16.27428681065648775 ) ) ;
#53892=CYLINDRICAL_SURFACE ( 'NONE', #64784, 7.500000000000013323 ) ;
#53894=CARTESIAN_POINT ( 'NONE',  ( 61.10129719786243641, 12.23677173834304988, 17.72406295025428946 ) ) ;
#53895=CARTESIAN_POINT ( 'NONE',  ( -59.57733000654213384, 15.94108165424593437, 58.66074221055215077 ) ) ;
#53897=ORIENTED_EDGE ( 'NONE', *, *, #138, .F. ) ;
#53898=CARTESIAN_POINT ( 'NONE',  ( 46.09329439034695497, 10.39313452975435048, 87.69915135060715272 ) ) ;
#53900=CARTESIAN_POINT ( 'NONE',  ( 105.4193882736795871, 26.71329717705294726, 31.34684377997668747 ) ) ;
#53904=CARTESIAN_POINT ( 'NONE',  ( -59.95707852844800811, 16.05120821151901467, -75.25667932634594592 ) ) ;
#53905=CARTESIAN_POINT ( 'NONE',  ( 32.67604581760324578, 7.629767527669975458, -12.94769449661993121 ) ) ;
#53906=CARTESIAN_POINT ( 'NONE',  ( 177.7964363391244831, 76.75162026635257462, -50.48114945074676996 ) ) ;
#53907=VECTOR ( 'NONE', #24183, 1000.000000000000000 ) ;
#53911=CARTESIAN_POINT ( 'NONE',  ( -51.77431913897918037, 14.86466849149171310, -35.95328652352582566 ) ) ;
#53913=CARTESIAN_POINT ( 'NONE',  ( 11.81843724556921238, 7.412394300769733491, 43.88267239520089902 ) ) ;
#53917=CARTESIAN_POINT ( 'NONE',  ( -48.41612563322100016, 13.00196567016870297, 94.99999999999866418 ) ) ;
#53922=CARTESIAN_POINT ( 'NONE',  ( -8.320652113663527416, 6.923290556636831461, -8.573520141480127421 ) ) ;
#53923=CARTESIAN_POINT ( 'NONE',  ( -172.2883581164155657, 87.70586714890205826, 84.53995063412840238 ) ) ;
#53926=CARTESIAN_POINT ( 'NONE',  ( -38.87871322265797858, 11.95691939779334234, 65.54233071554708090 ) ) ;
#53927=CARTESIAN_POINT ( 'NONE',  ( -8.800520192024524846, 7.964629484975262130, -23.52613853675388711 ) ) ;
#53929=CARTESIAN_POINT ( 'NONE',  ( 21.42484406671929520, 6.746536496442162800, -21.12818067883022266 ) ) ;
#53936=CARTESIAN_POINT ( 'NONE',  ( 117.7510095710447615, 32.51306356638684036, 90.73932576073276834 ) ) ;
#53938=CARTESIAN_POINT ( 'NONE',  ( -156.9262190792699130, 72.10659547035875505, 12.51482676534390848 ) ) ;
#53940=CARTESIAN_POINT ( 'NONE',  ( 21.88606409348644277, 6.772455198693822176, 33.14124745247766413 ) ) ;
#53941=CARTESIAN_POINT ( 'NONE',  ( -150.6785516065348531, 66.50778382752601203, 84.49707106786556210 ) ) ;
#53948=CARTESIAN_POINT ( 'NONE',  ( 198.4045886930829852, 99.71425793793713410, 59.46347056621107896 ) ) ;
#53953=CARTESIAN_POINT ( 'NONE',  ( 103.5839822277949622, 25.92130892112108143, 13.72661071236549724 ) ) ;
#53956=CARTESIAN_POINT ( 'NONE',  ( 21.73827885904430346, 6.764046335627706519, 59.78669074769747027 ) ) ;
#53958=CARTESIAN_POINT ( 'NONE',  ( 11.82322073186612421, 6.406156243758798219, -76.23436747048188522 ) ) ;
#53959=EDGE_CURVE ( 'NONE', #59320, #42164, #40072, .T. ) ;
#53964=CARTESIAN_POINT ( 'NONE',  ( 177.7960900018544805, 75.34533826015461955, 43.55310789600767407 ) ) ;
#53965=CARTESIAN_POINT ( 'NONE',  ( -132.8123438040340147, 51.22132183644642822, -39.50633901085532074 ) ) ;
#53968=EDGE_LOOP ( 'NONE', ( #56937, #15344 ) ) ;
#53973=CARTESIAN_POINT ( 'NONE',  ( 197.8598785550297237, 99.02620879292952338, 6.767166655171187095 ) ) ;
#53976=ORIENTED_EDGE ( 'NONE', *, *, #1502, .T. ) ;
#53977=CARTESIAN_POINT ( 'NONE',  ( 185.5412249395995730, 84.70425786165998261, 30.77240809119399145 ) ) ;
#53981=CARTESIAN_POINT ( 'NONE',  ( 110.2429982417149432, 29.99119854320844070, 71.45576479620103783 ) ) ;
#53982=CARTESIAN_POINT ( 'NONE',  ( 103.3187396002585672, 26.90210317967632747, -94.19991905147882960 ) ) ;
#53983=CARTESIAN_POINT ( 'NONE',  ( 137.5911612413395062, 44.91497189902065656, 70.36324336602153551 ) ) ;
#53984=CARTESIAN_POINT ( 'NONE',  ( -71.21970990337017327, 19.62334883444993494, -43.64161293005157916 ) ) ;
#53986=CARTESIAN_POINT ( 'NONE',  ( -101.3492134984965105, 32.31003911421601060, 45.47588113239901020 ) ) ;
#53987=CARTESIAN_POINT ( 'NONE',  ( 94.07616572255074061, 22.09777530676769430, -44.34594446716025828 ) ) ;
#53991=CARTESIAN_POINT ( 'NONE',  ( -7.825402957745087207, 6.891034867348159842, 71.96013162991091860 ) ) ;
#53992=CARTESIAN_POINT ( 'NONE',  ( 157.4703587214989113, 58.92748579479260229, -9.279633708673953763 ) ) ;
#53993=CARTESIAN_POINT ( 'NONE',  ( -142.0084862216822614, 59.34995487985345619, -41.73440649756038567 ) ) ;
#53994=CARTESIAN_POINT ( 'NONE',  ( -171.4943428135323131, 86.82484920477510570, -61.68648179989266822 ) ) ;
#53995=CARTESIAN_POINT ( 'NONE',  ( -142.5211356634642073, 58.47296527616907014, -45.05442505613748949 ) ) ;
#53997=CARTESIAN_POINT ( 'NONE',  ( 55.77012379229942240, 12.13428856597100491, 12.42136026870828047 ) ) ;
#54000=DIRECTION ( 'NONE',  ( -0.000000000000000000, 1.000000000000000000, -0.000000000000000000 ) ) ;
#54002=CARTESIAN_POINT ( 'NONE',  ( 79.38459371357852490, 17.07499996355400995, -14.47219513322666273 ) ) ;
#54004=CARTESIAN_POINT ( 'NONE',  ( 86.62931800182292363, 20.48449268398422163, -8.977013608448025650 ) ) ;
#54006=CARTESIAN_POINT ( 'NONE',  ( -101.3492134984965389, 32.31003911421601771, -61.90232122945574389 ) ) ;
#54007=ORIENTED_EDGE ( 'NONE', *, *, #19208, .T. ) ;
#54014=CARTESIAN_POINT ( 'NONE',  ( 105.8229724512851391, 27.98935528750254420, -76.33106803925247164 ) ) ;
#54017=CARTESIAN_POINT ( 'NONE',  ( -77.02112161466365592, 22.77583432622784798, -62.13887678495888167 ) ) ;
#54019=CARTESIAN_POINT ( 'NONE',  ( 46.23113030541875190, 10.41513832761375902, -40.00976335710233656 ) ) ;
#54022=CARTESIAN_POINT ( 'NONE',  ( -25.79929641484368830, 9.749255553662431240, 5.903164045998831710 ) ) ;
#54026=ADVANCED_FACE ( 'NONE', ( #30554 ), #20006, .F. ) ;
#54027=CARTESIAN_POINT ( 'NONE',  ( -33.84080342750782222, 9.997552308299120227, 3.750042810399141668 ) ) ;
#54028=FACE_OUTER_BOUND ( 'NONE', #45184, .T. ) ;
#54029=CARTESIAN_POINT ( 'NONE',  ( 90.30840373526895348, 21.77864858272155146, 57.51652433617496030 ) ) ;
#54030=CARTESIAN_POINT ( 'NONE',  ( 156.5977259323288138, 56.97512126940428345, -24.24178231028911057 ) ) ;
#54032=CARTESIAN_POINT ( 'NONE',  ( -98.67557579989350813, 32.10670856967970366, -75.95360591899348890 ) ) ;
#54039=CARTESIAN_POINT ( 'NONE',  ( 58.47885130911549112, 12.69429933094348506, 58.16495201468348597 ) ) ;
#54040=CARTESIAN_POINT ( 'NONE',  ( 12.68603346975295487, 7.427591953486040843, -63.03079970252639441 ) ) ;
#54041=DIRECTION ( 'NONE',  ( 0.000000000000000000, -0.000000000000000000, -1.000000000000000000 ) ) ;
#54044=CARTESIAN_POINT ( 'NONE',  ( -4.504169684898444714, 6.697401007565301434, 44.34460521785229048 ) ) ;
#54045=CARTESIAN_POINT ( 'NONE',  ( -105.8768181937898447, 34.64545164169047808, -62.76079459674738104 ) ) ;
#54047=CARTESIAN_POINT ( 'NONE',  ( 79.20873702246476000, 18.07356264622685771, 89.75976143019885001 ) ) ;
#54052=CARTESIAN_POINT ( 'NONE',  ( -128.7650348665117122, 48.41336321950709731, 18.20782630100844202 ) ) ;
#54053=CARTESIAN_POINT ( 'NONE',  ( -170.2951623264597458, 85.51757001115475987, -35.25191629578037578 ) ) ;
#54054=CARTESIAN_POINT ( 'NONE',  ( -125.8938041572051105, 47.69968343338781835, -34.91370389823391918 ) ) ;
#54059=CARTESIAN_POINT ( 'NONE',  ( -157.0089340775362814, 70.81267942336693011, 91.81416744909685690 ) ) ;
#54062=EDGE_LOOP ( 'NONE', ( #41750, #43826, #30108, #24681 ) ) ;
#54064=CARTESIAN_POINT ( 'NONE',  ( 110.7164744784864041, 29.10110206241301967, -62.76698815611734972 ) ) ;
#54068=EDGE_CURVE ( 'NONE', #49352, #62757, #47053, .T. ) ;
#54077=CARTESIAN_POINT ( 'NONE',  ( -119.6686548882513392, 42.52932972989362526, -91.89361949810667340 ) ) ;
#54078=CYLINDRICAL_SURFACE ( 'NONE', #60775, 7.500000000000020428 ) ;
#54079=CARTESIAN_POINT ( 'NONE',  ( 153.2208437558771550, 55.67531116261156399, 16.26249285195666161 ) ) ;
#54084=CARTESIAN_POINT ( 'NONE',  ( 39.40195752203892710, -170.0000000000000000, -23.77526687496409608 ) ) ;
#54086=CARTESIAN_POINT ( 'NONE',  ( -147.9238768789327025, 64.15721743195632598, -88.62461181704978230 ) ) ;
#54087=CARTESIAN_POINT ( 'NONE',  ( -35.17600017528511813, 10.23461991275926586, -22.47999145424725498 ) ) ;
#54088=CARTESIAN_POINT ( 'NONE',  ( -166.3175803736862122, 79.86140754556167565, 41.48986120324848059 ) ) ;
#54089=CARTESIAN_POINT ( 'NONE',  ( 131.3924949472282719, 41.12442122814101708, 56.76750252905168281 ) ) ;
#54090=VERTEX_POINT ( 'NONE', #15414 ) ;
#54092=ORIENTED_EDGE ( 'NONE', *, *, #50105, .T. ) ;
#54095=CARTESIAN_POINT ( 'NONE',  ( 63.01563776193091826, 12.67277567978498176, -77.56524142263344856 ) ) ;
#54104=FACE_OUTER_BOUND ( 'NONE', #31738, .T. ) ;
#54105=CARTESIAN_POINT ( 'NONE',  ( 183.9986899696430669, 81.60141257362811018, 29.88476414464218323 ) ) ;
#54107=CARTESIAN_POINT ( 'NONE',  ( -71.16584859396996876, 19.60484997908767113, 11.30861530554621730 ) ) ;
#54109=CARTESIAN_POINT ( 'NONE',  ( 23.03546163277112413, 7.848986635155157821, 39.46112786506829906 ) ) ;
#54113=CARTESIAN_POINT ( 'NONE',  ( 162.6205203824432317, 63.07332653227187791, -65.01131320985699347 ) ) ;
#54116=B_SPLINE_CURVE_WITH_KNOTS ( 'NONE', 3,
 ( #57926, #31205, #58596, #53311, #63550, #26603, #36821, #62519, #52637, #47350, #911, #27982, #32912, #38537, #1255, #60344, #59628, #16042, #33628, #22361, #32230, #11440, #21662, #64228, #55058, #53997, #65634, #59291, #59981, #17422, #53665, #37493, #54350, #6173, #5822, #28329, #27635, #5488, #49072, #43798, #65274, #6877, #16727 ),
 .UNSPECIFIED., .F., .F.,
 ( 4, 2, 2, 2, 2, 2, 2, 2, 2, 2, 2, 2, 1, 2, 2, 2, 2, 2, 2, 2, 2, 4 ),
 ( 0.02379577142314830140, 0.02527778373276530488, 0.02601878988757379968, 0.02675979604238229101, 0.02824180835199927714, 0.02972382066161625980, 0.03046482681642476154, 0.03120583297123326327, 0.03268784528085027369, 0.03416985759046728410, 0.03565186990008429452, 0.03639287605489279626, 0.03713388220970130493, 0.03787488836450979973, 0.03861589451931830147, 0.04009790682893531188, 0.04157991913855231536, 0.04306193144816932578, 0.04380293760297782057, 0.04454394375778632231, 0.04602595606740332579, 0.04750796837702032926 ),
 .UNSPECIFIED. ) ;
#54122=CARTESIAN_POINT ( 'NONE',  ( -78.66644367742111399, 22.32174330031316956, 45.41820113967312977 ) ) ;
#54125=CARTESIAN_POINT ( 'NONE',  ( 40.38132770291768026, 9.553709436640062336, 44.86553172969242098 ) ) ;
#54128=CARTESIAN_POINT ( 'NONE',  ( -23.99924996210628336, 8.487987924059023470, 65.54065325144799203 ) ) ;
#54136=PLANE ( 'NONE',  #22242 ) ;
#54137=CARTESIAN_POINT ( 'NONE',  ( 186.3463695477168187, 85.57362603246809840, -92.05568032583515503 ) ) ;
#54139=CARTESIAN_POINT ( 'NONE',  ( -4.506365319453815133, 7.705038994660848850, 57.73001332318100509 ) ) ;
#54148=CARTESIAN_POINT ( 'NONE',  ( 138.5721691894143532, 44.34516164557648210, -76.22048844638042908 ) ) ;
#54149=CARTESIAN_POINT ( 'NONE',  ( 68.61679388097590504, 14.04192738700836607, 32.31919998833575391 ) ) ;
#54153=ADVANCED_FACE ( 'NONE', ( #58646 ), #26655, .F. ) ;
#54155=CARTESIAN_POINT ( 'NONE',  ( 86.15410276028859471, 19.25894675708889991, 2.867536982015614910 ) ) ;
#54157=CARTESIAN_POINT ( 'NONE',  ( -74.19961951691010427, 20.67022044985851181, 31.88851621870251307 ) ) ;
#54160=EDGE_LOOP ( 'NONE', ( #5777, #5644, #24092, #49574 ) ) ;
#54162=CARTESIAN_POINT ( 'NONE',  ( 91.11342358617753234, 21.00000175105273570, 4.350741119497574694 ) ) ;
#54169=LINE ( 'NONE', #27103, #35727 ) ;
#54170=CARTESIAN_POINT ( 'NONE',  ( 151.7819978880463907, 53.35998893001570309, 32.01513195124016420 ) ) ;
#54171=CARTESIAN_POINT ( 'NONE',  ( -180.3114074031036296, 97.09758726817787533, -44.36644437796192619 ) ) ;
#54175=ORIENTED_EDGE ( 'NONE', *, *, #30646, .T. ) ;
#54176=CARTESIAN_POINT ( 'NONE',  ( 136.1215428813736708, 43.99260314811115080, -77.53266360357038423 ) ) ;
#54180=FACE_BOUND ( 'NONE', #42569, .T. ) ;
#54181=CARTESIAN_POINT ( 'NONE',  ( -6.126800896373019611, 6.786243985899685249, -77.07188336801345940 ) ) ;
#54184=CARTESIAN_POINT ( 'NONE',  ( -124.1095621208148572, 46.52671329146387791, -35.07131596630200221 ) ) ;
#54185=CARTESIAN_POINT ( 'NONE',  ( -81.24432217070636852, 24.40203426192926628, 18.12073039003383101 ) ) ;
#54187=CARTESIAN_POINT ( 'NONE',  ( -154.0718453320783681, 68.14976693162394383, 5.420520227110683820 ) ) ;
#54189=CARTESIAN_POINT ( 'NONE',  ( 68.61679388097593346, 14.04192738700836784, 5.474649397872059176 ) ) ;
#54190=CARTESIAN_POINT ( 'NONE',  ( 116.5096233816162226, 31.89062767870469273, 6.138510810235731974 ) ) ;
#54191=CARTESIAN_POINT ( 'NONE',  ( 89.20981392318256553, 21.38519354635265657, -9.430786644822518383 ) ) ;
#54194=CARTESIAN_POINT ( 'NONE',  ( 133.8566784816069344, 41.42467568809808398, -89.71241211332301191 ) ) ;
#54198=CARTESIAN_POINT ( 'NONE',  ( 117.6677778655470377, 33.59861415422441411, 89.68390048962857009 ) ) ;
#54199=CARTESIAN_POINT ( 'NONE',  ( -147.3669217311067712, 63.69361261596462498, 57.87395473753091579 ) ) ;
#54201=CARTESIAN_POINT ( 'NONE',  ( -23.99957301099517082, 9.503061049698471763, -43.79968545520912926 ) ) ;
#54202=CARTESIAN_POINT ( 'NONE',  ( -47.94536219817736367, 13.92422159065987408, -72.00662047797626997 ) ) ;
#54203=B_SPLINE_CURVE_WITH_KNOTS ( 'NONE', 3,
 ( #54122, #28107, #59416, #23200, #66129, #64705, #65407, #49550, #59755, #16514, #33045, #1382, #65056, #12640, #65766, #5946, #7371, #1038, #27406, #11227, #22489, #32693, #28465, #55538, #48844, #690, #34103, #22137, #17197, #39030, #60474, #43585, #44646, #17916, #16855, #38669, #60114, #11935, #55187, #33407, #38312, #12288, #54480, #6307, #48493, #54836, #27759 ),
 .UNSPECIFIED., .F., .F.,
 ( 4, 2, 2, 2, 2, 2, 2, 2, 2, 2, 2, 2, 1, 2, 2, 2, 2, 2, 2, 2, 2, 2, 2, 4 ),
 ( 0.000000000000000000, 0.001520400357568945033, 0.002280600536353434571, 0.003040800715137924760, 0.004561201072706896897, 0.005321401251491367571, 0.006081601430275837376, 0.007602001787844763978, 0.008362201966629231181, 0.009122402145413698385, 0.01064280250298265361, 0.01140300268176713816, 0.01216320286055162618, 0.01292340303933611073, 0.01368360321812059875, 0.01520400357568958000, 0.01596420375447406975, 0.01672440393325855951, 0.01824480429082751820, 0.01976520464839648036, 0.02052540482718096318, 0.02128560500596544600, 0.02280600536353444285, 0.02432640572110343971 ),
 .UNSPECIFIED. ) ;
#54208=EDGE_CURVE ( 'NONE', #1836, #51958, #59610, .T. ) ;
#54209=CARTESIAN_POINT ( 'NONE',  ( 32.89501968360929851, 8.663558833820820482, 68.02007762215981757 ) ) ;
#54210=CARTESIAN_POINT ( 'NONE',  ( -168.0052514572427071, 83.06849406765624622, 70.65604521105746016 ) ) ;
#54215=AXIS2_PLACEMENT_3D ( 'NONE', #38553, #1273, #59998 ) ;
#54220=CARTESIAN_POINT ( 'NONE',  ( 181.9295958320008140, 80.90438706151871884, -24.34483382478239832 ) ) ;
#54223=CARTESIAN_POINT ( 'NONE',  ( 46.64694836521739774, 9.462741877720626249, -18.23014210735218654 ) ) ;
#54224=CARTESIAN_POINT ( 'NONE',  ( 210.6475357757681763, 114.8748261044496388, -21.55495887534324950 ) ) ;
#54228=AXIS2_PLACEMENT_3D ( 'NONE', #59166, #6048, #63429 ) ;
#54231=CARTESIAN_POINT ( 'NONE',  ( 94.06416612695406343, 23.16920323269611970, -42.30311029455274507 ) ) ;
#54233=CARTESIAN_POINT ( 'NONE',  ( -47.56466076048272384, 13.83435953640667826, 64.17104296208425751 ) ) ;
#54235=DIRECTION ( 'NONE',  ( 0.000000000000000000, 0.000000000000000000, 1.000000000000000000 ) ) ;
#54243=CARTESIAN_POINT ( 'NONE',  ( 198.7765072002625288, 98.56267746775340299, 94.99999999999866418 ) ) ;
#54245=CARTESIAN_POINT ( 'NONE',  ( 106.4107271020440209, 27.14892220304137993, 30.65973466290294525 ) ) ;
#54249=CARTESIAN_POINT ( 'NONE',  ( 160.4986104110022609, 61.33701824525267199, 43.77471383263033289 ) ) ;
#54250=CARTESIAN_POINT ( 'NONE',  ( 110.2429982417149432, 29.99119854320847267, 2.766663615273645682 ) ) ;
#54253=CARTESIAN_POINT ( 'NONE',  ( -51.77779688167511551, 14.86590802019197000, -49.46793554282675132 ) ) ;
#54256=CARTESIAN_POINT ( 'NONE',  ( 10.83521140779424208, 7.398743030771590234, 31.86172333737584950 ) ) ;
#54258=CARTESIAN_POINT ( 'NONE',  ( 79.14402072927414622, 17.00139091204388819, 91.48213081605835839 ) ) ;
#54260=ORIENTED_EDGE ( 'NONE', *, *, #4760, .F. ) ;
#54264=CIRCLE ( 'NONE', #43025, 243.4957430088094839 ) ;
#54265=CARTESIAN_POINT ( 'NONE',  ( -11.78792974237933322, 7.181513757308651158, -22.44595994035757514 ) ) ;
#54266=CARTESIAN_POINT ( 'NONE',  ( -55.05276343752909440, 14.68156374112637863, 45.31732777293115788 ) ) ;
#54271=CARTESIAN_POINT ( 'NONE',  ( -33.38294402636584124, 10.93918551420889607, 71.82136885757543610 ) ) ;
#54275=CARTESIAN_POINT ( 'NONE',  ( 157.4703587214989113, 57.65129005721576760, -77.96873488960135035 ) ) ;
#54282=VERTEX_POINT ( 'NONE', #1309 ) ;
#54283=CARTESIAN_POINT ( 'NONE',  ( 63.99027454648602031, 13.93445177372599098, -23.82830888214883558 ) ) ;
#54286=CARTESIAN_POINT ( 'NONE',  ( -26.44231144410477086, 9.840790913154485509, 85.80307888686122908 ) ) ;
#54288=CARTESIAN_POINT ( 'NONE',  ( -109.3432140528234697, 36.51591785955881875, 13.74895797865885783 ) ) ;
#54290=CARTESIAN_POINT ( 'NONE',  ( 136.7507824285648610, 44.38599729999915411, -9.755793251951397238 ) ) ;
#54292=ORIENTED_EDGE ( 'NONE', *, *, #39306, .F. ) ;
#54295=CARTESIAN_POINT ( 'NONE',  ( -156.4966862384868591, 71.70877417666513054, -12.69550417867896286 ) ) ;
#54296=CARTESIAN_POINT ( 'NONE',  ( 32.03384598935271299, 8.576372641735986235, -41.65668636982230311 ) ) ;
#54299=CARTESIAN_POINT ( 'NONE',  ( -37.38262509017738466, 10.64263598035110192, 69.16181315953529918 ) ) ;
#54302=CARTESIAN_POINT ( 'NONE',  ( 188.0094179620990928, 87.39792407168449984, 60.76004803506884855 ) ) ;
#54303=CARTESIAN_POINT ( 'NONE',  ( -149.5074843970971017, 64.17983161892347255, 72.56537183036277838 ) ) ;
#54304=CARTESIAN_POINT ( 'NONE',  ( -2.172839205444464739, 7.595638683704372340, -47.87223819190520402 ) ) ;
#54305=CARTESIAN_POINT ( 'NONE',  ( 102.7571040248401033, 25.57023079238896912, 10.79413422094299690 ) ) ;
#54307=CARTESIAN_POINT ( 'NONE',  ( -84.54326985437107567, 24.64760594531649218, -37.92967292645255384 ) ) ;
#54308=CARTESIAN_POINT ( 'NONE',  ( 22.29513692215318343, 6.796052026456515627, 60.59742216850811758 ) ) ;
#54310=CARTESIAN_POINT ( 'NONE',  ( 15.78827728214693416, 6.500811158483329244, -62.36349468914946925 ) ) ;
#54311=B_SPLINE_CURVE_WITH_KNOTS ( 'NONE', 3,
 ( #25300, #56249, #8063, #8419, #13013, #7729, #29872, #40077, #51334, #3480, #61534, #13352, #40765, #24607, #50978, #46040, #24260, #9453, #48099, #4176, #64292, #5208, #52691, #69558, #59006, #47759, #20689, #26662, #30914, #52362, #32290, #15761, #15072, #63949, #21378, #36881, #42821, #37208, #53724, #25646, #4858, #16100, #47076, #41808, #63266, #58655 ),
 .UNSPECIFIED., .F., .F.,
 ( 4, 2, 2, 2, 2, 2, 2, 2, 2, 2, 2, 2, 2, 2, 2, 2, 2, 2, 2, 2, 2, 2, 4 ),
 ( 0.02404638330965504917, 0.02555608299537569239, 0.02631093283823601400, 0.02706578268109633562, 0.02857548236681698231, 0.02933033220967730392, 0.03008518205253762554, 0.03159488173825823754, 0.03310458142397884607, 0.03385943126683915033, 0.03461428110969945460, 0.03612398079542002843, 0.03687883063828029107, 0.03763368048114055370, 0.03838853032400082327, 0.03914338016686108590, 0.04065307985258157647, 0.04216277953830206704, 0.04367247922402255067, 0.04518217890974304124, 0.04593702875260328999, 0.04669187859546353181, 0.04820157828118398075 ),
 .UNSPECIFIED. ) ;
#54312=B_SPLINE_CURVE_WITH_KNOTS ( 'NONE', 3,
 ( #24298, #61902, #30261, #62618, #51710, #19346, #28876, #13052, #45740, #50327, #23597, #39767, #29216, #66518, #46077, #8457, #67220, #67898, #34511, #55954, #50664, #24987, #45388, #40457, #8809, #8103, #66867, #67548, #18666, #13725, #29910, #51020, #19693, #41158, #61575, #40802, #62257, #14426, #56287, #29553, #56991, #58021, #58688, #69257, #9147 ),
 .UNSPECIFIED., .F., .F.,
 ( 4, 2, 2, 1, 2, 2, 2, 2, 2, 2, 2, 2, 2, 2, 2, 2, 2, 2, 2, 2, 2, 2, 4 ),
 ( 0.02346464386237016517, 0.02493212228186624663, 0.02566586149161428909, 0.02639960070136233156, 0.02713333991111037402, 0.02786707912085841649, 0.02933455754035451182, 0.03006829675010256817, 0.03080203595985062451, 0.03226951437934675454, 0.03300325358909481782, 0.03373699279884288804, 0.03520447121833901460, 0.03667194963783514117, 0.03740568884758318363, 0.03813942805733122610, 0.03960690647682735266, 0.04107438489632347922, 0.04254186331581959885, 0.04327560252556765519, 0.04400934173531571847, 0.04547682015481184503, 0.04694429857430796466 ),
 .UNSPECIFIED. ) ;
#54313=ORIENTED_EDGE ( 'NONE', *, *, #59918, .F. ) ;
#54317=CARTESIAN_POINT ( 'NONE',  ( -131.6508182719823594, 50.40277850441010798, -74.09140414498664029 ) ) ;
#54318=CARTESIAN_POINT ( 'NONE',  ( -130.6002960060536680, 49.67125682092489569, -48.27322245354486796 ) ) ;
#54322=VECTOR ( 'NONE', #19379, 1000.000000000000000 ) ;
#54325=CARTESIAN_POINT ( 'NONE',  ( -133.1167005700037294, 51.43735670037489172, -94.02487124159708287 ) ) ;
#54330=VECTOR ( 'NONE', #26333, 1000.000000000000000 ) ;
#54331=CARTESIAN_POINT ( 'NONE',  ( 173.6020601204682805, 71.36108012062136652, -43.12795722065862947 ) ) ;
#54333=ORIENTED_EDGE ( 'NONE', *, *, #6991, .F. ) ;
#54335=CARTESIAN_POINT ( 'NONE',  ( 136.7690435008551617, 44.39743995805025634, 56.93957293383409279 ) ) ;
#54336=CARTESIAN_POINT ( 'NONE',  ( -73.10694748374054086, 20.28107308417882493, -47.67311660692905662 ) ) ;
#54338=CARTESIAN_POINT ( 'NONE',  ( 80.69264259299148989, 17.48002198187963430, -92.40914142493147665 ) ) ;
#54339=CARTESIAN_POINT ( 'NONE',  ( 19.78559780309666394, 6.660707902886499276, -90.30598456206999458 ) ) ;
#54340=B_SPLINE_CURVE_WITH_KNOTS ( 'NONE', 3,
 ( #68942, #20768, #25025, #25718, #24682, #52089, #41195, #62656, #62301, #52762, #68612, #4588, #14112, #46459, #35575, #57371, #57034, #51748, #68280, #35921, #9184, #3554, #3909, #36261, #25378, #20419, #46813, #41883, #30992, #47484, #20084, #15152, #41539, #57718, #14798, #9531, #52439, #36610, #58063, #26057, #56678, #8497, #29949, #26740, #38322, #15835, #10201, #27417, #5615, #37279 ),
 .UNSPECIFIED., .F., .F.,
 ( 4, 2, 2, 2, 2, 2, 2, 2, 2, 2, 2, 2, 2, 2, 2, 2, 2, 2, 2, 2, 2, 2, 2, 2, 4 ),
 ( 0.03126542424884325155, 0.03330676804260264412, 0.03534811183636203669, 0.03738945563012142231, 0.03943079942388081488, 0.04045147132076052504, 0.04147214321764023520, 0.04249281511451994536, 0.04351348701139965552, 0.04555483080515909666, 0.04657550270203882070, 0.04759617459891854474, 0.04810651054735841370, 0.04861684649579828266, 0.04963751839267800670, 0.05065819028955773073, 0.05167886218643745477, 0.05269953408331717881, 0.05372020598019690285, 0.05474087787707662689, 0.05576154977395635093, 0.05780289356771586839, 0.05984423736147539280, 0.06188558115523491721, 0.06392692494899443467 ),
 .UNSPECIFIED. ) ;
#54341=CARTESIAN_POINT ( 'NONE',  ( -49.43836229152576323, 14.28302414152159372, -20.86921515441098407 ) ) ;
#54343=CARTESIAN_POINT ( 'NONE',  ( -121.5677746760273692, 43.71038933438990881, -9.424279492981348483 ) ) ;
#54346=CARTESIAN_POINT ( 'NONE',  ( -142.3260422482980800, 59.60034523324941347, -40.07815075408650074 ) ) ;
#54350=CARTESIAN_POINT ( 'NONE',  ( 58.08938767906774103, 12.61185010801509776, 16.14489018905632989 ) ) ;
#54353=DIRECTION ( 'NONE',  ( 0.000000000000000000, 0.000000000000000000, 1.000000000000000000 ) ) ;
#54355=CARTESIAN_POINT ( 'NONE',  ( 188.4359598230020083, 86.36951380984521620, -18.39236985717185391 ) ) ;
#54357=CARTESIAN_POINT ( 'NONE',  ( 86.62931800182293784, 19.42108912189600645, -8.977013608448025650 ) ) ;
#54358=CARTESIAN_POINT ( 'NONE',  ( 86.62931800182293784, -170.0000000000000000, 64.05663816294301682 ) ) ;
#54360=CARTESIAN_POINT ( 'NONE',  ( 199.7255144154429445, 99.76581417577200739, 4.229220098907731540 ) ) ;
#54362=CARTESIAN_POINT ( 'NONE',  ( -96.76159256735193992, 30.06445763698410900, 16.27712563862165851 ) ) ;
#54368=CARTESIAN_POINT ( 'NONE',  ( 9.416603677636258496, 6.380307115728824030, 33.55093279848803434 ) ) ;
#54369=DIRECTION ( 'NONE',  ( 0.000000000000000000, 0.000000000000000000, 1.000000000000000000 ) ) ;
#54372=CARTESIAN_POINT ( 'NONE',  ( 205.5049354810105910, 109.1776577097390657, -51.32593103262160383 ) ) ;
#54373=CARTESIAN_POINT ( 'NONE',  ( -72.21947956767110099, 21.03570528348186031, -73.30056851817380448 ) ) ;
#54375=AXIS2_PLACEMENT_3D ( 'NONE', #34536, #23280, #17995 ) ;
#54376=CARTESIAN_POINT ( 'NONE',  ( 45.04506994399701370, 10.22854084020123899, -48.08472337634788119 ) ) ;
#54377=CARTESIAN_POINT ( 'NONE',  ( 211.8476521439973794, 116.6941316755177382, 65.83984939228595579 ) ) ;
#54378=ORIENTED_EDGE ( 'NONE', *, *, #57298, .F. ) ;
#54379=AXIS2_PLACEMENT_3D ( 'NONE', #14224, #7909, #35687 ) ;
#54380=CARTESIAN_POINT ( 'NONE',  ( -102.7456062648101209, 33.01749955571781214, -23.17002667451225406 ) ) ;
#54381=EDGE_LOOP ( 'NONE', ( #14359, #56015 ) ) ;
#54382=CARTESIAN_POINT ( 'NONE',  ( -14.19447842053094178, 7.389800932646227061, -38.94998986089500193 ) ) ;
#54385=CARTESIAN_POINT ( 'NONE',  ( 90.30732934992394689, 21.77797012484621320, 70.61059424602628098 ) ) ;
#54390=CARTESIAN_POINT ( 'NONE',  ( 116.5796390945666019, 33.05011449662006129, -93.07866499088535761 ) ) ;
#54391=CARTESIAN_POINT ( 'NONE',  ( 210.8249406480391883, 115.1412791740558106, 94.73500360378400842 ) ) ;
#54396=CARTESIAN_POINT ( 'NONE',  ( -26.87327614295024958, 8.886070347947290671, 16.84225167926756939 ) ) ;
#54397=CARTESIAN_POINT ( 'NONE',  ( 42.71680114082827373, 9.880016734137543111, -63.21884616217572983 ) ) ;
#54398=CARTESIAN_POINT ( 'NONE',  ( -0.5158933718595605233, 6.525180340836108428, 39.31287253911112600 ) ) ;
#54399=CARTESIAN_POINT ( 'NONE',  ( 110.2429982417149574, 29.99119854320844425, -62.76698815611734972 ) ) ;
#54400=CARTESIAN_POINT ( 'NONE',  ( 93.83003346581507742, 23.08044164087233341, 88.77615774936755599 ) ) ;
#54401=VERTEX_POINT ( 'NONE', #29776 ) ;
#54404=CARTESIAN_POINT ( 'NONE',  ( -125.8938041572051389, 46.49392987655491538, 18.77539728269342945 ) ) ;
#54405=CARTESIAN_POINT ( 'NONE',  ( -165.6208371326873703, 80.58821715390999429, -42.50979365522336195 ) ) ;
#54406=CARTESIAN_POINT ( 'NONE',  ( -180.3485529394662024, 95.55077600385843084, 89.97650250217222379 ) ) ;
#54408=CARTESIAN_POINT ( 'NONE',  ( -118.4622862908118890, 41.79153065058247307, -41.36719475118654543 ) ) ;
#54410=CARTESIAN_POINT ( 'NONE',  ( 133.8566784816069060, 41.42467568809810530, -51.02331093239568816 ) ) ;
#54416=CARTESIAN_POINT ( 'NONE',  ( 86.15454111412294935, 20.32174891186167187, 2.867536982015618019 ) ) ;
#54418=CARTESIAN_POINT ( 'NONE',  ( 181.0840389613909736, 78.60582251573003987, -78.06960825634331513 ) ) ;
#54420=CARTESIAN_POINT ( 'NONE',  ( 113.8724110608469431, 31.71510301790681652, 3.685887770946741693 ) ) ;
#54426=ORIENTED_EDGE ( 'NONE', *, *, #45337, .T. ) ;
#54428=CARTESIAN_POINT ( 'NONE',  ( -121.5528704565120819, 43.70117646488017016, -89.97093067013521761 ) ) ;
#54433=CARTESIAN_POINT ( 'NONE',  ( 160.5141379054754225, 60.05651755415394888, 43.77875689395856540 ) ) ;
#54437=CARTESIAN_POINT ( 'NONE',  ( -142.2711026674345760, 59.55689780112353304, -93.96688110664084093 ) ) ;
#54440=CARTESIAN_POINT ( 'NONE',  ( 152.0785009218370760, 53.57704863418404528, -92.08473246085713981 ) ) ;
#54441=CARTESIAN_POINT ( 'NONE',  ( -38.93878980550034186, 10.94326053663841769, -69.16458801474382767 ) ) ;
#54442=ORIENTED_EDGE ( 'NONE', *, *, #62514, .F. ) ;
#54444=VERTEX_POINT ( 'NONE', #30134 ) ;
#54445=EDGE_CURVE ( 'NONE', #5653, #50582, #57552, .T. ) ;
#54446=LINE ( 'NONE', #42857, #5881 ) ;
#54450=CARTESIAN_POINT ( 'NONE',  ( -37.79601571721867259, 10.72155118426296561, -38.82969307849655394 ) ) ;
#54451=CARTESIAN_POINT ( 'NONE',  ( -97.10826110816122991, 30.23021954617678020, 86.26777175360041383 ) ) ;
#54455=CARTESIAN_POINT ( 'NONE',  ( 79.38459371357852490, 17.07499996355401350, 66.06145663816440106 ) ) ;
#54458=ORIENTED_EDGE ( 'NONE', *, *, #53580, .T. ) ;
#54460=CARTESIAN_POINT ( 'NONE',  ( 209.9944361927103955, 113.8994774711241433, -75.98551876403080030 ) ) ;
#54465=CARTESIAN_POINT ( 'NONE',  ( -32.91766192354460685, 9.838705478717917785, -89.15043209282478642 ) ) ;
#54466=DIRECTION ( 'NONE',  ( 0.000000000000000000, 0.000000000000000000, 1.000000000000000000 ) ) ;
#54469=EDGE_CURVE ( 'NONE', #59450, #25590, #24396, .T. ) ;
#54471=CARTESIAN_POINT ( 'NONE',  ( 159.6614743841974757, 60.66237087206235401, -77.65552351392290120 ) ) ;
#54475=DIRECTION ( 'NONE',  ( 0.000000000000000000, 0.000000000000000000, 1.000000000000000000 ) ) ;
#54479=ORIENTED_EDGE ( 'NONE', *, *, #30736, .F. ) ;
#54480=CARTESIAN_POINT ( 'NONE',  ( -81.01337222286373674, 23.22902179892322749, 30.77879346308872144 ) ) ;
#54483=CARTESIAN_POINT ( 'NONE',  ( 39.40195752203891999, 9.424259417798149130, 44.91383430596327742 ) ) ;
#54484=CARTESIAN_POINT ( 'NONE',  ( -23.93965512371324067, 8.480096402797087762, 64.05595943103627121 ) ) ;
#54486=CARTESIAN_POINT ( 'NONE',  ( 127.4953815656694758, 37.71366486045443622, -12.67436558192646601 ) ) ;
#54491=FACE_OUTER_BOUND ( 'NONE', #25970, .T. ) ;
#54493=CARTESIAN_POINT ( 'NONE',  ( 55.51597771111713797, 11.05737652677075999, 64.65722201551544401 ) ) ;
#54494=CARTESIAN_POINT ( 'NONE',  ( -1.862553927312063706, 7.582910205528083480, 59.88481149980647444 ) ) ;
#54495=VERTEX_POINT ( 'NONE', #9711 ) ;
#54496=CARTESIAN_POINT ( 'NONE',  ( -119.1795380581000359, 42.22910606512926535, -72.61016301487133262 ) ) ;
#54502=CARTESIAN_POINT ( 'NONE',  ( 135.6842057900327632, 42.53841116629842389, -63.07930687841992068 ) ) ;
#54506=CARTESIAN_POINT ( 'NONE',  ( 83.60262962804348774, 18.41036205028016326, 3.501146626846444398 ) ) ;
#54508=CARTESIAN_POINT ( 'NONE',  ( -71.41745561414263932, 19.69148172991714318, 39.90720259758258237 ) ) ;
#54518=AXIS2_PLACEMENT_3D ( 'NONE', #8488, #45417, #55272 ) ;
#54519=AXIS2_PLACEMENT_3D ( 'NONE', #37044, #33158, #15929 ) ;
#54523=ADVANCED_FACE ( 'NONE', ( #63514 ), #63863, .T. ) ;
#54527=CARTESIAN_POINT ( 'NONE',  ( 33.93974911725172916, 8.773765372885550917, 32.26854139689001499 ) ) ;
#54530=CARTESIAN_POINT ( 'NONE',  ( -133.1093894320205493, 51.43221067881452768, -17.68593715264120192 ) ) ;
#54535=CARTESIAN_POINT ( 'NONE',  ( 137.6104751318277124, 44.92718313329109492, -76.86516922214269698 ) ) ;
#54538=EDGE_CURVE ( 'NONE', #1914, #29362, #11071, .T. ) ;
#54539=FACE_BOUND ( 'NONE', #33443, .T. ) ;
#54540=CARTESIAN_POINT ( 'NONE',  ( -1.083610669212420330, 6.545642299653470886, -66.43984342559842560 ) ) ;
#54541=CARTESIAN_POINT ( 'NONE',  ( -180.2243452982809231, 96.99029284948635166, 67.59096301620702718 ) ) ;
#54544=CARTESIAN_POINT ( 'NONE',  ( -85.95621526752228192, 26.32462117888281128, 9.292053853339920622 ) ) ;
#54545=CARTESIAN_POINT ( 'NONE',  ( 132.9440032680862771, 40.87616997986732059, 2.718024143144065707 ) ) ;
#54547=CARTESIAN_POINT ( 'NONE',  ( -71.71116731091892404, 19.79303856213887869, -93.48959018091433393 ) ) ;
#54548=CARTESIAN_POINT ( 'NONE',  ( -12.39770133248888584, 8.241491894828993026, 31.65004457334004329 ) ) ;
#54549=CARTESIAN_POINT ( 'NONE',  ( 164.9534461562627143, 63.71129898458563190, 9.487489937330947143 ) ) ;
#54550=CARTESIAN_POINT ( 'NONE',  ( 93.87650740736113164, 23.09802612281733758, -18.47339464351970761 ) ) ;
#54555=CARTESIAN_POINT ( 'NONE',  ( 83.37782009939533623, 19.39546426214656094, -63.40324210487996481 ) ) ;
#54556=CARTESIAN_POINT ( 'NONE',  ( 103.8353834748950533, 27.12366330047747454, 94.71338854545251706 ) ) ;
#54559=EDGE_CURVE ( 'NONE', #23453, #7404, #1703, .T. ) ;
#54561=CARTESIAN_POINT ( 'NONE',  ( -24.71604178686819253, 9.599501655372941755, -46.15064928016835211 ) ) ;
#54563=CARTESIAN_POINT ( 'NONE',  ( -50.52615126106341137, 14.55080735582892792, -75.56057009363912869 ) ) ;
#54564=CARTESIAN_POINT ( 'NONE',  ( -72.32580847922558576, 21.07301141147191359, -92.29252585439962786 ) ) ;
#54566=CARTESIAN_POINT ( 'NONE',  ( -125.8938041572051389, 47.69968343338778283, -23.06915330777029638 ) ) ;
#54567=ORIENTED_EDGE ( 'NONE', *, *, #66343, .F. ) ;
#54569=CARTESIAN_POINT ( 'NONE',  ( 34.82939798935584719, 8.870855050008906062, 70.22358934348724802 ) ) ;
#54570=CARTESIAN_POINT ( 'NONE',  ( 179.4279766878530040, 76.94722012158231905, 56.32619385280453628 ) ) ;
#54572=DIRECTION ( 'NONE',  ( 0.000000000000000000, 0.000000000000000000, 1.000000000000000000 ) ) ;
#54573=CARTESIAN_POINT ( 'NONE',  ( -172.3127615181936108, 87.73358064377640630, -22.83500978608775256 ) ) ;
#54577=CARTESIAN_POINT ( 'NONE',  ( 91.12448333640237763, 22.07449368110503229, 4.344509129112214652 ) ) ;
#54580=CARTESIAN_POINT ( 'NONE',  ( -11.57931195747592135, 7.164335452024272577, 70.97150444363501265 ) ) ;
#54581=CARTESIAN_POINT ( 'NONE',  ( -82.32750425780474757, 23.74963782027935011, -9.207586315752052997 ) ) ;
#54582=DIRECTION ( 'NONE',  ( -0.000000000000000000, 1.000000000000000000, -0.000000000000000000 ) ) ;
#54583=CARTESIAN_POINT ( 'NONE',  ( 45.02738683369922512, 9.207938468499236251, -21.24168803743694411 ) ) ;
#54584=CARTESIAN_POINT ( 'NONE',  ( 210.0292194063021896, 113.9511645670926328, -11.70118341294292286 ) ) ;
#54585=FACE_BOUND ( 'NONE', #7233, .T. ) ;
#54587=CARTESIAN_POINT ( 'NONE',  ( -62.53989795537026453, 16.81768094534200841, -42.21107432078621002 ) ) ;
#54592=CARTESIAN_POINT ( 'NONE',  ( 93.87650740736111743, 23.09802612281734113, -45.31794523398337304 ) ) ;
#54593=CARTESIAN_POINT ( 'NONE',  ( -51.34542473642582650, 14.75635007918829444, 58.13766928157564706 ) ) ;
#54595=CARTESIAN_POINT ( 'NONE',  ( 206.3053863259449940, 110.3084416756849464, 70.92284527924854842 ) ) ;
#54605=CARTESIAN_POINT ( 'NONE',  ( 103.1653143050726271, 25.74301230421575681, 39.64379936348838385 ) ) ;
#54606=ORIENTED_EDGE ( 'NONE', *, *, #35200, .T. ) ;
#54609=CARTESIAN_POINT ( 'NONE',  ( 163.2911130186310515, 63.63047778106599139, 41.64567797802362037 ) ) ;
#54611=CARTESIAN_POINT ( 'NONE',  ( 70.26936813788618963, 15.51386666370915179, 8.498182904468185583 ) ) ;
#54612=PLANE ( 'NONE',  #56773 ) ;
#54615=CARTESIAN_POINT ( 'NONE',  ( 104.3759779378692514, 27.35691041569134185, -11.87929481196654002 ) ) ;
#54616=AXIS2_PLACEMENT_3D ( 'NONE', #22898, #23605, #55960 ) ;
#54620=CARTESIAN_POINT ( 'NONE',  ( -156.3880368899749840, 71.60874093180113675, -93.00681123627661862 ) ) ;
#54622=EDGE_CURVE ( 'NONE', #63051, #9029, #27727, .T. ) ;
#54623=CARTESIAN_POINT ( 'NONE',  ( 82.33420414567002865, 17.99921649865971673, 84.71689430370859952 ) ) ;
#54626=VERTEX_POINT ( 'NONE', #45522 ) ;
#54630=CARTESIAN_POINT ( 'NONE',  ( -10.23402954931276554, 7.059791383763804440, -8.966552176226290527 ) ) ;
#54631=DIRECTION ( 'NONE',  ( 0.000000000000000000, 0.000000000000000000, 1.000000000000000000 ) ) ;
#54634=CARTESIAN_POINT ( 'NONE',  ( 134.3159642998340075, 41.70198410084974938, 56.35489142945900198 ) ) ;
#54635=CARTESIAN_POINT ( 'NONE',  ( -58.97243502469714826, 16.81420332340175605, -36.31741409159577927 ) ) ;
#54636=CARTESIAN_POINT ( 'NONE',  ( -14.92860730136983882, 8.468845235798738713, -18.49331991024065758 ) ) ;
#54639=ORIENTED_EDGE ( 'NONE', *, *, #34088, .F. ) ;
#54644=CARTESIAN_POINT ( 'NONE',  ( -142.0729208125266325, 59.40063722436774185, 12.51388629237925265 ) ) ;
#54647=CARTESIAN_POINT ( 'NONE',  ( -97.88309373898363219, 30.60238467438962218, -48.60923466570785223 ) ) ;
#54650=CYLINDRICAL_SURFACE ( 'NONE', #62914, 7.500000000000013323 ) ;
#54652=CARTESIAN_POINT ( 'NONE',  ( 140.4769819293527178, 46.76840769395177944, -20.21251253278985871 ) ) ;
#54654=ORIENTED_EDGE ( 'NONE', *, *, #48961, .T. ) ;
#54656=CARTESIAN_POINT ( 'NONE',  ( -12.39413342787890926, 7.231444436041488011, 16.73898743515862009 ) ) ;
#54657=CARTESIAN_POINT ( 'NONE',  ( 38.42020198992004509, 8.283430712587435352, -77.41584236862877333 ) ) ;
#54659=CARTESIAN_POINT ( 'NONE',  ( -38.69408084385327840, 10.89529537250242619, 66.52660731830836482 ) ) ;
#54662=CARTESIAN_POINT ( 'NONE',  ( -7.825402957745083654, 6.891034867348166060, -50.41807073194384259 ) ) ;
#54663=DIRECTION ( 'NONE',  ( -0.000000000000000000, 1.000000000000000000, -0.000000000000000000 ) ) ;
#54665=CARTESIAN_POINT ( 'NONE',  ( -1.095583923122880332, 7.553030873957009561, -39.59844992052428836 ) ) ;
#54666=CARTESIAN_POINT ( 'NONE',  ( 109.3079614081140818, 28.45126415661783170, 17.72277496343515324 ) ) ;
#54667=CARTESIAN_POINT ( 'NONE',  ( -166.5704851812740230, 80.12110537694668722, 7.814510292449148743 ) ) ;
#54668=CARTESIAN_POINT ( 'NONE',  ( -82.32931163805224628, 23.75065981441939655, -49.16463154184398121 ) ) ;
#54669=FACE_BOUND ( 'NONE', #6550, .T. ) ;
#54671=CARTESIAN_POINT ( 'NONE',  ( 11.21387192505585872, 6.397095920409659797, -75.82701624946969332 ) ) ;
#54673=ORIENTED_EDGE ( 'NONE', *, *, #41535, .F. ) ;
#54677=CARTESIAN_POINT ( 'NONE',  ( -131.6133495896317243, 50.37677745548730712, -37.55590930492478208 ) ) ;
#54678=CARTESIAN_POINT ( 'NONE',  ( 44.86216938219159545, 9.182565662897470560, -75.11176578098715595 ) ) ;
#54684=ORIENTED_EDGE ( 'NONE', *, *, #9538, .F. ) ;
#54685=CARTESIAN_POINT ( 'NONE',  ( 15.78827728214693416, -170.0000000000000000, 18.17015708224157322 ) ) ;
#54691=CARTESIAN_POINT ( 'NONE',  ( 173.9288990958749821, 71.66475105971927917, -41.40298165088110238 ) ) ;
#54693=ORIENTED_EDGE ( 'NONE', *, *, #54829, .F. ) ;
#54695=CARTESIAN_POINT ( 'NONE',  ( -76.78936026062119424, 21.61552955137052123, -49.88070520349071302 ) ) ;
#54697=CARTESIAN_POINT ( 'NONE',  ( 22.57527834893889107, 6.812418720475017508, -93.40615590320534523 ) ) ;
#54698=CARTESIAN_POINT ( 'NONE',  ( -53.13788504024111603, 15.21566150156364650, -23.13923814719157335 ) ) ;
#54700=ORIENTED_EDGE ( 'NONE', *, *, #68617, .T. ) ;
#54701=CARTESIAN_POINT ( 'NONE',  ( -122.3745688183166180, 44.21964839958061333, -8.929199399706153173 ) ) ;
#54704=CARTESIAN_POINT ( 'NONE',  ( -143.8756912989386763, 60.83492035645721074, -37.35355894080970529 ) ) ;
#54705=EDGE_CURVE ( 'NONE', #32490, #34184, #68000, .T. ) ;
#54707=CARTESIAN_POINT ( 'NONE',  ( -128.7316684282232870, 48.39061963499592878, 84.86076366594872411 ) ) ;
#54710=ORIENTED_EDGE ( 'NONE', *, *, #33673, .F. ) ;
#54711=CARTESIAN_POINT ( 'NONE',  ( -133.3958821919893012, 51.63629593114585248, 37.60575035420465184 ) ) ;
#54712=VECTOR ( 'NONE', #46738, 1000.000000000000000 ) ;
#54716=CARTESIAN_POINT ( 'NONE',  ( 85.67452303415197434, 19.09699411916382417, -9.022822218913626457 ) ) ;
#54719=FACE_OUTER_BOUND ( 'NONE', #19063, .T. ) ;
#54721=CARTESIAN_POINT ( 'NONE',  ( -156.1706799718432421, 70.04375536285918713, -92.55028558477887657 ) ) ;
#54726=CARTESIAN_POINT ( 'NONE',  ( 13.84120792123769306, 6.445822122644894847, 30.25530662355467726 ) ) ;
#54730=CARTESIAN_POINT ( 'NONE',  ( 210.6592759200688079, 116.7161312026394597, -39.26769195576843430 ) ) ;
#54731=CARTESIAN_POINT ( 'NONE',  ( -71.17846906053300415, 20.67346400882179225, -69.95449947810095637 ) ) ;
#54734=CARTESIAN_POINT ( 'NONE',  ( -23.99924996210628336, 8.487987924059027023, -41.83754911040676916 ) ) ;
#54735=CARTESIAN_POINT ( 'NONE',  ( -190.6985136298601731, 109.1272424661242582, -19.71767969763411799 ) ) ;
#54738=ORIENTED_EDGE ( 'NONE', *, *, #17953, .F. ) ;
#54741=CARTESIAN_POINT ( 'NONE',  ( -81.90266786693713641, 23.58030232261292269, 71.54568514678170743 ) ) ;
#54742=CARTESIAN_POINT ( 'NONE',  ( 126.6266894765173419, 38.37986986668737899, 39.07338674164753201 ) ) ;
#54743=CARTESIAN_POINT ( 'NONE',  ( 32.15284246740099405, 8.588257691344878708, 12.50862876416052138 ) ) ;
#54747=CARTESIAN_POINT ( 'NONE',  ( 204.4450048848729011, 105.9958458039796341, 82.88260271150369363 ) ) ;
#54750=CARTESIAN_POINT ( 'NONE',  ( 59.72647370436681769, 12.96353798836696569, 70.90221448876295085 ) ) ;
#54751=CARTESIAN_POINT ( 'NONE',  ( 13.36262230781615479, 7.441298897118794109, -62.74979327901514381 ) ) ;
#54752=CARTESIAN_POINT ( 'NONE',  ( -13.29455179262032871, 8.319166883236663423, 5.633120552283173765 ) ) ;
#54758=CARTESIAN_POINT ( 'NONE',  ( -132.9109786433856755, 51.29129389542019624, 13.93605864163157726 ) ) ;
#54760=EDGE_CURVE ( 'NONE', #11797, #18819, #36708, .T. ) ;
#54762=CARTESIAN_POINT ( 'NONE',  ( -133.3316503378477478, 52.82738260200861902, -43.51700776321061426 ) ) ;
#54764=CARTESIAN_POINT ( 'NONE',  ( -118.6157340058430094, 41.88485941274768010, -40.58329878568739701 ) ) ;
#54765=CARTESIAN_POINT ( 'NONE',  ( -4.070918861171931802, 6.675509947362630925, -9.576274108367087479 ) ) ;
#54769=CARTESIAN_POINT ( 'NONE',  ( -2.869721780807578781, 7.625909776230886727, -64.11188747930218312 ) ) ;
#54771=ADVANCED_FACE ( 'NONE', ( #5024 ), #15593, .F. ) ;
#54774=ORIENTED_EDGE ( 'NONE', *, *, #42590, .F. ) ;
#54775=CARTESIAN_POINT ( 'NONE',  ( -59.57462349605619067, 16.98779896904799358, 4.969145654779915766 ) ) ;
#54776=CARTESIAN_POINT ( 'NONE',  ( 203.1420903260745945, 104.2307086582027154, -36.44445549019010855 ) ) ;
#54779=CARTESIAN_POINT ( 'NONE',  ( -97.49665543375859045, 31.53324358035376918, 43.81673036652279052 ) ) ;
#54780=CARTESIAN_POINT ( 'NONE',  ( 23.03578842369135771, 6.840884649289439956, -44.96429564819586489 ) ) ;
#54782=CARTESIAN_POINT ( 'NONE',  ( 117.7417271423230147, 33.63613196344608269, 10.80182121036862419 ) ) ;
#54788=CARTESIAN_POINT ( 'NONE',  ( -75.64857587248467041, 21.19501514561450506, -8.900704809817050034 ) ) ;
#54790=CYLINDRICAL_SURFACE ( 'NONE', #41655, 7.500000000000020428 ) ;
#54791=CARTESIAN_POINT ( 'NONE',  ( -13.77312480593389488, 8.361845410302544579, -74.33815112409169501 ) ) ;
#54792=ORIENTED_EDGE ( 'NONE', *, *, #47937, .F. ) ;
#54793=CARTESIAN_POINT ( 'NONE',  ( 162.1014732644455307, 61.34312237409763213, 42.82812415200849898 ) ) ;
#54797=CARTESIAN_POINT ( 'NONE',  ( -145.2564783699978079, 61.95220470181592987, -89.80724196599325637 ) ) ;
#54798=CARTESIAN_POINT ( 'NONE',  ( -38.54881010929333485, 10.86689971295294477, -13.53486305356366515 ) ) ;
#54799=B_SPLINE_CURVE_WITH_KNOTS ( 'NONE', 3,
 ( #52370, #47086, #18631, #15768, #64655, #26332, #4865, #47770, #57994, #55037, #36889, #63956, #63274, #27007, #42159, #36545, #37566, #58666, #69226, #21056, #31953, #37917, #59361, #31601, #42828, #43177, #16461, #21727, #272, #25991, #20699, #42502, #15083, #37215, #28310, #12146, #10832, #53731, #10484, #53383, #5214, #26673, #48435, #48108 ),
 .UNSPECIFIED., .F., .F.,
 ( 4, 2, 2, 2, 2, 2, 2, 2, 2, 2, 2, 2, 2, 2, 2, 2, 2, 2, 2, 2, 2, 4 ),
 ( 7.757919228897728493E-18, 0.003360573201437767454, 0.004200716501797173430, 0.005040859802156579840, 0.006721146402875345822, 0.007561289703234706262, 0.008401433003594062365, 0.009241576303953422805, 0.01008171960431278324, 0.01176200620503151974, 0.01260214950539088018, 0.01344229280575023888, 0.01428243610610959932, 0.01512257940646895803, 0.01680286600718770146, 0.01764300930754707578, 0.01848315260790645009, 0.02016343920862517791, 0.02184372580934390573, 0.02352401241006263355, 0.02520429901078136137, 0.02688458561150008919 ),
 .UNSPECIFIED. ) ;
#54800=CARTESIAN_POINT ( 'NONE',  ( -176.3856149167965555, 92.38076834121982017, 45.08818581386256596 ) ) ;
#54801=DIRECTION ( 'NONE',  ( -0.000000000000000000, 1.000000000000000000, -0.000000000000000000 ) ) ;
#54802=CARTESIAN_POINT ( 'NONE',  ( 22.90619343622340764, 7.840927939412484449, 61.94537535831524622 ) ) ;
#54804=ORIENTED_EDGE ( 'NONE', *, *, #22449, .T. ) ;
#54809=CARTESIAN_POINT ( 'NONE',  ( -34.74312654625182972, 10.15703162223800682, -49.55465837260248918 ) ) ;
#54813=CARTESIAN_POINT ( 'NONE',  ( -61.84115830117593759, 17.65779703603521256, 94.71171141969601592 ) ) ;
#54814=CARTESIAN_POINT ( 'NONE',  ( 79.38020582286196714, 17.07365509555548755, 62.06798524717918752 ) ) ;
#54815=EDGE_LOOP ( 'NONE', ( #10090, #49534, #50251, #33847 ) ) ;
#54820=CARTESIAN_POINT ( 'NONE',  ( 185.1647878987785987, 82.82967084668430857, 30.50037864223945405 ) ) ;
#54822=AXIS2_PLACEMENT_3D ( 'NONE', #68375, #26748, #14215 ) ;
#54823=CARTESIAN_POINT ( 'NONE',  ( -71.37402418445427088, 19.67651958824262692, 9.303105102284899175 ) ) ;
#54824=CARTESIAN_POINT ( 'NONE',  ( -118.8392474096542202, 43.20060570451234128, 62.36526549987367929 ) ) ;
#54825=CARTESIAN_POINT ( 'NONE',  ( -48.57297291660696459, 13.03920345822339044, 7.163779599053963665 ) ) ;
#54829=EDGE_CURVE ( 'NONE', #6792, #60434, #26145, .T. ) ;
#54830=CYLINDRICAL_SURFACE ( 'NONE', #39797, 7.500000000000013323 ) ;
#54833=CYLINDRICAL_SURFACE ( 'NONE', #45459, 7.500000000000020428 ) ;
#54835=EDGE_LOOP ( 'NONE', ( #42998, #24975, #7058, #42225 ) ) ;
#54836=CARTESIAN_POINT ( 'NONE',  ( -79.14127775978546708, 22.50259208414363599, 30.41820113967310490 ) ) ;
#54837=CARTESIAN_POINT ( 'NONE',  ( -24.32776401346968953, 9.546905915310571089, -67.22867289442208971 ) ) ;
#54838=CARTESIAN_POINT ( 'NONE',  ( 45.04020069093783007, 10.22779424730543063, 42.38369278573359367 ) ) ;
#54839=DIRECTION ( 'NONE',  ( -0.000000000000000000, 1.000000000000000000, -0.000000000000000000 ) ) ;
#54845=CARTESIAN_POINT ( 'NONE',  ( 32.29578462738145817, 8.602609172809795979, -13.86424321593882070 ) ) ;
#54848=CARTESIAN_POINT ( 'NONE',  ( -0.7211439451572413395, 7.539282923622935506, 66.87669417409435368 ) ) ;
#54851=LINE ( 'NONE', #1054, #14679 ) ;
#54852=ORIENTED_EDGE ( 'NONE', *, *, #62489, .T. ) ;
#54853=CARTESIAN_POINT ( 'NONE',  ( -119.2982054035571196, 42.30181775808006961, -72.83786828249223788 ) ) ;
#54854=ORIENTED_EDGE ( 'NONE', *, *, #34901, .F. ) ;
#54856=CARTESIAN_POINT ( 'NONE',  ( 164.9709596662455624, 63.72607097915132357, -16.51597377340664252 ) ) ;
#54859=CARTESIAN_POINT ( 'NONE',  ( 136.9654665832768217, 44.52067472585214603, 16.99517226826078797 ) ) ;
#54864=ORIENTED_EDGE ( 'NONE', *, *, #4360, .T. ) ;
#54868=CARTESIAN_POINT ( 'NONE',  ( 127.5843554582764057, 37.76388480628244793, -93.07977588763110077 ) ) ;
#54876=DIRECTION ( 'NONE',  ( 0.000000000000000000, 0.000000000000000000, 1.000000000000000000 ) ) ;
#54880=CARTESIAN_POINT ( 'NONE',  ( 32.66883187925818532, 8.640402022338106391, 34.07364008131894195 ) ) ;
#54881=CARTESIAN_POINT ( 'NONE',  ( -174.7817412490652202, 90.52199442492063497, -49.53788585594068650 ) ) ;
#54887=CARTESIAN_POINT ( 'NONE',  ( -147.1538409485623049, 63.51600817366544049, -76.28201582439264428 ) ) ;
#54889=FACE_BOUND ( 'NONE', #45580, .T. ) ;
#54890=CARTESIAN_POINT ( 'NONE',  ( -7.330690860789854213, 6.858814156830895570, -62.26262132240749025 ) ) ;
#54891=CARTESIAN_POINT ( 'NONE',  ( -180.5234362879040191, 97.35934147644944403, 66.41375281865778391 ) ) ;
#54893=CARTESIAN_POINT ( 'NONE',  ( -122.3759299995709853, 45.41285412136511468, -49.05442115285750759 ) ) ;
#54894=CARTESIAN_POINT ( 'NONE',  ( -0.3252226420479328306, 7.525368746738511305, 37.12884226405564903 ) ) ;
#54895=CARTESIAN_POINT ( 'NONE',  ( -11.84006471019700335, 7.185574865082572593, -90.25816456928032494 ) ) ;
#54897=CARTESIAN_POINT ( 'NONE',  ( -119.1605144823340652, 43.39823405392967715, -72.57201457058890526 ) ) ;
#54898=CARTESIAN_POINT ( 'NONE',  ( -14.84903512415885452, 8.461292896365067762, 40.25741089538951201 ) ) ;
#54899=CARTESIAN_POINT ( 'NONE',  ( 164.0298848570286907, 62.93631132702877551, 13.74007122767754652 ) ) ;
#54901=VERTEX_POINT ( 'NONE', #16272 ) ;
#54902=CARTESIAN_POINT ( 'NONE',  ( -35.99414836699283882, 11.40630460607619590, 4.893268811183970612 ) ) ;
#54906=CARTESIAN_POINT ( 'NONE',  ( 113.3877257111496846, 31.48076025743010931, 83.98386345913559126 ) ) ;
#54911=EDGE_CURVE ( 'NONE', #44954, #40902, #20141, .T. ) ;
#54916=CARTESIAN_POINT ( 'NONE',  ( 35.44311777160621091, 8.940232499250161169, 70.63318520892174490 ) ) ;
#54919=EDGE_CURVE ( 'NONE', #15010, #41004, #6417, .T. ) ;
#54928=CARTESIAN_POINT ( 'NONE',  ( 105.8229724512851817, 27.98935528750253710, -49.48651744878882397 ) ) ;
#54929=CARTESIAN_POINT ( 'NONE',  ( 23.24047374271772881, 7.861801299833791390, -42.03981132063025683 ) ) ;
#54930=CARTESIAN_POINT ( 'NONE',  ( -86.09999398724997377, 25.29376521564880420, -14.74247839810679572 ) ) ;
#54933=CARTESIAN_POINT ( 'NONE',  ( 211.5175447467296408, 116.1901475271413915, -13.84624472280481200 ) ) ;
#54934=FACE_BOUND ( 'NONE', #55750, .T. ) ;
#54936=CARTESIAN_POINT ( 'NONE',  ( -61.75629144857964548, 16.58190704077737720, -39.34366674388692786 ) ) ;
#54937=EDGE_CURVE ( 'NONE', #55648, #65743, #1486, .T. ) ;
#54942=CARTESIAN_POINT ( 'NONE',  ( -52.68206656346372796, 15.09776187114413482, 71.78146491162712550 ) ) ;
#54945=CARTESIAN_POINT ( 'NONE',  ( 154.4429418375333114, 55.33424769452795999, 3.188201469828449319 ) ) ;
#54947=ORIENTED_EDGE ( 'NONE', *, *, #56614, .F. ) ;
#54948=CARTESIAN_POINT ( 'NONE',  ( 57.08336938683662964, 11.37442068895388836, 15.08384692392094450 ) ) ;
#54951=ORIENTED_EDGE ( 'NONE', *, *, #5859, .F. ) ;
#54954=CARTESIAN_POINT ( 'NONE',  ( 107.0471828278921009, 27.43080724084234134, 43.91305964950614538 ) ) ;
#54957=EDGE_LOOP ( 'NONE', ( #31021, #20341, #38295, #24315 ) ) ;
#54961=CARTESIAN_POINT ( 'NONE',  ( 159.2258951716709987, 60.31399909112332125, 29.60431511090013856 ) ) ;
#54965=CARTESIAN_POINT ( 'NONE',  ( 70.11969827741711470, 15.47408882293424703, 12.92314886639808869 ) ) ;
#54967=CARTESIAN_POINT ( 'NONE',  ( -50.52615126106343268, 14.55080735582893325, -48.71601950317546681 ) ) ;
#54968=CARTESIAN_POINT ( 'NONE',  ( -48.23389383802711450, 13.99288361739331066, 7.839931237048672230 ) ) ;
#54969=CARTESIAN_POINT ( 'NONE',  ( -132.4896623150434039, 52.22616402022728721, -11.98991211083652075 ) ) ;
#54972=CARTESIAN_POINT ( 'NONE',  ( 85.04740456388582004, 18.88715044253751429, 83.56261749178500509 ) ) ;
#54979=CARTESIAN_POINT ( 'NONE',  ( -167.9514378334966977, 83.01160612846800291, 86.56910000124806004 ) ) ;
#54981=CARTESIAN_POINT ( 'NONE',  ( 109.7724924842966203, 28.66436020578543875, -9.077886975190001095 ) ) ;
#54982=CARTESIAN_POINT ( 'NONE',  ( -62.49137879463569334, 17.85440472148626867, -41.72647759500893727 ) ) ;
#54984=CARTESIAN_POINT ( 'NONE',  ( -71.17819443284074055, 19.60909329639479637, -68.96902843604570421 ) ) ;
#54985=LINE ( 'NONE', #49699, #57805 ) ;
#54991=CARTESIAN_POINT ( 'NONE',  ( 117.4727955442972984, 32.37277428084794906, 92.82555064614152229 ) ) ;
#54992=VECTOR ( 'NONE', #31890, 1000.000000000000000 ) ;
#54993=CARTESIAN_POINT ( 'NONE',  ( 117.7442255600443275, 33.63739995216997869, -17.07680329598102276 ) ) ;
#54995=CYLINDRICAL_SURFACE ( 'NONE', #30371, 7.500000000000013323 ) ;
#55003=CARTESIAN_POINT ( 'NONE',  ( 32.90878072717891456, 7.653588083204843073, -66.20281501231022503 ) ) ;
#55004=CARTESIAN_POINT ( 'NONE',  ( 57.39674746172460118, 11.43903079040059012, -11.38430605732729006 ) ) ;
#55006=CARTESIAN_POINT ( 'NONE',  ( -53.14475157111025538, 14.17819596930906201, 30.56003773838011739 ) ) ;
#55009=ORIENTED_EDGE ( 'NONE', *, *, #24586, .T. ) ;
#55010=CARTESIAN_POINT ( 'NONE',  ( 187.6511924654682275, 87.00187850361884045, 60.02042712270064584 ) ) ;
#55011=CARTESIAN_POINT ( 'NONE',  ( 177.7960900018544805, 75.34533826015463376, -63.82509446584703738 ) ) ;
#55015=CARTESIAN_POINT ( 'NONE',  ( -166.5686015187717999, 80.11916873959168583, 15.13637275916411973 ) ) ;
#55016=CARTESIAN_POINT ( 'NONE',  ( -79.14127775978546708, 22.50259208414362533, -50.11545063171792691 ) ) ;
#55027=CARTESIAN_POINT ( 'NONE',  ( 46.13856685535756696, 9.381502944822535994, -66.63088862529708933 ) ) ;
#55029=DIRECTION ( 'NONE',  ( -0.000000000000000000, 1.000000000000000000, -0.000000000000000000 ) ) ;
#55031=ORIENTED_EDGE ( 'NONE', *, *, #14460, .T. ) ;
#55033=CARTESIAN_POINT ( 'NONE',  ( 179.8066339122161708, 77.32395502108371943, 83.10161394449548311 ) ) ;
#55034=ORIENTED_EDGE ( 'NONE', *, *, #9122, .T. ) ;
#55036=CARTESIAN_POINT ( 'NONE',  ( 175.3815143714021474, 73.02838262206999786, -38.84691806896955057 ) ) ;
#55037=CARTESIAN_POINT ( 'NONE',  ( 162.6205203824432317, 63.07332653227189212, 15.52233856153403124 ) ) ;
#55040=CARTESIAN_POINT ( 'NONE',  ( 117.3246714514015565, 33.42485879931864901, 61.43420873138611427 ) ) ;
#55041=CARTESIAN_POINT ( 'NONE',  ( 138.5943620234098717, 45.55242290395135285, 58.02036038869290735 ) ) ;
#55042=CARTESIAN_POINT ( 'NONE',  ( -72.20490592113146988, 19.96451062593609649, -38.77557629329852062 ) ) ;
#55047=CARTESIAN_POINT ( 'NONE',  ( 88.30010642107259855, 19.99780058782973668, -36.00606560305973147 ) ) ;
#55048=CARTESIAN_POINT ( 'NONE',  ( -54.57263979903869711, 15.59415114099631872, -23.37177340799620495 ) ) ;
#55052=CARTESIAN_POINT ( 'NONE',  ( -125.8938041572051389, 46.49392987655490828, -8.069153307770243089 ) ) ;
#55053=CARTESIAN_POINT ( 'NONE',  ( -71.17984086584779391, 20.67393782512343137, 11.58859701068692871 ) ) ;
#55054=CARTESIAN_POINT ( 'NONE',  ( 42.03492317486905705, 8.766487167902370814, -50.14667375286791895 ) ) ;
#55056=CARTESIAN_POINT ( 'NONE',  ( -119.4574925226536237, 42.39917684031088640, 87.90653636692998418 ) ) ;
#55058=CARTESIAN_POINT ( 'NONE',  ( 55.64941047419414133, 12.11006143146460978, 11.94197868491970915 ) ) ;
#55061=CARTESIAN_POINT ( 'NONE',  ( -149.5074843970971017, 64.17983161892348676, 57.56537183036274996 ) ) ;
#55062=DIRECTION ( 'NONE',  ( 0.000000000000000000, 0.000000000000000000, 1.000000000000000000 ) ) ;
#55064=CARTESIAN_POINT ( 'NONE',  ( 181.9295719569815049, 79.46350097013164770, -24.34495040295407620 ) ) ;
#55065=CARTESIAN_POINT ( 'NONE',  ( 140.2332932573541768, 45.41010019581507606, -12.69871729523817727 ) ) ;
#55067=CARTESIAN_POINT ( 'NONE',  ( 92.51858280840787074, 21.51505926344916730, -74.83681589150050684 ) ) ;
#55068=CARTESIAN_POINT ( 'NONE',  ( -29.34031752350706412, 9.255998326330892922, -89.29320561667297795 ) ) ;
#55069=CARTESIAN_POINT ( 'NONE',  ( -54.08816720029309977, 15.46531105893042302, 45.27054875321893945 ) ) ;
#55073=CARTESIAN_POINT ( 'NONE',  ( 197.2200752504831769, 96.62072041958363400, -16.31714441260212212 ) ) ;
#55075=CARTESIAN_POINT ( 'NONE',  ( -190.0468231512975308, 108.2116162189844459, 61.86802075691926461 ) ) ;
#55077=CARTESIAN_POINT ( 'NONE',  ( 211.3757499519976761, 117.8130818709823586, -40.40091158434037055 ) ) ;
#55079=LINE ( 'NONE', #39270, #66350 ) ;
#55080=CARTESIAN_POINT ( 'NONE',  ( -29.02794087136069123, 9.207646203414331154, -35.69869208938506944 ) ) ;
#55085=CARTESIAN_POINT ( 'NONE',  ( 86.62931800182293784, 19.42108912189598158, 2.867536982015618019 ) ) ;
#55086=EDGE_CURVE ( 'NONE', #32665, #2286, #20878, .T. ) ;
#55089=CARTESIAN_POINT ( 'NONE',  ( 131.3924949472282719, 41.12442122814098866, 29.92295193858798186 ) ) ;
#55093=CARTESIAN_POINT ( 'NONE',  ( -95.52093927227217307, 30.58993121475388577, -12.40980231041914195 ) ) ;
#55095=CARTESIAN_POINT ( 'NONE',  ( 210.9858733471680239, 115.3838960844459933, 86.29496074341011536 ) ) ;
#55100=CARTESIAN_POINT ( 'NONE',  ( -11.79249160485393588, 8.191429102467035150, 17.14070543632877275 ) ) ;
#55101=EDGE_CURVE ( 'NONE', #42689, #28520, #47158, .T. ) ;
#55104=EDGE_CURVE ( 'NONE', #55930, #19164, #5295, .T. ) ;
#55105=CARTESIAN_POINT ( 'NONE',  ( -94.95309908913763763, 29.21194990959874360, -94.53409306187226946 ) ) ;
#55106=ADVANCED_FACE ( 'NONE', ( #63352 ), #68622, .F. ) ;
#55107=EDGE_CURVE ( 'NONE', #68773, #62204, #8311, .T. ) ;
#55112=CARTESIAN_POINT ( 'NONE',  ( -131.1078488676299116, 50.02394948559178545, 16.67182174600359801 ) ) ;
#55113=CARTESIAN_POINT ( 'NONE',  ( -166.5742238910466426, 81.57147158222491612, -45.88140790838662042 ) ) ;
#55115=CARTESIAN_POINT ( 'NONE',  ( -172.2786706323828696, 86.19570483525345139, 84.55397788683201554 ) ) ;
#55117=CARTESIAN_POINT ( 'NONE',  ( -122.8118341587044853, 44.49743491855736721, -49.26647034107312351 ) ) ;
#55119=CARTESIAN_POINT ( 'NONE',  ( -149.0782809666403637, 63.81577337591402710, -22.96827994102829962 ) ) ;
#55120=CARTESIAN_POINT ( 'NONE',  ( -1.328627985309862591, 7.561890325089885678, -73.51797458872181323 ) ) ;
#55121=CARTESIAN_POINT ( 'NONE',  ( -125.8938041572051105, 46.49392987655492959, 3.775397282693376599 ) ) ;
#55123=CARTESIAN_POINT ( 'NONE',  ( 164.5345649067969021, 64.67444685591088671, -94.78372339538049118 ) ) ;
#55125=CARTESIAN_POINT ( 'NONE',  ( -102.2801239173131052, 33.91021738430207932, 30.51907450641510522 ) ) ;
#55126=CARTESIAN_POINT ( 'NONE',  ( 19.54475376904848005, 6.649964688461123430, -36.52285208494490121 ) ) ;
#55127=CARTESIAN_POINT ( 'NONE',  ( -55.53469534616550618, 14.81076603075803888, 3.472777182467473356 ) ) ;
#55131=ORIENTED_EDGE ( 'NONE', *, *, #29785, .F. ) ;
#55133=CARTESIAN_POINT ( 'NONE',  ( 176.6238742729555327, 75.60943990211369226, 30.76015344212299851 ) ) ;
#55134=DIRECTION ( 'NONE',  ( -0.000000000000000000, 1.000000000000000000, -0.000000000000000000 ) ) ;
#55135=CARTESIAN_POINT ( 'NONE',  ( -14.56151485655250255, 8.434196591921343966, -73.09670765900315814 ) ) ;
#55137=CARTESIAN_POINT ( 'NONE',  ( 159.2319614735955895, 59.03334608081210177, 29.60582811906876799 ) ) ;
#55143=CARTESIAN_POINT ( 'NONE',  ( -143.3273709291075875, 60.39554735433492993, -91.72452606276587517 ) ) ;
#55145=CARTESIAN_POINT ( 'NONE',  ( -36.37371824399144060, 10.45334302951138206, -21.64224812475993431 ) ) ;
#55147=CARTESIAN_POINT ( 'NONE',  ( -133.2787743207940991, 52.78950725740546090, 12.61127779455901710 ) ) ;
#55148=CARTESIAN_POINT ( 'NONE',  ( -102.2801239173131194, 33.91021738430207932, -61.85912785543958847 ) ) ;
#55153=CARTESIAN_POINT ( 'NONE',  ( 208.3164187557410116, 111.4385528447316318, -90.93565301021618552 ) ) ;
#55157=CARTESIAN_POINT ( 'NONE',  ( -37.92511097250854846, 10.74631978746601213, -39.04328897955974753 ) ) ;
#55158=CARTESIAN_POINT ( 'NONE',  ( -103.7931824998358792, 33.55607161175042563, 84.35638170082560805 ) ) ;
#55159=CARTESIAN_POINT ( 'NONE',  ( -144.2188519266539970, 59.82027639618910797, 32.89713914446858922 ) ) ;
#55160=EDGE_CURVE ( 'NONE', #43438, #2040, #60142, .T. ) ;
#55161=CARTESIAN_POINT ( 'NONE',  ( -133.3392045760936355, 51.59583146030204404, 63.91024170815089178 ) ) ;
#55162=CARTESIAN_POINT ( 'NONE',  ( -73.80418150970712077, 21.59712875466423299, -21.50274857840328124 ) ) ;
#55169=CARTESIAN_POINT ( 'NONE',  ( 63.01563776193091826, -170.0000000000000000, 37.31296093922129131 ) ) ;
#55174=CARTESIAN_POINT ( 'NONE',  ( 38.90894112122322923, 8.345444037631242651, 18.06928371549960488 ) ) ;
#55176=CARTESIAN_POINT ( 'NONE',  ( -49.14234466229832776, 13.17605306081206251, 6.349177895488338663 ) ) ;
#55177=CARTESIAN_POINT ( 'NONE',  ( 149.9838583332408177, 52.05699766415859386, -44.15268191325389324 ) ) ;
#55178=CARTESIAN_POINT ( 'NONE',  ( 158.3516718297675823, 59.61984652322049527, -77.92999794994581464 ) ) ;
#55180=CARTESIAN_POINT ( 'NONE',  ( -109.1685085742250294, 36.41998174028086765, -93.20135381603594737 ) ) ;
#55187=CARTESIAN_POINT ( 'NONE',  ( -82.53770812813168334, 23.83403279300014077, 31.49003151132006550 ) ) ;
#55188=CARTESIAN_POINT ( 'NONE',  ( -8.320652113663527416, 6.923290556636831461, -62.26262132240749025 ) ) ;
#55189=CARTESIAN_POINT ( 'NONE',  ( 46.89016064832838993, 10.52130577388959587, 36.92564426630246288 ) ) ;
#55196=ORIENTED_EDGE ( 'NONE', *, *, #70, .F. ) ;
#55197=CARTESIAN_POINT ( 'NONE',  ( 31.96192885395476679, 8.569232728322420556, -15.29726466815624697 ) ) ;
#55201=CARTESIAN_POINT ( 'NONE',  ( 137.2367873612328424, 44.69120782157546756, 83.99673694943189162 ) ) ;
#55203=CARTESIAN_POINT ( 'NONE',  ( 200.5149448373513508, 102.4289237596961044, -91.27880272729396438 ) ) ;
#55211=CARTESIAN_POINT ( 'NONE',  ( 163.7607557204680404, 62.71181783708028235, -12.66404714983320368 ) ) ;
#55214=CARTESIAN_POINT ( 'NONE',  ( 141.2811136745703777, 46.09188267874204570, -71.46311027019235951 ) ) ;
#55223=CARTESIAN_POINT ( 'NONE',  ( -149.5074843970971301, 64.17983161892345834, -76.65738112195568021 ) ) ;
#55224=CARTESIAN_POINT ( 'NONE',  ( 93.92910382125421620, 22.04227458821882379, 12.10717395489050929 ) ) ;
#55230=CARTESIAN_POINT ( 'NONE',  ( 64.94098077424391136, 14.16208887966257457, 30.04812862234404491 ) ) ;
#55231=CARTESIAN_POINT ( 'NONE',  ( -133.2698123908828620, 51.54642138335022139, -14.18505733217823561 ) ) ;
#55233=CARTESIAN_POINT ( 'NONE',  ( 130.7531879853686405, 39.58149302537893277, -63.52440237893536334 ) ) ;
#55239=DIRECTION ( 'NONE',  ( -0.8160245890732938934, -0.5780171883497599028, 0.000000000000000000 ) ) ;
#55240=CYLINDRICAL_SURFACE ( 'NONE', #62381, 7.500000000000013323 ) ;
#55241=CARTESIAN_POINT ( 'NONE',  ( -37.93379515072632557, 11.77251734620211643, 33.93346572377289050 ) ) ;
#55243=CARTESIAN_POINT ( 'NONE',  ( -144.2038301586456726, 61.09856042007388055, -20.79348971481011432 ) ) ;
#55247=CARTESIAN_POINT ( 'NONE',  ( -47.61380558691494969, 12.81230778489788058, -68.57384386193655246 ) ) ;
#55253=CARTESIAN_POINT ( 'NONE',  ( 164.3702714028688945, 63.22112480708620552, 13.01656737544070452 ) ) ;
#55254=CARTESIAN_POINT ( 'NONE',  ( 46.68054346512387554, 10.48734223171576829, -95.00000000000133582 ) ) ;
#55256=CARTESIAN_POINT ( 'NONE',  ( -99.10904156412040322, 32.31949011661295401, -35.70134815719908516 ) ) ;
#55261=LINE ( 'NONE', #38389, #2880 ) ;
#55262=CARTESIAN_POINT ( 'NONE',  ( 40.38414441725701209, 8.538832720399533116, 71.71009557933999190 ) ) ;
#55270=ORIENTED_EDGE ( 'NONE', *, *, #57210, .T. ) ;
#55272=DIRECTION ( 'NONE',  ( 0.000000000000000000, 0.000000000000000000, 1.000000000000000000 ) ) ;
#55273=CARTESIAN_POINT ( 'NONE',  ( 173.9288990958749537, 71.66475105971926496, 65.97522071097360197 ) ) ;
#55276=DIRECTION ( 'NONE',  ( -0.000000000000000000, 1.000000000000000000, -0.000000000000000000 ) ) ;
#55280=CARTESIAN_POINT ( 'NONE',  ( 105.7953515382196201, 27.97683113100023533, -37.36414706739255109 ) ) ;
#55281=CARTESIAN_POINT ( 'NONE',  ( 23.04797191264875522, 7.849755664016355716, -44.96511804298085480 ) ) ;
#55283=CARTESIAN_POINT ( 'NONE',  ( -55.05276343752910151, -170.0000000000000000, 37.81732777293115078 ) ) ;
#55285=FACE_BOUND ( 'NONE', #58959, .T. ) ;
#55286=CARTESIAN_POINT ( 'NONE',  ( 159.6614743841975042, 60.66237087206236822, 56.56722943839550055 ) ) ;
#55297=B_SPLINE_CURVE_WITH_KNOTS ( 'NONE', 3,
 ( #36169, #41103, #15403, #47393, #14019, #25629, #47063, #51659, #57966, #19640, #9096, #68850, #63249, #36513, #15059, #24928, #46361, #62562, #4839, #31247, #14374, #52677, #30545, #25280, #4502, #42131, #63594, #36862, #58303, #46718, #57629, #16772, #11846, #54396, #32615, #63933, #11150, #31929, #59337, #6218, #16082, #27674, #43499 ),
 .UNSPECIFIED., .F., .F.,
 ( 4, 2, 2, 2, 2, 2, 2, 2, 2, 2, 2, 2, 1, 2, 2, 2, 2, 2, 2, 2, 2, 4 ),
 ( 0.02362927190606132349, 0.02510248541563189772, 0.02583909217041719178, 0.02657569892520248236, 0.02804891243477306700, 0.02952212594434364817, 0.03025873269912893876, 0.03099533945391423281, 0.03246855296348481745, 0.03394176647305539862, 0.03541497998262597979, 0.03615158673741127038, 0.03688819349219656096, 0.03762480024698185155, 0.03836140700176714213, 0.03983462051133771636, 0.04130783402090829060, 0.04278104753047886483, 0.04351765428526414847, 0.04425426104004943906, 0.04572747454962002023, 0.04720068805919060140 ),
 .UNSPECIFIED. ) ;
#55299=DIRECTION ( 'NONE',  ( 0.000000000000000000, -1.000000000000000000, 0.000000000000000000 ) ) ;
#55305=CARTESIAN_POINT ( 'NONE',  ( -59.57462349605615515, 16.98779896904799358, -21.87540493568376831 ) ) ;
#55306=CARTESIAN_POINT ( 'NONE',  ( 93.72687053612526142, 23.04134601640627622, -72.64113259414895651 ) ) ;
#55310=CARTESIAN_POINT ( 'NONE',  ( 41.33434189587761409, 9.684413566891869607, 71.50931503011094037 ) ) ;
#55312=CARTESIAN_POINT ( 'NONE',  ( 104.7227067006896561, 27.50728936118537149, 5.166247656402080501 ) ) ;
#55313=CARTESIAN_POINT ( 'NONE',  ( 63.01563776193091826, 13.70579113808096849, 17.96841034875761878 ) ) ;
#55316=EDGE_CURVE ( 'NONE', #22488, #55692, #47779, .T. ) ;
#55317=CARTESIAN_POINT ( 'NONE',  ( -48.34500911884041585, 14.01939034823941554, 14.33699677132702099 ) ) ;
#55318=CARTESIAN_POINT ( 'NONE',  ( -132.8257891167039304, 52.46553896898735303, -12.69414959889051886 ) ) ;
#55319=CARTESIAN_POINT ( 'NONE',  ( -151.5161158480891856, 67.23556208791072208, -88.76439689521589571 ) ) ;
#55320=CARTESIAN_POINT ( 'NONE',  ( 115.7561705820729117, 31.51689401996056361, -21.68569513149070715 ) ) ;
#55321=CARTESIAN_POINT ( 'NONE',  ( -55.05276343752910151, -170.0000000000000000, -50.21632399845989170 ) ) ;
#55323=VERTEX_POINT ( 'NONE', #67518 ) ;
#55324=VERTEX_POINT ( 'NONE', #55562 ) ;
#55326=CARTESIAN_POINT ( 'NONE',  ( -9.763294602873862971, 7.024900256480052896, -8.824033836334688630 ) ) ;
#55328=CARTESIAN_POINT ( 'NONE',  ( -47.80896875121165834, 12.85816703949531004, -13.91236320614654964 ) ) ;
#55329=CARTESIAN_POINT ( 'NONE',  ( 103.5839822277949906, 25.92130892112108853, -13.11793987809817885 ) ) ;
#55331=CARTESIAN_POINT ( 'NONE',  ( -35.17718245314462422, 11.25729435722175609, 71.06764365538327866 ) ) ;
#55333=CARTESIAN_POINT ( 'NONE',  ( 157.4703587214989398, -170.0000000000000000, 56.25401806271706562 ) ) ;
#55335=CARTESIAN_POINT ( 'NONE',  ( -8.807541152391516803, 6.956521193351524524, 45.06700915991218181 ) ) ;
#55341=CIRCLE ( 'NONE', #50836, 242.4895526022646379 ) ;
#55342=CARTESIAN_POINT ( 'NONE',  ( -172.3038663181179970, 87.72015621195187407, 45.82169460664105998 ) ) ;
#55346=CARTESIAN_POINT ( 'NONE',  ( -103.2129897037410728, 33.25684593987699600, 18.63071618642112881 ) ) ;
#55356=VECTOR ( 'NONE', #34761, 1000.000000000000000 ) ;
#55357=CARTESIAN_POINT ( 'NONE',  ( 55.61382797299288683, 11.07686102552914953, -17.61099702755072371 ) ) ;
#55360=CARTESIAN_POINT ( 'NONE',  ( -49.62489392740899774, 13.29305723289026275, 32.63583538682032525 ) ) ;
#55363=ADVANCED_FACE ( 'NONE', ( #3839 ), #62589, .F. ) ;
#55366=CARTESIAN_POINT ( 'NONE',  ( 197.6329787101073805, 98.74106466892197886, -73.20637281266709806 ) ) ;
#55367=CARTESIAN_POINT ( 'NONE',  ( -3.862560291631544906, 7.672660553664872651, -49.29031988421443344 ) ) ;
#55368=CARTESIAN_POINT ( 'NONE',  ( 103.0026233023292974, 25.67408295205787994, 8.243349890369009003 ) ) ;
#55369=CARTESIAN_POINT ( 'NONE',  ( -165.6754884515988522, 79.20562145685592270, -95.00000000000133582 ) ) ;
#55371=FACE_BOUND ( 'NONE', #58758, .T. ) ;
#55375=CARTESIAN_POINT ( 'NONE',  ( -133.3926783185151521, 51.63401075114363437, -68.95695763348717833 ) ) ;
#55376=CARTESIAN_POINT ( 'NONE',  ( 8.000000000000007105, 249.8719672152120381, 94.99999999999866418 ) ) ;
#55380=CARTESIAN_POINT ( 'NONE',  ( 8.000000000000007105, 249.8719672152120381, 94.99999999999866418 ) ) ;
#55381=CARTESIAN_POINT ( 'NONE',  ( 175.3026482967971162, 72.95361582193056904, 85.70764415495648336 ) ) ;
#55382=ORIENTED_EDGE ( 'NONE', *, *, #9367, .T. ) ;
#55384=CARTESIAN_POINT ( 'NONE',  ( 175.5406524085945819, 73.17873692326776336, -48.80246454543877377 ) ) ;
#55385=CARTESIAN_POINT ( 'NONE',  ( 150.9013375937531407, 53.96275732797612079, 40.53801543753266401 ) ) ;
#55387=ORIENTED_EDGE ( 'NONE', *, *, #44878, .T. ) ;
#55389=CARTESIAN_POINT ( 'NONE',  ( -178.5790738944854184, 93.41591512785082330, 16.62680291879139105 ) ) ;
#55390=CARTESIAN_POINT ( 'NONE',  ( -76.31381168750411348, 21.43908608416557371, -35.47797508748302420 ) ) ;
#55393=CARTESIAN_POINT ( 'NONE',  ( 19.05389411040262004, 6.625946609665808396, -89.90362069605247086 ) ) ;
#55395=CARTESIAN_POINT ( 'NONE',  ( -51.77779688167514394, 14.86590802019197355, -22.62338495236307878 ) ) ;
#55401=EDGE_CURVE ( 'NONE', #51654, #47113, #44423, .T. ) ;
#55405=DIRECTION ( 'NONE',  ( -0.000000000000000000, 1.000000000000000000, -0.000000000000000000 ) ) ;
#55406=CARTESIAN_POINT ( 'NONE',  ( 56.67004931728209982, 12.31690113431407951, 94.99999999999866418 ) ) ;
#55408=CARTESIAN_POINT ( 'NONE',  ( 81.04675113612954362, 17.59091904316106891, -38.28904491945431943 ) ) ;
#55411=CYLINDRICAL_SURFACE ( 'NONE', #39141, 7.500000000000020428 ) ;
#55414=ADVANCED_FACE ( 'NONE', ( #65254 ), #7575, .F. ) ;
#55415=CARTESIAN_POINT ( 'NONE',  ( 93.08073375333744082, 22.79826000593201840, 33.37906321384794950 ) ) ;
#55417=CARTESIAN_POINT ( 'NONE',  ( -122.8118341587044853, 44.49743491855734590, 58.11173202078160216 ) ) ;
#55420=CARTESIAN_POINT ( 'NONE',  ( -156.7398303041269116, 70.56491326691592292, -93.95181625296153527 ) ) ;
#55421=ORIENTED_EDGE ( 'NONE', *, *, #62514, .T. ) ;
#55424=CARTESIAN_POINT ( 'NONE',  ( 46.90141780929663895, 9.503798448769780194, 36.90919837786481850 ) ) ;
#55426=CARTESIAN_POINT ( 'NONE',  ( 157.9130201331580565, 57.99550255803045928, 56.25401806271705851 ) ) ;
#55428=LINE ( 'NONE', #1989, #4124 ) ;
#55431=CARTESIAN_POINT ( 'NONE',  ( -27.48703802937313512, 8.975952825337596863, -36.43818875052794226 ) ) ;
#55432=CARTESIAN_POINT ( 'NONE',  ( 164.4615316623335275, 63.29763980349834185, -73.19771330824563904 ) ) ;
#55433=ORIENTED_EDGE ( 'NONE', *, *, #63842, .T. ) ;
#55436=CARTESIAN_POINT ( 'NONE',  ( -79.30552041445847067, 22.56523793503362896, 84.10971841195282650 ) ) ;
#55437=CARTESIAN_POINT ( 'NONE',  ( -86.15275984831843914, 25.31588180512571995, 65.28274353219886450 ) ) ;
#55441=CARTESIAN_POINT ( 'NONE',  ( -94.77890319529971919, 30.24118571794803145, -16.17010367493866596 ) ) ;
#55446=CARTESIAN_POINT ( 'NONE',  ( 62.04382205963241148, 13.48099884269679549, 44.76576134482495206 ) ) ;
#55447=CARTESIAN_POINT ( 'NONE',  ( 36.82834578791594993, 8.088597268192994960, 84.05056018580073385 ) ) ;
#55449=ORIENTED_EDGE ( 'NONE', *, *, #55160, .T. ) ;
#55453=ADVANCED_FACE ( 'NONE', ( #60672 ), #2291, .T. ) ;
#55456=CARTESIAN_POINT ( 'NONE',  ( -105.8879439778144729, 34.65133284149107595, -75.95163754952972113 ) ) ;
#55458=CARTESIAN_POINT ( 'NONE',  ( -96.30817042286538765, 29.84904329666579059, -91.64453525374615595 ) ) ;
#55464=CARTESIAN_POINT ( 'NONE',  ( -38.69449158134469968, 11.92067517118074527, -44.77975842212855184 ) ) ;
#55467=CARTESIAN_POINT ( 'NONE',  ( -166.1022426123342655, 79.64087030515175059, 94.67701969901513337 ) ) ;
#55469=CARTESIAN_POINT ( 'NONE',  ( -118.8504142000305421, 42.02789424825281372, -39.82313612425161864 ) ) ;
#55471=CARTESIAN_POINT ( 'NONE',  ( -144.7571537022064376, 60.25265659240449168, -21.27708794859261943 ) ) ;
#55472=CARTESIAN_POINT ( 'NONE',  ( -5.888165822225384538, 7.780336669456523246, -62.51295767058608277 ) ) ;
#55474=DIRECTION ( 'NONE',  ( 0.000000000000000000, 0.000000000000000000, 1.000000000000000000 ) ) ;
#55476=CARTESIAN_POINT ( 'NONE',  ( 157.4703587214989113, 58.92748579479259519, -89.81328548006499091 ) ) ;
#55477=CARTESIAN_POINT ( 'NONE',  ( 86.14890207173844772, 20.31981596387579714, 17.86753698201564688 ) ) ;
#55479=CARTESIAN_POINT ( 'NONE',  ( 20.36314374176838271, 6.689939636827348934, -48.98252730634334995 ) ) ;
#55481=ORIENTED_EDGE ( 'NONE', *, *, #3440, .F. ) ;
#55482=CARTESIAN_POINT ( 'NONE',  ( 55.76298701799387914, 11.10663440745151576, 39.28782614698545927 ) ) ;
#55485=CARTESIAN_POINT ( 'NONE',  ( -123.8527606835264550, 45.16425545704599642, -88.87375819088765638 ) ) ;
#55487=CARTESIAN_POINT ( 'NONE',  ( -36.49774120431530378, 11.49988540678358895, -90.95249728063662076 ) ) ;
#55489=CARTESIAN_POINT ( 'NONE',  ( -14.33060720034882962, 8.412649192293178757, -73.52734388806258892 ) ) ;
#55495=ORIENTED_EDGE ( 'NONE', *, *, #1847, .F. ) ;
#55496=CARTESIAN_POINT ( 'NONE',  ( 176.4131312624861891, 75.40601160939048953, -91.53289336470793103 ) ) ;
#55497=EDGE_CURVE ( 'NONE', #58864, #36637, #49390, .T. ) ;
#55504=CARTESIAN_POINT ( 'NONE',  ( 21.75198946226450758, 7.772524967554916842, 59.78508500779173573 ) ) ;
#55505=ORIENTED_EDGE ( 'NONE', *, *, #3110, .F. ) ;
#55508=ORIENTED_EDGE ( 'NONE', *, *, #42505, .F. ) ;
#55512=CARTESIAN_POINT ( 'NONE',  ( -33.84080342750782222, 9.997552308299095358, -49.93905837052822250 ) ) ;
#55513=CARTESIAN_POINT ( 'NONE',  ( -97.57502601200189929, 30.45419729933975361, 85.85939687630843764 ) ) ;
#55514=CARTESIAN_POINT ( 'NONE',  ( -145.5261806899006558, 60.87473129144525075, 31.86056720367915673 ) ) ;
#55515=CARTESIAN_POINT ( 'NONE',  ( -132.2352756077771119, 50.81350938245626736, 60.95178715509886302 ) ) ;
#55516=CARTESIAN_POINT ( 'NONE',  ( -76.10382222627278281, 22.43453174720079346, -8.718168199828413734 ) ) ;
#55518=CARTESIAN_POINT ( 'NONE',  ( 79.14129363775928994, 17.00055658855362850, 63.56359600498407048 ) ) ;
#55520=CARTESIAN_POINT ( 'NONE',  ( 32.14349651933087415, 7.576119504381656711, 35.46268199549083988 ) ) ;
#55523=FACE_OUTER_BOUND ( 'NONE', #20116, .T. ) ;
#55525=CARTESIAN_POINT ( 'NONE',  ( -119.5404913382139824, 43.63271406506959949, 60.97046577758045771 ) ) ;
#55526=CARTESIAN_POINT ( 'NONE',  ( -52.45215874217871033, 13.99961488531757858, 3.933950466555594883 ) ) ;
#55527=CARTESIAN_POINT ( 'NONE',  ( 153.4268936273268196, 54.57409659828383042, -49.94518735799756826 ) ) ;
#55529=ORIENTED_EDGE ( 'NONE', *, *, #10309, .F. ) ;
#55530=CARTESIAN_POINT ( 'NONE',  ( -103.9519010518735911, 33.63790860794365045, -88.88018785531716048 ) ) ;
#55531=CARTESIAN_POINT ( 'NONE',  ( -153.7005182577090068, 67.81869626254727734, -9.233257554413990320 ) ) ;
#55533=DIRECTION ( 'NONE',  ( 0.000000000000000000, 0.000000000000000000, 1.000000000000000000 ) ) ;
#55537=EDGE_LOOP ( 'NONE', ( #37075, #3343, #20638, #7278 ) ) ;
#55538=CARTESIAN_POINT ( 'NONE',  ( -86.15275984831842493, 25.31588180512566666, 38.43819294173514578 ) ) ;
#55539=CARTESIAN_POINT ( 'NONE',  ( 149.9714610887121466, 53.28792066194169763, -70.77614368036395831 ) ) ;
#55540=CARTESIAN_POINT ( 'NONE',  ( 41.80869235728135891, 9.750404582811610155, 30.29359847640873227 ) ) ;
#55541=CARTESIAN_POINT ( 'NONE',  ( 140.5781926063689298, 45.63383190293699698, -46.86065139210757025 ) ) ;
#55543=ORIENTED_EDGE ( 'NONE', *, *, #63973, .T. ) ;
#55544=( NAMED_UNIT ( * ) PLANE_ANGLE_UNIT ( ) SI_UNIT ( $, .RADIAN. ) );
#55547=CARTESIAN_POINT ( 'NONE',  ( 38.42095780754792145, 9.297684251045556181, -8.823390837636260642 ) ) ;
#55550=CARTESIAN_POINT ( 'NONE',  ( -1.327237339234996538, 7.561837009978232160, 14.52392135664211636 ) ) ;
#55560=CARTESIAN_POINT ( 'NONE',  ( 164.9697211531230039, 63.72502658717166213, -17.07644040156450416 ) ) ;
#55562=CARTESIAN_POINT ( 'NONE',  ( 211.7634543339367781, 118.4123239814494610, -95.00000000000133582 ) ) ;
#55563=CARTESIAN_POINT ( 'NONE',  ( 139.7928618793172859, 45.12615179300590285, -65.77714084613532464 ) ) ;
#55570=CYLINDRICAL_SURFACE ( 'NONE', #35118, 7.500000000000013323 ) ;
#55577=CARTESIAN_POINT ( 'NONE',  ( 93.09528872995973359, 21.72934119836186184, 14.19978795179650710 ) ) ;
#55578=CARTESIAN_POINT ( 'NONE',  ( 164.8471526211111495, 63.62172173173271972, -42.24226993237041938 ) ) ;
#55581=CARTESIAN_POINT ( 'NONE',  ( 56.17775956989186881, 12.21653819234432703, 87.90252147785352577 ) ) ;
#55584=CARTESIAN_POINT ( 'NONE',  ( -180.6215424137752166, 97.48070480470860844, -41.90601408175744069 ) ) ;
#55585=CARTESIAN_POINT ( 'NONE',  ( -126.3458714439411921, 46.79154809309481777, -23.06915330777030348 ) ) ;
#55586=CARTESIAN_POINT ( 'NONE',  ( 154.0401952541423327, 55.03227529428313147, 70.42760438175315585 ) ) ;
#55589=ORIENTED_EDGE ( 'NONE', *, *, #25969, .F. ) ;
#55590=CARTESIAN_POINT ( 'NONE',  ( 139.7883986595928434, 46.32091287009614433, -74.96433037504790775 ) ) ;
#55595=CARTESIAN_POINT ( 'NONE',  ( -149.7268278745401346, 65.68859631971237434, -49.81283053149198992 ) ) ;
#55596=CARTESIAN_POINT ( 'NONE',  ( 209.6698611676811481, 115.2210955123518517, -11.34831209349323267 ) ) ;
#55599=CARTESIAN_POINT ( 'NONE',  ( -31.92572261726339633, 10.69135962481465185, 30.21645440618915046 ) ) ;
#55600=CARTESIAN_POINT ( 'NONE',  ( -171.4867114763004849, 85.32693843184998173, -49.54345430716655585 ) ) ;
#55601=CARTESIAN_POINT ( 'NONE',  ( -7.330587818645181386, 7.867004275019547244, 45.11558103944723541 ) ) ;
#55604=CARTESIAN_POINT ( 'NONE',  ( -0.5178428571329629637, 7.532057582089302983, -14.36748065752867909 ) ) ;
#55606=CARTESIAN_POINT ( 'NONE',  ( 114.6890011751075917, 30.99337387307411973, 16.32607591214094356 ) ) ;
#55607=CARTESIAN_POINT ( 'NONE',  ( -55.05276343752910151, 15.72344139423345588, -88.90542517938717992 ) ) ;
#55609=CARTESIAN_POINT ( 'NONE',  ( -97.49665543375861887, 31.53324358035377983, -36.71692140486827327 ) ) ;
#55612=CARTESIAN_POINT ( 'NONE',  ( 110.2429982417149432, 28.88204397445228722, -62.76698815611734972 ) ) ;
#55613=CARTESIAN_POINT ( 'NONE',  ( 46.12611922993085756, 10.39838587005582227, -19.60643483645174356 ) ) ;
#55614=CARTESIAN_POINT ( 'NONE',  ( 46.85206196242843646, 9.495795933269468136, 63.26480904775041836 ) ) ;
#55618=CARTESIAN_POINT ( 'NONE',  ( 62.60807349995172189, 13.61084778855394184, -89.40979201309710334 ) ) ;
#55625=CARTESIAN_POINT ( 'NONE',  ( -168.7329347389696181, 83.83901812802760389, 59.06544427237531636 ) ) ;
#55628=EDGE_LOOP ( 'NONE', ( #2978, #37198, #66146, #40917 ) ) ;
#55629=CARTESIAN_POINT ( 'NONE',  ( 93.72687053612523300, 23.04134601640628333, 7.892519177242094841 ) ) ;
#55631=CARTESIAN_POINT ( 'NONE',  ( 11.82929895397812814, 7.412564870773603154, 57.98450507560617950 ) ) ;
#55632=B_SPLINE_CURVE_WITH_KNOTS ( 'NONE', 3,
 ( #4966, #26, #37312, #69335, #15186, #42265, #47515, #59111, #21158, #48540, #68974, #43276, #32401, #48890, #58766, #375, #64055, #10928, #64397, #16209, #42601, #63724, #31704, #26775, #15534, #31368, #27449, #10579, #11271, #32052, #53826, #32740, #36986, #54170, #5992, #36647, #38014, #52797, #21826, #58424, #64752, #16558, #48201, #50656, #60516, #43626, #2476 ),
 .UNSPECIFIED., .F., .F.,
 ( 4, 2, 2, 2, 2, 2, 2, 2, 2, 2, 2, 1, 2, 2, 2, 2, 2, 2, 2, 2, 2, 2, 2, 4 ),
 ( 0.000000000000000000, 0.003297771944419079955, 0.004122214930523814165, 0.004946657916628548375, 0.006595543888838025469, 0.007419986874942737128, 0.008244429861047451388, 0.009068872847152163047, 0.009893315833256876440, 0.01154220180546630149, 0.01236664479157101315, 0.01319108777767572481, 0.01401553076378043820, 0.01483997374988514986, 0.01566441673598986326, 0.01648885972209457318, 0.01813774569430401384, 0.01896218868040875152, 0.01978663166651348920, 0.02061107465261822688, 0.02143551763872296456, 0.02308440361093244339, 0.02473328958314192222, 0.02638217555535139758 ),
 .UNSPECIFIED. ) ;
#55633=DIRECTION ( 'NONE',  ( 0.000000000000000000, 0.000000000000000000, 1.000000000000000000 ) ) ;
#55634=DIRECTION ( 'NONE',  ( 0.000000000000000000, 0.000000000000000000, 1.000000000000000000 ) ) ;
#55635=FACE_BOUND ( 'NONE', #53678, .T. ) ;
#55643=CARTESIAN_POINT ( 'NONE',  ( 155.7277429502854602, 56.30804678861343149, 2.756809054777331625 ) ) ;
#55644=CARTESIAN_POINT ( 'NONE',  ( 82.95057496836383848, 18.19812356106674400, -63.61242132756339629 ) ) ;
#55645=EDGE_CURVE ( 'NONE', #51139, #27226, #15090, .T. ) ;
#55648=VERTEX_POINT ( 'NONE', #30396 ) ;
#55649=CARTESIAN_POINT ( 'NONE',  ( 57.39674746172462960, 11.43903079040059190, 15.46024453313638247 ) ) ;
#55651=CARTESIAN_POINT ( 'NONE',  ( 201.9721407532275066, 104.3507814346147740, -36.82671456535588561 ) ) ;
#55659=ADVANCED_FACE ( 'NONE', ( #34989 ), #3660, .F. ) ;
#55661=ORIENTED_EDGE ( 'NONE', *, *, #56622, .T. ) ;
#55663=ORIENTED_EDGE ( 'NONE', *, *, #43023, .F. ) ;
#55665=CARTESIAN_POINT ( 'NONE',  ( 163.1313205310724470, 63.49733392291054201, 41.83532195775659090 ) ) ;
#55666=CARTESIAN_POINT ( 'NONE',  ( -150.3850953947692801, 66.25368649589884740, -61.69593361462676739 ) ) ;
#55667=CARTESIAN_POINT ( 'NONE',  ( 66.07923263163411320, 14.44036440558000223, 3.618334148579396725 ) ) ;
#55670=LINE ( 'NONE', #39500, #28948 ) ;
#55671=CARTESIAN_POINT ( 'NONE',  ( -55.05276343752909440, 15.72344139423348430, 18.47277718246750311 ) ) ;
#55672=CARTESIAN_POINT ( 'NONE',  ( -127.6894679065405143, 48.89973668460848444, -8.273314918213934277 ) ) ;
#55673=CARTESIAN_POINT ( 'NONE',  ( -156.0562654606047488, 71.30334311561915683, -92.33834972157848142 ) ) ;
#55675=CARTESIAN_POINT ( 'NONE',  ( 112.1164716692773027, 29.75790342121397813, -9.300245223945209361 ) ) ;
#55677=CARTESIAN_POINT ( 'NONE',  ( 94.10318957145940999, 22.10801446288250105, 91.83129037648295423 ) ) ;
#55679=VERTEX_POINT ( 'NONE', #4014 ) ;
#55682=CARTESIAN_POINT ( 'NONE',  ( 42.71504753277076816, 8.863481902720399930, 17.30229059452629414 ) ) ;
#55683=DIRECTION ( 'NONE',  ( -0.000000000000000000, 1.000000000000000000, -0.000000000000000000 ) ) ;
#55684=DIRECTION ( 'NONE',  ( 0.000000000000000000, -1.000000000000000000, 0.000000000000000000 ) ) ;
#55686=CARTESIAN_POINT ( 'NONE',  ( 181.0840389613909736, -170.0000000000000000, -43.72505766587962484 ) ) ;
#55687=CARTESIAN_POINT ( 'NONE',  ( 209.0197447343145711, 114.2532834725572002, 84.26074548200141123 ) ) ;
#55688=B_SPLINE_CURVE_WITH_KNOTS ( 'NONE', 3,
 ( #69496, #63888, #53994, #59625, #15698, #21314, #58593, #64577, #5819, #32567, #31880, #16390, #43452, #5141, #16039, #6169, #37490, #58940, #32227, #53662, #48716, #5485, #26939, #48366, #197, #21659, #64931, #37843, #34319, #39587, #28687, #27979, #17790, #33277, #1252, #39929, #65631, #56109, #50486, #66685, #44515, #17418, #22705, #61387, #45203, #61039 ),
 .UNSPECIFIED., .F., .F.,
 ( 4, 2, 2, 2, 2, 2, 2, 2, 2, 2, 2, 2, 2, 2, 2, 2, 2, 2, 2, 2, 2, 2, 4 ),
 ( 0.000000000000000000, 0.003635178948345886823, 0.005452768422518803129, 0.007270357896691719002, 0.008179152633778141376, 0.009087947370864565486, 0.01090553684503748136, 0.01181433158212392975, 0.01272312631921037988, 0.01363192105629682828, 0.01454071579338327667, 0.01544951053046972854, 0.01635830526755617867, 0.01726710000464262706, 0.01817589474172907546, 0.01908468947881552386, 0.01999348421590197225, 0.02090227895298842412, 0.02181107369007487251, 0.02362866316424780053, 0.02544625263842072507, 0.02726384211259365309, 0.02908143158676657763 ),
 .UNSPECIFIED. ) ;
#55691=CARTESIAN_POINT ( 'NONE',  ( -11.78792974237933144, 7.181513757308655599, 31.24314124056975928 ) ) ;
#55692=VERTEX_POINT ( 'NONE', #50812 ) ;
#55698=AXIS2_PLACEMENT_3D ( 'NONE', #63236, #36502, #53347 ) ;
#55699=CARTESIAN_POINT ( 'NONE',  ( -55.05276343752909440, 14.68156374112638041, -35.21632399845986328 ) ) ;
#55700=CARTESIAN_POINT ( 'NONE',  ( -38.17834711144558213, 11.81993749040892006, 94.71300855358852289 ) ) ;
#55701=CARTESIAN_POINT ( 'NONE',  ( 117.6853163455685234, 33.60747889659833021, -15.51686428253033334 ) ) ;
#55706=CARTESIAN_POINT ( 'NONE',  ( 140.9141742510256847, 47.05414327990550305, -19.26942019242481052 ) ) ;
#55708=EDGE_LOOP ( 'NONE', ( #28787, #14705, #42137, #45233 ) ) ;
#55712=VECTOR ( 'NONE', #12789, 1000.000000000000000 ) ;
#55715=CARTESIAN_POINT ( 'NONE',  ( 55.51547041749725508, 11.05727559334829735, -16.61830272299990696 ) ) ;
#55718=CARTESIAN_POINT ( 'NONE',  ( -52.45215874217871033, 13.99961488531755727, 30.77850105701925187 ) ) ;
#55719=CARTESIAN_POINT ( 'NONE',  ( 202.7506655727288489, 105.3943386412348957, 70.80670385009113943 ) ) ;
#55725=B_SPLINE_CURVE_WITH_KNOTS ( 'NONE', 3,
 ( #23669, #23335, #22977, #49683, #29289, #13462, #44420, #50052, #34921, #56363, #44779, #66256, #22620, #34592, #2562, #50742, #12770, #12422, #61301, #38809, #18046, #66944, #28602, #60949, #44060, #34232, #50403, #12073, #1881, #17703, #55318, #39162, #54969, #40196, #18737, #65904, #60255, #2220, #1166, #45113, #66596, #33541, #7139, #18385, #55672, #30332, #41570, #8881 ),
 .UNSPECIFIED., .F., .F.,
 ( 4, 2, 2, 2, 2, 2, 2, 2, 2, 2, 2, 2, 2, 2, 2, 2, 2, 2, 2, 2, 2, 2, 2, 4 ),
 ( 0.02554216173022672010, 0.02715505844859231535, 0.02796150680777513900, 0.02876795516695796265, 0.03038085188532356137, 0.03199374860368915663, 0.03360664532205475535, 0.03441309368123755819, 0.03521954204042036102, 0.03602599039960316385, 0.03683243875878596668, 0.03844533547715157235, 0.03925178383633436824, 0.04005823219551716413, 0.04086468055469996696, 0.04167112891388276286, 0.04247757727306555875, 0.04328402563224835464, 0.04489692235061398806, 0.04650981906897962148, 0.04731626742816243125, 0.04812271578734524796, 0.04973561250571081893, 0.05134850922407639684 ),
 .UNSPECIFIED. ) ;
#55726=EDGE_CURVE ( 'NONE', #39251, #168, #15895, .T. ) ;
#55727=CARTESIAN_POINT ( 'NONE',  ( -180.4643341113398094, 95.69224917234934935, -40.65656990911850244 ) ) ;
#55728=CARTESIAN_POINT ( 'NONE',  ( 103.8093541423578898, 26.01745837747064982, 6.379909146910426543 ) ) ;
#55729=CARTESIAN_POINT ( 'NONE',  ( -169.1041038606267364, 82.76530082651281361, 5.127983675400830776 ) ) ;
#55731=FACE_BOUND ( 'NONE', #51239, .T. ) ;
#55732=CARTESIAN_POINT ( 'NONE',  ( -189.4135091951039271, 107.3303746924218274, 93.77231123529229251 ) ) ;
#55733=CARTESIAN_POINT ( 'NONE',  ( -1.319107422865894108, 6.554467368239800251, 60.69727779971288584 ) ) ;
#55736=CARTESIAN_POINT ( 'NONE',  ( -125.8938041572051105, 46.49392987655492959, -61.75825448869760237 ) ) ;
#55741=FACE_OUTER_BOUND ( 'NONE', #17218, .T. ) ;
#55747=CARTESIAN_POINT ( 'NONE',  ( 173.5843421840238250, 71.34465141434347402, -43.42181600850904744 ) ) ;
#55748=CARTESIAN_POINT ( 'NONE',  ( 154.4435090467314069, 56.59612921827834242, 43.77540956279869278 ) ) ;
#55750=EDGE_LOOP ( 'NONE', ( #66936, #35142 ) ) ;
#55754=CARTESIAN_POINT ( 'NONE',  ( -0.5780275525703886252, 6.527356703336898214, 8.825157539075730639 ) ) ;
#55756=CARTESIAN_POINT ( 'NONE',  ( -80.31482177285907653, 24.03632224640838189, 30.59770256097123919 ) ) ;
#55758=CARTESIAN_POINT ( 'NONE',  ( -27.70115495247213033, 10.02455692117576547, -9.452150211312456918 ) ) ;
#55759=CARTESIAN_POINT ( 'NONE',  ( -52.00092620775821217, 14.92276858858357969, -22.72708555046020251 ) ) ;
#55763=CARTESIAN_POINT ( 'NONE',  ( 117.3281529665581786, 32.29994712002882551, -40.90972925606320842 ) ) ;
#55767=CARTESIAN_POINT ( 'NONE',  ( 46.70715146412977958, 9.472433765546995232, -44.83575853474970074 ) ) ;
#55769=CARTESIAN_POINT ( 'NONE',  ( -120.8809492823584435, 43.28069332005611614, 86.22209529451693300 ) ) ;
#55771=CARTESIAN_POINT ( 'NONE',  ( 81.03898448521320574, 17.58847173596444335, -48.34590843317131004 ) ) ;
#55775=B_SPLINE_CURVE_WITH_KNOTS ( 'NONE', 3,
 ( #2468, #7752, #56978, #62605, #23922, #51005, #35864, #14412, #24278, #67201, #23580, #3502, #66504, #28860, #50310, #13373, #40784, #50646, #61887, #56269, #29534, #46062, #18294, #67531, #19331, #45374, #2814, #62241, #66852, #18643, #35518, #45724, #8795, #2128, #40103, #67883, #41138, #20364, #63968, #62939, #58679, #37227, #42172, #47782 ),
 .UNSPECIFIED., .F., .F.,
 ( 4, 2, 2, 2, 2, 2, 2, 2, 2, 2, 2, 2, 2, 2, 2, 2, 2, 2, 2, 2, 2, 4 ),
 ( 0.000000000000000000, 0.003360573201437790872, 0.004200716501797208992, 0.005040859802156626678, 0.006721146402875383119, 0.007561289703234740957, 0.008401433003594098795, 0.009241576303953457500, 0.01008171960431281620, 0.01176200620503154576, 0.01260214950539091140, 0.01344229280575027705, 0.01428243610610964269, 0.01512257940646901180, 0.01680286600718775003, 0.01764300930754711741, 0.01848315260790648826, 0.02016343920862520914, 0.02184372580934392655, 0.02352401241006264743, 0.02520429901078136484, 0.02688458561150008225 ),
 .UNSPECIFIED. ) ;
#55777=CARTESIAN_POINT ( 'NONE',  ( 81.74250361646207352, 18.86685472882137304, 42.92257895484420516 ) ) ;
#55780=CARTESIAN_POINT ( 'NONE',  ( 139.6203063421347395, 45.01495791936838486, -21.50363658416259582 ) ) ;
#55781=CARTESIAN_POINT ( 'NONE',  ( 43.14565945994674223, 9.942782559600559011, 4.065828422660362484 ) ) ;
#55782=CARTESIAN_POINT ( 'NONE',  ( 18.65373113224114832, 7.616233774882145369, -89.76416870551544491 ) ) ;
#55786=CARTESIAN_POINT ( 'NONE',  ( 109.7724924842965777, 28.66436020578542809, 71.45576479620103783 ) ) ;
#55787=CARTESIAN_POINT ( 'NONE',  ( 164.8886903222557407, 63.65672212134879260, 62.61455516568165081 ) ) ;
#55791=CARTESIAN_POINT ( 'NONE',  ( -108.9452487746634120, 36.29752968355630571, 61.38692384849660755 ) ) ;
#55792=CYLINDRICAL_SURFACE ( 'NONE', #62037, 7.500000000000013323 ) ;
#55796=EDGE_LOOP ( 'NONE', ( #66090, #63867, #22411, #3706 ) ) ;
#55797=VERTEX_POINT ( 'NONE', #54243 ) ;
#55800=CYLINDRICAL_SURFACE ( 'NONE', #31895, 7.500000000000020428 ) ;
#55801=CARTESIAN_POINT ( 'NONE',  ( -84.54326985437108988, 24.64760594531652771, 69.44852943540219314 ) ) ;
#55806=CARTESIAN_POINT ( 'NONE',  ( -95.20053778133913625, 30.43887292928078381, -18.19781731286621707 ) ) ;
#55808=CARTESIAN_POINT ( 'NONE',  ( 37.00112095025831138, 8.109340230899352520, 71.36796680436268048 ) ) ;
#55812=ORIENTED_EDGE ( 'NONE', *, *, #11980, .F. ) ;
#55814=CARTESIAN_POINT ( 'NONE',  ( -0.5751131641471393108, 6.527254166626919485, -40.98318541392706038 ) ) ;
#55816=CARTESIAN_POINT ( 'NONE',  ( -7.825402957745085430, 7.899365992529246761, 18.27103044898354511 ) ) ;
#55817=CARTESIAN_POINT ( 'NONE',  ( -147.3614567344830277, 62.37986555269947786, 18.57643577236105870 ) ) ;
#55819=CARTESIAN_POINT ( 'NONE',  ( 201.9869293910475392, 102.6997661182766990, 70.55695970202656042 ) ) ;
#55820=CARTESIAN_POINT ( 'NONE',  ( 126.6266894765172850, 38.37986986668738609, -14.61571443927980418 ) ) ;
#55823=ORIENTED_EDGE ( 'NONE', *, *, #11261, .F. ) ;
#55826=CARTESIAN_POINT ( 'NONE',  ( -31.43908319763709969, 10.61114334766715928, -50.31719736520186359 ) ) ;
#55830=CARTESIAN_POINT ( 'NONE',  ( -120.4586945679390766, 43.01762219615312688, -37.22256326113324576 ) ) ;
#55832=CARTESIAN_POINT ( 'NONE',  ( -142.0062637385110236, 58.06920992247432167, -14.91780738418984420 ) ) ;
#55833=CARTESIAN_POINT ( 'NONE',  ( -7.330587818645182274, 7.867004275019543691, -62.26262132240751157 ) ) ;
#55835=CARTESIAN_POINT ( 'NONE',  ( 164.2838686904782151, 64.46257747810135186, 93.81936057118011263 ) ) ;
#55838=CARTESIAN_POINT ( 'NONE',  ( 161.3396229061448821, 62.02013338058599601, -90.87705086538740318 ) ) ;
#55841=EDGE_CURVE ( 'NONE', #33379, #8644, #22602, .T. ) ;
#55842=CARTESIAN_POINT ( 'NONE',  ( 16.28371206594635723, 6.516665886438624433, -35.51894409868580738 ) ) ;
#55843=CARTESIAN_POINT ( 'NONE',  ( 117.7442255600443275, 33.63739995216996448, 9.767747294482646225 ) ) ;
#55845=CARTESIAN_POINT ( 'NONE',  ( 56.53635105806416306, 11.26263375223564367, 33.52739349540972569 ) ) ;
#55849=CARTESIAN_POINT ( 'NONE',  ( 173.5844030397476274, 72.71952271766126330, 36.50363886079529863 ) ) ;
#55851=CARTESIAN_POINT ( 'NONE',  ( 16.28371206594634657, 6.516665886438621769, -62.36349468914946215 ) ) ;
#55853=CARTESIAN_POINT ( 'NONE',  ( -13.92109095214679648, 8.375243258322925044, -74.13901166531486808 ) ) ;
#55856=CARTESIAN_POINT ( 'NONE',  ( -23.93895920923072396, 9.495000752338446759, 37.47437177380988516 ) ) ;
#55859=CARTESIAN_POINT ( 'NONE',  ( -76.32456871438915869, 22.51591205926308703, -49.75660205866648056 ) ) ;
#55861=EDGE_LOOP ( 'NONE', ( #35523, #62497, #51269, #64558 ) ) ;
#55863=CARTESIAN_POINT ( 'NONE',  ( 210.5008983495072243, 116.4753531594350733, -65.91294173661489708 ) ) ;
#55866=CARTESIAN_POINT ( 'NONE',  ( 154.9796718954650601, 55.73967834827486456, -90.22953998753959581 ) ) ;
#55867=CARTESIAN_POINT ( 'NONE',  ( -7.825402957745085430, -170.0000000000000000, -23.57352014148015584 ) ) ;
#55868=CARTESIAN_POINT ( 'NONE',  ( 21.43750346857337519, 7.754771113113076986, 69.31663613037677862 ) ) ;
#55874=CARTESIAN_POINT ( 'NONE',  ( -37.07086358537071646, 10.58360809068249964, -37.84001496053501512 ) ) ;
#55878=CARTESIAN_POINT ( 'NONE',  ( -71.57660578921959882, 20.81129687646279436, -13.27386354321084383 ) ) ;
#55880=CARTESIAN_POINT ( 'NONE',  ( 85.67138972405898301, 19.09593469918313957, 56.60270476246709137 ) ) ;
#55882=CARTESIAN_POINT ( 'NONE',  ( 35.65685430025423841, 7.951642554322390311, 43.93025521648888798 ) ) ;
#55886=CARTESIAN_POINT ( 'NONE',  ( -125.8938041572051389, 47.69968343338778283, -23.06915330777029638 ) ) ;
#55887=CARTESIAN_POINT ( 'NONE',  ( -51.77439426130688815, 13.82695438436703128, 17.72271401957979364 ) ) ;
#55889=ORIENTED_EDGE ( 'NONE', *, *, #5396, .F. ) ;
#55895=CARTESIAN_POINT ( 'NONE',  ( -61.53550548562874667, 17.56596194025584978, 68.46545811016181915 ) ) ;
#55899=CARTESIAN_POINT ( 'NONE',  ( 151.1827182658834374, 54.16800928478855326, -74.58909220960448749 ) ) ;
#55900=CARTESIAN_POINT ( 'NONE',  ( -33.83558513595454542, 9.996963989836507025, 44.82747360581453933 ) ) ;
#55903=CARTESIAN_POINT ( 'NONE',  ( -30.46060138092287772, 9.432375387772214737, 72.01313598860062370 ) ) ;
#55908=CARTESIAN_POINT ( 'NONE',  ( -124.3250225421925990, 45.46958056770281331, 45.45752980411683097 ) ) ;
#55913=CARTESIAN_POINT ( 'NONE',  ( 128.2049106864180601, 39.27214849547761588, 85.72287850017508504 ) ) ;
#55919=CARTESIAN_POINT ( 'NONE',  ( -121.2008155373973608, 43.48033530165983507, -75.12874222293449122 ) ) ;
#55922=CARTESIAN_POINT ( 'NONE',  ( 160.9241720448059425, 60.38677655937337363, -10.10604509194042500 ) ) ;
#55924=CARTESIAN_POINT ( 'NONE',  ( 64.93495251696904802, 13.12601614965099728, 56.90318657735401331 ) ) ;
#55925=CARTESIAN_POINT ( 'NONE',  ( 140.4897729434290454, 45.57634363643753517, -66.82868248181939919 ) ) ;
#55927=ORIENTED_EDGE ( 'NONE', *, *, #47177, .T. ) ;
#55928=CARTESIAN_POINT ( 'NONE',  ( 161.7031777507226877, 62.31724004902782355, -10.57123460863781261 ) ) ;
#55929=CARTESIAN_POINT ( 'NONE',  ( 14.08699529666005823, 6.452200550165255066, 44.82328613664139993 ) ) ;
#55930=VERTEX_POINT ( 'NONE', #12405 ) ;
#55931=CARTESIAN_POINT ( 'NONE',  ( -125.8938041572051105, 47.69968343338781835, 45.61994787315711619 ) ) ;
#55932=CARTESIAN_POINT ( 'NONE',  ( 129.2374845572065851, 38.70429341380298638, -91.29071524815627470 ) ) ;
#55934=CARTESIAN_POINT ( 'NONE',  ( -148.4259959918497600, 63.26767374754766138, -61.73259096974960869 ) ) ;
#55938=CARTESIAN_POINT ( 'NONE',  ( 164.9709596662455340, 63.72607097915130936, -43.36052436387029729 ) ) ;
#55941=EDGE_CURVE ( 'NONE', #42689, #14285, #38571, .T. ) ;
#55943=CARTESIAN_POINT ( 'NONE',  ( 69.72022767004882837, 15.36837594864515388, 94.43018735991657309 ) ) ;
#55945=CARTESIAN_POINT ( 'NONE',  ( 34.83823433017388282, 8.871835168107979896, 31.44169914746493788 ) ) ;
#55947=CARTESIAN_POINT ( 'NONE',  ( -125.8938041572051389, 46.49392987655490828, -8.069153307770243089 ) ) ;
#55948=CARTESIAN_POINT ( 'NONE',  ( 34.13137819193417499, 8.793608427416353734, -91.40789414581379901 ) ) ;
#55949=CARTESIAN_POINT ( 'NONE',  ( 130.7260704202054455, 39.56565398554879920, -77.19931493661745492 ) ) ;
#55950=B_SPLINE_CURVE_WITH_KNOTS ( 'NONE', 3,
 ( #59377, #5905, #54086, #16813, #28416, #59031, #54797, #32659, #49868, #649, #23154, #11889, #55143, #44241, #22448, #54437, #5573, #65017 ),
 .UNSPECIFIED., .F., .F.,
 ( 4, 2, 2, 2, 2, 2, 2, 2, 4 ),
 ( 0.01277287546153429119, 0.01590198764852522595, 0.01746654374202068205, 0.01903109983551613815, 0.01981337788226390437, 0.02059565592901167058, 0.02216021202250712668, 0.02372476811600258279, 0.02528932420949803542 ),
 .UNSPECIFIED. ) ;
#55954=CARTESIAN_POINT ( 'NONE',  ( -14.92860730136983705, 8.468845235798745819, 62.04033186115039911 ) ) ;
#55960=DIRECTION ( 'NONE',  ( 0.000000000000000000, 0.000000000000000000, 1.000000000000000000 ) ) ;
#55962=CARTESIAN_POINT ( 'NONE',  ( -49.45858366215606594, 13.25262207532078662, -74.56246164764421280 ) ) ;
#55964=CARTESIAN_POINT ( 'NONE',  ( -10.92576759990585700, 8.121994053275061631, 44.44912068652092785 ) ) ;
#55966=ORIENTED_EDGE ( 'NONE', *, *, #8844, .T. ) ;
#55968=CARTESIAN_POINT ( 'NONE',  ( -95.04371414958063724, 30.36527049547254720, -44.55352501167941881 ) ) ;
#55970=CARTESIAN_POINT ( 'NONE',  ( 109.3047266816502088, 28.44977739115300253, -77.72287105795275863 ) ) ;
#55971=CARTESIAN_POINT ( 'NONE',  ( 46.84154678921882464, 10.51341196666389521, -17.25711569787797828 ) ) ;
#55972=CARTESIAN_POINT ( 'NONE',  ( 46.90141780929663895, 9.503798448769778417, 63.75374896832851590 ) ) ;
#55974=CARTESIAN_POINT ( 'NONE',  ( -15.16549112504216268, 7.480664377850763103, 92.87927133262334678 ) ) ;
#55975=B_SPLINE_CURVE_WITH_KNOTS ( 'NONE', 3,
 ( #16515, #11228, #691, #32694, #11571, #6308, #27760, #66130, #22840, #13675, #65768, #60475, #23550, #1741, #2098, #55899, #23890, #60814, #7012, #29503, #12289, #28466, #18613, #8407, #55539, #24249, #7718, #12641, #18958, #50967, #61174, #34461, #29166, #50615, #7372, #2433, #44988, #50274, #45336, #45692, #29857, #40067, #61522, #56586, #1383, #44281, #2779, #66818, #39371, #13341 ),
 .UNSPECIFIED., .F., .F.,
 ( 4, 2, 2, 2, 2, 2, 2, 2, 2, 2, 2, 2, 2, 2, 2, 2, 2, 2, 2, 2, 2, 2, 2, 2, 4 ),
 ( 0.02688458561150013429, 0.02770990876165297517, 0.02853523191180581606, 0.03018587821211148742, 0.03183652451241715531, 0.03266184766256999272, 0.03348717081272283708, 0.03513781711302847027, 0.03678846341333410347, 0.03761378656348691313, 0.03843910971363971585, 0.03926443286379251857, 0.04008975601394532129, 0.04174040231425089204, 0.04256572546440369476, 0.04339104861455649748, 0.04421637176470930020, 0.04504169491486210292, 0.04586701806501490564, 0.04669234121516771530, 0.04834298751547328604, 0.04916831066562603325, 0.04999363381577878046, 0.05164428011608426794, 0.05329492641638975542 ),
 .UNSPECIFIED. ) ;
#55977=DIRECTION ( 'NONE',  ( -0.000000000000000000, 1.000000000000000000, -0.000000000000000000 ) ) ;
#55988=CARTESIAN_POINT ( 'NONE',  ( 57.57684776206768618, 12.50442334002048561, -21.54617277829715505 ) ) ;
#55990=CARTESIAN_POINT ( 'NONE',  ( 89.87840278991586729, 21.62393877508910123, 3.603499079925511328 ) ) ;
#55991=CARTESIAN_POINT ( 'NONE',  ( 21.43750346857337874, 7.754771113113079650, -38.06156623147796125 ) ) ;
#55992=CARTESIAN_POINT ( 'NONE',  ( 13.37708032728285623, 7.441924986912758833, 57.25317478596774379 ) ) ;
#55994=B_SPLINE_CURVE_WITH_KNOTS ( 'NONE', 3,
 ( #7386, #33069, #50627, #66487, #43947, #60137, #18279, #65425, #17217, #38692, #55919, #60491, #33427, #65073, #16872, #54853, #54496, #6677, #49572, #22854, #44303, #17582, #24262, #24953, #46736, #56961, #30920, #29518, #40768, #9459, #67864, #36190, #52365, #41472, #23905, #50984, #3483, #9112, #56601, #3833, #20018, #57649, #46384, #2800, #45355, #46044 ),
 .UNSPECIFIED., .F., .F.,
 ( 4, 2, 2, 2, 2, 2, 2, 2, 2, 2, 2, 2, 2, 2, 2, 2, 2, 2, 2, 2, 2, 2, 4 ),
 ( 0.02584318557310393699, 0.02743529570732774342, 0.02823135077443962929, 0.02902740584155151862, 0.03061951597577525913, 0.03221162610999900311, 0.03380373624422274015, 0.03459979131133462255, 0.03539584637844649800, 0.03619190144555838040, 0.03698795651267025586, 0.03858006664689401372, 0.03937612171400586836, 0.04017217678111772994, 0.04096823184822958458, 0.04176428691534143922, 0.04335639704956512075, 0.04494850718378880228, 0.04654061731801248381, 0.04813272745223615839, 0.04892878251934799916, 0.04972483758645983298, 0.05131694772068345900 ),
 .UNSPECIFIED. ) ;
#55995=LINE ( 'NONE', #12735, #42090 ) ;
#55996=FACE_BOUND ( 'NONE', #49754, .T. ) ;
#55998=VECTOR ( 'NONE', #5207, 1000.000000000000000 ) ;
#56002=ADVANCED_FACE ( 'NONE', ( #27756 ), #54833, .F. ) ;
#56004=CARTESIAN_POINT ( 'NONE',  ( 88.53025347111699261, 21.14438024052373066, -50.59242619532921736 ) ) ;
#56007=CARTESIAN_POINT ( 'NONE',  ( 207.8398359204632868, 112.5208221429021478, 56.73900988323001826 ) ) ;
#56009=CIRCLE ( 'NONE', #58249, 242.4895526022646379 ) ;
#56012=CARTESIAN_POINT ( 'NONE',  ( 197.4121679705847612, 98.46451029407252520, -45.61355052951746814 ) ) ;
#56014=CARTESIAN_POINT ( 'NONE',  ( 63.01563776193091826, -170.0000000000000000, -8.876140241706055534 ) ) ;
#56015=ORIENTED_EDGE ( 'NONE', *, *, #814, .F. ) ;
#56016=CARTESIAN_POINT ( 'NONE',  ( -84.22570405563702423, 24.51726571826274181, -64.40185529543865073 ) ) ;
#56018=CARTESIAN_POINT ( 'NONE',  ( 90.30840373526891085, 21.77864858272155146, -76.70622861614346277 ) ) ;
#56021=CARTESIAN_POINT ( 'NONE',  ( 46.65860211212412878, 10.48377752989033951, 66.21745745935314176 ) ) ;
#56023=CARTESIAN_POINT ( 'NONE',  ( 22.89234820949993576, 6.832052815347870123, 8.252930022751796102 ) ) ;
#56026=CARTESIAN_POINT ( 'NONE',  ( -125.8938041572051105, 46.49392987655492959, -61.75825448869760237 ) ) ;
#56027=CARTESIAN_POINT ( 'NONE',  ( 62.52762183777209515, 13.59210632617625159, -35.72069083216972984 ) ) ;
#56029=CARTESIAN_POINT ( 'NONE',  ( 117.4830770399668012, 32.37795270233553424, -14.55398040625970957 ) ) ;
#56030=CARTESIAN_POINT ( 'NONE',  ( 90.96235852665459731, 20.94448655708621487, 84.74411175189248979 ) ) ;
#56031=CARTESIAN_POINT ( 'NONE',  ( -168.9893587165131521, 84.11247246121824617, -89.62666367685146440 ) ) ;
#56032=ORIENTED_EDGE ( 'NONE', *, *, #54760, .F. ) ;
#56033=ORIENTED_EDGE ( 'NONE', *, *, #6454, .F. ) ;
#56036=CARTESIAN_POINT ( 'NONE',  ( -180.2731542922991252, 97.04988144230624414, 94.37081299702376214 ) ) ;
#56037=CARTESIAN_POINT ( 'NONE',  ( -49.45858366215605884, 13.25262207532078307, -20.87336046671682155 ) ) ;
#56040=CARTESIAN_POINT ( 'NONE',  ( 197.8192566318489298, 98.97502303561493875, 87.37853646849281120 ) ) ;
#56045=CARTESIAN_POINT ( 'NONE',  ( 12.04188192036245297, 7.416006018508748632, -22.67628800238064457 ) ) ;
#56048=CARTESIAN_POINT ( 'NONE',  ( -146.5230751932348596, 62.99205605665031271, 4.481088983380310253 ) ) ;
#56049=CARTESIAN_POINT ( 'NONE',  ( 184.0001683447903815, 83.06228184427187955, -77.49291610268716113 ) ) ;
#56050=CARTESIAN_POINT ( 'NONE',  ( -167.4844853368928455, 82.52074065752739784, 33.36765669216441665 ) ) ;
#56057=CARTESIAN_POINT ( 'NONE',  ( 133.8566784816069060, 41.42467568809810530, -51.02331093239568816 ) ) ;
#56061=CARTESIAN_POINT ( 'NONE',  ( 188.5677332624426299, 88.01870958063736339, 89.96319809774311693 ) ) ;
#56065=LINE ( 'NONE', #38487, #44238 ) ;
#56067=CARTESIAN_POINT ( 'NONE',  ( -54.09522495088361183, 14.42642983673693813, 30.36297380349473229 ) ) ;
#56071=CARTESIAN_POINT ( 'NONE',  ( -59.58556642339448217, 16.99097764963620705, -63.56561058464538405 ) ) ;
#56072=CARTESIAN_POINT ( 'NONE',  ( 203.1423857108908919, 105.9238244286950135, -78.01806626934511257 ) ) ;
#56075=CARTESIAN_POINT ( 'NONE',  ( -166.2028657618940883, 79.74389853943290518, 14.38770061196751726 ) ) ;
#56076=CARTESIAN_POINT ( 'NONE',  ( -80.55742067659896577, 23.05042616197511762, -49.88874770082764343 ) ) ;
#56077=FACE_BOUND ( 'NONE', #43483, .T. ) ;
#56080=CARTESIAN_POINT ( 'NONE',  ( -0.8055628312658249524, 6.535476276302840226, 61.80831115705540668 ) ) ;
#56082=ADVANCED_FACE ( 'NONE', ( #33404 ), #60471, .F. ) ;
#56084=CARTESIAN_POINT ( 'NONE',  ( 151.8005253678162774, 54.62151558044534738, 58.81795113802257902 ) ) ;
#56088=ORIENTED_EDGE ( 'NONE', *, *, #30839, .F. ) ;
#56092=ORIENTED_EDGE ( 'NONE', *, *, #25680, .T. ) ;
#56094=CARTESIAN_POINT ( 'NONE',  ( -173.1211646369891355, 87.12891641440857882, -61.55650775521367279 ) ) ;
#56102=AXIS2_PLACEMENT_3D ( 'NONE', #55380, #28664, #50117 ) ;
#56103=CARTESIAN_POINT ( 'NONE',  ( 150.3320035166323976, 52.30731334295649049, 88.26711376708068713 ) ) ;
#56104=CARTESIAN_POINT ( 'NONE',  ( 140.8984307802396359, 45.84194788389001474, 7.533282231769419468 ) ) ;
#56107=CARTESIAN_POINT ( 'NONE',  ( -71.17846906053298994, 20.67346400882179935, 10.57915229329010565 ) ) ;
#56108=CARTESIAN_POINT ( 'NONE',  ( 45.49006904354232717, 9.279592366778887325, -47.50676418804506085 ) ) ;
#56109=CARTESIAN_POINT ( 'NONE',  ( -168.7329347389696181, 83.83901812802758968, -75.15730867994311382 ) ) ;
#56110=CARTESIAN_POINT ( 'NONE',  ( -118.4102557275056142, 41.75991974097812687, 92.41143590757182835 ) ) ;
#56115=B_SPLINE_CURVE_WITH_KNOTS ( 'NONE', 3,
 ( #4428, #58915, #37458, #47323, #20594, #46644, #37123, #26572, #31850, #36793, #14974, #63865, #62835, #42057, #15674, #5111, #14637, #63516, #58565, #48010, #36101, #51922, #58234, #52942, #57554, #25893, #41719, #9713, #63178, #9361, #64198, #10381, #30826, #68119, #4767, #16007, #31507, #26230, #25212, #10729, #47667, #3733, #68779, #53283 ),
 .UNSPECIFIED., .F., .F.,
 ( 4, 2, 2, 2, 2, 2, 2, 2, 2, 2, 2, 2, 2, 2, 2, 2, 2, 2, 2, 2, 2, 4 ),
 ( 0.02477387709520258510, 0.02633314402883775787, 0.02711277749565534079, 0.02789241096247292370, 0.02945167789610812423, 0.03023131136292571408, 0.03101094482974330047, 0.03257021176337848711, 0.03334984523019606656, 0.03412947869701364600, 0.03568874563064879796, 0.03646837909746637740, 0.03724801256428394991, 0.03802764603110152242, 0.03880727949791910186, 0.04036654643155426075, 0.04192581336518942658, 0.04348508029882458548, 0.04504434723245974437, 0.04660361416609490326, 0.04816288109973006215, 0.04972214803336522798 ),
 .UNSPECIFIED. ) ;
#56116=CARTESIAN_POINT ( 'NONE',  ( 79.37778929114108450, 18.12554302172301490, 39.19102792528236279 ) ) ;
#56121=CARTESIAN_POINT ( 'NONE',  ( -178.5848962563134421, 94.99295350784009884, -10.20532857645564917 ) ) ;
#56122=CARTESIAN_POINT ( 'NONE',  ( -155.2912910578197057, 69.24479901948498650, -37.53156387900870783 ) ) ;
#56125=CARTESIAN_POINT ( 'NONE',  ( 106.0171289417043994, 26.97542621030654075, 70.15651320696453297 ) ) ;
#56130=CARTESIAN_POINT ( 'NONE',  ( 188.2950202724320832, 86.21411212788224532, -45.80789658381507223 ) ) ;
#56131=CARTESIAN_POINT ( 'NONE',  ( -102.2801239173131052, 32.78103895658057354, 57.36362509687880618 ) ) ;
#56133=DIRECTION ( 'NONE',  ( 0.000000000000000000, 0.000000000000000000, 1.000000000000000000 ) ) ;
#56137=ORIENTED_EDGE ( 'NONE', *, *, #33436, .T. ) ;
#56138=CARTESIAN_POINT ( 'NONE',  ( 86.62931800182293784, -170.0000000000000000, -70.16611478937539914 ) ) ;
#56141=CARTESIAN_POINT ( 'NONE',  ( 128.0882145863933488, 39.20607399008168414, 32.19109523275562168 ) ) ;
#56145=CARTESIAN_POINT ( 'NONE',  ( -100.4347360276019288, 32.97716872911836816, -22.95435981532398984 ) ) ;
#56146=CARTESIAN_POINT ( 'NONE',  ( 59.08202327466401726, 12.82375733818950536, 43.70333317471333601 ) ) ;
#56147=CARTESIAN_POINT ( 'NONE',  ( 32.31938840494672149, 7.593698200002521936, 88.61355331186805984 ) ) ;
#56150=CARTESIAN_POINT ( 'NONE',  ( -5.416136198635860488, 6.745992685878682948, -50.02480415146536785 ) ) ;
#56153=CARTESIAN_POINT ( 'NONE',  ( -149.0732005398557760, 63.81212100765654327, 18.86682848876648322 ) ) ;
#56155=CARTESIAN_POINT ( 'NONE',  ( 197.1974290009104891, 96.59277840252781289, 63.22824731097590245 ) ) ;
#56156=CARTESIAN_POINT ( 'NONE',  ( 126.4318266066172214, 38.27072266789467392, -17.77050837306448727 ) ) ;
#56161=CARTESIAN_POINT ( 'NONE',  ( 130.3035708464390154, 40.48418876551453849, -36.90095733877659967 ) ) ;
#56162=CARTESIAN_POINT ( 'NONE',  ( -37.07436112751821611, 11.60822760208522553, -37.84398108377252612 ) ) ;
#56167=CARTESIAN_POINT ( 'NONE',  ( 130.3281282802763315, 40.49854652972190650, 3.530804043226662969 ) ) ;
#56168=DIRECTION ( 'NONE',  ( -0.000000000000000000, 1.000000000000000000, -0.000000000000000000 ) ) ;
#56169=CARTESIAN_POINT ( 'NONE',  ( 202.7540649946182612, 105.3989460363904556, 2.608031559926723197 ) ) ;
#56170=B_SPLINE_CURVE_WITH_KNOTS ( 'NONE', 3,
 ( #7452, #58543, #5089, #60555, #66211, #44015, #38761, #27494, #31828, #48932, #22926, #34189, #50358, #774, #6742, #28551, #55273, #43664, #18000, #39448, #59842, #2174, #60900, #12721, #23629, #65492, #45065, #1828, #22573, #22227, #66551, #28189, #16937, #65852, #49997, #17651, #60203, #12024, #49639, #53260, #54570, #23287, #6397, #65143 ),
 .UNSPECIFIED., .F., .F.,
 ( 4, 2, 2, 2, 2, 2, 2, 2, 2, 2, 2, 2, 2, 2, 2, 2, 2, 2, 2, 2, 2, 4 ),
 ( 1.387778780781445676E-17, 0.003518733725596352984, 0.004398417156995421823, 0.005278100588394489361, 0.007037467451192665202, 0.007917150882591726668, 0.008796834313990788135, 0.01055620117678895444, 0.01231556803958712074, 0.01319525147098622384, 0.01407493490238532520, 0.01495461833378442830, 0.01583430176518352966, 0.01671398519658263276, 0.01759366862798173933, 0.01935303549077990737, 0.02111240235357807887, 0.02199208578497713687, 0.02287176921637619487, 0.02463113607917434902, 0.02639050294197250318, 0.02814986980477065734 ),
 .UNSPECIFIED. ) ;
#56171=CARTESIAN_POINT ( 'NONE',  ( 149.9779033028198683, 53.29256572657026680, 90.09284245516512613 ) ) ;
#56173=CARTESIAN_POINT ( 'NONE',  ( -57.65574514524056582, 16.43983577669857254, 3.934844714199217997 ) ) ;
#56174=CARTESIAN_POINT ( 'NONE',  ( 203.1511228994173166, 104.2426341584998823, -51.21072795959794632 ) ) ;
#56177=CARTESIAN_POINT ( 'NONE',  ( 21.44031696305385282, 6.747195267824409370, -38.06475470450458687 ) ) ;
#56178=CARTESIAN_POINT ( 'NONE',  ( 86.14852828165528820, 19.25704475759651402, 17.86753698201565754 ) ) ;
#56184=CARTESIAN_POINT ( 'NONE',  ( -169.1116812882276008, 84.24296059722695418, 17.83128106548857872 ) ) ;
#56185=CARTESIAN_POINT ( 'NONE',  ( 22.80839748737787787, 6.826915557457463812, -72.51456902026779971 ) ) ;
#56186=CARTESIAN_POINT ( 'NONE',  ( -11.57950265606958062, 8.174070387114797498, -63.26516250596657187 ) ) ;
#56188=CARTESIAN_POINT ( 'NONE',  ( -95.04384172745170645, 30.36531739257813101, 93.78841958355275210 ) ) ;
#56189=CARTESIAN_POINT ( 'NONE',  ( -24.71604178686819253, 9.599501655372943532, 34.38300249122266905 ) ) ;
#56191=CARTESIAN_POINT ( 'NONE',  ( -73.80418150970714919, 21.59712875466422943, -48.34729916886697509 ) ) ;
#56194=CARTESIAN_POINT ( 'NONE',  ( 212.1734186221015932, 119.0499290057855291, -69.97830959964204567 ) ) ;
#56195=EDGE_CURVE ( 'NONE', #29969, #63871, #43923, .T. ) ;
#56196=CARTESIAN_POINT ( 'NONE',  ( 141.3036441389950539, 47.31002705502927341, 35.97038062019882432 ) ) ;
#56198=FACE_OUTER_BOUND ( 'NONE', #31334, .T. ) ;
#56199=CARTESIAN_POINT ( 'NONE',  ( 70.26936813788618963, 15.51386666370915357, -72.03546886692284090 ) ) ;
#56201=VERTEX_POINT ( 'NONE', #17194 ) ;
#56213=CARTESIAN_POINT ( 'NONE',  ( -109.7811201291769549, 37.90784085457602970, 38.24940268311721780 ) ) ;
#56216=CARTESIAN_POINT ( 'NONE',  ( 37.47081272996201307, 8.166145978397521432, 44.66509977773299767 ) ) ;
#56223=CARTESIAN_POINT ( 'NONE',  ( -49.43915770973591606, 13.24768844696975378, 15.97056682900100810 ) ) ;
#56225=VECTOR ( 'NONE', #10114, 1000.000000000000000 ) ;
#56226=CARTESIAN_POINT ( 'NONE',  ( 154.0293889979056416, 55.02370422818216866, -50.30463981601170786 ) ) ;
#56227=VERTEX_POINT ( 'NONE', #51265 ) ;
#56229=CARTESIAN_POINT ( 'NONE',  ( -154.0775378574014098, 68.15437918458557931, -9.502335120361516729 ) ) ;
#56230=EDGE_LOOP ( 'NONE', ( #64161, #1679 ) ) ;
#56231=CARTESIAN_POINT ( 'NONE',  ( -58.32860549785896609, 15.58423118879329294, 31.06615926810922801 ) ) ;
#56232=CARTESIAN_POINT ( 'NONE',  ( -57.42826130032238297, 16.37596353166457419, 57.54390146367184400 ) ) ;
#56233=DIRECTION ( 'NONE',  ( -0.000000000000000000, 1.000000000000000000, -0.000000000000000000 ) ) ;
#56237=CARTESIAN_POINT ( 'NONE',  ( -96.78198318406111866, 30.07417864442862054, -20.79432951231798299 ) ) ;
#56238=CARTESIAN_POINT ( 'NONE',  ( 138.5721691894142680, 44.34516164557648210, -49.37593785591674589 ) ) ;
#56245=CARTESIAN_POINT ( 'NONE',  ( -125.8938041572051105, 46.49392987655495091, 45.61994787315711619 ) ) ;
#56248=CARTESIAN_POINT ( 'NONE',  ( 188.2133404574783242, 86.12414067617878288, 12.31026140296448013 ) ) ;
#56249=CARTESIAN_POINT ( 'NONE',  ( 87.10668362745094839, 19.58396519288863402, 56.55663816294299551 ) ) ;
#56253=ORIENTED_EDGE ( 'NONE', *, *, #30434, .F. ) ;
#56254=CARTESIAN_POINT ( 'NONE',  ( 157.4703587214989113, 57.65129005721576050, -9.279633708673953763 ) ) ;
#56256=CARTESIAN_POINT ( 'NONE',  ( 63.50528314073028469, 12.78634332146813435, 71.65751152968502424 ) ) ;
#56261=ORIENTED_EDGE ( 'NONE', *, *, #60699, .T. ) ;
#56264=CARTESIAN_POINT ( 'NONE',  ( 9.288975942802419894, 6.379608420846960115, 41.26562237599018346 ) ) ;
#56266=CARTESIAN_POINT ( 'NONE',  ( 69.83617901654358207, 15.39919709983075968, 61.02833969872266096 ) ) ;
#56267=CARTESIAN_POINT ( 'NONE',  ( 127.3115382175395780, 37.60999379334474213, 94.42761284291371737 ) ) ;
#56269=CARTESIAN_POINT ( 'NONE',  ( 164.8433205901839642, 64.93586312665803462, -42.22151823635311274 ) ) ;
#56276=CARTESIAN_POINT ( 'NONE',  ( -99.99439884168255332, 32.75762661251356889, 18.33352629368685527 ) ) ;
#56277=CARTESIAN_POINT ( 'NONE',  ( 59.84433950768821830, 12.98867007234732540, 84.17292290978423352 ) ) ;
#56280=PLANE ( 'NONE',  #36464 ) ;
#56281=CARTESIAN_POINT ( 'NONE',  ( -167.6413528428655866, 81.22881971256911982, 33.17534743252404894 ) ) ;
#56283=CARTESIAN_POINT ( 'NONE',  ( 126.6576865394845868, 37.24426596493988484, -68.24804092954708779 ) ) ;
#56284=B_SPLINE_CURVE_WITH_KNOTS ( 'NONE', 3,
 ( #2410, #50246, #45665, #67143, #45307, #3107, #1711, #55514, #24569, #13647, #17891, #44962, #55159, #39005, #65739, #60449, #18932, #12970, #40381, #35102, #56557, #23521, #7342, #2067, #66447, #18234, #39689, #61147, #34435, #7691, #42111, #31225, #9417, #41427, #62178, #51972, #68170, #25939, #15035, #35454, #3445, #51637, #62881, #14351, #9763, #52656, #30875, #46339 ),
 .UNSPECIFIED., .F., .F.,
 ( 4, 2, 2, 2, 2, 2, 2, 2, 2, 2, 2, 2, 2, 2, 2, 2, 2, 2, 2, 2, 2, 2, 2, 4 ),
 ( 0.02746511744866864460, 0.02914922134997103079, 0.03083332525127341350, 0.03251742915257578581, 0.03335948110322694421, 0.03420153305387810261, 0.03504358500452926101, 0.03588563695518041247, 0.03756974085648268069, 0.03841179280713380439, 0.03925384475778492810, 0.04009589670843605180, 0.04093794865908717551, 0.04262205256038943679, 0.04430615646169169808, 0.04514820841234285648, 0.04599026036299401488, 0.04767436426429631779, 0.04935846816559862071, 0.05020052011624975830, 0.05104257206690090282, 0.05272667596820317104, 0.05356872791885429475, 0.05441077986950541845 ),
 .UNSPECIFIED. ) ;
#56286=CARTESIAN_POINT ( 'NONE',  ( -99.99439884168261017, 32.75762661251357599, 72.02262747461425363 ) ) ;
#56287=CARTESIAN_POINT ( 'NONE',  ( -11.14668121284975832, 8.139398342256729535, 71.18912459828850103 ) ) ;
#56289=CARTESIAN_POINT ( 'NONE',  ( -153.6994314938755792, 69.16570456337669270, -36.07705819171143702 ) ) ;
#56290=CYLINDRICAL_SURFACE ( 'NONE', #26422, 7.500000000000020428 ) ;
#56291=CARTESIAN_POINT ( 'NONE',  ( -5.412684891282530053, 7.753215344827980360, 30.49725765081104001 ) ) ;
#56294=EDGE_CURVE ( 'NONE', #67008, #20980, #7994, .T. ) ;
#56297=CARTESIAN_POINT ( 'NONE',  ( 173.8575673535406452, 71.59843387604338716, 7.936245129884297533 ) ) ;
#56298=CARTESIAN_POINT ( 'NONE',  ( -62.53989795537025032, 16.81768094534200841, 11.47802686014114038 ) ) ;
#56303=CARTESIAN_POINT ( 'NONE',  ( 103.1653143050726129, 25.74301230421574616, -67.73440299836630629 ) ) ;
#56305=CARTESIAN_POINT ( 'NONE',  ( 45.89268866913130296, 10.36133864615985800, -12.50948627268672375 ) ) ;
#56313=CARTESIAN_POINT ( 'NONE',  ( -166.7049310409072405, 80.25944422923579680, 69.05890086907660930 ) ) ;
#56314=ORIENTED_EDGE ( 'NONE', *, *, #276, .T. ) ;
#56319=CARTESIAN_POINT ( 'NONE',  ( 42.62674880747476180, 8.849563476334237677, -89.98647070695761840 ) ) ;
#56322=LINE ( 'NONE', #51407, #66722 ) ;
#56324=CARTESIAN_POINT ( 'NONE',  ( 59.73312635112158375, 12.96464920523511388, -23.13701263744227532 ) ) ;
#56328=CARTESIAN_POINT ( 'NONE',  ( 45.80999061969644970, 9.329701754959341287, 94.99999999999866418 ) ) ;
#56330=CARTESIAN_POINT ( 'NONE',  ( -79.14127775978548129, 22.50259208414360756, -23.27090004125422595 ) ) ;
#56332=DIRECTION ( 'NONE',  ( 0.000000000000000000, 0.000000000000000000, 1.000000000000000000 ) ) ;
#56334=ORIENTED_EDGE ( 'NONE', *, *, #22947, .T. ) ;
#56340=CARTESIAN_POINT ( 'NONE',  ( 63.49940197359693883, 12.78497925206076147, 29.81296093922127000 ) ) ;
#56341=CARTESIAN_POINT ( 'NONE',  ( 79.14129363775931836, 17.00055658855363205, -70.65915694733433838 ) ) ;
#56344=CARTESIAN_POINT ( 'NONE',  ( 197.3756653044963514, 98.41886189307118116, -45.45805580265201939 ) ) ;
#56347=VERTEX_POINT ( 'NONE', #3413 ) ;
#56348=CARTESIAN_POINT ( 'NONE',  ( -81.90020664963803654, 23.57971581008656869, -76.23134889676580883 ) ) ;
#56349=CARTESIAN_POINT ( 'NONE',  ( -62.29496909743951960, 17.79481128341706508, -13.90640243752122807 ) ) ;
#56350=CARTESIAN_POINT ( 'NONE',  ( 88.53025347111696419, 21.14438024052372356, -77.43697678579287924 ) ) ;
#56354=CARTESIAN_POINT ( 'NONE',  ( 14.08699529666006178, 6.452200550165256843, -35.71036563474962833 ) ) ;
#56355=CARTESIAN_POINT ( 'NONE',  ( -103.3308778225766815, 34.44988434361755480, -88.77464374387059820 ) ) ;
#56356=CARTESIAN_POINT ( 'NONE',  ( 22.81270948571149404, 6.827178363529886163, 13.30984265512818077 ) ) ;
#56363=CARTESIAN_POINT ( 'NONE',  ( -130.1938957973835329, 50.61368074696266461, -21.73168917496282404 ) ) ;
#56364=CARTESIAN_POINT ( 'NONE',  ( 117.7447573007802788, 32.50990724960316669, -16.08767966913922010 ) ) ;
#56365=CARTESIAN_POINT ( 'NONE',  ( 80.73462811483980772, 18.54763808182591589, -47.98554289559778141 ) ) ;
#56366=CARTESIAN_POINT ( 'NONE',  ( -173.1211646369891355, 87.12891641440857882, -76.55650775521370122 ) ) ;
#56368=ORIENTED_EDGE ( 'NONE', *, *, #61156, .F. ) ;
#56369=AXIS2_PLACEMENT_3D ( 'NONE', #9818, #16113, #30580 ) ;
#56371=CARTESIAN_POINT ( 'NONE',  ( 46.85206196242844356, 9.495795933269485900, 9.575707866823087500 ) ) ;
#56373=CARTESIAN_POINT ( 'NONE',  ( -50.52927270563905182, 13.51486287463704627, -21.87426322953785629 ) ) ;
#56375=CARTESIAN_POINT ( 'NONE',  ( 197.1980152960109365, 96.59350208824301376, 10.20049193452572744 ) ) ;
#56376=CARTESIAN_POINT ( 'NONE',  ( -26.37870220071948069, 8.815136099259133218, -90.95400284204914954 ) ) ;
#56378=CARTESIAN_POINT ( 'NONE',  ( 211.5400400709320650, 118.0665875834716019, 93.47395779939256499 ) ) ;
#56379=CARTESIAN_POINT ( 'NONE',  ( 207.8398359204632868, 112.5208221429021194, 29.89445929276630665 ) ) ;
#56380=CARTESIAN_POINT ( 'NONE',  ( -79.61235761536670452, 23.76245710489568452, 57.30737474656424979 ) ) ;
#56381=CARTESIAN_POINT ( 'NONE',  ( -9.771516655894554759, 7.025139475821124968, 30.35594508498904531 ) ) ;
#56382=ORIENTED_EDGE ( 'NONE', *, *, #36756, .F. ) ;
#56383=CARTESIAN_POINT ( 'NONE',  ( 10.82760985890677752, 7.398654328676805392, -10.52802355588776351 ) ) ;
#56386=B_SPLINE_CURVE_WITH_KNOTS ( 'NONE', 3,
 ( #30958, #19351, #62262, #9152, #30607, #4221, #58357, #52060, #46778, #52403, #9843, #68581, #35541, #24992, #46424, #41164, #40807, #68909, #31304, #67902, #20382, #14081, #4556, #56995, #20053, #52731, #19700, #14433, #30266, #53068, #51715, #35884, #41506, #3873, #62958, #41850, #63310, #25342, #68248, #47449 ),
 .UNSPECIFIED., .F., .F.,
 ( 4, 2, 2, 2, 2, 2, 2, 2, 2, 2, 2, 2, 2, 2, 2, 2, 2, 2, 2, 4 ),
 ( 0.02472759712254455483, 0.02626001169882808198, 0.02779242627511161259, 0.02932484085139513974, 0.03009104813953689117, 0.03085725542767863566, 0.03238967000396208301, 0.03315587729210382750, 0.03392208458024557199, 0.03545449915652904710, 0.03698691373281252220, 0.03851932830909599731, 0.04005174288537947241, 0.04158415746166294058, 0.04311657203794641569, 0.04464898661422989079, 0.04541519390237163528, 0.04618140119051337977, 0.04771381576679688263, 0.04924623034308039937 ),
 .UNSPECIFIED. ) ;
#56389=CARTESIAN_POINT ( 'NONE',  ( -142.8492950481059438, 60.01492924994605715, 7.913576728738202171 ) ) ;
#56390=CARTESIAN_POINT ( 'NONE',  ( 185.5457097283155008, 84.70846743303874860, -64.52296994192434454 ) ) ;
#56391=CARTESIAN_POINT ( 'NONE',  ( -168.7314919967217577, 83.83749564070829763, 44.42116658107412519 ) ) ;
#56392=DIRECTION ( 'NONE',  ( -0.000000000000000000, 1.000000000000000000, -0.000000000000000000 ) ) ;
#56394=CARTESIAN_POINT ( 'NONE',  ( -23.98747857548121232, 9.501432345103351551, 11.85715207713718122 ) ) ;
#56397=CARTESIAN_POINT ( 'NONE',  ( 127.1040286383415605, 37.49395136275128948, -46.79722293648432441 ) ) ;
#56398=EDGE_LOOP ( 'NONE', ( #46052, #21804, #35446, #11471 ) ) ;
#56403=CARTESIAN_POINT ( 'NONE',  ( -28.35330809568272059, 9.105138953156460602, -62.82163295736274478 ) ) ;
#56406=CARTESIAN_POINT ( 'NONE',  ( 8.288451200428832877, 6.376395059685423305, 11.16205334907189162 ) ) ;
#56409=CARTESIAN_POINT ( 'NONE',  ( -57.65574514524056582, 16.43983577669855833, -76.59880705719182004 ) ) ;
#56410=CARTESIAN_POINT ( 'NONE',  ( 200.8383807319520713, 102.8517715783672912, -77.11560942651001938 ) ) ;
#56413=CARTESIAN_POINT ( 'NONE',  ( -24.03640295269301674, 9.507963273819775907, 63.33170168683827228 ) ) ;
#56415=ADVANCED_FACE ( 'NONE', ( #58251 ), #16380, .F. ) ;
#56416=CARTESIAN_POINT ( 'NONE',  ( -47.55235941796721733, 12.79790236059689867, 64.89954721557026573 ) ) ;
#56418=CARTESIAN_POINT ( 'NONE',  ( -99.60580143997752600, 31.44299022783583197, -89.19348776790582178 ) ) ;
#56423=DIRECTION ( 'NONE',  ( -0.000000000000000000, 1.000000000000000000, -0.000000000000000000 ) ) ;
#56425=CARTESIAN_POINT ( 'NONE',  ( -0.4403665414075291773, 7.529347476604110412, 89.95601636005106627 ) ) ;
#56427=CYLINDRICAL_SURFACE ( 'NONE', #5569, 7.500000000000013323 ) ;
#56431=DIRECTION ( 'NONE',  ( -0.000000000000000000, 1.000000000000000000, -0.000000000000000000 ) ) ;
#56436=CARTESIAN_POINT ( 'NONE',  ( -173.9656771507954431, 88.06879734510549440, 18.97714401617737323 ) ) ;
#56437=CARTESIAN_POINT ( 'NONE',  ( -4.513903087372272083, 6.697902023160579255, 4.037233194458375252 ) ) ;
#56438=CARTESIAN_POINT ( 'NONE',  ( 56.52205390515079841, 12.28646189164059166, -39.43576307262695479 ) ) ;
#56439=CARTESIAN_POINT ( 'NONE',  ( -86.06525741550311182, 26.37048289224653885, 39.17186844186085892 ) ) ;
#56440=CARTESIAN_POINT ( 'NONE',  ( -24.03640295269300964, 9.507963273819775907, -17.20195008455281993 ) ) ;
#56441=CARTESIAN_POINT ( 'NONE',  ( 141.3403471770512851, 46.13063628128485760, 9.603197491847479839 ) ) ;
#56444=ORIENTED_EDGE ( 'NONE', *, *, #15088, .F. ) ;
#56445=CARTESIAN_POINT ( 'NONE',  ( 115.0692128464502417, 31.17922615202198600, -37.66088901092161478 ) ) ;
#56447=CARTESIAN_POINT ( 'NONE',  ( -76.32456871438914447, 22.51591205926308703, 3.932499122260883606 ) ) ;
#56451=ORIENTED_EDGE ( 'NONE', *, *, #63766, .T. ) ;
#56452=CARTESIAN_POINT ( 'NONE',  ( 84.73231936899557581, 18.78199960571076943, -50.59343781656497896 ) ) ;
#56457=DIRECTION ( 'NONE',  ( 0.000000000000000000, 0.000000000000000000, 1.000000000000000000 ) ) ;
#56461=CARTESIAN_POINT ( 'NONE',  ( -123.4531143159639157, 44.90777521523903459, 57.86905838940393210 ) ) ;
#56462=CARTESIAN_POINT ( 'NONE',  ( -81.89510452344293867, 24.66033552777455284, -22.55706376423087178 ) ) ;
#56463=CARTESIAN_POINT ( 'NONE',  ( -180.5801285865471471, 97.42945596116095430, -16.16651611906625163 ) ) ;
#56464=AXIS2_PLACEMENT_3D ( 'NONE', #22932, #39807, #17656 ) ;
#56465=CARTESIAN_POINT ( 'NONE',  ( -47.94960849910474110, 13.92522873833625141, 40.27489391830895471 ) ) ;
#56471=CARTESIAN_POINT ( 'NONE',  ( 110.2429982417149432, 28.88204397445228722, 71.45576479620103783 ) ) ;
#56473=CARTESIAN_POINT ( 'NONE',  ( 164.7250737226290198, 63.51898362052162383, 65.67648673783554614 ) ) ;
#56474=CARTESIAN_POINT ( 'NONE',  ( -189.9554299271397326, 108.0836897899587967, 68.49611169383959464 ) ) ;
#56477=CARTESIAN_POINT ( 'NONE',  ( -142.3939495481492372, 59.65374914730258382, 94.38145074191702122 ) ) ;
#56482=CARTESIAN_POINT ( 'NONE',  ( -71.15978761293872878, 19.60276553435116753, 91.52478201086924514 ) ) ;
#56483=CARTESIAN_POINT ( 'NONE',  ( 174.3239633726426803, 72.03325965189267777, -94.13525938529653558 ) ) ;
#56484=CARTESIAN_POINT ( 'NONE',  ( 66.29961816943398389, 13.45804302849870204, -49.98079997445120881 ) ) ;
#56485=DIRECTION ( 'NONE',  ( 0.000000000000000000, 0.000000000000000000, 1.000000000000000000 ) ) ;
#56486=CARTESIAN_POINT ( 'NONE',  ( -57.43883374585513479, 16.37892664338858495, 44.93176015419845726 ) ) ;
#56488=CARTESIAN_POINT ( 'NONE',  ( 63.01563776193090405, 13.70579113808097738, 44.81296093922130552 ) ) ;
#56489=CARTESIAN_POINT ( 'NONE',  ( 38.09561781553523474, 8.243036803495508380, 83.71016925063842962 ) ) ;
#56493=CARTESIAN_POINT ( 'NONE',  ( 133.8566784816069344, 42.60093787723652525, -77.86786152285937135 ) ) ;
#56494=CARTESIAN_POINT ( 'NONE',  ( -189.9554299271397895, 108.0836897899587825, -38.88209066801512392 ) ) ;
#56497=CARTESIAN_POINT ( 'NONE',  ( 199.7278513351971299, 99.76879341361768638, 69.18835753365968344 ) ) ;
#56499=ORIENTED_EDGE ( 'NONE', *, *, #36220, .T. ) ;
#56502=CARTESIAN_POINT ( 'NONE',  ( 126.3554864210862121, 38.22801630372146775, -43.29534180877571004 ) ) ;
#56503=CARTESIAN_POINT ( 'NONE',  ( -35.38962320578853138, 11.29584325137385470, -36.43726333423634145 ) ) ;
#56506=ORIENTED_EDGE ( 'NONE', *, *, #65680, .F. ) ;
#56509=B_SPLINE_CURVE_WITH_KNOTS ( 'NONE', 3,
 ( #55607, #30181, #41425, #62879, #66192, #46336, #65834, #46002, #39429, #3105, #17631, #3783, #19616, #25254, #39099, #17985, #7074, #67469, #22905, #44715, #62176, #19263, #41076, #46690 ),
 .UNSPECIFIED., .F., .F.,
 ( 4, 2, 2, 2, 2, 2, 2, 2, 2, 2, 2, 4 ),
 ( 0.01054657901234073818, 0.01186033960812336516, 0.01251721990601467951, 0.01317410020390599387, 0.01448786079968862606, 0.01514474109757995256, 0.01580162139547127906, 0.01711538199125392859, 0.01777226228914526723, 0.01842914258703660935, 0.01974290318281925541, 0.02105666377860190147 ),
 .UNSPECIFIED. ) ;
#56512=CARTESIAN_POINT ( 'NONE',  ( 188.1848725084043110, 86.09288252323347024, -95.00000000000133582 ) ) ;
#56516=CARTESIAN_POINT ( 'NONE',  ( 156.9750372531276525, 58.53928062478365746, 83.09115216898715062 ) ) ;
#56520=CARTESIAN_POINT ( 'NONE',  ( -156.6862310659955710, 71.88416263379569671, 40.46439280054978838 ) ) ;
#56524=DIRECTION ( 'NONE',  ( 0.000000000000000000, 0.000000000000000000, 1.000000000000000000 ) ) ;
#56526=ORIENTED_EDGE ( 'NONE', *, *, #19929, .T. ) ;
#56527=CARTESIAN_POINT ( 'NONE',  ( 62.52742438962774685, 12.55954017561947822, 44.81296093922129131 ) ) ;
#56528=EDGE_CURVE ( 'NONE', #23369, #61020, #65767, .T. ) ;
#56531=CARTESIAN_POINT ( 'NONE',  ( -166.3231866619663037, 81.31146386205584520, 14.65755802791554174 ) ) ;
#56533=CARTESIAN_POINT ( 'NONE',  ( 20.74093720376648875, 6.709541214524347374, -75.51682261295336218 ) ) ;
#56534=B_SPLINE_CURVE_WITH_KNOTS ( 'NONE', 3,
 ( #12700, #51028, #2842, #19015, #61910, #13735, #28885, #2154, #23608, #4561, #67907, #41510, #51719, #9848, #3525, #63314, #36583, #20386, #57692, #24997, #14769, #52409, #68253, #20058, #46428, #10177, #26024, #53073, #19705, #25347, #35888, #9501, #41168, #52064, #68585, #36234, #46782, #62266, #62627, #14438, #58029, #62962, #35545, #21093, #15122, #20739, #25693, #31308, #63661, #4903 ),
 .UNSPECIFIED., .F., .F.,
 ( 4, 2, 2, 2, 2, 2, 2, 2, 2, 2, 2, 2, 2, 2, 2, 2, 2, 2, 2, 2, 2, 2, 2, 2, 4 ),
 ( 0.03126542424884321686, 0.03330676804260263718, 0.03534811183636205056, 0.03738945563012147089, 0.03943079942388089121, 0.04045147132076060137, 0.04147214321764031153, 0.04249281511452002169, 0.04351348701139972491, 0.04555483080515914524, 0.04657550270203887621, 0.04759617459891860025, 0.04810651054735845533, 0.04861684649579831041, 0.04963751839267802057, 0.05065819028955773073, 0.05167886218643744090, 0.05269953408331715106, 0.05372020598019686122, 0.05474087787707657138, 0.05576154977395628154, 0.05780289356771577125, 0.05984423736147527484, 0.06188558115523477149, 0.06392692494899426814 ),
 .UNSPECIFIED. ) ;
#56535=CARTESIAN_POINT ( 'NONE',  ( -132.2286325684322605, 52.04087929935078449, 68.98771376788437237 ) ) ;
#56536=ORIENTED_EDGE ( 'NONE', *, *, #25121, .F. ) ;
#56537=CARTESIAN_POINT ( 'NONE',  ( -97.11368346811575236, 31.34882221015812576, 86.26249857170712687 ) ) ;
#56539=CARTESIAN_POINT ( 'NONE',  ( -74.18622060908363380, 21.73430079572374396, -48.64965096766535879 ) ) ;
#56541=CARTESIAN_POINT ( 'NONE',  ( 204.6977192012829789, 108.0580384837235073, -63.17048162308526571 ) ) ;
#56542=CARTESIAN_POINT ( 'NONE',  ( 139.2794027252094224, 45.99190465195511024, 42.21385594671063046 ) ) ;
#56544=CARTESIAN_POINT ( 'NONE',  ( 113.8724110608469005, 31.71510301790680941, 30.53043836141040046 ) ) ;
#56546=CARTESIAN_POINT ( 'NONE',  ( 66.30636076182545935, 14.49616748423541424, -63.30812756663202379 ) ) ;
#56548=B_SPLINE_CURVE_WITH_KNOTS ( 'NONE', 3,
 ( #50954, #55174, #2766, #17903, #43915, #36504, #67484, #19632, #67833, #3123, #41784, #51986, #29842, #41093, #62194, #57619, #30887, #9086, #24583, #51650, #14011, #57956, #41440, #30537, #62895, #14698, #61837, #24920, #13663, #68184, #46708, #51312, #62554, #15050, #36160, #3803, #14364, #35821, #19280, #9776, #31238, #57274, #25271, #19988, #68512 ),
 .UNSPECIFIED., .F., .F.,
 ( 4, 2, 2, 2, 2, 2, 2, 2, 1, 2, 2, 2, 2, 2, 2, 2, 2, 2, 2, 2, 2, 2, 4 ),
 ( 0.000000000000000000, 0.001470449819620692038, 0.002205674729431027214, 0.002940899639241362391, 0.004411349458862014530, 0.005881799278482666669, 0.007352249098103315339, 0.008087474007913642710, 0.008822698917723968345, 0.009557923827534293981, 0.01029314873734462135, 0.01176359855696526915, 0.01249882346677558959, 0.01323404837658591002, 0.01470449819620655435, 0.01543972310601688346, 0.01617494801582720909, 0.01764539783544786383, 0.01911584765506852204, 0.01985107256487885982, 0.02058629747468919760, 0.02205674729430986969, 0.02352719711393054525 ),
 .UNSPECIFIED. ) ;
#56553=CARTESIAN_POINT ( 'NONE',  ( 8.000000000000007105, 249.8719672152120381, -95.00000000000133582 ) ) ;
#56555=CARTESIAN_POINT ( 'NONE',  ( -54.20011053040712312, 14.45452627381339461, -88.95099551034488172 ) ) ;
#56557=CARTESIAN_POINT ( 'NONE',  ( -142.2626321327577443, 58.26997216742664421, 36.26161877387822585 ) ) ;
#56558=CARTESIAN_POINT ( 'NONE',  ( -128.1384526288949814, 47.98891607499721346, 57.79359961142665014 ) ) ;
#56559=CARTESIAN_POINT ( 'NONE',  ( -165.9986675144415642, 79.53506019208350608, -66.68918146554828752 ) ) ;
#56561=B_SPLINE_CURVE_WITH_KNOTS ( 'NONE', 3,
 ( #35616, #57070, #8883, #25757, #31372, #5651, #4298, #47187, #42936, #21161, #27110, #36650, #4624, #26088, #26780, #48206, #21833, #64403, #42605, #68643, #64059, #31, #381, #59116, #37317, #69338, #20455, #10242, #26439, #53832, #16215, #63380, #52801, #41918, #21486, #15871, #58096, #15190, #53139, #15538, #5322, #63728, #47875 ),
 .UNSPECIFIED., .F., .F.,
 ( 4, 2, 2, 2, 2, 2, 2, 2, 2, 2, 2, 2, 1, 2, 2, 2, 2, 2, 2, 2, 2, 4 ),
 ( 0.02362927190606132002, 0.02510248541563186997, 0.02583909217041715015, 0.02657569892520242685, 0.02804891243477298374, 0.02952212594434354409, 0.03025873269912882080, 0.03099533945391410097, 0.03246855296348467868, 0.03394176647305524597, 0.03541497998262582714, 0.03615158673741111772, 0.03688819349219642219, 0.03762480024698171971, 0.03836140700176701723, 0.03983462051133761228, 0.04130783402090821427, 0.04278104753047881625, 0.04351765428526410684, 0.04425426104004939742, 0.04572747454961999247, 0.04720068805919059446 ),
 .UNSPECIFIED. ) ;
#56563=CARTESIAN_POINT ( 'NONE',  ( -102.7447593990059289, 34.14748189312174276, 30.51907450641510522 ) ) ;
#56565=CARTESIAN_POINT ( 'NONE',  ( -176.9364071963078686, 91.47427511280444890, -89.38709468048955387 ) ) ;
#56568=CARTESIAN_POINT ( 'NONE',  ( 83.38619203015946368, 19.39783821526630803, 57.27713636182927814 ) ) ;
#56571=CARTESIAN_POINT ( 'NONE',  ( -189.2352924136013428, 107.0839554967701162, -69.40233452781009760 ) ) ;
#56575=CARTESIAN_POINT ( 'NONE',  ( -15.32584732649904424, 8.506915958926391852, -42.42966520005830233 ) ) ;
#56580=ORIENTED_EDGE ( 'NONE', *, *, #54622, .T. ) ;
#56582=CARTESIAN_POINT ( 'NONE',  ( -60.66101049381766330, 17.30588917955501671, 69.66552825106393243 ) ) ;
#56584=ORIENTED_EDGE ( 'NONE', *, *, #62660, .T. ) ;
#56586=CARTESIAN_POINT ( 'NONE',  ( 154.4435090467314922, 56.59612921827835663, -63.60279279905601868 ) ) ;
#56587=CARTESIAN_POINT ( 'NONE',  ( -38.93878980550034896, 10.94326053663842302, 38.21361434711087668 ) ) ;
#56588=CARTESIAN_POINT ( 'NONE',  ( 135.6842057900327347, 42.53841116629840968, -36.23475628795622328 ) ) ;
#56592=CARTESIAN_POINT ( 'NONE',  ( -119.5576859660651508, 42.46117483543969939, 34.09885795874915715 ) ) ;
#56593=CARTESIAN_POINT ( 'NONE',  ( -61.86845765289634613, 16.61548683002701665, -45.85609512080901595 ) ) ;
#56594=VERTEX_POINT ( 'NONE', #48359 ) ;
#56595=CARTESIAN_POINT ( 'NONE',  ( -180.2243452982808662, 96.99029284948635166, -66.63178993611138878 ) ) ;
#56597=CARTESIAN_POINT ( 'NONE',  ( 128.9420992581156042, 39.69520347227675217, 85.02391764104523020 ) ) ;
#56598=CARTESIAN_POINT ( 'NONE',  ( 111.1767565371974769, 29.31586421952251698, 29.65471990763289512 ) ) ;
#56601=CARTESIAN_POINT ( 'NONE',  ( -122.7930600691577894, 44.48546375740913561, -62.41358845972529679 ) ) ;
#56602=ORIENTED_EDGE ( 'NONE', *, *, #44367, .F. ) ;
#56603=CARTESIAN_POINT ( 'NONE',  ( 197.1974290009104891, 96.59277840252784131, 36.38369672051224057 ) ) ;
#56606=CARTESIAN_POINT ( 'NONE',  ( 69.49862690228272299, 14.27023134440514340, 60.35422735765934021 ) ) ;
#56612=CARTESIAN_POINT ( 'NONE',  ( 164.1352994389932576, 64.33767534192698179, -20.22913284204803475 ) ) ;
#56614=EDGE_CURVE ( 'NONE', #30648, #35148, #67001, .T. ) ;
#56617=CARTESIAN_POINT ( 'NONE',  ( 129.7260862822010665, 38.98566587309944964, 84.43068361936597910 ) ) ;
#56621=CARTESIAN_POINT ( 'NONE',  ( -142.8450945664715448, 58.72815783657284783, -65.70266265617578938 ) ) ;
#56622=EDGE_CURVE ( 'NONE', #37519, #629, #60243, .T. ) ;
#56625=CARTESIAN_POINT ( 'NONE',  ( 164.9559213734324885, 63.71338633026439879, -43.08067803092567516 ) ) ;
#56626=ORIENTED_EDGE ( 'NONE', *, *, #55645, .T. ) ;
#56627=LINE ( 'NONE', #56982, #58068 ) ;
#56628=DIRECTION ( 'NONE',  ( -0.000000000000000000, 1.000000000000000000, -0.000000000000000000 ) ) ;
#56629=CARTESIAN_POINT ( 'NONE',  ( 152.0703578754941248, 54.82056822058789436, -92.09310849956577272 ) ) ;
#56631=CARTESIAN_POINT ( 'NONE',  ( -143.6073342927367946, 59.33214134111805294, -91.36572565367391974 ) ) ;
#56638=EDGE_CURVE ( 'NONE', #22146, #62158, #62421, .T. ) ;
#56639=EDGE_CURVE ( 'NONE', #33379, #8399, #63694, .T. ) ;
#56640=CARTESIAN_POINT ( 'NONE',  ( -155.5977325361978103, 70.88311713755696530, -37.92850440926633837 ) ) ;
#56642=CARTESIAN_POINT ( 'NONE',  ( -38.54712373114178092, 11.89174538567467820, 35.27342008138545282 ) ) ;
#56644=CARTESIAN_POINT ( 'NONE',  ( -156.6819053601226130, 70.51177710383653618, -66.89866658464235627 ) ) ;
#56646=CARTESIAN_POINT ( 'NONE',  ( -48.32993240732255913, 12.98137013984324817, -66.19890796893723461 ) ) ;
#56648=CARTESIAN_POINT ( 'NONE',  ( 179.4279766878530040, 76.94722012158231905, 2.637092671877164118 ) ) ;
#56649=CARTESIAN_POINT ( 'NONE',  ( 111.1868021579656727, 29.32055685204859330, 17.72207817859029078 ) ) ;
#56650=ORIENTED_EDGE ( 'NONE', *, *, #47020, .F. ) ;
#56655=B_SPLINE_CURVE_WITH_KNOTS ( 'NONE', 3,
 ( #30389, #51840, #25127, #41635, #68703, #57814, #20513, #63438, #34981, #56425, #31427, #69035, #20866, #37047, #799, #64819, #27168, #42325, #48265, #21218, #58483, #43688, #15931, #48605, #63788, #10299, #36711, #27516, #9975, #4683, #37377, #15596, #58834, #92, #37732, #5027, #31769, #43346, #26150, #6057, #26493, #22253, #69399, #38075, #21546, #47928, #32806, #16618, #5382, #42993, #64464, #16276, #42664, #59175, #10646 ),
 .UNSPECIFIED., .F., .F.,
 ( 4, 2, 2, 2, 2, 2, 2, 2, 2, 2, 2, 2, 2, 2, 2, 2, 2, 2, 2, 1, 2, 2, 2, 2, 2, 2, 2, 4 ),
 ( 0.000000000000000000, 0.001947665408787207977, 0.002921498113180811748, 0.003895330817574415953, 0.004869163521968020159, 0.005842996226361623496, 0.006816828930755227701, 0.007790661635148831907, 0.009738327043936040317, 0.01071215974832964365, 0.01168599245272324699, 0.01265982515711685207, 0.01363365786151045540, 0.01460749056590405874, 0.01558132327029766381, 0.01752898867908487396, 0.01850282138347847383, 0.01947665408787208063, 0.02045048679226568397, 0.02142431949665928731, 0.02239815220105289065, 0.02337198490544649399, 0.02434581760984010079, 0.02531965031423370413, 0.02726731572302086917, 0.02824114842741447598, 0.02921498113180807585, 0.03116264654059524436 ),
 .UNSPECIFIED. ) ;
#56656=CARTESIAN_POINT ( 'NONE',  ( 46.23304607317102466, 10.41544405387738337, -19.38122357973218968 ) ) ;
#56660=CARTESIAN_POINT ( 'NONE',  ( -9.450810044394341247, 7.002157412775469325, 83.97576989457125762 ) ) ;
#56663=CARTESIAN_POINT ( 'NONE',  ( 141.0229350107040887, 45.92325889728665800, -95.00000000000133582 ) ) ;
#56666=VECTOR ( 'NONE', #28184, 1000.000000000000000 ) ;
#56672=CARTESIAN_POINT ( 'NONE',  ( 105.8229724512851107, 27.98935528750253710, 57.89168491306591591 ) ) ;
#56678=CARTESIAN_POINT ( 'NONE',  ( 209.5118425285948831, 113.1852661712287329, 15.61864072547802351 ) ) ;
#56679=CARTESIAN_POINT ( 'NONE',  ( -143.2587158300142107, 60.34092810886539837, 42.37670143261917843 ) ) ;
#56681=EDGE_CURVE ( 'NONE', #30296, #17040, #41315, .T. ) ;
#56682=CARTESIAN_POINT ( 'NONE',  ( 12.53962518824996408, 6.418270956987105258, -89.93529441773186761 ) ) ;
#56686=VERTEX_POINT ( 'NONE', #23751 ) ;
#56691=CARTESIAN_POINT ( 'NONE',  ( 21.54731028615039534, 6.753297381550458667, 86.38792578528536126 ) ) ;
#56692=CARTESIAN_POINT ( 'NONE',  ( 83.60262962804348774, 18.41036205028015260, -77.03250514454457232 ) ) ;
#56694=CARTESIAN_POINT ( 'NONE',  ( -196.7348448768811409, -170.0000000000000000, -95.80018497893539120 ) ) ;
#56699=LINE ( 'NONE', #56014, #38473 ) ;
#56703=LINE ( 'NONE', #3246, #63482 ) ;
#56704=CYLINDRICAL_SURFACE ( 'NONE', #3281, 7.500000000000020428 ) ;
#56705=EDGE_LOOP ( 'NONE', ( #57184, #48164, #4263, #14001 ) ) ;
#56711=CARTESIAN_POINT ( 'NONE',  ( 107.2614272668149056, 28.62909081796204092, 17.15260657237848463 ) ) ;
#56717=CARTESIAN_POINT ( 'NONE',  ( 177.0027897064244655, 75.97676392242549070, -64.26111881574348672 ) ) ;
#56720=CARTESIAN_POINT ( 'NONE',  ( 115.0454575488273434, 31.16784721673997893, -22.34374271908251686 ) ) ;
#56721=CARTESIAN_POINT ( 'NONE',  ( 83.59652366361575559, 19.46709838196857945, -36.45791133507715642 ) ) ;
#56727=CARTESIAN_POINT ( 'NONE',  ( 43.14356474118743989, 8.925336319666879348, 4.050586556182519615 ) ) ;
#56728=CARTESIAN_POINT ( 'NONE',  ( 178.1965488566139868, 77.14488558164482868, 3.028789085135533465 ) ) ;
#56729=CARTESIAN_POINT ( 'NONE',  ( -38.02163356681019479, 11.78964455120423693, 94.99999999999866418 ) ) ;
#56730=CARTESIAN_POINT ( 'NONE',  ( 210.6189312023034574, 114.8321746285510301, 94.99999999999866418 ) ) ;
#56732=CARTESIAN_POINT ( 'NONE',  ( -55.05276343752909440, 15.72344139423348430, 3.472777182467473800 ) ) ;
#56734=CARTESIAN_POINT ( 'NONE',  ( 211.8348321742968778, 118.5227572644700160, 92.73579468022644789 ) ) ;
#56735=CARTESIAN_POINT ( 'NONE',  ( 212.1669304543881935, 119.0398299474538675, 36.00701586133611443 ) ) ;
#56736=CARTESIAN_POINT ( 'NONE',  ( -81.89510452344296709, 24.66033552777453863, 57.97658800716016003 ) ) ;
#56738=ORIENTED_EDGE ( 'NONE', *, *, #15580, .T. ) ;
#56739=CARTESIAN_POINT ( 'NONE',  ( 12.91653430408660697, 7.431946598423014194, -23.11569640008216098 ) ) ;
#56740=VERTEX_POINT ( 'NONE', #9992 ) ;
#56741=CARTESIAN_POINT ( 'NONE',  ( 200.8410151090926092, 101.2014854111317277, -10.53460766635205559 ) ) ;
#56744=CARTESIAN_POINT ( 'NONE',  ( 188.5838389098762775, 88.03667982118678026, -70.26040297313004146 ) ) ;
#56745=CARTESIAN_POINT ( 'NONE',  ( -38.55173488399534421, 11.89269613674691328, 93.80691191228474679 ) ) ;
#56746=CARTESIAN_POINT ( 'NONE',  ( -95.86612279493103017, 29.64021615886205652, -38.61911933511777306 ) ) ;
#56747=B_SPLINE_CURVE_WITH_KNOTS ( 'NONE', 3,
 ( #25090, #68345, #14863, #63059, #10272, #32433, #60, #69367, #15904, #64090, #26806, #38395, #69010, #64785, #42633, #59835, #10614, #33130 ),
 .UNSPECIFIED., .F., .F.,
 ( 4, 2, 2, 2, 2, 2, 2, 2, 4 ),
 ( 0.01321666563952497188, 0.01669835041696196912, 0.01843919280568048769, 0.02018003519439900625, 0.02192087758311752482, 0.02366171997183604339, 0.02540256236055456196, 0.02627298355491380216, 0.02714340474927304583 ),
 .UNSPECIFIED. ) ;
#56748=CARTESIAN_POINT ( 'NONE',  ( 31.90184941268614693, 7.552181687745345151, -43.36186114419296445 ) ) ;
#56750=CARTESIAN_POINT ( 'NONE',  ( 15.29305096970403000, 7.491604910111008486, -35.51894409868578606 ) ) ;
#56751=DIRECTION ( 'NONE',  ( -0.000000000000000000, 1.000000000000000000, -0.000000000000000000 ) ) ;
#56754=VECTOR ( 'NONE', #7437, 1000.000000000000000 ) ;
#56755=FACE_OUTER_BOUND ( 'NONE', #5056, .T. ) ;
#56761=ORIENTED_EDGE ( 'NONE', *, *, #50768, .T. ) ;
#56765=CARTESIAN_POINT ( 'NONE',  ( -60.66101049381764909, 17.30588917955502026, -64.55722470125444090 ) ) ;
#56768=CARTESIAN_POINT ( 'NONE',  ( -179.2262621278718200, 94.19039042964671182, -37.82663789750925787 ) ) ;
#56769=CARTESIAN_POINT ( 'NONE',  ( 105.8022841538864185, 26.88074187880708976, 4.203527470635210150 ) ) ;
#56770=CARTESIAN_POINT ( 'NONE',  ( -24.71604178686820319, 9.599501655372948861, 61.22755308168638777 ) ) ;
#56773=AXIS2_PLACEMENT_3D ( 'NONE', #28229, #18042, #39158 ) ;
#56776=CARTESIAN_POINT ( 'NONE',  ( -1.876547441458561005, 6.576559737910137038, 59.88607102599485188 ) ) ;
#56781=CARTESIAN_POINT ( 'NONE',  ( -52.66507163626136645, 14.05394608175174653, -35.59014718343654238 ) ) ;
#56784=B_SPLINE_CURVE_WITH_KNOTS ( 'NONE', 3,
 ( #29566, #62268, #40130, #51030, #67558, #57003, #19708, #2844, #19358, #40814, #13062, #61239, #8470, #29229, #61587, #40468, #13399, #19017, #51721, #14088, #34522, #50675, #46430, #56298, #24311, #30272, #7777, #34861, #8822, #45399, #3527, #67232, #25000, #39778, #23950, #66881, #45752, #18677, #61912, #67909, #41170, #40004, #38971, #12939, #28052, #55127, #61114 ),
 .UNSPECIFIED., .F., .F.,
 ( 4, 2, 2, 2, 2, 2, 2, 2, 2, 2, 2, 2, 1, 2, 2, 2, 2, 2, 2, 2, 2, 2, 2, 4 ),
 ( 1.734723475976807094E-18, 0.001493793014771601681, 0.002240689522157399919, 0.002987586029543198157, 0.004481379044314774684, 0.005228275551700562948, 0.005975172059086351212, 0.007468965073857914728, 0.008215861581243703859, 0.008962758088629493858, 0.01045655110340106171, 0.01120344761078684824, 0.01195034411817263130, 0.01269724062555841609, 0.01344413713294419915, 0.01493793014771577048, 0.01568482665510155527, 0.01643172316248733139, 0.01792551617725889751, 0.01941930919203046363, 0.02016620569941623281, 0.02091310220680200893, 0.02240689522157355423, 0.02390068823634509954 ),
 .UNSPECIFIED. ) ;
#56787=EDGE_CURVE ( 'NONE', #15010, #25468, #58610, .T. ) ;
#56789=VERTEX_POINT ( 'NONE', #6075 ) ;
#56799=CARTESIAN_POINT ( 'NONE',  ( -2.874437057892795355, 6.618922960888052209, 5.116205444759493126 ) ) ;
#56801=CARTESIAN_POINT ( 'NONE',  ( -79.62207341875655686, 23.76621716825512109, 45.37247973810714541 ) ) ;
#56802=CARTESIAN_POINT ( 'NONE',  ( 156.9739725704451985, 57.26595269248011988, 83.10889256476860965 ) ) ;
#56803=CARTESIAN_POINT ( 'NONE',  ( 134.7770330630253284, 41.98246829846536343, 17.62339256512675689 ) ) ;
#56804=VERTEX_POINT ( 'NONE', #1508 ) ;
#56808=CARTESIAN_POINT ( 'NONE',  ( 45.90128843543708115, 9.343910238294478532, -46.89477593665989019 ) ) ;
#56809=CARTESIAN_POINT ( 'NONE',  ( -76.58306521830746760, 22.61222690308086669, 84.39593471637930122 ) ) ;
#56815=ADVANCED_FACE ( 'NONE', ( #66251 ), #54612, .T. ) ;
#56819=CARTESIAN_POINT ( 'NONE',  ( -142.0062637385109952, 58.06920992247431457, 65.61584438720122137 ) ) ;
#56820=CARTESIAN_POINT ( 'NONE',  ( 79.22872707466397912, 18.07970189365809688, 38.45465439937479601 ) ) ;
#56821=CARTESIAN_POINT ( 'NONE',  ( 197.1974290009105459, 96.59277840252785552, -70.99450564134252772 ) ) ;
#56824=CARTESIAN_POINT ( 'NONE',  ( 188.0141161196706321, 85.90515114331884661, -13.99854441431428498 ) ) ;
#56826=CARTESIAN_POINT ( 'NONE',  ( -85.66184035008926401, 26.20110535976566979, -13.05454194820700486 ) ) ;
#56827=CARTESIAN_POINT ( 'NONE',  ( -173.9617926765114362, 89.58633395456783433, -7.902830288932056746 ) ) ;
#56829=CARTESIAN_POINT ( 'NONE',  ( -48.71337292867757895, 14.10768470390589258, 41.83269798608346690 ) ) ;
#56832=CARTESIAN_POINT ( 'NONE',  ( -107.7886332494339143, 36.81249801143971467, 16.28760631461256736 ) ) ;
#56834=CARTESIAN_POINT ( 'NONE',  ( 162.6190874793280159, 61.76782592053311305, 58.29531679009903655 ) ) ;
#56835=CARTESIAN_POINT ( 'NONE',  ( -189.8071159312682994, 107.8771087123619878, 62.38726094205951256 ) ) ;
#56836=CARTESIAN_POINT ( 'NONE',  ( 188.2076037774874635, 86.11782719225438143, -46.08847689396432656 ) ) ;
#56838=CARTESIAN_POINT ( 'NONE',  ( 163.1495034066983862, 62.20479872133083887, -65.54385288365227780 ) ) ;
#56839=EDGE_LOOP ( 'NONE', ( #32608, #67605, #32367, #14513 ) ) ;
#56842=CARTESIAN_POINT ( 'NONE',  ( -71.23432872518910131, 19.62839606228986256, 90.54878966649707195 ) ) ;
#56844=CARTESIAN_POINT ( 'NONE',  ( 66.73594759725095571, 13.56641407806657007, -36.70390389039621937 ) ) ;
#56846=CARTESIAN_POINT ( 'NONE',  ( -61.76386578474847511, 17.63453064612500754, 34.43260724535770123 ) ) ;
#56847=CARTESIAN_POINT ( 'NONE',  ( -38.87871322265797858, 11.95691939779335300, -68.68042223677132085 ) ) ;
#56849=CARTESIAN_POINT ( 'NONE',  ( 55.52751777340356654, 12.08567914268658505, 37.80264004355908725 ) ) ;
#56850=CARTESIAN_POINT ( 'NONE',  ( 44.25717266065687028, 9.090606898751403264, 85.37709734524574401 ) ) ;
#56853=CARTESIAN_POINT ( 'NONE',  ( -2.190131154568196070, 6.589492063460818727, -47.87333299203348957 ) ) ;
#56855=CARTESIAN_POINT ( 'NONE',  ( -119.5267374018686866, 42.44190186039715229, 15.27167418143519484 ) ) ;
#56857=CARTESIAN_POINT ( 'NONE',  ( 128.3856248084844935, 38.21741401878868771, -21.83233341589641796 ) ) ;
#56860=CARTESIAN_POINT ( 'NONE',  ( 86.62931800182293784, -170.0000000000000000, 90.90118875340668581 ) ) ;
#56862=VERTEX_POINT ( 'NONE', #38806 ) ;
#56865=CARTESIAN_POINT ( 'NONE',  ( 127.4992165631961569, 38.87141012667722606, -47.53367025290549464 ) ) ;
#56867=CARTESIAN_POINT ( 'NONE',  ( 55.76286625948333864, 12.13284185313540142, -95.00000000000133582 ) ) ;
#56868=CARTESIAN_POINT ( 'NONE',  ( 183.7875981612219505, 82.83906702837190039, -36.72598982284740998 ) ) ;
#56873=EDGE_LOOP ( 'NONE', ( #62772, #35241, #67820, #15692 ) ) ;
#56874=CARTESIAN_POINT ( 'NONE',  ( -28.81317668042940028, 9.175023678939290050, -23.00213673641785306 ) ) ;
#56877=CARTESIAN_POINT ( 'NONE',  ( 200.4590013143046860, 102.3556155835303088, 3.658552749324740727 ) ) ;
#56881=CARTESIAN_POINT ( 'NONE',  ( 150.0666142602886168, 53.35666697496139932, 89.34269639003078112 ) ) ;
#56883=CARTESIAN_POINT ( 'NONE',  ( 126.4757069339777473, 38.29528077539269049, -71.72474436022167765 ) ) ;
#56884=CARTESIAN_POINT ( 'NONE',  ( 128.0848616812662613, 38.04676222636084049, 41.82567121914378561 ) ) ;
#56891=CARTESIAN_POINT ( 'NONE',  ( 56.30171512200999473, 11.21502580416395922, 40.66478564769037263 ) ) ;
#56894=CARTESIAN_POINT ( 'NONE',  ( -165.7140086129056158, 80.68381997492572566, 10.26169782557952992 ) ) ;
#56895=CARTESIAN_POINT ( 'NONE',  ( 21.88606409348644277, 6.772455198693823952, -74.23695490937706154 ) ) ;
#56896=CARTESIAN_POINT ( 'NONE',  ( -127.4644500646575125, 48.74852676951795161, 57.62729058137536953 ) ) ;
#56897=ORIENTED_EDGE ( 'NONE', *, *, #68516, .T. ) ;
#56899=CARTESIAN_POINT ( 'NONE',  ( -71.42546113164834765, 20.75891408601218657, -40.59665863684374898 ) ) ;
#56901=CARTESIAN_POINT ( 'NONE',  ( 212.0779786303466210, 118.9010947973413437, -72.04810227374618137 ) ) ;
#56904=DIRECTION ( 'NONE',  ( -0.000000000000000000, -1.000000000000000000, 0.000000000000000000 ) ) ;
#56905=CARTESIAN_POINT ( 'NONE',  ( -129.6079169496901784, 50.20899308323959787, 17.79538119927901718 ) ) ;
#56906=CARTESIAN_POINT ( 'NONE',  ( 63.49941241090385802, 13.81848793187418423, -77.56524142263344856 ) ) ;
#56910=CARTESIAN_POINT ( 'NONE',  ( 8.678106553679038271, 7.383286152329689322, -94.17589882202238982 ) ) ;
#56918=CARTESIAN_POINT ( 'NONE',  ( 65.39792658623288446, 14.27332852928127949, -36.10495004355786364 ) ) ;
#56920=CARTESIAN_POINT ( 'NONE',  ( -166.5686015187717999, 80.11916873959174268, -65.39727901222690321 ) ) ;
#56921=ORIENTED_EDGE ( 'NONE', *, *, #50561, .F. ) ;
#56922=CARTESIAN_POINT ( 'NONE',  ( -109.6752351740181410, 37.84903014964772439, 39.29581709369001885 ) ) ;
#56924=CARTESIAN_POINT ( 'NONE',  ( -34.74740905761646559, 10.15745573515589228, 17.62056773612129135 ) ) ;
#56933=CARTESIAN_POINT ( 'NONE',  ( -15.32495246574476155, 8.506829480038513580, -43.42002976355023947 ) ) ;
#56937=ORIENTED_EDGE ( 'NONE', *, *, #29596, .F. ) ;
#56938=CARTESIAN_POINT ( 'NONE',  ( -56.02358673658415000, 14.94347049174936792, 30.36477236479575126 ) ) ;
#56939=CARTESIAN_POINT ( 'NONE',  ( -60.64199216239837398, 17.30050036439947547, 59.65478111955487606 ) ) ;
#56940=FACE_OUTER_BOUND ( 'NONE', #43102, .T. ) ;
#56943=CARTESIAN_POINT ( 'NONE',  ( -57.36093876233154276, 15.31244721770222306, -89.26622691136491028 ) ) ;
#56945=CARTESIAN_POINT ( 'NONE',  ( -33.84080342750781512, 9.997552308299097135, 30.59459340086282353 ) ) ;
#56946=CARTESIAN_POINT ( 'NONE',  ( 135.6651581599210203, 42.52720121194707303, -50.80564077755548169 ) ) ;
#56952=FACE_OUTER_BOUND ( 'NONE', #43874, .T. ) ;
#56953=EDGE_LOOP ( 'NONE', ( #29598, #19623 ) ) ;
#56954=CARTESIAN_POINT ( 'NONE',  ( -178.5750994113944330, 94.98114813978523330, -74.22894033587822094 ) ) ;
#56955=CARTESIAN_POINT ( 'NONE',  ( 130.5700081980325251, 40.64031760446221853, 83.95029887580108152 ) ) ;
#56957=CARTESIAN_POINT ( 'NONE',  ( 115.7746371641014775, 31.52600568297706829, 42.19931404672254871 ) ) ;
#56961=CARTESIAN_POINT ( 'NONE',  ( -118.4622862908118890, 41.79153065058245886, -68.21174534165025705 ) ) ;
#56963=CARTESIAN_POINT ( 'NONE',  ( 200.4559562755961792, 100.7034888016685557, 30.50516796803767150 ) ) ;
#56964=CARTESIAN_POINT ( 'NONE',  ( 112.5721302457195634, 29.97407549554797868, -63.12220954116383353 ) ) ;
#56965=CARTESIAN_POINT ( 'NONE',  ( 70.50372867914782660, 14.53505678900967624, 64.64800341258842309 ) ) ;
#56966=CARTESIAN_POINT ( 'NONE',  ( 141.0792860804899362, 47.16255757051794006, 8.074677092446195914 ) ) ;
#56971=CARTESIAN_POINT ( 'NONE',  ( 164.9547823171480161, 65.03046442419434925, -17.33931518955914441 ) ) ;
#56974=DIRECTION ( 'NONE',  ( -0.000000000000000000, 1.000000000000000000, -0.000000000000000000 ) ) ;
#56975=CARTESIAN_POINT ( 'NONE',  ( 133.3039865199672533, 41.09165617245334801, 83.21332837341623190 ) ) ;
#56978=CARTESIAN_POINT ( 'NONE',  ( 159.2325040199866919, 60.31699144791974732, -36.27868694413073314 ) ) ;
#56980=CARTESIAN_POINT ( 'NONE',  ( 162.0835148203877054, 61.32844276806159911, -49.55681444341564656 ) ) ;
#56982=CARTESIAN_POINT ( 'NONE',  ( 218.0000000000000000, 126.6235316737731296, 94.99999999999866418 ) ) ;
#56983=CARTESIAN_POINT ( 'NONE',  ( -130.5740389938243311, 49.65308610043483384, 44.00008722492239599 ) ) ;
#56985=CARTESIAN_POINT ( 'NONE',  ( 86.62931800182293784, 20.48449268398422518, -23.97701360844805407 ) ) ;
#56986=CARTESIAN_POINT ( 'NONE',  ( -172.3057147739577033, 86.22480007276998037, 30.85461157478519212 ) ) ;
#56990=CARTESIAN_POINT ( 'NONE',  ( -95.21085197937826194, 30.44372064875430439, 67.42056744027632931 ) ) ;
#56991=CARTESIAN_POINT ( 'NONE',  ( -10.24974837193995469, 8.069704751038631940, 71.57424783662469281 ) ) ;
#56992=ORIENTED_EDGE ( 'NONE', *, *, #27629, .T. ) ;
#56993=CARTESIAN_POINT ( 'NONE',  ( 152.8373718734504791, 55.38925997611394791, -10.86163724592964819 ) ) ;
#56995=CARTESIAN_POINT ( 'NONE',  ( 103.0004140566503423, 26.76634862952792915, 39.12544781792537663 ) ) ;
#56997=CARTESIAN_POINT ( 'NONE',  ( -1.328627985309864146, 7.561890325089883014, 33.86022777313294085 ) ) ;
#56999=CARTESIAN_POINT ( 'NONE',  ( 62.71028589264315656, 12.60192304540389863, 83.50116889568769807 ) ) ;
#57003=CARTESIAN_POINT ( 'NONE',  ( -57.42615654242917600, 15.33060010148602714, 18.09145754529776084 ) ) ;
#57010=VECTOR ( 'NONE', #19384, 1000.000000000000000 ) ;
#57013=CARTESIAN_POINT ( 'NONE',  ( -2.533432677019553658, 6.603837116479292391, 85.96053544918321165 ) ) ;
#57017=CARTESIAN_POINT ( 'NONE',  ( 61.01080120047389244, 13.24737680938180695, -89.67107551088051309 ) ) ;
#57019=CARTESIAN_POINT ( 'NONE',  ( -165.6212796729685408, 79.15047440262053158, 64.85932769107682816 ) ) ;
#57020=ORIENTED_EDGE ( 'NONE', *, *, #22542, .T. ) ;
#57022=CARTESIAN_POINT ( 'NONE',  ( -154.2585856850055279, 68.31650218414627318, 32.41269129084507483 ) ) ;
#57024=CARTESIAN_POINT ( 'NONE',  ( 157.4703587214989398, -170.0000000000000000, -16.77963370867396975 ) ) ;
#57027=AXIS2_PLACEMENT_3D ( 'NONE', #22030, #38554, #11461 ) ;
#57030=CARTESIAN_POINT ( 'NONE',  ( 55.91494169499917177, 12.16343363043255899, -13.94887811350051798 ) ) ;
#57031=EDGE_LOOP ( 'NONE', ( #21558, #23295, #15166, #32612 ) ) ;
#57034=CARTESIAN_POINT ( 'NONE',  ( 211.0967808702091304, 115.5516932918877586, 5.941490033705162155 ) ) ;
#57035=CARTESIAN_POINT ( 'NONE',  ( 9.275903038161098735, 7.385619229189523516, 68.11142882406396382 ) ) ;
#57036=CARTESIAN_POINT ( 'NONE',  ( 211.5066273949819333, 116.1727691518061505, 33.51412873826703986 ) ) ;
#57037=CARTESIAN_POINT ( 'NONE',  ( 8.000000000000007105, 249.8719672152120381, 0.000000000000000000 ) ) ;
#57038=B_SPLINE_CURVE_WITH_KNOTS ( 'NONE', 3,
 ( #37964, #43577, #41949, #28098, #20835, #9945, #17188, #1030, #22480, #38660, #42296, #17552, #63757, #22831, #44271, #65755, #59408, #11220, #39020, #60464, #32686, #12278, #63412, #55177, #7000, #47215, #68673, #31401, #61840, #51314, #1727, #34787, #34093, #66808, #2768, #40055, #24235, #35120, #40395, #55527, #56226, #45682, #7358, #50605, #18247, #23879, #8042 ),
 .UNSPECIFIED., .F., .F.,
 ( 4, 2, 2, 2, 2, 2, 2, 2, 2, 2, 2, 1, 2, 2, 2, 2, 2, 2, 2, 2, 2, 2, 2, 4 ),
 ( 0.000000000000000000, 0.003297771944419005796, 0.004122214930523721357, 0.004946657916628437353, 0.006595543888837858068, 0.007419986874942590543, 0.008244429861047323019, 0.009068872847152055494, 0.009893315833256787969, 0.01154220180546625119, 0.01236664479157098366, 0.01319108777767571614, 0.01401553076378044688, 0.01483997374988517762, 0.01566441673598990836, 0.01648885972209463910, 0.01813774569430405201, 0.01896218868040878622, 0.01978663166651352043, 0.02061107465261825464, 0.02143551763872298885, 0.02308440361093245380, 0.02473328958314192222, 0.02638217555535139064 ),
 .UNSPECIFIED. ) ;
#57040=VERTEX_POINT ( 'NONE', #26002 ) ;
#57043=CARTESIAN_POINT ( 'NONE',  ( -132.3448531020190160, 52.12286071311145719, 87.93207172015587503 ) ) ;
#57044=CARTESIAN_POINT ( 'NONE',  ( 32.30062460741315533, 8.603096374765343057, -72.38972614245851389 ) ) ;
#57046=CARTESIAN_POINT ( 'NONE',  ( 18.37289129162609314, 6.596424546175636117, 84.13215553489163767 ) ) ;
#57047=CARTESIAN_POINT ( 'NONE',  ( 79.11678624235125312, 16.99307331934756604, -70.15752560060720100 ) ) ;
#57052=ORIENTED_EDGE ( 'NONE', *, *, #9525, .F. ) ;
#57060=ORIENTED_EDGE ( 'NONE', *, *, #12915, .T. ) ;
#57061=CARTESIAN_POINT ( 'NONE',  ( 14.80582440982707659, 6.470883766728822373, -35.56753452839079443 ) ) ;
#57062=CARTESIAN_POINT ( 'NONE',  ( -109.6064662507157266, 37.81086785902052583, -94.52989562943487556 ) ) ;
#57066=CARTESIAN_POINT ( 'NONE',  ( -30.17641273894449938, 9.386748470934174193, 83.98431897038294380 ) ) ;
#57067=CARTESIAN_POINT ( 'NONE',  ( -51.34542473642582650, 14.75635007918829267, 4.448568100648282453 ) ) ;
#57069=CARTESIAN_POINT ( 'NONE',  ( 105.8203563788590600, 26.88901185006198702, -37.36032832094576150 ) ) ;
#57070=CARTESIAN_POINT ( 'NONE',  ( -30.95355748062276291, 9.511738996772320931, 30.21645440618916112 ) ) ;
#57075=CARTESIAN_POINT ( 'NONE',  ( 116.5873858943359807, 31.92924745533265352, -93.09020542203545290 ) ) ;
#57079=CARTESIAN_POINT ( 'NONE',  ( 138.7884383316737171, 44.48287833083414000, -91.54775918821466973 ) ) ;
#57081=CARTESIAN_POINT ( 'NONE',  ( 200.7511827984944830, 102.7381817183304804, 84.01209064570359430 ) ) ;
#57082=CARTESIAN_POINT ( 'NONE',  ( 212.0075063341773500, 118.7912820769029167, 34.99884505030436088 ) ) ;
#57087=CARTESIAN_POINT ( 'NONE',  ( 8.767814708128311096, 7.383611927972575373, -18.82455866429043922 ) ) ;
#57088=ORIENTED_EDGE ( 'NONE', *, *, #5859, .T. ) ;
#57089=CARTESIAN_POINT ( 'NONE',  ( 200.4559562755961224, 100.7034888016685272, -23.18393321288967002 ) ) ;
#57092=CARTESIAN_POINT ( 'NONE',  ( 188.4374648754671568, 87.87346242052443301, -72.07443739198600952 ) ) ;
#57093=CARTESIAN_POINT ( 'NONE',  ( -143.7133518487516710, 60.70463114991426323, 69.83424584982832073 ) ) ;
#57094=CARTESIAN_POINT ( 'NONE',  ( 38.91493890549796930, 8.346224043800599901, -50.61981746542777927 ) ) ;
#57096=CARTESIAN_POINT ( 'NONE',  ( 12.91653430408660697, 7.431946598423015082, -49.96024699054583351 ) ) ;
#57097=CARTESIAN_POINT ( 'NONE',  ( 130.3245512970360380, 39.33195360491890114, -36.89023367850691670 ) ) ;
#57100=ORIENTED_EDGE ( 'NONE', *, *, #61796, .T. ) ;
#57101=EDGE_CURVE ( 'NONE', #36484, #41593, #30061, .T. ) ;
#57110=CARTESIAN_POINT ( 'NONE',  ( 13.37820144534468980, 6.435512790162279728, 17.77664207586528988 ) ) ;
#57114=CARTESIAN_POINT ( 'NONE',  ( 15.78827728214693416, 7.507518794609589818, -77.36349468914950478 ) ) ;
#57117=CARTESIAN_POINT ( 'NONE',  ( 87.10668362745094839, 19.58396519288862336, -23.97701360844806118 ) ) ;
#57119=DIRECTION ( 'NONE',  ( -0.000000000000000000, 1.000000000000000000, -0.000000000000000000 ) ) ;
#57120=CARTESIAN_POINT ( 'NONE',  ( -50.13771638889894433, 13.41835215703894058, 70.34807068584244405 ) ) ;
#57122=CARTESIAN_POINT ( 'NONE',  ( -102.0721892947742049, 32.67541014876152161, -88.70367844590329298 ) ) ;
#57125=CARTESIAN_POINT ( 'NONE',  ( 155.2992895652387801, 57.24699634758577815, 56.56127440692515052 ) ) ;
#57126=FACE_OUTER_BOUND ( 'NONE', #9898, .T. ) ;
#57127=CARTESIAN_POINT ( 'NONE',  ( -47.95468448182521115, 12.89252559348046034, -40.28134454572786893 ) ) ;
#57129=DIRECTION ( 'NONE',  ( 0.000000000000000000, 0.000000000000000000, 1.000000000000000000 ) ) ;
#57133=B_SPLINE_CURVE_WITH_KNOTS ( 'NONE', 3,
 ( #69279, #27395, #38303, #6297, #38659, #39018, #55526, #23188, #33739, #49189, #6646, #33396, #23535, #55176, #34450, #54825, #29152, #18245, #34786, #1726, #12983, #40054, #39358, #65398, #13329, #50260, #11923, #65754, #60801, #1371, #43916, #56223, #6998, #45323, #22829, #17186, #55887, #12628, #44270, #7357, #28451, #61510, #22478 ),
 .UNSPECIFIED., .F., .F.,
 ( 4, 2, 2, 2, 2, 2, 2, 2, 2, 2, 2, 2, 1, 2, 2, 2, 2, 2, 2, 2, 2, 4 ),
 ( 0.02390068823634509954, 0.02538837671117071676, 0.02613222094858352537, 0.02687606518599633398, 0.02836375366082196856, 0.02985144213564760313, 0.03059528637306042909, 0.03133913061047325505, 0.03282681908529891390, 0.03431450756012457970, 0.03580219603495024550, 0.03654604027236307839, 0.03728988450977591129, 0.03803372874718874419, 0.03877757298460157015, 0.04026526145942722901, 0.04175294993425288093, 0.04324063840907853978, 0.04398448264649136574, 0.04472832688390419170, 0.04621601535872983668, 0.04770370383355547472 ),
 .UNSPECIFIED. ) ;
#57140=CARTESIAN_POINT ( 'NONE',  ( -180.0175713311536754, 95.14770835574077523, -72.01836099242309785 ) ) ;
#57147=CARTESIAN_POINT ( 'NONE',  ( -85.66184035008927822, 26.20110535976568045, 40.63455923272034909 ) ) ;
#57148=DIRECTION ( 'NONE',  ( 0.000000000000000000, 0.000000000000000000, 1.000000000000000000 ) ) ;
#57149=CARTESIAN_POINT ( 'NONE',  ( -190.4966031023458868, 108.8421921967459127, 42.59989763244942651 ) ) ;
#57151=CARTESIAN_POINT ( 'NONE',  ( 109.7782172510783170, 29.77507867835876709, -24.07788697519002241 ) ) ;
#57152=DIRECTION ( 'NONE',  ( -0.8118923937861950435, -0.5838071093367415143, 0.000000000000000000 ) ) ;
#57153=CARTESIAN_POINT ( 'NONE',  ( 39.89571693415784637, 8.473773298340391946, -35.61981746542776506 ) ) ;
#57156=FACE_OUTER_BOUND ( 'NONE', #55628, .T. ) ;
#57158=CARTESIAN_POINT ( 'NONE',  ( 133.8566784816069060, 41.42467568809810530, -77.86786152285937135 ) ) ;
#57159=EDGE_LOOP ( 'NONE', ( #55889, #55421, #4249, #43123 ) ) ;
#57160=AXIS2_PLACEMENT_3D ( 'NONE', #66094, #49884, #44614 ) ;
#57170=CARTESIAN_POINT ( 'NONE',  ( -149.5074843970971017, 64.17983161892347255, -34.81283053149196149 ) ) ;
#57172=VERTEX_POINT ( 'NONE', #32995 ) ;
#57173=CARTESIAN_POINT ( 'NONE',  ( -108.9444157621018263, 37.44493815491210853, 14.65362961424871813 ) ) ;
#57174=CARTESIAN_POINT ( 'NONE',  ( 108.3819860115547158, 28.02992728837241287, 56.67516201583306668 ) ) ;
#57175=CARTESIAN_POINT ( 'NONE',  ( 109.0263699319888957, 28.32214139819616960, 83.37130228228382123 ) ) ;
#57179=CARTESIAN_POINT ( 'NONE',  ( 160.9241720448059425, 60.38677655937337363, -63.79514627286779671 ) ) ;
#57183=ADVANCED_FACE ( 'NONE', ( #32647 ), #69239, .F. ) ;
#57184=ORIENTED_EDGE ( 'NONE', *, *, #40760, .F. ) ;
#57187=CARTESIAN_POINT ( 'NONE',  ( -82.32931163805226049, 23.75065981441938234, 58.21357082001073024 ) ) ;
#57189=CARTESIAN_POINT ( 'NONE',  ( 106.5117512545002825, 27.19336236623133374, -90.59354463606661056 ) ) ;
#57190=ADVANCED_FACE ( 'NONE', ( #50224 ), #8002, .F. ) ;
#57192=CARTESIAN_POINT ( 'NONE',  ( -31.43908319763709969, 10.61114334766717171, -62.16174795566551836 ) ) ;
#57194=CARTESIAN_POINT ( 'NONE',  ( 32.15641333221389431, 7.577415570152254531, 66.21096673341479288 ) ) ;
#57195=CARTESIAN_POINT ( 'NONE',  ( 46.79315560871277313, 9.486230672254121643, 92.53801376008529189 ) ) ;
#57198=CARTESIAN_POINT ( 'NONE',  ( 183.3913492984168272, 80.96922346472078402, 56.51364387551240043 ) ) ;
#57199=CARTESIAN_POINT ( 'NONE',  ( -123.6619986853277879, 45.04188181212060016, 18.43930124660816716 ) ) ;
#57202=CARTESIAN_POINT ( 'NONE',  ( 23.28845814680231996, 7.864847136539609096, -16.66102632038655429 ) ) ;
#57203=CARTESIAN_POINT ( 'NONE',  ( 198.8687991397275994, 98.67887821384411495, 58.82597387875455297 ) ) ;
#57206=CARTESIAN_POINT ( 'NONE',  ( 129.5225439633634608, 40.02995148249141977, -49.66244657560051223 ) ) ;
#57207=CARTESIAN_POINT ( 'NONE',  ( -126.3508039230932525, 46.79479538767113667, -34.91370389823391207 ) ) ;
#57208=ADVANCED_FACE ( 'NONE', ( #17866 ), #39667, .T. ) ;
#57210=EDGE_CURVE ( 'NONE', #12795, #30189, #20821, .T. ) ;
#57212=CARTESIAN_POINT ( 'NONE',  ( 185.1710994180821785, 84.30654632312743502, -37.42057970017137336 ) ) ;
#57213=ORIENTED_EDGE ( 'NONE', *, *, #48506, .F. ) ;
#57219=CARTESIAN_POINT ( 'NONE',  ( 164.8776669336225780, 64.96501004561835657, 89.40796121432521204 ) ) ;
#57221=CARTESIAN_POINT ( 'NONE',  ( -60.66101049381767751, 17.30588917955502026, 15.97642707013661045 ) ) ;
#57223=CARTESIAN_POINT ( 'NONE',  ( -156.1477286774994013, 71.38742644140633331, 41.71781464117591298 ) ) ;
#57226=CARTESIAN_POINT ( 'NONE',  ( -96.45845418068302024, 29.92035703021964821, 33.26432808515374973 ) ) ;
#57232=EDGE_LOOP ( 'NONE', ( #20219, #51872, #19475, #37809 ) ) ;
#57233=CARTESIAN_POINT ( 'NONE',  ( 175.5429257635131250, 74.57009623370765894, 41.88879822895370353 ) ) ;
#57234=CARTESIAN_POINT ( 'NONE',  ( 19.75784582661441391, 6.660183274347811100, -63.49536201651760337 ) ) ;
#57235=CARTESIAN_POINT ( 'NONE',  ( -126.8016613879753294, 48.30316697011515004, 72.42301449268042290 ) ) ;
#57241=CARTESIAN_POINT ( 'NONE',  ( 204.6977192012829789, 108.0580384837234789, -36.32593103262158252 ) ) ;
#57242=CARTESIAN_POINT ( 'NONE',  ( 136.7690435008550764, 44.39743995805023502, 30.09502234337038118 ) ) ;
#57244=DIRECTION ( 'NONE',  ( 0.000000000000000000, 0.000000000000000000, 1.000000000000000000 ) ) ;
#57249=ORIENTED_EDGE ( 'NONE', *, *, #33090, .T. ) ;
#57250=CARTESIAN_POINT ( 'NONE',  ( -142.0070007485041117, 59.34878529741513375, -15.73778325578669524 ) ) ;
#57254=B_SPLINE_CURVE_WITH_KNOTS ( 'NONE', 3,
 ( #51447, #46150, #41232, #41569, #57752, #2907, #13798, #29628, #29983, #19077, #19419, #9219, #35613, #25412, #30330, #40877, #61980, #51782, #4294, #51097, #35258, #67974, #9568, #68315, #3592, #31028, #25062, #19773, #35950, #57401, #62693, #14493, #52470, #20118, #30676, #52123, #68640, #46847, #56717, #8537, #63023, #14829, #34920, #36298 ),
 .UNSPECIFIED., .F., .F.,
 ( 4, 2, 2, 2, 2, 2, 2, 2, 2, 2, 2, 2, 2, 2, 2, 2, 2, 2, 2, 2, 2, 4 ),
 ( 0.02895403260893137515, 0.03071603688922228473, 0.03247804116951319431, 0.03424004544980410042, 0.03600204973009500653, 0.03776405401038591958, 0.03864505615053134835, 0.03952605829067677712, 0.04040706043082220589, 0.04128806257096763466, 0.04216906471111306343, 0.04305006685125849220, 0.04393106899140392096, 0.04481207113154934973, 0.04569307327169477850, 0.04657407541184020727, 0.04745507755198563604, 0.04833607969213106481, 0.05009808397242192235, 0.05186008825271277989, 0.05362209253300363743, 0.05714610109358538720 ),
 .UNSPECIFIED. ) ;
#57255=CARTESIAN_POINT ( 'NONE',  ( -50.14405925094052918, 13.42012186841128418, -90.73077881499243347 ) ) ;
#57258=CARTESIAN_POINT ( 'NONE',  ( 70.26936813788616121, 15.51386666370915357, -45.19091827645912929 ) ) ;
#57260=CARTESIAN_POINT ( 'NONE',  ( 209.4789161463551750, 113.1367444519304115, 57.76954579875279450 ) ) ;
#57262=ORIENTED_EDGE ( 'NONE', *, *, #51937, .T. ) ;
#57265=CARTESIAN_POINT ( 'NONE',  ( -37.79601571721867259, 10.72155118426296205, 14.85940810243080534 ) ) ;
#57268=ORIENTED_EDGE ( 'NONE', *, *, #24718, .T. ) ;
#57269=CARTESIAN_POINT ( 'NONE',  ( -83.06245155374612921, 24.04494455745185633, -90.22407819767580861 ) ) ;
#57270=B_SPLINE_CURVE_WITH_KNOTS ( 'NONE', 3,
 ( #14501, #68325, #10250, #37325, #15194, #25764, #46858, #58103, #47193, #9576, #20125, #20460, #20812, #68648, #31035, #36654, #67982, #46502, #41577, #41244, #4302, #14840, #36307, #41923, #47523, #9921, #62701, #35960, #57413, #30684, #64066, #58433, #42271, #9229, #63387, #57762, #52134, #31376, #52809, #4629, #26093, #3952, #30340, #21166, #3601, #25419 ),
 .UNSPECIFIED., .F., .F.,
 ( 4, 2, 2, 2, 2, 2, 2, 2, 2, 2, 2, 2, 2, 2, 2, 2, 2, 2, 2, 2, 2, 2, 4 ),
 ( 0.02420077021543439941, 0.02572112563160181692, 0.02648130333968554823, 0.02724148104776927953, 0.02876183646393674215, 0.02952201417202046652, 0.03028219188010418741, 0.03180254729627166044, 0.03332290271243912999, 0.03408308042052287518, 0.03484325812860662036, 0.03636361354477407604, 0.03712379125285780040, 0.03788396896094152477, 0.03864414666902524914, 0.03940432437710897351, 0.04092467979327645000, 0.04244503520944392649, 0.04396539062561140299, 0.04548574604177887948, 0.04624592374986261079, 0.04700610145794634903, 0.04852645687411386022 ),
 .UNSPECIFIED. ) ;
#57272=DIRECTION ( 'NONE',  ( 0.000000000000000000, 0.000000000000000000, 1.000000000000000000 ) ) ;
#57273=ADVANCED_FACE ( 'NONE', ( #3085 ), #67120, .F. ) ;
#57274=CARTESIAN_POINT ( 'NONE',  ( 37.46254810722764006, 8.164772623042704680, 3.307947441784442333 ) ) ;
#57275=DIRECTION ( 'NONE',  ( -0.000000000000000000, 1.000000000000000000, -0.000000000000000000 ) ) ;
#57276=AXIS2_PLACEMENT_3D ( 'NONE', #11999, #17623, #45748 ) ;
#57281=CARTESIAN_POINT ( 'NONE',  ( -58.76006735892197952, 15.70681061434692616, 31.29311785761185050 ) ) ;
#57282=CARTESIAN_POINT ( 'NONE',  ( -62.49137879463569334, 17.85440472148629709, 65.65172476684578839 ) ) ;
#57285=CARTESIAN_POINT ( 'NONE',  ( -14.32241591711279938, 7.401556312061829956, -66.00773135621913923 ) ) ;
#57286=CARTESIAN_POINT ( 'NONE',  ( -99.11448999425219597, 31.20120877265620152, -22.48539650098521392 ) ) ;
#57291=CARTESIAN_POINT ( 'NONE',  ( -154.6085044440278295, 69.98390342970667177, 59.56211392109398872 ) ) ;
#57292=CARTESIAN_POINT ( 'NONE',  ( 175.8874477961783214, 74.89984466412599318, -11.45168165142409578 ) ) ;
#57293=CARTESIAN_POINT ( 'NONE',  ( -122.8118341587045137, 44.49743491855734590, 31.26718143031790476 ) ) ;
#57296=CARTESIAN_POINT ( 'NONE',  ( -180.6158171975815776, 97.47361786002632300, -69.38088246809070370 ) ) ;
#57297=CARTESIAN_POINT ( 'NONE',  ( 126.8027934882252339, 38.47872101784862053, 88.12645126614253854 ) ) ;
#57298=EDGE_CURVE ( 'NONE', #54282, #33561, #40151, .T. ) ;
#57299=CARTESIAN_POINT ( 'NONE',  ( 115.2288739107204378, 31.25773204386718263, 31.50320768227159007 ) ) ;
#57304=CARTESIAN_POINT ( 'NONE',  ( 157.4703587214989113, 57.65129005721576760, 29.40946747225336466 ) ) ;
#57305=CARTESIAN_POINT ( 'NONE',  ( 112.5554747942045850, 29.96654954475020816, -77.40549949264581642 ) ) ;
#57306=CARTESIAN_POINT ( 'NONE',  ( 188.4374648754671568, 87.87346242052444723, 35.30376496986874457 ) ) ;
#57307=CARTESIAN_POINT ( 'NONE',  ( 181.0840389613909736, 78.60582251573003987, -89.91415884680696990 ) ) ;
#57310=ORIENTED_EDGE ( 'NONE', *, *, #4674, .T. ) ;
#57311=CARTESIAN_POINT ( 'NONE',  ( 157.9121974517528031, 59.27335488206247760, -24.27963370867398396 ) ) ;
#57314=CARTESIAN_POINT ( 'NONE',  ( 141.2947372838333990, 46.10078095604043824, 91.72802395535696007 ) ) ;
#57317=CARTESIAN_POINT ( 'NONE',  ( -142.4991775570126151, 58.45550857435406300, -66.43273307728649968 ) ) ;
#57322=CARTESIAN_POINT ( 'NONE',  ( -94.83091526606381194, 30.26550147229322718, 10.15853931445705705 ) ) ;
#57325=CARTESIAN_POINT ( 'NONE',  ( -132.2199390322348620, 50.80243550247266882, 42.17967972708286339 ) ) ;
#57327=CARTESIAN_POINT ( 'NONE',  ( 82.14396250120410059, 18.99560174459422157, -22.49292728426798860 ) ) ;
#57328=EDGE_CURVE ( 'NONE', #44581, #57471, #39276, .T. ) ;
#57329=CARTESIAN_POINT ( 'NONE',  ( -166.3188283541502699, 79.86268666707378827, 35.15081015259792707 ) ) ;
#57331=CARTESIAN_POINT ( 'NONE',  ( 91.67776154311744108, 22.27748043241296116, 42.76395149726314315 ) ) ;
#57337=VECTOR ( 'NONE', #35030, 1000.000000000000000 ) ;
#57339=CARTESIAN_POINT ( 'NONE',  ( 211.4997502125519304, 118.0043045815490359, -20.15512624053809176 ) ) ;
#57341=CARTESIAN_POINT ( 'NONE',  ( -5.879983509979052947, 7.779504553499496211, 30.35576161878026014 ) ) ;
#57348=VERTEX_POINT ( 'NONE', #4796 ) ;
#57349=CARTESIAN_POINT ( 'NONE',  ( 105.8022841538864469, 26.88074187880710753, -76.33012430075584120 ) ) ;
#57351=CARTESIAN_POINT ( 'NONE',  ( 58.48209831743722731, 11.66636741727084825, -64.07070076514432344 ) ) ;
#57358=CARTESIAN_POINT ( 'NONE',  ( -76.32962633615589709, 21.44528079176262025, 57.63206797190907338 ) ) ;
#57359=CARTESIAN_POINT ( 'NONE',  ( -166.5686015187718283, 80.11916873959170005, 68.82547394009152697 ) ) ;
#57361=ORIENTED_EDGE ( 'NONE', *, *, #61006, .T. ) ;
#57362=CARTESIAN_POINT ( 'NONE',  ( -154.6171773099879658, 68.63761944777705537, 43.71609283412200853 ) ) ;
#57363=FACE_OUTER_BOUND ( 'NONE', #45291, .T. ) ;
#57364=CARTESIAN_POINT ( 'NONE',  ( 177.2011275744679608, 74.76848439756739140, -23.30107000260681360 ) ) ;
#57367=AXIS2_PLACEMENT_3D ( 'NONE', #11145, #27669, #6572 ) ;
#57369=CARTESIAN_POINT ( 'NONE',  ( -55.05276343752910151, -170.0000000000000000, 3.472777182467474244 ) ) ;
#57371=CARTESIAN_POINT ( 'NONE',  ( 210.9506883977752523, 115.3310071214937693, 5.713674614841949939 ) ) ;
#57372=CARTESIAN_POINT ( 'NONE',  ( 9.689943677145722134, 7.388265075009366356, 59.98655866053932328 ) ) ;
#57373=VECTOR ( 'NONE', #1317, 1000.000000000000000 ) ;
#57374=CARTESIAN_POINT ( 'NONE',  ( 210.9747454890631957, 115.3673079504855821, 40.82073227286706896 ) ) ;
#57375=CYLINDRICAL_SURFACE ( 'NONE', #17180, 243.4957430088094839 ) ;
#57377=ORIENTED_EDGE ( 'NONE', *, *, #42307, .F. ) ;
#57380=CARTESIAN_POINT ( 'NONE',  ( -129.5122926757072719, 50.14302427363037395, 85.23333541525167334 ) ) ;
#57381=CARTESIAN_POINT ( 'NONE',  ( 39.40195752203891999, 9.424259417798142024, -62.46436805589144114 ) ) ;
#57383=CARTESIAN_POINT ( 'NONE',  ( 23.10939849154102887, 6.845445181420994452, 92.86463421238133265 ) ) ;
#57385=CARTESIAN_POINT ( 'NONE',  ( 79.53408731553403754, 17.12082763744058767, -67.68499423098313628 ) ) ;
#57386=ORIENTED_EDGE ( 'NONE', *, *, #65947, .F. ) ;
#57388=CARTESIAN_POINT ( 'NONE',  ( 203.9203998321607969, 106.9845510704142271, -36.35590919959582834 ) ) ;
#57390=CARTESIAN_POINT ( 'NONE',  ( -81.23297981660239486, 23.31577157498399089, 18.12494301450533385 ) ) ;
#57393=VERTEX_POINT ( 'NONE', #55406 ) ;
#57401=CARTESIAN_POINT ( 'NONE',  ( 174.1348882614951776, 73.23561817543361485, -67.73415502738041027 ) ) ;
#57402=EDGE_CURVE ( 'NONE', #23678, #24054, #29047, .T. ) ;
#57404=DIRECTION ( 'NONE',  ( 0.000000000000000000, 0.000000000000000000, 1.000000000000000000 ) ) ;
#57405=CARTESIAN_POINT ( 'NONE',  ( 84.74089592029042706, 19.84571403269344714, -50.58391462091437063 ) ) ;
#57406=CARTESIAN_POINT ( 'NONE',  ( 110.2429982417149574, -170.0000000000000000, -9.077886975189999319 ) ) ;
#57407=B_SPLINE_CURVE_WITH_KNOTS ( 'NONE', 3,
 ( #7057, #33794, #23936, #7421, #34847, #55233, #29549, #18663, #49600, #2141, #1433, #28515, #1796, #45385, #28872, #56283, #44696, #51017, #13386, #22888, #23593, #2826, #40454, #34508, #60520, #12337, #2480, #8099, #50323, #24295, #39414, #60862, #12686, #45031, #45737, #66515, #66864, #18307, #55949, #7764, #29213, #61899, #67216, #19002, #41499, #30949 ),
 .UNSPECIFIED., .F., .F.,
 ( 4, 2, 2, 2, 2, 2, 2, 2, 2, 2, 2, 2, 2, 2, 2, 2, 2, 2, 2, 2, 2, 2, 4 ),
 ( 3.103167691559091397E-17, 0.001572224531395634414, 0.003144449062791238036, 0.004716673594186841442, 0.006288898125582444848, 0.007861122656978048254, 0.009433347188373651659, 0.01021945945407147331, 0.01100557171976929496, 0.01179168398546711662, 0.01257779625116493827, 0.01415002078256057810, 0.01493613304825838935, 0.01572224531395620406, 0.01650835757965401704, 0.01729446984535183002, 0.01886669437674749761, 0.01965280664244534181, 0.02043891890814318255, 0.02201114343953889177, 0.02358336797093459752, 0.02436948023663241050, 0.02515559250233022348 ),
 .UNSPECIFIED. ) ;
#57411=EDGE_LOOP ( 'NONE', ( #24595, #47932, #19946, #27349 ) ) ;
#57413=CARTESIAN_POINT ( 'NONE',  ( -85.90077524418998678, 26.30132018890136436, -67.46541528951036071 ) ) ;
#57415=CARTESIAN_POINT ( 'NONE',  ( 173.6024011093110460, 72.73634049052009232, 9.360915578664817716 ) ) ;
#57419=CARTESIAN_POINT ( 'NONE',  ( 32.89621043149783475, 7.652303554303282240, -93.07142327913575741 ) ) ;
#57420=CARTESIAN_POINT ( 'NONE',  ( -121.2119672714299412, 44.67540322905998096, -63.37905527228651437 ) ) ;
#57422=CARTESIAN_POINT ( 'NONE',  ( 212.0779786303465642, 118.9010947973413579, 35.33010008810850167 ) ) ;
#57424=CARTESIAN_POINT ( 'NONE',  ( -78.18913509716431065, 22.13995206110505265, -61.96000122218156747 ) ) ;
#57426=VERTEX_POINT ( 'NONE', #1966 ) ;
#57428=CARTESIAN_POINT ( 'NONE',  ( -62.50344214308532997, 17.85806481441974469, 90.58836406955566645 ) ) ;
#57432=EDGE_CURVE ( 'NONE', #54495, #43039, #24205, .T. ) ;
#57434=CARTESIAN_POINT ( 'NONE',  ( 15.78827728214693416, 7.507518794609588042, 56.85925826316891829 ) ) ;
#57435=CARTESIAN_POINT ( 'NONE',  ( -171.0950923142953854, 86.38958441093224394, 31.08788057152530016 ) ) ;
#57439=CARTESIAN_POINT ( 'NONE',  ( 32.28603806442401236, 7.590310383548729334, -45.53980477190197007 ) ) ;
#57441=CARTESIAN_POINT ( 'NONE',  ( 13.36262230781615123, 7.441298897118797662, -35.90524268855146062 ) ) ;
#57442=CARTESIAN_POINT ( 'NONE',  ( 126.8015497489690375, 37.32461426945041438, -46.08151831055564429 ) ) ;
#57445=PLANE ( 'NONE',  #66435 ) ;
#57447=CARTESIAN_POINT ( 'NONE',  ( -25.80058235236790054, 8.733375263008326783, -64.69209604585124396 ) ) ;
#57448=CARTESIAN_POINT ( 'NONE',  ( 8.670103207226931730, 6.377073801252347351, 8.257049701868895752 ) ) ;
#57452=CARTESIAN_POINT ( 'NONE',  ( 173.8575673535406452, 71.59843387604340137, -72.59740664150669431 ) ) ;
#57454=CARTESIAN_POINT ( 'NONE',  ( -178.7483298110140026, 93.61800926271540391, -47.17654204188055900 ) ) ;
#57455=CARTESIAN_POINT ( 'NONE',  ( 91.11342358617748971, 21.00000175105270372, -22.49380947096609518 ) ) ;
#57456=CARTESIAN_POINT ( 'NONE',  ( -55.05276343752910151, -170.0000000000000000, -8.371773407996171201 ) ) ;
#57461=ORIENTED_EDGE ( 'NONE', *, *, #55104, .T. ) ;
#57465=CARTESIAN_POINT ( 'NONE',  ( -109.7643866341847314, 37.89854104106755273, -69.91044693626231776 ) ) ;
#57466=CARTESIAN_POINT ( 'NONE',  ( -52.68007207639879397, 14.05813534436550682, -49.83524973432806604 ) ) ;
#57471=VERTEX_POINT ( 'NONE', #2650 ) ;
#57472=DIRECTION ( 'NONE',  ( 0.000000000000000000, 0.000000000000000000, 1.000000000000000000 ) ) ;
#57478=CARTESIAN_POINT ( 'NONE',  ( 177.2011275744679040, 74.76848439756736298, -50.14562059307051101 ) ) ;
#57479=CARTESIAN_POINT ( 'NONE',  ( -180.4654253355436708, 95.69358270527507671, -70.60706783670912046 ) ) ;
#57486=CARTESIAN_POINT ( 'NONE',  ( 61.09977118998601497, 13.26754120022606287, -50.47593651538998927 ) ) ;
#57487=LINE ( 'NONE', #41313, #68552 ) ;
#57488=CARTESIAN_POINT ( 'NONE',  ( -23.93895920923072040, 9.495000752338444983, -16.21472940711745281 ) ) ;
#57495=CARTESIAN_POINT ( 'NONE',  ( -26.50207385662995918, 9.849226639603651634, 32.04887038639355268 ) ) ;
#57496=CARTESIAN_POINT ( 'NONE',  ( 199.3764470687682149, 100.9548044849099284, 41.99854440117639598 ) ) ;
#57499=EDGE_LOOP ( 'NONE', ( #59104, #63148, #38385, #34834 ) ) ;
#57500=CARTESIAN_POINT ( 'NONE',  ( 70.46579300139244140, 15.56614468937218909, 38.31143274373327046 ) ) ;
#57504=CARTESIAN_POINT ( 'NONE',  ( 112.5537757279407032, 31.07998172410696114, -63.11594588500084058 ) ) ;
#57507=CARTESIAN_POINT ( 'NONE',  ( -38.88884187334146247, 11.95889603743729346, 63.56416379048864229 ) ) ;
#57511=CARTESIAN_POINT ( 'NONE',  ( -50.52615126106341137, 14.55080735582892792, 31.81763226821556501 ) ) ;
#57517=CARTESIAN_POINT ( 'NONE',  ( -85.35172689181705152, 26.07142112926218758, -46.05152394499496182 ) ) ;
#57518=CARTESIAN_POINT ( 'NONE',  ( 115.0566045393160550, 31.17277249902146252, 85.01040373191897004 ) ) ;
#57521=ADVANCED_FACE ( 'NONE', ( #57156 ), #18825, .F. ) ;
#57523=CARTESIAN_POINT ( 'NONE',  ( 187.2354698746857764, 85.05376776489248414, -48.04494933370835241 ) ) ;
#57525=CARTESIAN_POINT ( 'NONE',  ( 157.9160637431159273, 57.99786926216935257, -62.96873488960130771 ) ) ;
#57533=CARTESIAN_POINT ( 'NONE',  ( 69.49862690228275142, 14.27023134440514873, -47.02397500419540677 ) ) ;
#57537=CARTESIAN_POINT ( 'NONE',  ( -38.93847286785604211, 11.96870349976818737, -70.16847028595665847 ) ) ;
#57539=CARTESIAN_POINT ( 'NONE',  ( 183.7875981612220073, 82.83906702837188618, 70.65221253900733700 ) ) ;
#57540=CARTESIAN_POINT ( 'NONE',  ( 10.83046137699561662, 6.392429922561257527, -10.52554053518067789 ) ) ;
#57542=CARTESIAN_POINT ( 'NONE',  ( 16.27775141556968919, 7.523247835309962106, 3.170157082241546131 ) ) ;
#57543=CARTESIAN_POINT ( 'NONE',  ( 181.5127080940606845, 79.03904173130084132, 71.15314469597512925 ) ) ;
#57544=CARTESIAN_POINT ( 'NONE',  ( -118.4063383664800000, 41.75753822095644097, 11.78578461217687590 ) ) ;
#57547=CARTESIAN_POINT ( 'NONE',  ( 20.74185656603722094, 7.717159106492277765, -21.82745635861012445 ) ) ;
#57548=CARTESIAN_POINT ( 'NONE',  ( 9.819093282782493048, 7.389085782749407194, 15.23728359609124894 ) ) ;
#57550=CARTESIAN_POINT ( 'NONE',  ( 188.4389256074243804, 86.37278721358585187, 11.46150878901021919 ) ) ;
#57552=LINE ( 'NONE', #13599, #68895 ) ;
#57554=CARTESIAN_POINT ( 'NONE',  ( -109.7790042512817905, 37.90666514836943435, -42.80576273198390425 ) ) ;
#57563=CARTESIAN_POINT ( 'NONE',  ( 116.8937673311173029, 32.08228998570056234, 60.48004562628608483 ) ) ;
#57564=B_SPLINE_CURVE_WITH_KNOTS ( 'NONE', 3,
 ( #4801, #26265, #51959, #31886, #46677, #47355, #52642, #53316, #68153, #20628, #31541, #68812, #36826, #36131, #63211, #62522, #47697, #47028, #63895, #41752, #58264, #15014, #4466, #69162, #58600, #36477, #19962, #10417, #35791, #57929, #30505, #26607, #41413, #48046, #10083, #14667, #19600, #14336, #57590, #9401, #30858, #52304, #4122, #25592, #6179, #59633, #33631 ),
 .UNSPECIFIED., .F., .F.,
 ( 4, 2, 2, 2, 2, 2, 2, 2, 2, 2, 2, 2, 1, 2, 2, 2, 2, 2, 2, 2, 2, 2, 2, 4 ),
 ( 7.152448122690996019E-18, 0.001493793014771594959, 0.002240689522157387776, 0.002987586029543181244, 0.004481379044314751266, 0.005228275551700536927, 0.005975172059086323456, 0.007468965073857915596, 0.008215861581243707329, 0.008962758088629495593, 0.01045655110340106171, 0.01120344761078684304, 0.01195034411817262089, 0.01269724062555839007, 0.01344413713294415752, 0.01493793014771570456, 0.01568482665510148935, 0.01643172316248727241, 0.01792551617725884894, 0.01941930919203042200, 0.02016620569941620159, 0.02091310220680198464, 0.02240689522157354382, 0.02390068823634510300 ),
 .UNSPECIFIED. ) ;
#57565=ORIENTED_EDGE ( 'NONE', *, *, #25885, .T. ) ;
#57566=CARTESIAN_POINT ( 'NONE',  ( 126.3580464630938991, 38.22944795020838171, -70.66847772514068993 ) ) ;
#57570=CARTESIAN_POINT ( 'NONE',  ( -94.89192151156323973, 29.18342430963128464, 36.70293385600623282 ) ) ;
#57575=EDGE_CURVE ( 'NONE', #32966, #48407, #9305, .T. ) ;
#57576=CARTESIAN_POINT ( 'NONE',  ( 110.2429982417149432, 29.99119854320847267, -24.07788697519002596 ) ) ;
#57577=B_SPLINE_CURVE_WITH_KNOTS ( 'NONE', 3,
 ( #52451, #56340, #8156, #27087, #4951, #21810, #11253, #8, #42583, #48522, #31346, #52774, #54149, #37644, #36969, #16193, #43255, #58744, #353, #59094, #5974, #32381, #10566, #64734, #26068, #63704, #15514, #10910, #53807, #32725, #5631, #32034, #63354, #53465, #4602, #59440, #58075, #717, #47496, #15164, #27433, #15848, #16543 ),
 .UNSPECIFIED., .F., .F.,
 ( 4, 2, 2, 2, 2, 2, 2, 2, 2, 2, 2, 2, 1, 2, 2, 2, 2, 2, 2, 2, 2, 4 ),
 ( 0.02371951416048008118, 0.02520633211177541674, 0.02594974108742306371, 0.02669315006307071067, 0.02817996801436600113, 0.02966678596566128812, 0.03041019494130892814, 0.03115360391695656470, 0.03264042186825183434, 0.03412723981954710745, 0.03561405777084238056, 0.03635746674649002752, 0.03710087572213767448, 0.03784428469778532145, 0.03858769367343296841, 0.04007451162472827622, 0.04156132957602358402, 0.04304814752731889183, 0.04379155650296655267, 0.04453496547861421351, 0.04602178342990952825, 0.04750860138120484299 ),
 .UNSPECIFIED. ) ;
#57582=CARTESIAN_POINT ( 'NONE',  ( -171.5023337025455703, 86.83681590836891928, 4.142432042481735799 ) ) ;
#57583=CARTESIAN_POINT ( 'NONE',  ( -180.6213815675304772, 95.88446356933845038, -15.67696249584733437 ) ) ;
#57587=CARTESIAN_POINT ( 'NONE',  ( -102.6338077722834043, 34.09093689858332255, 84.21073488133825435 ) ) ;
#57590=CARTESIAN_POINT ( 'NONE',  ( -58.96922974609609724, 15.76655591015168412, -22.27256446023782388 ) ) ;
#57591=B_SPLINE_CURVE_WITH_KNOTS ( 'NONE', 3,
 ( #65771, #11938, #48498, #43588, #16518, #33410, #28110, #33048, #332, #693, #1387, #64709, #37975, #22842, #49205, #7015, #64353, #32360, #59419, #11230, #54484, #6310, #32696, #54128, #1041, #22492, #23893, #66132, #1743, #62208, #14024, #34801, #24251, #44650, #40752, #13003, #18264, #49913, #45339, #24599, #55903, #17919, #66820 ),
 .UNSPECIFIED., .F., .F.,
 ( 4, 2, 2, 2, 2, 2, 2, 2, 2, 2, 2, 2, 1, 2, 2, 2, 2, 2, 2, 2, 2, 4 ),
 ( 0.02362927190606133043, 0.02510248541563191854, 0.02583909217041721607, 0.02657569892520251359, 0.02804891243477309823, 0.02952212594434368634, 0.03025873269912898039, 0.03099533945391427098, 0.03246855296348487296, 0.03394176647305548189, 0.03541497998262608388, 0.03615158673741138140, 0.03688819349219668586, 0.03762480024698199033, 0.03836140700176728785, 0.03983462051133786208, 0.04130783402090842937, 0.04278104753047899667, 0.04351765428526427337, 0.04425426104004954314, 0.04572747454962008268, 0.04720068805919061528 ),
 .UNSPECIFIED. ) ;
#57596=ORIENTED_EDGE ( 'NONE', *, *, #44296, .T. ) ;
#57597=EDGE_LOOP ( 'NONE', ( #32887, #65413, #46446, #54458 ) ) ;
#57598=CARTESIAN_POINT ( 'NONE',  ( 9.907111016279298354, 7.389490965936898803, -91.97754063910812761 ) ) ;
#57599=CARTESIAN_POINT ( 'NONE',  ( -167.6386155194958292, 81.22597462185134987, -37.06873647268641037 ) ) ;
#57608=DIRECTION ( 'NONE',  ( -0.000000000000000000, 1.000000000000000000, -0.000000000000000000 ) ) ;
#57609=CARTESIAN_POINT ( 'NONE',  ( -165.6393662153604396, 79.16886183052815795, -68.45080963872082691 ) ) ;
#57611=DIRECTION ( 'NONE',  ( -0.000000000000000000, 1.000000000000000000, -0.000000000000000000 ) ) ;
#57612=VERTEX_POINT ( 'NONE', #53917 ) ;
#57613=CARTESIAN_POINT ( 'NONE',  ( -35.17686701826946205, 10.23452050416468317, 17.39241332462970036 ) ) ;
#57614=CARTESIAN_POINT ( 'NONE',  ( 83.37782009939535044, 19.39546426214656449, 70.81951084743843694 ) ) ;
#57616=DIRECTION ( 'NONE',  ( 1.000000000000000000, 0.000000000000000000, -0.000000000000000000 ) ) ;
#57619=CARTESIAN_POINT ( 'NONE',  ( 32.67604581760324578, 7.629767527669949700, 13.89685609384374487 ) ) ;
#57620=CARTESIAN_POINT ( 'NONE',  ( -14.56151485655250077, 8.434196591921342190, -46.25215706853945363 ) ) ;
#57621=VECTOR ( 'NONE', #40177, 1000.000000000000000 ) ;
#57623=B_SPLINE_CURVE_WITH_KNOTS ( 'NONE', 3,
 ( #20132, #9583, #3272, #35630, #63042, #40896, #14848, #19092, #68657, #61997, #62708, #46512, #63396, #35278, #36314, #3608, #31043, #24732, #46167, #25076, #8200, #14168, #57770, #56735, #30691, #57422, #57082, #19789, #52487, #25771, #8895, #8551, #47200, #67306, #67990, #30003, #15201, #67640, #56379, #29651, #19435, #14509, #35968, #51113 ),
 .UNSPECIFIED., .F., .F.,
 ( 4, 2, 2, 2, 2, 2, 2, 2, 2, 2, 2, 2, 2, 2, 2, 2, 2, 2, 2, 2, 2, 4 ),
 ( 1.551583845779545699E-17, 0.004120577325733583603, 0.006180865988600344613, 0.008241154651467106490, 0.01030144331433386490, 0.01133158764576721635, 0.01236173197720056779, 0.01339187630863392271, 0.01442202064006727416, 0.01545216497150062561, 0.01648230930293397359, 0.01699738146865065885, 0.01751245363436734759, 0.01854259796580074587, 0.01957274229723415110, 0.02060288662866755285, 0.02266317529153432167, 0.02472346395440109049, 0.02678375261726785930, 0.02781389694870120208, 0.02884404128013454832, 0.03296461860586802350 ),
 .UNSPECIFIED. ) ;
#57625=CARTESIAN_POINT ( 'NONE',  ( -119.6718585611729679, 43.71387783726355281, -91.88895242600902691 ) ) ;
#57629=CARTESIAN_POINT ( 'NONE',  ( -25.48237668717800375, 8.689083390666771933, 15.45542771530772441 ) ) ;
#57631=CARTESIAN_POINT ( 'NONE',  ( -11.78792974237933500, 7.181513757308657375, -76.13506112128496284 ) ) ;
#57634=CARTESIAN_POINT ( 'NONE',  ( 149.9714610887121466, 53.28792066194168342, -43.93159308990031064 ) ) ;
#57644=DIRECTION ( 'NONE',  ( 0.000000000000000000, -1.000000000000000000, 0.000000000000000000 ) ) ;
#57645=CARTESIAN_POINT ( 'NONE',  ( -1.876547441458561893, 6.576559737910139702, -20.64758074539619770 ) ) ;
#57646=CARTESIAN_POINT ( 'NONE',  ( 117.4696399285658543, 32.37118663718646872, 35.03847803874900535 ) ) ;
#57647=CARTESIAN_POINT ( 'NONE',  ( -173.1211646369891355, -170.0000000000000000, 18.97714401617737323 ) ) ;
#57649=CARTESIAN_POINT ( 'NONE',  ( -124.1033713525885389, 45.32626312604504193, -61.97149759412182135 ) ) ;
#57651=CARTESIAN_POINT ( 'NONE',  ( 197.6145711261845008, 97.10888456119690204, 34.16122082187249731 ) ) ;
#57653=CARTESIAN_POINT ( 'NONE',  ( 188.2091813586561386, 87.61952156613882892, 39.16720350456787969 ) ) ;
#57658=CARTESIAN_POINT ( 'NONE',  ( 175.0696098417091662, 74.11936424544843760, 59.16513549669191008 ) ) ;
#57660=CARTESIAN_POINT ( 'NONE',  ( -104.1244073710070239, 33.72720758483609416, -35.23009648099888125 ) ) ;
#57661=CARTESIAN_POINT ( 'NONE',  ( 141.0352762984948356, 45.93128157562509983, 88.49822799473426471 ) ) ;
#57662=ADVANCED_FACE ( 'NONE', ( #59203 ), #43374, .F. ) ;
#57666=CARTESIAN_POINT ( 'NONE',  ( 157.0357419681844533, 58.58786672900119186, 2.574317928867096317 ) ) ;
#57667=ORIENTED_EDGE ( 'NONE', *, *, #34158, .T. ) ;
#57668=CARTESIAN_POINT ( 'NONE',  ( -180.6011569556094969, 95.85968111394265634, 37.69164199392516679 ) ) ;
#57670=CARTESIAN_POINT ( 'NONE',  ( 110.2429982417149432, 29.99119854320846201, -35.92243756565368784 ) ) ;
#57679=AXIS2_PLACEMENT_3D ( 'NONE', #27591, #22321, #37112 ) ;
#57680=CARTESIAN_POINT ( 'NONE',  ( 150.0433793199863430, 52.09973307442956525, 62.67375200242342004 ) ) ;
#57683=CARTESIAN_POINT ( 'NONE',  ( 39.89582146299188281, 9.488756994579087944, 18.06928371549960488 ) ) ;
#57685=CARTESIAN_POINT ( 'NONE',  ( 156.5890478960376981, 58.24007662587948886, -9.318429201860791267 ) ) ;
#57686=CARTESIAN_POINT ( 'NONE',  ( 211.7318474105134385, 118.3631723164074714, -19.60079423289586487 ) ) ;
#57688=CARTESIAN_POINT ( 'NONE',  ( -153.1121305730336815, 67.29834700374524914, -62.57647805126995166 ) ) ;
#57692=CARTESIAN_POINT ( 'NONE',  ( 211.7419975634644800, 116.5322580952101674, -46.48037847538860490 ) ) ;
#57693=CARTESIAN_POINT ( 'NONE',  ( 110.2429982417149574, -170.0000000000000000, 10.26666361527366078 ) ) ;
#57694=ORIENTED_EDGE ( 'NONE', *, *, #57101, .T. ) ;
#57697=CARTESIAN_POINT ( 'NONE',  ( -71.57660578921959882, 20.81129687646280502, 67.25978822818018443 ) ) ;
#57698=CARTESIAN_POINT ( 'NONE',  ( 57.39083379741712321, 11.43779987330584547, -75.05095958129902556 ) ) ;
#57701=CARTESIAN_POINT ( 'NONE',  ( -4.384507269342570623, 6.691209796733446069, 84.63264704995823706 ) ) ;
#57702=CARTESIAN_POINT ( 'NONE',  ( -109.0291978193666722, 37.49173305805086898, -18.95094030686922082 ) ) ;
#57703=EDGE_LOOP ( 'NONE', ( #15613, #68081, #12297, #44352 ) ) ;
#57704=CARTESIAN_POINT ( 'NONE',  ( -76.77329340382466683, 21.60914066444074066, 72.03569539077717820 ) ) ;
#57706=EDGE_LOOP ( 'NONE', ( #16077, #59270 ) ) ;
#57708=CARTESIAN_POINT ( 'NONE',  ( -153.6931187576189188, 67.81270084382354923, 31.99307535251548629 ) ) ;
#57710=CARTESIAN_POINT ( 'NONE',  ( 179.4279766878530609, 76.94722012158237590, -24.20745791858651330 ) ) ;
#57713=CARTESIAN_POINT ( 'NONE',  ( -142.0251973982165339, 58.08401473564118334, 10.78919118282799339 ) ) ;
#57718=CARTESIAN_POINT ( 'NONE',  ( 211.1200456646896839, 115.5868795682033010, 13.74673903110627293 ) ) ;
#57719=CARTESIAN_POINT ( 'NONE',  ( 110.2429982417149574, -170.0000000000000000, 44.61121420573733332 ) ) ;
#57720=AXIS2_PLACEMENT_3D ( 'NONE', #33834, #55276, #28913 ) ;
#57721=CARTESIAN_POINT ( 'NONE',  ( 209.4789161463551750, 113.1367444519304257, 30.92499520828909709 ) ) ;
#57722=CARTESIAN_POINT ( 'NONE',  ( 9.681512146547785136, 6.381925336433647900, -92.33363154823911145 ) ) ;
#57727=ORIENTED_EDGE ( 'NONE', *, *, #24510, .F. ) ;
#57728=CARTESIAN_POINT ( 'NONE',  ( -149.5074843970971017, 65.50121172469319220, 57.56537183036274286 ) ) ;
#57729=CARTESIAN_POINT ( 'NONE',  ( -121.5894932252149800, 44.91329912928144097, 85.63689221737818968 ) ) ;
#57731=CARTESIAN_POINT ( 'NONE',  ( -166.7068579965637412, 80.26142964949316649, -19.26318465954255643 ) ) ;
#57732=DIRECTION ( 'NONE',  ( -0.000000000000000000, 1.000000000000000000, -0.000000000000000000 ) ) ;
#57733=CARTESIAN_POINT ( 'NONE',  ( 22.95565677133307148, 6.835936356918209889, 88.97060043287888220 ) ) ;
#57734=CARTESIAN_POINT ( 'NONE',  ( 23.28997038562041055, 7.864942668124619729, 90.91843093332407477 ) ) ;
#57737=CARTESIAN_POINT ( 'NONE',  ( -95.21430597939261986, 29.33390900154316938, 62.29818221739061102 ) ) ;
#57740=CARTESIAN_POINT ( 'NONE',  ( -85.90441187606239737, 25.21188850826090899, 13.10346238197241853 ) ) ;
#57744=ORIENTED_EDGE ( 'NONE', *, *, #66674, .T. ) ;
#57747=CARTESIAN_POINT ( 'NONE',  ( 8.288104306525690745, 6.376394648992967262, -43.50552248815810685 ) ) ;
#57749=CARTESIAN_POINT ( 'NONE',  ( 128.0848616812662613, 38.04676222636086891, 68.67022180960751143 ) ) ;
#57750=ORIENTED_EDGE ( 'NONE', *, *, #20805, .T. ) ;
#57752=CARTESIAN_POINT ( 'NONE',  ( 179.0091171455098049, 77.94933395983136393, -77.78972269939623629 ) ) ;
#57753=AXIS2_PLACEMENT_3D ( 'NONE', #31122, #53827, #63121 ) ;
#57756=CARTESIAN_POINT ( 'NONE',  ( 79.39764314491567632, 18.13166883367084736, -45.32563429318312842 ) ) ;
#57762=CARTESIAN_POINT ( 'NONE',  ( -83.53167274806556009, 25.32068190668985253, -63.73130560477633111 ) ) ;
#57763=CARTESIAN_POINT ( 'NONE',  ( 175.5429257635130966, 74.57009623370765894, 15.04424763849001501 ) ) ;
#57765=CARTESIAN_POINT ( 'NONE',  ( -188.6739852773920347, 108.2139733222100375, -13.56090942305224267 ) ) ;
#57766=CARTESIAN_POINT ( 'NONE',  ( 127.4750938923429828, 37.70245908594343831, 6.217222705552873485 ) ) ;
#57769=CARTESIAN_POINT ( 'NONE',  ( 197.2438487909066396, 98.25413800600045988, 89.45392550497817297 ) ) ;
#57770=CARTESIAN_POINT ( 'NONE',  ( 212.1913428512247037, 119.0779339498137546, 36.35316656546646641 ) ) ;
#57771=CARTESIAN_POINT ( 'NONE',  ( 162.0835148203877054, 61.32844276806159201, 4.132286737511699393 ) ) ;
#57772=CARTESIAN_POINT ( 'NONE',  ( -109.3432140528234697, 36.51591785955880454, 40.59350856912254102 ) ) ;
#57774=AXIS2_PLACEMENT_3D ( 'NONE', #37918, #53044, #32303 ) ;
#57775=CARTESIAN_POINT ( 'NONE',  ( -62.32077575123996382, 17.80262092668387197, 89.62707857507018616 ) ) ;
#57779=CARTESIAN_POINT ( 'NONE',  ( 18.88468164817598449, 7.626722602998420975, -76.69889805417930972 ) ) ;
#57780=PLANE ( 'NONE',  #16624 ) ;
#57782=CARTESIAN_POINT ( 'NONE',  ( 141.2361973397653401, 47.26569015399787332, -42.15863887015712663 ) ) ;
#57783=CARTESIAN_POINT ( 'NONE',  ( 32.56927464314649967, 7.618924692399907883, -46.22225308106595776 ) ) ;
#57786=DIRECTION ( 'NONE',  ( 0.000000000000000000, 0.000000000000000000, 1.000000000000000000 ) ) ;
#57791=CARTESIAN_POINT ( 'NONE',  ( -24.32937228292060539, 8.531905774118438757, -72.09986348764125808 ) ) ;
#57793=CARTESIAN_POINT ( 'NONE',  ( 13.84120792123768773, 6.445822122644893959, 3.410756033091004724 ) ) ;
#57794=ADVANCED_FACE ( 'NONE', ( #64495 ), #15277, .F. ) ;
#57795=CARTESIAN_POINT ( 'NONE',  ( 45.89232972084000295, 10.36128169546909739, -73.73081192014224428 ) ) ;
#57798=CARTESIAN_POINT ( 'NONE',  ( -178.0658882571760842, 92.80593104957425510, -47.85589308113880946 ) ) ;
#57799=CARTESIAN_POINT ( 'NONE',  ( 87.58098510096633049, 19.74745174099417255, -23.93185505127985380 ) ) ;
#57800=CARTESIAN_POINT ( 'NONE',  ( -29.50439180771547854, 10.29976981300625205, 57.29848261981403112 ) ) ;
#57802=B_SPLINE_CURVE_WITH_KNOTS ( 'NONE', 3,
 ( #4345, #34970, #30729, #8589, #47232, #46196, #68690, #36348, #63428, #51829, #41282, #68365, #14545, #3996, #8931, #19471, #52176, #8236, #63077, #67676, #13850, #3639, #45865, #62034, #56413, #67337, #24763, #46901, #56770, #30038, #51500, #25114, #3302, #46546, #19829, #9268, #20166, #62741, #36005, #14881, #57800, #9620, #37036, #42653 ),
 .UNSPECIFIED., .F., .F.,
 ( 4, 2, 2, 2, 2, 2, 2, 2, 2, 2, 2, 2, 2, 2, 2, 2, 2, 2, 2, 2, 2, 4 ),
 ( 0.000000000000000000, 0.001473754749730416067, 0.002210632124595628221, 0.002947509499460839941, 0.004421264249191274656, 0.005895018998921709372, 0.007368773748652143220, 0.008105651123517363180, 0.008842528498382584007, 0.01031628324811306209, 0.01179003799784354191, 0.01252691537270880263, 0.01326379274757406336, 0.01473754749730458134, 0.01547442487216983166, 0.01621130224703508371, 0.01768505699676558435, 0.01915881174649608845, 0.01989568912136133877, 0.02063256649622658562, 0.02210632124595708972, 0.02358007599568759036 ),
 .UNSPECIFIED. ) ;
#57803=CARTESIAN_POINT ( 'NONE',  ( -49.62489392740899063, 13.29305723289026986, 59.48038597728405819 ) ) ;
#57805=VECTOR ( 'NONE', #32159, 1000.000000000000000 ) ;
#57807=ORIENTED_EDGE ( 'NONE', *, *, #12873, .T. ) ;
#57808=CARTESIAN_POINT ( 'NONE',  ( 132.9557829392755082, 42.05591979570414907, 2.706097766650628955 ) ) ;
#57811=CARTESIAN_POINT ( 'NONE',  ( 153.2208437558772118, 55.67531116261157109, 69.95159403288403155 ) ) ;
#57812=CARTESIAN_POINT ( 'NONE',  ( -109.7686203588200868, 37.90089348911612888, -68.86741973818818963 ) ) ;
#57814=CARTESIAN_POINT ( 'NONE',  ( -0.3423060809770838708, 7.525952860323299021, 91.90469597356303666 ) ) ;
#57816=ORIENTED_EDGE ( 'NONE', *, *, #51620, .F. ) ;
#57820=CARTESIAN_POINT ( 'NONE',  ( -55.05276343752910151, 14.68156374112636797, 72.16187836339486239 ) ) ;
#57824=CARTESIAN_POINT ( 'NONE',  ( 33.84530598357039111, 8.763572915769019644, 86.05493817697373515 ) ) ;
#57831=CARTESIAN_POINT ( 'NONE',  ( -0.3740447803642799607, 7.527031846085010081, 9.787104204890834325 ) ) ;
#57832=CARTESIAN_POINT ( 'NONE',  ( -85.75002235020438945, 26.23806300442547723, 40.39546564861201006 ) ) ;
#57836=CARTESIAN_POINT ( 'NONE',  ( 104.4006536356073980, 27.36759527624477073, -21.30726361956479664 ) ) ;
#57837=CARTESIAN_POINT ( 'NONE',  ( 9.416603677636260272, 6.380307115728824918, 60.39548338895173174 ) ) ;
#57839=CARTESIAN_POINT ( 'NONE',  ( 198.8732368717152212, 100.3103976497390732, 41.43945101493392258 ) ) ;
#57840=CARTESIAN_POINT ( 'NONE',  ( -71.97767679134960872, 20.95111989827391596, 94.99999999999866418 ) ) ;
#57843=CARTESIAN_POINT ( 'NONE',  ( 70.45451534980409747, 15.56315969138429089, 36.32525407553249153 ) ) ;
#57846=CARTESIAN_POINT ( 'NONE',  ( 116.9197133427646804, 33.22079464767578827, -73.72094471291028128 ) ) ;
#57848=CARTESIAN_POINT ( 'NONE',  ( 200.8298320869470217, 101.1869877914233342, -77.11050760436773999 ) ) ;
#57850=CARTESIAN_POINT ( 'NONE',  ( 70.26840926437850499, 14.47268499222803584, -95.00000000000133582 ) ) ;
#57851=CARTESIAN_POINT ( 'NONE',  ( -83.51110947562233378, 25.31252704029285638, -21.50135568052127866 ) ) ;
#57857=CARTESIAN_POINT ( 'NONE',  ( 64.69738688745241006, 14.10375742873388560, -9.063140076922552524 ) ) ;
#57859=CARTESIAN_POINT ( 'NONE',  ( -84.23336401058610079, 25.60798568215573923, -37.56591546589165631 ) ) ;
#57860=CARTESIAN_POINT ( 'NONE',  ( 115.9898432474883805, 31.63259700092694615, 85.96951199300247026 ) ) ;
#57863=B_SPLINE_CURVE_WITH_KNOTS ( 'NONE', 3,
 ( #36854, #9777, #10797, #48075, #58295, #11141, #68842, #42799, #52669, #22047, #16426, #32267, #53699, #25955, #5520, #26974, #63583, #48404, #43493, #237, #21020, #21694, #43145, #63924, #15396, #10113, #31570, #59327, #32605, #54032, #4830, #5858, #64970, #16762, #38223, #23460 ),
 .UNSPECIFIED., .F., .F.,
 ( 4, 2, 2, 2, 2, 2, 2, 2, 2, 2, 2, 2, 2, 2, 2, 2, 2, 4 ),
 ( 1.551583845779545699E-17, 0.001548367318450189758, 0.003096734636900363904, 0.004645101955350544772, 0.006193469273800726073, 0.007741836592250900435, 0.008516020251475976341, 0.009290203910701053114, 0.01083857122915120319, 0.01238693854760135500, 0.01393530586605150681, 0.01548367318450165862, 0.01703204050295181043, 0.01858040782140196051, 0.02012877513985211753, 0.02167714245830227107, 0.02322550977675242809, 0.02477387709520258163 ),
 .UNSPECIFIED. ) ;
#57865=CARTESIAN_POINT ( 'NONE',  ( 188.4389256074244088, 86.37278721358585187, -42.22759239191712055 ) ) ;
#57867=CARTESIAN_POINT ( 'NONE',  ( 162.8142581494936110, 61.92799983924231810, -65.18475365324361803 ) ) ;
#57869=ORIENTED_EDGE ( 'NONE', *, *, #24455, .T. ) ;
#57874=CARTESIAN_POINT ( 'NONE',  ( -83.52505811737951547, 24.23179517241435832, 59.02801608792132981 ) ) ;
#57879=CARTESIAN_POINT ( 'NONE',  ( 9.416603677636260272, 6.380307115728824030, -20.13816838243932494 ) ) ;
#57881=CARTESIAN_POINT ( 'NONE',  ( 187.8959968237853673, 85.77553094678178525, 60.50337096870740083 ) ) ;
#57882=CARTESIAN_POINT ( 'NONE',  ( -123.6699087229882394, 45.04696784753412686, 4.109065455722274329 ) ) ;
#57884=CARTESIAN_POINT ( 'NONE',  ( 126.4324872316702795, 37.11876756822024248, -15.58278715265817382 ) ) ;
#57886=CARTESIAN_POINT ( 'NONE',  ( 12.03162622199373644, 7.415834979634797541, 17.16615268946964079 ) ) ;
#57889=CARTESIAN_POINT ( 'NONE',  ( 188.2950202724321116, 86.21411212788227374, 7.881204597112279053 ) ) ;
#57892=CARTESIAN_POINT ( 'NONE',  ( 173.7227242028391743, 71.47307702680407715, 35.34404529599159872 ) ) ;
#57894=CARTESIAN_POINT ( 'NONE',  ( 41.09671232177015554, 8.635892912882347616, -77.27450094475904052 ) ) ;
#57895=CARTESIAN_POINT ( 'NONE',  ( 186.2680729609084835, 85.48839327635668894, -49.16545261310956505 ) ) ;
#57898=CARTESIAN_POINT ( 'NONE',  ( -23.98903001682803549, 8.486614814224619607, -16.96685653807542593 ) ) ;
#57899=CARTESIAN_POINT ( 'NONE',  ( 199.2049631873262854, 100.7347227143600321, 14.97624135697880021 ) ) ;
#57901=AXIS2_PLACEMENT_3D ( 'NONE', #34249, #35280, #8897 ) ;
#57902=CARTESIAN_POINT ( 'NONE',  ( 113.4351684956570807, 30.38657459074489964, 57.15270542610819859 ) ) ;
#57903=ADVANCED_FACE ( 'NONE', ( #44065 ), #43713, .F. ) ;
#57906=CARTESIAN_POINT ( 'NONE',  ( 126.4754729582248132, 37.14269484129876986, 38.36551284386316496 ) ) ;
#57908=EDGE_CURVE ( 'NONE', #28889, #62698, #17707, .T. ) ;
#57912=CYLINDRICAL_SURFACE ( 'NONE', #33873, 7.500000000000020428 ) ;
#57920=CARTESIAN_POINT ( 'NONE',  ( -121.2008155373973892, 43.48033530165984217, -21.43964104200714615 ) ) ;
#57923=CARTESIAN_POINT ( 'NONE',  ( -144.9412191745148846, 61.69548892475975066, -36.34343113144615955 ) ) ;
#57926=CARTESIAN_POINT ( 'NONE',  ( 63.01563776193091826, 13.70579113808095073, 2.968410348757589468 ) ) ;
#57928=ORIENTED_EDGE ( 'NONE', *, *, #5920, .T. ) ;
#57929=CARTESIAN_POINT ( 'NONE',  ( -62.15799747763098537, 16.70234469631018115, -18.32392564386741896 ) ) ;
#57930=CARTESIAN_POINT ( 'NONE',  ( -128.1267916618074594, 49.19573276651588145, -62.08358998231160797 ) ) ;
#57931=CARTESIAN_POINT ( 'NONE',  ( 61.40360494384000845, 12.30429482808983721, -89.57394958506790772 ) ) ;
#57933=CARTESIAN_POINT ( 'NONE',  ( -95.04120270830171080, 29.25306318840327791, -67.33052735652132981 ) ) ;
#57935=VERTEX_POINT ( 'NONE', #1170 ) ;
#57936=CARTESIAN_POINT ( 'NONE',  ( 188.0141161196705752, 85.90515114331887503, -67.68764559524167623 ) ) ;
#57940=CARTESIAN_POINT ( 'NONE',  ( -75.43495400358861502, 22.18831810339349886, 31.14574269627557612 ) ) ;
#57942=CARTESIAN_POINT ( 'NONE',  ( 81.74909803672915132, 17.81295302817862947, 31.49550494790652522 ) ) ;
#57945=CARTESIAN_POINT ( 'NONE',  ( -165.9122696334865168, 79.44688201528255433, -71.14683853636709898 ) ) ;
#57946=ORIENTED_EDGE ( 'NONE', *, *, #11506, .F. ) ;
#57947=CARTESIAN_POINT ( 'NONE',  ( -109.7078892845591582, 36.71702188566215597, -14.59872168737284781 ) ) ;
#57950=CARTESIAN_POINT ( 'NONE',  ( -180.5668408223793904, 95.81768001203278118, -95.00000000000133582 ) ) ;
#57956=CARTESIAN_POINT ( 'NONE',  ( 31.90217595456442012, 7.552213897210513949, 11.06335214983522874 ) ) ;
#57957=LINE ( 'NONE', #47731, #45754 ) ;
#57958=CARTESIAN_POINT ( 'NONE',  ( -38.45778834351241926, 11.87434869453507247, -13.31764495626525857 ) ) ;
#57962=FACE_OUTER_BOUND ( 'NONE', #41432, .T. ) ;
#57966=CARTESIAN_POINT ( 'NONE',  ( -27.70562707895079768, 9.007984652865420827, 4.348468677708457797 ) ) ;
#57970=CARTESIAN_POINT ( 'NONE',  ( -55.05276343752910151, 14.68156374112637330, -88.90542517938719413 ) ) ;
#57971=CARTESIAN_POINT ( 'NONE',  ( -96.43148989374459745, 29.90755650959363621, -10.94842023032891376 ) ) ;
#57973=CARTESIAN_POINT ( 'NONE',  ( 154.0515132159917755, 56.29926936869309628, -50.31581255231360927 ) ) ;
#57980=CARTESIAN_POINT ( 'NONE',  ( 173.7225111622554437, 72.84868911716897344, -15.41689420582882697 ) ) ;
#57982=CARTESIAN_POINT ( 'NONE',  ( -128.1282195935087600, 49.19720162550164844, -49.57677375076018222 ) ) ;
#57984=CARTESIAN_POINT ( 'NONE',  ( -178.2328124332056518, 94.56955476227570045, -74.56460458710455441 ) ) ;
#57985=CARTESIAN_POINT ( 'NONE',  ( -0.8055628312658243972, 6.535476276302841114, -18.72534061433564290 ) ) ;
#57986=CARTESIAN_POINT ( 'NONE',  ( 204.3750762779230001, 107.6105286537017207, -90.01503221354896311 ) ) ;
#57987=LINE ( 'NONE', #40767, #40538 ) ;
#57988=CARTESIAN_POINT ( 'NONE',  ( 135.6651581599210203, 42.52720121194704461, 29.72801099383555723 ) ) ;
#57989=ADVANCED_FACE ( 'NONE', ( #18740 ), #8541, .F. ) ;
#57990=ORIENTED_EDGE ( 'NONE', *, *, #55401, .T. ) ;
#57991=CARTESIAN_POINT ( 'NONE',  ( -149.5074843970971017, 64.17983161892347255, 45.72082123989907387 ) ) ;
#57993=CARTESIAN_POINT ( 'NONE',  ( 186.7642514597453385, 86.02880938169742819, 41.71253118051657083 ) ) ;
#57994=CARTESIAN_POINT ( 'NONE',  ( 162.0812592823605485, 62.62783216273698628, 15.99956616506345952 ) ) ;
#57999=CARTESIAN_POINT ( 'NONE',  ( 181.0840389613909736, 80.03940679743415387, 17.46404351504774866 ) ) ;
#58001=VECTOR ( 'NONE', #12697, 1000.000000000000000 ) ;
#58003=CARTESIAN_POINT ( 'NONE',  ( 70.45466089417030275, 14.52203022703030832, -69.07882228772790256 ) ) ;
#58004=CARTESIAN_POINT ( 'NONE',  ( -62.30463872474475551, 16.74658165105247676, 35.83966074286138337 ) ) ;
#58006=VERTEX_POINT ( 'NONE', #56366 ) ;
#58007=CARTESIAN_POINT ( 'NONE',  ( -174.7869898116916545, 88.99756909636809610, 45.68310981282044025 ) ) ;
#58009=CARTESIAN_POINT ( 'NONE',  ( 110.7117404013331452, 30.20916032354563185, -50.92243756565370916 ) ) ;
#58010=VECTOR ( 'NONE', #38068, 1000.000000000000000 ) ;
#58017=DIRECTION ( 'NONE',  ( 0.000000000000000000, 0.000000000000000000, 1.000000000000000000 ) ) ;
#58018=CARTESIAN_POINT ( 'NONE',  ( 153.4268936273268480, 54.57409659828383752, 57.43301500385714320 ) ) ;
#58021=CARTESIAN_POINT ( 'NONE',  ( -9.779603649692301559, 8.034615131607075966, 71.71790837464678248 ) ) ;
#58023=CARTESIAN_POINT ( 'NONE',  ( 155.7265855639938650, 57.57443315515121895, -24.08749366127067049 ) ) ;
#58024=CARTESIAN_POINT ( 'NONE',  ( 210.0055645826033981, 115.7254585628714523, -22.30316490195718160 ) ) ;
#58025=DIRECTION ( 'NONE',  ( -0.8118923937861950435, -0.5838071093367415143, 0.000000000000000000 ) ) ;
#58026=CARTESIAN_POINT ( 'NONE',  ( -154.0718453320783112, 68.14976693162391541, -75.11313154428037819 ) ) ;
#58027=CARTESIAN_POINT ( 'NONE',  ( 56.03258084883530188, 11.16066123285296641, 93.81981338172488449 ) ) ;
#58028=CARTESIAN_POINT ( 'NONE',  ( 181.0840389613909736, 80.03940679743415387, 17.46404351504774866 ) ) ;
#58029=CARTESIAN_POINT ( 'NONE',  ( 209.5118425285948547, 113.1852661712287329, -38.07046045544934998 ) ) ;
#58030=CARTESIAN_POINT ( 'NONE',  ( -78.66644367742111399, -170.0000000000000000, 37.91820113967311556 ) ) ;
#58033=DIRECTION ( 'NONE',  ( -0.000000000000000000, 1.000000000000000000, -0.000000000000000000 ) ) ;
#58035=CARTESIAN_POINT ( 'NONE',  ( -72.21889834709581635, 21.03534256744171671, 68.62594976653699064 ) ) ;
#58036=CARTESIAN_POINT ( 'NONE',  ( 204.6977192012829789, 106.3443248447423599, -78.17048162308530834 ) ) ;
#58037=CARTESIAN_POINT ( 'NONE',  ( 56.53776994993147298, 11.26292242501182450, -66.27727168919989253 ) ) ;
#58039=CARTESIAN_POINT ( 'NONE',  ( -31.43908319763709969, 9.591432048623756756, -89.00629854612920155 ) ) ;
#58040=CARTESIAN_POINT ( 'NONE',  ( -149.5074843970971301, -170.0000000000000000, 72.56537183036277838 ) ) ;
#58041=CARTESIAN_POINT ( 'NONE',  ( -102.2801239173131052, 33.91021738430207222, -8.170026674512225640 ) ) ;
#58043=CARTESIAN_POINT ( 'NONE',  ( -71.21970990337014484, 19.62334883444994560, 63.73658943180317493 ) ) ;
#58046=ORIENTED_EDGE ( 'NONE', *, *, #15115, .T. ) ;
#58047=ADVANCED_FACE ( 'NONE', ( #67297 ), #30680, .F. ) ;
#58048=EDGE_CURVE ( 'NONE', #18940, #11337, #63596, .T. ) ;
#58049=CARTESIAN_POINT ( 'NONE',  ( -157.0069704378501569, 70.81086990254192415, 38.80300155337447165 ) ) ;
#58050=CARTESIAN_POINT ( 'NONE',  ( 59.72897338775216269, 11.93428797217974768, -49.96663325469457817 ) ) ;
#58052=EDGE_CURVE ( 'NONE', #60277, #44118, #52128, .T. ) ;
#58055=B_SPLINE_CURVE_WITH_KNOTS ( 'NONE', 3,
 ( #50074, #49356, #44804, #7529, #65932, #17727, #28979, #64863, #17003, #39185, #23694, #1189, #65566, #38472, #59913, #11734, #60627, #16666, #38119, #54644, #12443, #33903, #7166, #17357, #38834, #40554, #3282, #56389, #13149, #8208, #24740, #61667, #9245, #67648, #50764, #3969, #67315, #2585, #56048, #19100, #19444, #39866, #34613, #30012, #41261, #35977 ),
 .UNSPECIFIED., .F., .F.,
 ( 4, 2, 2, 2, 2, 2, 2, 2, 2, 2, 2, 2, 2, 2, 2, 2, 2, 2, 2, 2, 2, 2, 4 ),
 ( 0.000000000000000000, 0.003373244802897278679, 0.004216556003621594988, 0.005059867204345911730, 0.006746489605794545215, 0.007589800806518857620, 0.008433112007243172628, 0.009276423207967485901, 0.01011973440869179917, 0.01180635681014042572, 0.01349297921158905053, 0.01433629041231336033, 0.01517960161303767187, 0.01686622401448626893, 0.01770953521521054924, 0.01855284641593482955, 0.02023946881738342488, 0.02108278001810769825, 0.02192609121883197509, 0.02361271362028052878, 0.02445602482100480216, 0.02529933602172907553, 0.02698595842317762922 ),
 .UNSPECIFIED. ) ;
#58056=CARTESIAN_POINT ( 'NONE',  ( -144.2188519266539970, 59.82027639618912929, 6.052588554004912247 ) ) ;
#58063=CARTESIAN_POINT ( 'NONE',  ( 210.0292194063021896, 113.9511645670926470, 15.14336717752075323 ) ) ;
#58064=CARTESIAN_POINT ( 'NONE',  ( -142.0860844253782886, 59.41107357617636353, 37.10142862026528121 ) ) ;
#58066=CARTESIAN_POINT ( 'NONE',  ( -6.125624616441583292, 7.794071945221088704, 71.76905348450266331 ) ) ;
#58068=VECTOR ( 'NONE', #62245, 1000.000000000000000 ) ;
#58072=CARTESIAN_POINT ( 'NONE',  ( -123.7116175647536096, 46.27018554618426549, 84.61033409315344045 ) ) ;
#58073=CARTESIAN_POINT ( 'NONE',  ( 32.66364305947234214, 8.639871491745250154, -66.63435592309144795 ) ) ;
#58074=CARTESIAN_POINT ( 'NONE',  ( 141.0645618855930365, 45.95036951196540542, -72.50746714427457107 ) ) ;
#58075=CARTESIAN_POINT ( 'NONE',  ( 66.30567821786755189, 13.45988234822860896, 44.05720671718261627 ) ) ;
#58076=EDGE_CURVE ( 'NONE', #26121, #40620, #25820, .T. ) ;
#58077=CARTESIAN_POINT ( 'NONE',  ( 8.401684033729910794, 7.382743251898692627, 92.54379397006360364 ) ) ;
#58081=CARTESIAN_POINT ( 'NONE',  ( -95.88718821240198054, 29.65015105908826953, 60.93360808619399904 ) ) ;
#58083=CARTESIAN_POINT ( 'NONE',  ( -86.17927978631389863, 25.32700573188346738, 11.08567002189708717 ) ) ;
#58086=ORIENTED_EDGE ( 'NONE', *, *, #35735, .T. ) ;
#58087=CARTESIAN_POINT ( 'NONE',  ( 9.290502160020462696, 6.379616279862541539, -46.77255880539932065 ) ) ;
#58089=CARTESIAN_POINT ( 'NONE',  ( 16.77391662606470746, 6.533867394142989227, 18.12154318931471408 ) ) ;
#58091=CARTESIAN_POINT ( 'NONE',  ( -27.21071548940745544, 8.935354224959075609, 85.20262481687709055 ) ) ;
#58095=CARTESIAN_POINT ( 'NONE',  ( 181.0840389613909736, -170.0000000000000000, -43.72505766587962484 ) ) ;
#58096=CARTESIAN_POINT ( 'NONE',  ( -28.13266652174639759, 9.071935854491412599, 44.45274732610694457 ) ) ;
#58097=VECTOR ( 'NONE', #59339, 1000.000000000000000 ) ;
#58098=CARTESIAN_POINT ( 'NONE',  ( -142.9843132609581744, 60.12226089556227038, -65.44703247124222401 ) ) ;
#58103=CARTESIAN_POINT ( 'NONE',  ( -81.89510452344296709, 24.66033552777454929, -76.24616494515825593 ) ) ;
#58104=CARTESIAN_POINT ( 'NONE',  ( -4.530419073632062421, 6.697511735426034285, -89.81587080412703017 ) ) ;
#58108=CARTESIAN_POINT ( 'NONE',  ( 126.6576865394845584, 37.24426596493989194, 12.28561084184393870 ) ) ;
#58109=CARTESIAN_POINT ( 'NONE',  ( 36.57758730571628547, 8.058950843173096956, -89.85795502034081039 ) ) ;
#58111=EDGE_CURVE ( 'NONE', #37531, #27576, #35954, .T. ) ;
#58112=CARTESIAN_POINT ( 'NONE',  ( 66.94779593213119995, 13.61918177102165650, 16.85966954521656547 ) ) ;
#58113=CARTESIAN_POINT ( 'NONE',  ( -79.62207341875654265, 23.76621716825510688, 72.21703032857082860 ) ) ;
#58114=CARTESIAN_POINT ( 'NONE',  ( -102.2801239173131052, 32.78103895658057354, 30.51907450641510522 ) ) ;
#58116=AXIS2_PLACEMENT_3D ( 'NONE', #9313, #58186, #63125 ) ;
#58119=CARTESIAN_POINT ( 'NONE',  ( -52.01032469896254185, 14.92508508686765367, 84.64386905501486069 ) ) ;
#58123=CARTESIAN_POINT ( 'NONE',  ( 17.48988570800758424, 7.568061572928496794, -62.55499197079009122 ) ) ;
#58126=CARTESIAN_POINT ( 'NONE',  ( 63.49940197359692462, 12.78497925206075969, -23.87614024170608573 ) ) ;
#58127=CARTESIAN_POINT ( 'NONE',  ( 136.9654665832768501, 44.52067472585216734, -36.69392891266659262 ) ) ;
#58128=CARTESIAN_POINT ( 'NONE',  ( 32.09567473596477072, 7.571373529017937365, -41.40819426019592697 ) ) ;
#58132=EDGE_LOOP ( 'NONE', ( #65748, #67896, #6975, #41297 ) ) ;
#58135=CARTESIAN_POINT ( 'NONE',  ( 175.3045235163616837, 74.34220674874238455, 85.66341389582093768 ) ) ;
#58146=CARTESIAN_POINT ( 'NONE',  ( 89.87518614971250486, 20.55373388674512825, -23.25513048290722296 ) ) ;
#58150=( BOUNDED_CURVE ( )  B_SPLINE_CURVE ( 3, ( #18537, #60402, #34727, #39989 ),
 .UNSPECIFIED., .F., .F. ) 
 B_SPLINE_CURVE_WITH_KNOTS ( ( 4, 4 ),
 ( 2.506209174768084580, 3.776976132411492326 ),
 .UNSPECIFIED. ) 
 CURVE ( )  GEOMETRIC_REPRESENTATION_ITEM ( )  RATIONAL_B_SPLINE_CURVE ( ( 1.000000000000000000, 0.8698961108463052483, 0.8698961108463052483, 1.000000000000000000 ) ) 
 REPRESENTATION_ITEM ( '' )  );
#58152=CARTESIAN_POINT ( 'NONE',  ( 126.7877523219523539, 38.47018873135925077, 12.72568023100204293 ) ) ;
#58154=DIRECTION ( 'NONE',  ( -0.000000000000000000, 1.000000000000000000, -0.000000000000000000 ) ) ;
#58156=CARTESIAN_POINT ( 'NONE',  ( -47.95193882091084703, 12.89180642785319009, -45.18069670428837270 ) ) ;
#58164=AXIS2_PLACEMENT_3D ( 'NONE', #58614, #15025, #10429 ) ;
#58166=CARTESIAN_POINT ( 'NONE',  ( 32.99392442438140449, 8.673943046035248017, 94.99999999999866418 ) ) ;
#58167=CARTESIAN_POINT ( 'NONE',  ( -180.3158531669106139, 95.51092859788505507, -71.19633455476439110 ) ) ;
#58168=CARTESIAN_POINT ( 'NONE',  ( 136.8043112934651617, 44.41959649939953181, -90.31326922588782224 ) ) ;
#58172=CARTESIAN_POINT ( 'NONE',  ( 32.14349651933086705, 7.576119504381661152, -18.22641918543651585 ) ) ;
#58173=CARTESIAN_POINT ( 'NONE',  ( 180.2565361171341181, 79.19912802278405195, -51.19124638010620032 ) ) ;
#58174=CARTESIAN_POINT ( 'NONE',  ( 162.0913721763116087, 61.33513738594646725, 84.68278974389512825 ) ) ;
#58177=CARTESIAN_POINT ( 'NONE',  ( 110.2429982417149432, 29.99119854320847267, -24.07788697519002596 ) ) ;
#58178=CARTESIAN_POINT ( 'NONE',  ( 15.29899606819417279, 6.485153354884285015, 56.85925826316891118 ) ) ;
#58179=CARTESIAN_POINT ( 'NONE',  ( 12.04188192036245297, 7.416006018508747744, 31.01281317854670760 ) ) ;
#58180=CARTESIAN_POINT ( 'NONE',  ( 199.3764173596861724, 100.9540560740992134, 31.39806225150986663 ) ) ;
#58182=CARTESIAN_POINT ( 'NONE',  ( -149.5074843970971301, -170.0000000000000000, 65.06537183036276417 ) ) ;
#58184=ORIENTED_EDGE ( 'NONE', *, *, #66326, .F. ) ;
#58186=DIRECTION ( 'NONE',  ( 0.000000000000000000, 0.000000000000000000, 1.000000000000000000 ) ) ;
#58188=CYLINDRICAL_SURFACE ( 'NONE', #1330, 7.500000000000013323 ) ;
#58190=CARTESIAN_POINT ( 'NONE',  ( -123.6619986853277879, 45.04188181212062148, 72.12840242753554776 ) ) ;
#58192=CARTESIAN_POINT ( 'NONE',  ( 150.0501577908836737, 52.10460126680128212, -69.34286162853243241 ) ) ;
#58193=CARTESIAN_POINT ( 'NONE',  ( 22.86512557549835378, 7.838421172085543454, -94.18957475688611680 ) ) ;
#58196=ORIENTED_EDGE ( 'NONE', *, *, #13276, .F. ) ;
#58201=CARTESIAN_POINT ( 'NONE',  ( -83.53167274806556009, 25.32068190668983831, -36.88675501431261949 ) ) ;
#58202=CARTESIAN_POINT ( 'NONE',  ( 102.8207208422076491, 25.59711495857310837, 89.66725988627140964 ) ) ;
#58203=CARTESIAN_POINT ( 'NONE',  ( -156.6644740249450933, 71.86407434531903959, 9.117256437103197442 ) ) ;
#58212=CARTESIAN_POINT ( 'NONE',  ( 31.96192885395475614, 8.569232728322425885, -42.14181525861992839 ) ) ;
#58216=CARTESIAN_POINT ( 'NONE',  ( -35.38962320578854559, 11.29584325137389200, -63.28181392470004596 ) ) ;
#58218=ORIENTED_EDGE ( 'NONE', *, *, #37814, .F. ) ;
#58220=CYLINDRICAL_SURFACE ( 'NONE', #58496, 7.500000000000013323 ) ;
#58222=CARTESIAN_POINT ( 'NONE',  ( 22.28556289340101060, 7.803548444155008035, 6.915694015335128952 ) ) ;
#58224=CARTESIAN_POINT ( 'NONE',  ( -119.6995109608660925, 42.54844499216736153, 7.039243325925482964 ) ) ;
#58226=CARTESIAN_POINT ( 'NONE',  ( 126.6576865394845584, 37.24426596493988484, -14.55893974861973916 ) ) ;
#58228=CARTESIAN_POINT ( 'NONE',  ( 11.82929895397812636, 7.412564870773630687, 4.295403894678821111 ) ) ;
#58230=CARTESIAN_POINT ( 'NONE',  ( 181.9406741394862195, 79.47484497224793643, 17.42709078222137009 ) ) ;
#58232=CARTESIAN_POINT ( 'NONE',  ( 175.5406524085945534, 73.17873692326779178, 31.73118722595227936 ) ) ;
#58234=CARTESIAN_POINT ( 'NONE',  ( -109.7079446832839125, 37.86719386855315861, -43.58491357317385706 ) ) ;
#58235=CARTESIAN_POINT ( 'NONE',  ( 187.2384682876462421, 86.54721710842892435, -39.40919725149962005 ) ) ;
#58237=ORIENTED_EDGE ( 'NONE', *, *, #57298, .T. ) ;
#58238=DIRECTION ( 'NONE',  ( -0.000000000000000000, 1.000000000000000000, -0.000000000000000000 ) ) ;
#58239=CARTESIAN_POINT ( 'NONE',  ( 173.5979703267912271, 71.35727699437038041, 89.88741889385630657 ) ) ;
#58242=CARTESIAN_POINT ( 'NONE',  ( 117.6865880453676283, 32.48051379280607165, 62.90051310914670779 ) ) ;
#58248=CARTESIAN_POINT ( 'NONE',  ( 161.3420394500905957, 60.72502592113882969, -90.87834266692578922 ) ) ;
#58249=AXIS2_PLACEMENT_3D ( 'NONE', #36229, #15464, #58025 ) ;
#58251=FACE_OUTER_BOUND ( 'NONE', #57411, .T. ) ;
#58256=CARTESIAN_POINT ( 'NONE',  ( -118.5043919384111746, 41.81711884544878899, -14.25870488645683842 ) ) ;
#58258=CARTESIAN_POINT ( 'NONE',  ( -180.0179082103088035, 95.14811732286300128, -12.40625655228225988 ) ) ;
#58259=CARTESIAN_POINT ( 'NONE',  ( -148.6426981422629297, 63.44891673852537650, -49.77548511292598477 ) ) ;
#58261=CARTESIAN_POINT ( 'NONE',  ( -106.0230121908585375, 35.86256082048880955, 85.20199266763809476 ) ) ;
#58264=CARTESIAN_POINT ( 'NONE',  ( -62.30100056228381789, 16.74548393487071607, -13.88027663460116123 ) ) ;
#58265=EDGE_CURVE ( 'NONE', #145, #39302, #16578, .T. ) ;
#58266=CARTESIAN_POINT ( 'NONE',  ( -125.8938041572051389, 47.69968343338780414, -61.75825448869760237 ) ) ;
#58268=CARTESIAN_POINT ( 'NONE',  ( -95.04120270830166817, 29.25306318840326369, 13.20312441486970911 ) ) ;
#58269=CARTESIAN_POINT ( 'NONE',  ( -101.8145602049406051, 32.54453702486151201, -61.85912785543960268 ) ) ;
#58270=ORIENTED_EDGE ( 'NONE', *, *, #67137, .T. ) ;
#58272=EDGE_CURVE ( 'NONE', #32966, #18071, #65821, .T. ) ;
#58273=CARTESIAN_POINT ( 'NONE',  ( 188.2988323915788840, 86.21831227955483712, -68.49994268373441741 ) ) ;
#58276=CARTESIAN_POINT ( 'NONE',  ( 109.3154830994003675, 29.56170298203815250, -77.72415834473385132 ) ) ;
#58277=CARTESIAN_POINT ( 'NONE',  ( -75.00636493611887090, 22.03142602679956852, 44.48221497804134117 ) ) ;
#58278=CARTESIAN_POINT ( 'NONE',  ( -75.43271753227890031, 22.18711452892411273, -62.67581109114816940 ) ) ;
#58280=CARTESIAN_POINT ( 'NONE',  ( -120.1650841064593749, 44.02024060322521137, 42.96702436344589415 ) ) ;
#58285=CARTESIAN_POINT ( 'NONE',  ( -12.78015296493257935, 7.264294661536299103, -37.26654318863142379 ) ) ;
#58286=CARTESIAN_POINT ( 'NONE',  ( 84.26390409839193296, 19.68678207880320485, 71.19001783865050470 ) ) ;
#58289=CARTESIAN_POINT ( 'NONE',  ( 157.4703587214989113, 57.65129005721576050, -9.279633708673953763 ) ) ;
#58294=CARTESIAN_POINT ( 'NONE',  ( 38.90894112122322213, 8.345444037631240874, -62.46436805589143404 ) ) ;
#58295=CARTESIAN_POINT ( 'NONE',  ( -99.99439884168252490, 32.75762661251357599, -62.20012547770417655 ) ) ;
#58296=CARTESIAN_POINT ( 'NONE',  ( -35.38962320578853138, 11.29584325137385292, -9.592712743772663586 ) ) ;
#58301=CARTESIAN_POINT ( 'NONE',  ( 204.6977192012829505, 108.0580384837234931, -51.32593103262161094 ) ) ;
#58303=CARTESIAN_POINT ( 'NONE',  ( -24.70354720400823112, 8.582324684301863016, 14.20767813331848117 ) ) ;
#58304=DIRECTION ( 'NONE',  ( -0.000000000000000000, 1.000000000000000000, -0.000000000000000000 ) ) ;
#58305=CARTESIAN_POINT ( 'NONE',  ( -11.14445507968271976, 7.129894202659276203, -76.49272796307144517 ) ) ;
#58307=CARTESIAN_POINT ( 'NONE',  ( 149.9683128897950155, 53.28564708287392904, -43.09392792187862398 ) ) ;
#58311=CARTESIAN_POINT ( 'NONE',  ( 178.1965488566140152, 77.14488558164481447, -23.81576150532814040 ) ) ;
#58315=CARTESIAN_POINT ( 'NONE',  ( -125.8938041572051389, -170.0000000000000000, -8.069153307770243089 ) ) ;
#58316=CARTESIAN_POINT ( 'NONE',  ( -0.3258398948454893640, 6.518608385615800138, -16.57484821353645188 ) ) ;
#58317=CARTESIAN_POINT ( 'NONE',  ( 198.2588776805010582, 99.52972231602376496, -20.83770437927799435 ) ) ;
#58318=CARTESIAN_POINT ( 'NONE',  ( -155.7921081844114894, 69.69879669332561889, 87.80423241437721060 ) ) ;
#58319=CARTESIAN_POINT ( 'NONE',  ( 135.4423125506059478, 42.39015362494588146, 29.67632823401072173 ) ) ;
#58322=CARTESIAN_POINT ( 'NONE',  ( -149.5074843970971301, -170.0000000000000000, 11.37627064943538890 ) ) ;
#58323=CARTESIAN_POINT ( 'NONE',  ( 181.9295958320008708, 80.90438706151871884, 29.34426735614494319 ) ) ;
#58324=CARTESIAN_POINT ( 'NONE',  ( 154.0515132159917755, 56.29926936869308918, 30.21783921907742609 ) ) ;
#58328=CARTESIAN_POINT ( 'NONE',  ( 173.8576514579035859, 72.97529922124009261, 65.68134040125295314 ) ) ;
#58331=CARTESIAN_POINT ( 'NONE',  ( -109.5025362253418564, 36.60371748273998094, -40.42792366826092376 ) ) ;
#58332=CARTESIAN_POINT ( 'NONE',  ( 68.45098769362921587, 13.99935947269945480, -75.23886394023182334 ) ) ;
#58335=CARTESIAN_POINT ( 'NONE',  ( 155.7167524447090159, 57.56687707799950715, 17.37047274630594274 ) ) ;
#58337=CARTESIAN_POINT ( 'NONE',  ( -180.5230320745700965, 95.76406004447552789, 37.07285121458210853 ) ) ;
#58342=DIRECTION ( 'NONE',  ( 0.000000000000000000, 0.000000000000000000, 1.000000000000000000 ) ) ;
#58345=CARTESIAN_POINT ( 'NONE',  ( 139.6359093656973585, 45.02518919224739591, 68.64155198831963389 ) ) ;
#58346=CARTESIAN_POINT ( 'NONE',  ( -174.7817412490651918, 90.52199442492064918, 30.99576591545036308 ) ) ;
#58348=CARTESIAN_POINT ( 'NONE',  ( 92.52113039222217594, 22.58921125235801952, 41.87899094217726059 ) ) ;
#58352=B_SPLINE_CURVE_WITH_KNOTS ( 'NONE', 3,
 ( #31495, #47307, #41367, #15662, #3718, #36426, #57198, #31835, #20935, #14961, #68767, #25197, #20582, #52927, #68106, #57881, #4753, #26216, #46632, #42044, #4079, #68438, #14287, #19912, #52257, #62820, #25544, #42391, #14624, #63853, #47655, #69460, #9700, #37110, #53271, #5100, #47997, #21279, #41704, #36087, #42728, #35747, #57543, #9346 ),
 .UNSPECIFIED., .F., .F.,
 ( 4, 2, 2, 2, 2, 2, 2, 2, 2, 2, 2, 2, 2, 2, 2, 2, 2, 2, 2, 2, 2, 4 ),
 ( 0.02814986980477065734, 0.02995274102020802770, 0.03085417662792672502, 0.03175561223564542235, 0.03355848345108278924, 0.03536135466652016307, 0.03716422588195752996, 0.03896709709739489685, 0.03986853270511355601, 0.04076996831283221517, 0.04167140392055087433, 0.04257283952826951268, 0.04347427513598819959, 0.04437571074370687263, 0.04527714635142555955, 0.04617858195914423952, 0.04798145317458163417, 0.04978432439001902882, 0.05158719560545642346, 0.05339006682089381811, 0.05519293803633121276, 0.05699580925176860741 ),
 .UNSPECIFIED. ) ;
#58356=CARTESIAN_POINT ( 'NONE',  ( -61.99282085258081310, 16.65258086416814010, 94.42360237343419271 ) ) ;
#58357=CARTESIAN_POINT ( 'NONE',  ( 106.6322547488295385, 28.34756922280616465, 30.52000857272038914 ) ) ;
#58367=CARTESIAN_POINT ( 'NONE',  ( -94.84390436305042726, 29.16104988397310294, -41.50425148441384238 ) ) ;
#58369=CARTESIAN_POINT ( 'NONE',  ( 62.52742438962774685, 12.55954017561948000, -62.56524142263339172 ) ) ;
#58370=CARTESIAN_POINT ( 'NONE',  ( -55.05276343752909440, 15.72344139423348786, -77.06087458892358200 ) ) ;
#58371=CARTESIAN_POINT ( 'NONE',  ( -122.8202784017355498, 45.69728649588467562, 71.80980446227590619 ) ) ;
#58372=CARTESIAN_POINT ( 'NONE',  ( 16.27775141556967853, 7.523247835309960330, 30.01470767270521733 ) ) ;
#58376=CARTESIAN_POINT ( 'NONE',  ( 163.5944442552009832, 63.88381951184481267, -66.13186425301876170 ) ) ;
#58380=CARTESIAN_POINT ( 'NONE',  ( 201.4688124904258189, 102.0170968684381450, -90.70582092648642458 ) ) ;
#58383=CARTESIAN_POINT ( 'NONE',  ( -154.7934364910360614, 68.79594655117534785, 43.54706751354447647 ) ) ;
#58389=CARTESIAN_POINT ( 'NONE',  ( -129.3970594949620079, 50.06339481638099187, 31.47202801301698116 ) ) ;
#58393=CARTESIAN_POINT ( 'NONE',  ( 62.52742438962774685, 12.55954017561948000, 71.65751152968499582 ) ) ;
#58394=CARTESIAN_POINT ( 'NONE',  ( -1.866625526081663988, 7.583073082893622363, 69.04121920335192897 ) ) ;
#58401=CARTESIAN_POINT ( 'NONE',  ( -173.1211646369891071, 87.12891641440859303, -22.86740657428632773 ) ) ;
#58403=CARTESIAN_POINT ( 'NONE',  ( -48.41612563322100016, 14.03642305406760471, 94.99999999999866418 ) ) ;
#58405=CARTESIAN_POINT ( 'NONE',  ( 21.96910889293877034, 7.784886455511741410, 86.90482503240505707 ) ) ;
#58406=VERTEX_POINT ( 'NONE', #1799 ) ;
#58407=EDGE_CURVE ( 'NONE', #22455, #44611, #17969, .T. ) ;
#58414=ORIENTED_EDGE ( 'NONE', *, *, #21048, .F. ) ;
#58416=CARTESIAN_POINT ( 'NONE',  ( -118.6727642982647524, 43.09863379477474155, 9.178398134959156351 ) ) ;
#58418=CARTESIAN_POINT ( 'NONE',  ( -175.9970298498767249, 90.38640259140136379, 58.22642001971374981 ) ) ;
#58419=CARTESIAN_POINT ( 'NONE',  ( 18.89064107370903045, 6.619789970027398773, 17.50279535283585375 ) ) ;
#58422=ADVANCED_FACE ( 'NONE', ( #61224 ), #2484, .F. ) ;
#58423=CARTESIAN_POINT ( 'NONE',  ( -27.48409822889280463, 8.975441763201041923, 85.02499692473053017 ) ) ;
#58424=CARTESIAN_POINT ( 'NONE',  ( 153.4268936273268764, 54.57409659828383752, 30.58846441339344580 ) ) ;
#58426=CARTESIAN_POINT ( 'NONE',  ( 105.4193882736796297, 26.71329717705295081, -49.18680799141433369 ) ) ;
#58427=ADVANCED_FACE ( 'NONE', ( #51369 ), #13389, .F. ) ;
#58428=CARTESIAN_POINT ( 'NONE',  ( 140.2058232509808704, 46.59155168125936086, -66.34433898568947541 ) ) ;
#58433=CARTESIAN_POINT ( 'NONE',  ( -85.36298448216594181, 26.07611629625833416, -66.04488118901366533 ) ) ;
#58434=CARTESIAN_POINT ( 'NONE',  ( 117.4396227366912626, 32.35611529020199129, -95.00000000000133582 ) ) ;
#58435=CARTESIAN_POINT ( 'NONE',  ( -118.4709174626548531, 42.97515378817186615, -41.30754075210906251 ) ) ;
#58436=CARTESIAN_POINT ( 'NONE',  ( -86.16504208171677703, 26.41251233979375712, 10.54396692358523779 ) ) ;
#58440=CYLINDRICAL_SURFACE ( 'NONE', #18658, 7.500000000000020428 ) ;
#58442=CARTESIAN_POINT ( 'NONE',  ( -173.1211646369891355, -170.0000000000000000, -61.55650775521367279 ) ) ;
#58449=CARTESIAN_POINT ( 'NONE',  ( 22.51798020284706681, 7.817376421459704794, -73.18340610876502694 ) ) ;
#58452=CARTESIAN_POINT ( 'NONE',  ( 70.26722489419891815, 14.47234958177329212, -18.35366578844314134 ) ) ;
#58453=AXIS2_PLACEMENT_3D ( 'NONE', #46338, #29478, #25606 ) ;
#58456=CARTESIAN_POINT ( 'NONE',  ( 140.2200249818744169, 46.60103563593122544, -47.50120530054586965 ) ) ;
#58457=CARTESIAN_POINT ( 'NONE',  ( -52.67596829228263289, 15.09584868440940220, -76.69087494152185513 ) ) ;
#58458=LINE ( 'NONE', #5002, #2739 ) ;
#58460=CARTESIAN_POINT ( 'NONE',  ( -119.5563837756079693, 43.64229894412654431, -11.52668347953698280 ) ) ;
#58463=CARTESIAN_POINT ( 'NONE',  ( 180.1110850744962022, 79.05158019587979368, 83.03841359423326196 ) ) ;
#58469=CARTESIAN_POINT ( 'NONE',  ( 91.49210130311618627, 22.20929244416438308, 16.08268542465916795 ) ) ;
#58470=CARTESIAN_POINT ( 'NONE',  ( 185.1710994180822354, 84.30654632312743502, -10.57602910970770616 ) ) ;
#58471=CARTESIAN_POINT ( 'NONE',  ( -85.75222301046103723, 25.14826148333820299, -13.26214896379232400 ) ) ;
#58473=CARTESIAN_POINT ( 'NONE',  ( 92.19920907511537678, 21.39700525884451210, -21.52306413018001052 ) ) ;
#58478=CARTESIAN_POINT ( 'NONE',  ( 133.4058733589412782, 42.32720528873922206, 2.665790248531677786 ) ) ;
#58482=CARTESIAN_POINT ( 'NONE',  ( 8.000000000000007105, 249.8719672152120381, -95.00000000000133582 ) ) ;
#58483=CARTESIAN_POINT ( 'NONE',  ( -3.810800745967052539, 7.670052258724785688, 84.96130854411160271 ) ) ;
#58486=CARTESIAN_POINT ( 'NONE',  ( -56.96214175905167565, 15.20165595797839231, 71.91879777619202230 ) ) ;
#58487=ORIENTED_EDGE ( 'NONE', *, *, #50771, .T. ) ;
#58488=VERTEX_POINT ( 'NONE', #23939 ) ;
#58489=EDGE_CURVE ( 'NONE', #69371, #40284, #54312, .T. ) ;
#58490=CARTESIAN_POINT ( 'NONE',  ( 34.30959576864569271, 8.813794125124662315, 85.58691292226393443 ) ) ;
#58491=CARTESIAN_POINT ( 'NONE',  ( -180.4643341113398378, 95.69224917234934935, -67.50112049958217142 ) ) ;
#58494=FACE_OUTER_BOUND ( 'NONE', #20438, .T. ) ;
#58496=AXIS2_PLACEMENT_3D ( 'NONE', #10036, #37108, #38140 ) ;
#58497=CARTESIAN_POINT ( 'NONE',  ( -4.072522659361690778, 7.683023425615369106, 4.272846646336744492 ) ) ;
#58498=CARTESIAN_POINT ( 'NONE',  ( 175.8874477961783498, 74.89984466412600739, -38.29623224188777897 ) ) ;
#58499=CARTESIAN_POINT ( 'NONE',  ( -154.0716379918897303, 69.49957566103796580, -75.12760008809200940 ) ) ;
#58506=CARTESIAN_POINT ( 'NONE',  ( 102.7983318509015049, 26.68040613344513545, -17.62410043733592957 ) ) ;
#58509=CARTESIAN_POINT ( 'NONE',  ( -55.05276343752910151, -170.0000000000000000, 37.81732777293115078 ) ) ;
#58512=CARTESIAN_POINT ( 'NONE',  ( -85.93597956139524285, 26.31611237855608820, 93.48078942079631304 ) ) ;
#58523=CARTESIAN_POINT ( 'NONE',  ( -8.320534640989468045, 7.931748412542454219, -8.573520141480125645 ) ) ;
#58524=CARTESIAN_POINT ( 'NONE',  ( 149.9552318559266837, 52.03645904563055069, -70.44558198621334100 ) ) ;
#58525=CARTESIAN_POINT ( 'NONE',  ( 19.74724861314306779, 6.659670522263895442, -22.54914667598139388 ) ) ;
#58526=FACE_OUTER_BOUND ( 'NONE', #18199, .T. ) ;
#58529=CARTESIAN_POINT ( 'NONE',  ( 70.26639875985991068, 15.51307715494295891, -14.39416547209034647 ) ) ;
#58530=CARTESIAN_POINT ( 'NONE',  ( -85.12122836439579032, 25.97531040437158723, -38.76424601805629777 ) ) ;
#58531=CARTESIAN_POINT ( 'NONE',  ( 103.0509289023981125, 25.69456821447926842, 88.64481294647117693 ) ) ;
#58532=CARTESIAN_POINT ( 'NONE',  ( -155.7457403566965581, 71.01814553754121562, 7.182542572017481142 ) ) ;
#58534=CARTESIAN_POINT ( 'NONE',  ( 19.11168290073779019, 6.629794975642857580, 44.24265699935381235 ) ) ;
#58536=CARTESIAN_POINT ( 'NONE',  ( -156.8260034364761282, 72.01363188529046511, 90.23433487043809009 ) ) ;
#58537=VERTEX_POINT ( 'NONE', #35878 ) ;
#58538=B_SPLINE_CURVE_WITH_KNOTS ( 'NONE', 3,
 ( #10520, #31991, #22119, #21424, #11549, #60094, #11914, #65036, #16836, #47812, #33026, #69272, #42866, #64336, #16147, #28443, #23527, #44968, #17541, #39699, #29485, #50947, #66453, #18240 ),
 .UNSPECIFIED., .F., .F.,
 ( 4, 2, 2, 2, 2, 2, 2, 2, 2, 2, 2, 4 ),
 ( 0.01129708592246000433, 0.01269909149731377786, 0.01410109707216755312, 0.01550310264702132665, 0.01620410543444821341, 0.01690510822187510018, 0.01830711379672887024, 0.01900811658415573965, 0.01970911937158260907, 0.02111112494643635137, 0.02181212773386321385, 0.02251313052129007633 ),
 .UNSPECIFIED. ) ;
#58541=CARTESIAN_POINT ( 'NONE',  ( -151.2428028786328014, 66.99705074331123456, -22.77775578256537514 ) ) ;
#58543=CARTESIAN_POINT ( 'NONE',  ( 180.2473887773228398, 77.76029175826239737, 71.15314469597515767 ) ) ;
#58545=CARTESIAN_POINT ( 'NONE',  ( -34.06864996337443330, 10.03773626259441798, 71.58918042140540194 ) ) ;
#58546=DIRECTION ( 'NONE',  ( -0.000000000000000000, 1.000000000000000000, -0.000000000000000000 ) ) ;
#58549=CARTESIAN_POINT ( 'NONE',  ( 8.848532525911927848, 6.377649276597440853, -13.29886354056554509 ) ) ;
#58554=CARTESIAN_POINT ( 'NONE',  ( -80.54757501605355685, 23.04700348514568375, -35.35128041769551999 ) ) ;
#58555=CARTESIAN_POINT ( 'NONE',  ( 17.74393407086868635, 6.570779001277777809, 71.61667146331731715 ) ) ;
#58557=CARTESIAN_POINT ( 'NONE',  ( 8.478575283864733692, 7.382882227715640511, 12.36660011482083199 ) ) ;
#58559=EDGE_LOOP ( 'NONE', ( #16053, #44508, #1138, #22597 ) ) ;
#58563=CARTESIAN_POINT ( 'NONE',  ( 133.8566784816069060, 42.60093787723652525, -36.02331093239566684 ) ) ;
#58565=CARTESIAN_POINT ( 'NONE',  ( -109.0291978193666438, 37.49173305805086898, -45.79549089733289691 ) ) ;
#58566=CARTESIAN_POINT ( 'NONE',  ( 59.73312635112155533, 12.96464920523512276, -76.82611381836962039 ) ) ;
#58570=EDGE_CURVE ( 'NONE', #56686, #41593, #15112, .T. ) ;
#58571=CARTESIAN_POINT ( 'NONE',  ( -24.41864932425148993, 8.543938959778813569, -13.32222848996388365 ) ) ;
#58573=CARTESIAN_POINT ( 'NONE',  ( 197.5344433744249670, 98.61756151884684130, 12.10789136445144898 ) ) ;
#58575=EDGE_CURVE ( 'NONE', #59876, #61401, #65116, .T. ) ;
#58576=DIRECTION ( 'NONE',  ( 0.000000000000000000, 0.000000000000000000, 1.000000000000000000 ) ) ;
#58580=CARTESIAN_POINT ( 'NONE',  ( 39.40195752203892710, -170.0000000000000000, -89.30891864635511013 ) ) ;
#58581=CARTESIAN_POINT ( 'NONE',  ( -95.50384525802328994, 29.46973564057715933, 41.24368704753796777 ) ) ;
#58582=CARTESIAN_POINT ( 'NONE',  ( 93.86680996363766383, 22.01878169039502708, -41.33864978769346266 ) ) ;
#58584=ORIENTED_EDGE ( 'NONE', *, *, #33846, .T. ) ;
#58587=ORIENTED_EDGE ( 'NONE', *, *, #874, .F. ) ;
#58588=CARTESIAN_POINT ( 'NONE',  ( -119.5267374018686724, 42.44190186039715229, -11.57287640902848302 ) ) ;
#58591=CARTESIAN_POINT ( 'NONE',  ( -173.1211646369891071, 87.12891641440859303, -7.867406574286297527 ) ) ;
#58592=ADVANCED_FACE ( 'NONE', ( #39600 ), #7602, .F. ) ;
#58593=CARTESIAN_POINT ( 'NONE',  ( -168.7314919967217861, 83.83749564070829763, -62.95703578078057205 ) ) ;
#58594=CARTESIAN_POINT ( 'NONE',  ( -146.1142527948576344, 61.35394402951020965, -35.62045372895397577 ) ) ;
#58596=CARTESIAN_POINT ( 'NONE',  ( 62.05396267233468421, 13.48332220860126363, 3.014455481275966964 ) ) ;
#58599=CARTESIAN_POINT ( 'NONE',  ( 55.93149085255341646, 12.16676074274502106, 93.48784098346216354 ) ) ;
#58600=CARTESIAN_POINT ( 'NONE',  ( -62.56514138729678365, 16.82532522382519602, -15.86430600984316541 ) ) ;
#58603=CARTESIAN_POINT ( 'NONE',  ( 134.3159642998340644, 41.70198410084978491, -24.17876034193201207 ) ) ;
#58604=CARTESIAN_POINT ( 'NONE',  ( -132.2286325684322605, 52.04087929935081291, -65.23503918443411465 ) ) ;
#58607=CARTESIAN_POINT ( 'NONE',  ( -151.7098557585652543, 66.07042764902350029, -88.82961873973066247 ) ) ;
#58608=ORIENTED_EDGE ( 'NONE', *, *, #16575, .F. ) ;
#58610=B_SPLINE_CURVE_WITH_KNOTS ( 'NONE', 3,
 ( #26509, #47948, #10663, #69417, #21233, #37746, #42680, #52207, #11012, #47263, #58853, #32131, #41652, #63108, #9649, #5400, #26854, #15267, #48280, #108, #31111, #41995, #43008, #59191, #25493, #46931, #52547, #68394, #68719, #4370, #36730, #14909, #20528, #22971, #27895, #43704, #38091, #38449, #23330, #27188, #16635, #17332, #7133, #17697, #49330, #28595 ),
 .UNSPECIFIED., .F., .F.,
 ( 4, 2, 2, 2, 2, 2, 2, 2, 2, 2, 2, 2, 2, 2, 2, 2, 2, 2, 2, 2, 2, 2, 4 ),
 ( 0.02404638330965502488, 0.02555608299537557096, 0.02631093283823584400, 0.02706578268109611704, 0.02857548236681666312, 0.02933033220967693616, 0.03008518205253720573, 0.03159488173825774487, 0.03310458142397829095, 0.03385943126683856746, 0.03461428110969884397, 0.03612398079541942475, 0.03687883063827971514, 0.03763368048114000552, 0.03838853032400028897, 0.03914338016686057936, 0.04065307985258115320, 0.04216277953830172703, 0.04367247922402230087, 0.04518217890974287471, 0.04593702875260315122, 0.04669187859546342079, 0.04820157828118395993 ),
 .UNSPECIFIED. ) ;
#58611=CARTESIAN_POINT ( 'NONE',  ( 181.5072453427590347, 79.03352099595183233, -78.06960825634332934 ) ) ;
#58614=CARTESIAN_POINT ( 'NONE',  ( 8.000000000000007105, 249.8719672152120381, -95.00000000000133582 ) ) ;
#58616=CARTESIAN_POINT ( 'NONE',  ( 102.7983318509014907, 26.68040613344513901, -71.31320161826326398 ) ) ;
#58618=CARTESIAN_POINT ( 'NONE',  ( 86.14852828165531662, 19.25704475759651402, 44.71208757247934074 ) ) ;
#58620=CARTESIAN_POINT ( 'NONE',  ( -124.7710763417278486, 46.96042092553523162, 30.70098044976807472 ) ) ;
#58621=CARTESIAN_POINT ( 'NONE',  ( 208.6132326550594200, 111.8685719053116543, 69.96301817913980869 ) ) ;
#58623=CARTESIAN_POINT ( 'NONE',  ( -103.2129897037410871, 33.25684593987702442, -8.213834404042543724 ) ) ;
#58625=CARTESIAN_POINT ( 'NONE',  ( -33.37566357177431087, 9.916833145467597532, 3.609876264789644296 ) ) ;
#58627=CARTESIAN_POINT ( 'NONE',  ( 86.62931800182293784, 20.48449268398422163, 71.55663816294304524 ) ) ;
#58628=CARTESIAN_POINT ( 'NONE',  ( 153.8366942494330942, 54.87992279068317458, -10.21455127450128408 ) ) ;
#58630=CARTESIAN_POINT ( 'NONE',  ( 31.91375106836930087, 7.553354707452896832, -70.45236121604933999 ) ) ;
#58633=ORIENTED_EDGE ( 'NONE', *, *, #30497, .T. ) ;
#58635=ORIENTED_EDGE ( 'NONE', *, *, #34550, .F. ) ;
#58636=FACE_OUTER_BOUND ( 'NONE', #36891, .T. ) ;
#58637=CARTESIAN_POINT ( 'NONE',  ( 14.08810621383466888, 7.458732232275139040, -77.17239911336513103 ) ) ;
#58640=CARTESIAN_POINT ( 'NONE',  ( -7.330690860789852437, 6.858814156830895570, 45.11558103944722831 ) ) ;
#58646=FACE_OUTER_BOUND ( 'NONE', #55708, .T. ) ;
#58648=CARTESIAN_POINT ( 'NONE',  ( -104.7956873821848944, 35.21322275870666374, 57.79421275118836832 ) ) ;
#58651=CARTESIAN_POINT ( 'NONE',  ( -131.6399667378751417, 51.62465701391630546, -37.56756705236779936 ) ) ;
#58655=CARTESIAN_POINT ( 'NONE',  ( 86.62931800182293784, 19.42108912189599579, 71.55663816294304524 ) ) ;
#58657=CARTESIAN_POINT ( 'NONE',  ( 197.1979149960397990, 98.19687999752001417, -17.31673455087552682 ) ) ;
#58660=CARTESIAN_POINT ( 'NONE',  ( -142.0099858798915022, 58.07212099904398883, 92.31482491311859917 ) ) ;
#58662=CARTESIAN_POINT ( 'NONE',  ( 141.2470358420065395, 46.06959063280892508, 38.31547528062654351 ) ) ;
#58663=EDGE_LOOP ( 'NONE', ( #26817, #21576 ) ) ;
#58665=CARTESIAN_POINT ( 'NONE',  ( 79.18180043629685372, 18.06526831600447380, 9.348947895539573949 ) ) ;
#58666=CARTESIAN_POINT ( 'NONE',  ( 164.4760519199596160, 64.62478832434439369, 12.79513189614267077 ) ) ;
#58668=CARTESIAN_POINT ( 'NONE',  ( -99.99439884168255332, 32.75762661251358310, 45.17807688415053491 ) ) ;
#58671=CARTESIAN_POINT ( 'NONE',  ( 177.7964363391245115, 76.75162026635254620, 56.89705291110796281 ) ) ;
#58673=CARTESIAN_POINT ( 'NONE',  ( -78.19460645047368530, 22.14203592077026173, -23.27090004125422951 ) ) ;
#58674=CARTESIAN_POINT ( 'NONE',  ( 70.51601918574516503, 14.53832276813546187, -69.82681846071810128 ) ) ;
#58679=CARTESIAN_POINT ( 'NONE',  ( 159.2258951716709703, 60.31399909112330704, -50.92933666049088259 ) ) ;
#58680=LINE ( 'NONE', #53394, #33937 ) ;
#58683=CARTESIAN_POINT ( 'NONE',  ( -7.825402957745085430, 6.891034867348157178, 18.27103044898354511 ) ) ;
#58684=CARTESIAN_POINT ( 'NONE',  ( 133.8566784816069344, 41.42467568809808398, 71.35489142945907304 ) ) ;
#58685=CARTESIAN_POINT ( 'NONE',  ( -177.1381400275772364, 93.26609858452822266, 31.97318544253296224 ) ) ;
#58686=CARTESIAN_POINT ( 'NONE',  ( -31.43908319763709969, 9.591432048623765638, -77.16174795566554678 ) ) ;
#58688=CARTESIAN_POINT ( 'NONE',  ( -8.810383862755525541, 7.965311326754787480, 71.91157687480138350 ) ) ;
#58689=ORIENTED_EDGE ( 'NONE', *, *, #18316, .T. ) ;
#58691=AXIS2_PLACEMENT_3D ( 'NONE', #47860, #69322, #3928 ) ;
#58693=CARTESIAN_POINT ( 'NONE',  ( -61.75345348739024587, 16.58105022592818401, 88.12184266525186160 ) ) ;
#58705=CARTESIAN_POINT ( 'NONE',  ( -77.71490760329791669, 23.03637365463981013, 57.30817650044996014 ) ) ;
#58706=CARTESIAN_POINT ( 'NONE',  ( 210.1633650091869754, 114.1507944623967035, -75.81224102313898072 ) ) ;
#58707=CARTESIAN_POINT ( 'NONE',  ( 63.01563776193091826, 12.67277567978498176, -77.56524142263344856 ) ) ;
#58708=CARTESIAN_POINT ( 'NONE',  ( -71.67841390531691559, 19.78168466957076177, 8.338739886184526995 ) ) ;
#58709=CARTESIAN_POINT ( 'NONE',  ( -33.53812060177524756, 9.945300800226871019, -89.30285964580421876 ) ) ;
#58712=CARTESIAN_POINT ( 'NONE',  ( 197.7251597135301040, 97.24643299060919333, 93.16756453888348233 ) ) ;
#58713=CARTESIAN_POINT ( 'NONE',  ( 79.40386128751609363, 17.08093333150470627, -95.00000000000133582 ) ) ;
#58718=ORIENTED_EDGE ( 'NONE', *, *, #59298, .T. ) ;
#58720=CARTESIAN_POINT ( 'NONE',  ( -25.80443741485378695, 9.749985135376002532, -64.68774352177892695 ) ) ;
#58721=CARTESIAN_POINT ( 'NONE',  ( 55.76298701799387914, 11.10663440745151576, -41.24582562440557609 ) ) ;
#58727=CARTESIAN_POINT ( 'NONE',  ( -129.4036885357273832, 50.06837984316181434, 44.75204449613408997 ) ) ;
#58730=CARTESIAN_POINT ( 'NONE',  ( -145.3246383987844581, 62.00818849034185121, 31.99110557883703976 ) ) ;
#58731=CARTESIAN_POINT ( 'NONE',  ( 56.53635105806415595, 11.26263375223564189, 60.37194408587342309 ) ) ;
#58741=CARTESIAN_POINT ( 'NONE',  ( -167.1534554062404823, 80.72263015867909530, -10.81749311186897522 ) ) ;
#58742=CARTESIAN_POINT ( 'NONE',  ( 139.6203063421347395, 45.01495791936839197, -75.19273776508998708 ) ) ;
#58744=CARTESIAN_POINT ( 'NONE',  ( 70.11766033381772445, 14.43277633974326868, 34.85218099568896832 ) ) ;
#58745=CARTESIAN_POINT ( 'NONE',  ( 9.004128196032667120, 7.384459627096075174, 94.41859741811346396 ) ) ;
#58747=ORIENTED_EDGE ( 'NONE', *, *, #22784, .F. ) ;
#58749=CARTESIAN_POINT ( 'NONE',  ( -99.11448999425216755, 31.20120877265620507, 58.04825527040586763 ) ) ;
#58752=CARTESIAN_POINT ( 'NONE',  ( -74.79002408692176118, 20.88280597089421420, 44.34336250310679617 ) ) ;
#58754=AXIS2_PLACEMENT_3D ( 'NONE', #37633, #42229, #26404 ) ;
#58755=B_SPLINE_CURVE_WITH_KNOTS ( 'NONE', 3,
 ( #13154, #1196, #34618, #60288, #7872, #35986, #57096, #68006, #8913, #24404, #36330, #62013, #30710, #35647, #67655, #67321, #35295, #9252, #25446, #45845, #41267, #61674, #46182, #25788, #68346, #52159, #3976, #46885, #20150, #40225, #3622, #2941, #30363, #62723, #51815, #14527, #41601, #63060, #19107, #25093, #57441, #40561, #19452, #56750, #62372 ),
 .UNSPECIFIED., .F., .F.,
 ( 4, 2, 2, 1, 2, 2, 2, 2, 2, 2, 2, 2, 2, 2, 2, 2, 2, 2, 2, 2, 2, 2, 4 ),
 ( 0.02346057189573570387, 0.02492590417315496479, 0.02565857031186459525, 0.02639123645057422224, 0.02712390258928384923, 0.02785656872799347969, 0.02932190100541272326, 0.03005456714412233984, 0.03078723328283195643, 0.03225256556025118265, 0.03298523169896080964, 0.03371789783767042969, 0.03518323011508967674, 0.03664856239250892378, 0.03738122853121855771, 0.03811389466992819164, 0.03957922694734745950, 0.04104455922476672736, 0.04250989150218598828, 0.04324255764089562915, 0.04397522377960525614, 0.04544055605702452399, 0.04690588833444379185 ),
 .UNSPECIFIED. ) ;
#58758=EDGE_LOOP ( 'NONE', ( #51367, #53728 ) ) ;
#58759=CARTESIAN_POINT ( 'NONE',  ( 10.13405324523498585, 6.385324379632244529, -47.97120849243911067 ) ) ;
#58760=EDGE_CURVE ( 'NONE', #28360, #62965, #50049, .T. ) ;
#58761=DIRECTION ( 'NONE',  ( -0.000000000000000000, 1.000000000000000000, -0.000000000000000000 ) ) ;
#58763=CARTESIAN_POINT ( 'NONE',  ( 126.4083787442700242, 37.10531539900951259, 62.82957637863194122 ) ) ;
#58766=CARTESIAN_POINT ( 'NONE',  ( 151.1873096904020883, 52.92629247302094342, 41.01321652849342314 ) ) ;
#58768=LINE ( 'NONE', #737, #46913 ) ;
#58774=CYLINDRICAL_SURFACE ( 'NONE', #47651, 242.4895526022646663 ) ;
#58778=CARTESIAN_POINT ( 'NONE',  ( -120.1346137380982100, 44.00127440773567145, -47.22450605392604928 ) ) ;
#58779=CARTESIAN_POINT ( 'NONE',  ( -78.66644367742109978, 23.39876645725288284, 3.573650549209446137 ) ) ;
#58781=CARTESIAN_POINT ( 'NONE',  ( -155.2912910578197057, 69.24479901948497229, 16.15753730191864435 ) ) ;
#58782=CARTESIAN_POINT ( 'NONE',  ( -118.3948752128398496, 42.92869324237091178, -68.96088763400301502 ) ) ;
#58783=CARTESIAN_POINT ( 'NONE',  ( 69.74037587279241279, 14.33355757956375420, 13.82632352699276623 ) ) ;
#58785=CARTESIAN_POINT ( 'NONE',  ( 42.22820723387685149, 9.810205105131432290, -89.85872570437997808 ) ) ;
#58786=ORIENTED_EDGE ( 'NONE', *, *, #13048, .T. ) ;
#58788=CARTESIAN_POINT ( 'NONE',  ( -37.07436112751822321, 11.60822760208521309, 15.84512009715484737 ) ) ;
#58790=DIRECTION ( 'NONE',  ( 0.000000000000000000, 0.000000000000000000, 1.000000000000000000 ) ) ;
#58792=CARTESIAN_POINT ( 'NONE',  ( 21.74799039132243905, 7.772294950329605712, -65.28364649508232276 ) ) ;
#58794=CARTESIAN_POINT ( 'NONE',  ( 181.0840389613909736, -170.0000000000000000, 56.15314469597509373 ) ) ;
#58797=CARTESIAN_POINT ( 'NONE',  ( 139.1306635769909690, 45.89653412152167533, -48.86132841697280327 ) ) ;
#58798=CARTESIAN_POINT ( 'NONE',  ( -54.57263979903868290, 15.59415114099632227, -77.06087458892358200 ) ) ;
#58800=B_SPLINE_CURVE_WITH_KNOTS ( 'NONE', 3,
 ( #51825, #24759, #41618, #46542, #51497, #63073, #52515, #3635, #67672, #25111, #9617, #4342, #59505, #48588, #22235, #27156, #53537, #65151, #38061, #26822, #64803, #10979, #64106, #428, #27502, #16603, #21532, #16258, #21878, #59852, #5698, #37033, #48941, #21202, #5365, #42977, #42650, #15584, #11321, #53876, #15917, #48249, #783, #26480 ),
 .UNSPECIFIED., .F., .F.,
 ( 4, 2, 2, 2, 2, 2, 2, 2, 2, 2, 2, 2, 2, 2, 2, 2, 2, 2, 2, 2, 2, 4 ),
 ( 1.430489624538199204E-17, 0.004120577325733403191, 0.006180865988600120833, 0.008241154651466839343, 0.01030144331433355785, 0.01133158764576691277, 0.01236173197720026595, 0.01339187630863362261, 0.01442202064006697752, 0.01545216497150033244, 0.01648230930293368562, 0.01699738146865036742, 0.01751245363436704575, 0.01854259796580040934, 0.01957274229723377640, 0.02060288662866714693, 0.02266317529153388799, 0.02472346395440062905, 0.02678375261726737358, 0.02781389694870078227, 0.02884404128013419444, 0.03296461860586794024 ),
 .UNSPECIFIED. ) ;
#58806=ORIENTED_EDGE ( 'NONE', *, *, #32620, .T. ) ;
#58808=CARTESIAN_POINT ( 'NONE',  ( 63.01563776193091826, 12.67277567978500130, -35.72069083216973695 ) ) ;
#58810=FACE_OUTER_BOUND ( 'NONE', #69168, .T. ) ;
#58811=AXIS2_PLACEMENT_3D ( 'NONE', #48870, #47849, #53118 ) ;
#58812=CARTESIAN_POINT ( 'NONE',  ( -173.1211646369891355, 88.63826465341152527, -7.867406574286299303 ) ) ;
#58817=CARTESIAN_POINT ( 'NONE',  ( 183.1873354889583254, 82.20882912211250471, -24.09245173917307881 ) ) ;
#58818=CARTESIAN_POINT ( 'NONE',  ( -85.09761763353360209, 24.87634954265997678, -11.90396085173015095 ) ) ;
#58820=CARTESIAN_POINT ( 'NONE',  ( 44.86216938219162387, 9.182565662897477665, -21.42266460005981799 ) ) ;
#58821=CARTESIAN_POINT ( 'NONE',  ( 206.6955592216991420, 109.1214665502618004, -24.22191070065747098 ) ) ;
#58824=CARTESIAN_POINT ( 'NONE',  ( 164.9547823171480729, 65.03046442419433504, 63.19433658183190516 ) ) ;
#58832=EDGE_CURVE ( 'NONE', #48157, #43438, #29871, .T. ) ;
#58833=CARTESIAN_POINT ( 'NONE',  ( 151.7819978880463054, 53.35998893001565335, 5.170581360776508539 ) ) ;
#58834=CARTESIAN_POINT ( 'NONE',  ( -10.38356729277384005, 8.080077440779504627, 84.24699796321192480 ) ) ;
#58835=VERTEX_POINT ( 'NONE', #59215 ) ;
#58840=CARTESIAN_POINT ( 'NONE',  ( 42.90062197766265228, 9.906944503464883311, 84.46083066505832448 ) ) ;
#58845=CARTESIAN_POINT ( 'NONE',  ( -58.96922974609609014, 15.76655591015166458, -75.96166564116519737 ) ) ;
#58847=CARTESIAN_POINT ( 'NONE',  ( 36.08729376665095145, 8.001156100723203934, -9.529628389809701616 ) ) ;
#58849=CARTESIAN_POINT ( 'NONE',  ( 174.6307688320643479, 73.70327352127000609, -47.55585792078556295 ) ) ;
#58851=CARTESIAN_POINT ( 'NONE',  ( 164.4125506877668101, 63.25654226895625953, 93.46064493613914692 ) ) ;
#58853=CARTESIAN_POINT ( 'NONE',  ( 91.11342358617754655, 21.00000175105273215, 31.19529170996127476 ) ) ;
#58855=CARTESIAN_POINT ( 'NONE',  ( 103.0004140566502997, 26.76634862952791138, -14.56365336300195601 ) ) ;
#58857=DIRECTION ( 'NONE',  ( 0.000000000000000000, 0.000000000000000000, 1.000000000000000000 ) ) ;
#58858=CARTESIAN_POINT ( 'NONE',  ( -29.50439180771547854, 10.29976981300626981, 30.45393202935034438 ) ) ;
#58864=VERTEX_POINT ( 'NONE', #44435 ) ;
#58865=CARTESIAN_POINT ( 'NONE',  ( 117.7417271423230147, 33.63613196344607559, -69.73183056102243427 ) ) ;
#58870=CARTESIAN_POINT ( 'NONE',  ( 150.0889146124742695, 52.13243511955542431, -71.82499747338286511 ) ) ;
#58872=ORIENTED_EDGE ( 'NONE', *, *, #20307, .T. ) ;
#58873=DIRECTION ( 'NONE',  ( 0.000000000000000000, 0.000000000000000000, 1.000000000000000000 ) ) ;
#58876=B_SPLINE_CURVE_WITH_KNOTS ( 'NONE', 3,
 ( #69108, #26559, #69459, #32872, #27238, #1214, #60651, #1559, #33235, #12464, #22319, #6493, #38861, #43759, #28289, #54665, #23021, #44473, #49382, #33586, #50100, #65230, #17024, #27940, #33929, #22667, #37801, #49730, #21964, #44106, #59248, #54304, #1929, #866, #55367, #44826, #12123, #23388, #38142, #59582, #65589, #7188, #48671 ),
 .UNSPECIFIED., .F., .F.,
 ( 4, 2, 2, 2, 2, 2, 2, 2, 1, 2, 2, 2, 2, 2, 2, 2, 2, 2, 2, 2, 2, 4 ),
 ( 0.000000000000000000, 0.001466540241398136407, 0.002199810362097204611, 0.002933080482796272814, 0.004399620724194415293, 0.005866160965592556904, 0.007332701206990699383, 0.008065971327689771056, 0.008799241448388842729, 0.009532511569087912667, 0.01026578168978698261, 0.01173232193118512422, 0.01319886217258326756, 0.01466540241398140744, 0.01539867253468046870, 0.01613194265537952823, 0.01759848289677765423, 0.01906502313817577329, 0.01979829325887483282, 0.02053156337957389582, 0.02199810362097202529, 0.02346464386237015476 ),
 .UNSPECIFIED. ) ;
#58878=CARTESIAN_POINT ( 'NONE',  ( -62.21585762900409833, 17.77081916367992420, -94.14025316589223280 ) ) ;
#58879=CARTESIAN_POINT ( 'NONE',  ( -30.17038805258401624, 10.40524961744439736, 84.00665816972750122 ) ) ;
#58880=CARTESIAN_POINT ( 'NONE',  ( -151.2428028786327445, 66.99705074331119192, 4.066794807898307162 ) ) ;
#58882=CARTESIAN_POINT ( 'NONE',  ( 23.03864809957654103, 6.841061756139152905, 39.44928671615922156 ) ) ;
#58884=EDGE_LOOP ( 'NONE', ( #490, #31788, #41712, #21625 ) ) ;
#58885=VERTEX_POINT ( 'NONE', #27556 ) ;
#58890=CARTESIAN_POINT ( 'NONE',  ( 32.66364305947235636, 8.639871491745257259, -39.78980533262777897 ) ) ;
#58891=B_SPLINE_CURVE_WITH_KNOTS ( 'NONE', 3,
 ( #49958, #1794, #23250, #60861, #44695, #55586, #12685, #50322, #2140, #66513, #23935, #13047, #34507, #9142, #25332, #52721, #41843, #62252, #30256, #40798, #68573, #41153, #36568, #9836, #57680, #3512, #30598, #62614, #46769, #24639, #20374, #3865, #67894, #46415, #42181, #14422, #36909, #25678, #68901, #58018, #36219, #46073, #15457, #19689, #68237, #20045, #51705 ),
 .UNSPECIFIED., .F., .F.,
 ( 4, 2, 2, 2, 2, 2, 2, 2, 2, 2, 2, 1, 2, 2, 2, 2, 2, 2, 2, 2, 2, 2, 2, 4 ),
 ( 0.000000000000000000, 0.003297771944419005796, 0.004122214930523717021, 0.004946657916628427812, 0.006595543888837832915, 0.007419986874942573196, 0.008244429861047314345, 0.009068872847152055494, 0.009893315833256796643, 0.01154220180546627027, 0.01236664479157100795, 0.01319108777767574216, 0.01401553076378047984, 0.01483997374988521752, 0.01566441673598995346, 0.01648885972209469114, 0.01813774569430418038, 0.01896218868040890071, 0.01978663166651362104, 0.02061107465261834484, 0.02143551763872306518, 0.02308440361093250931, 0.02473328958314195691, 0.02638217555535139758 ),
 .UNSPECIFIED. ) ;
#58893=CARTESIAN_POINT ( 'NONE',  ( -37.79601571721867259, 10.72155118426296738, 68.54850928335817173 ) ) ;
#58894=CARTESIAN_POINT ( 'NONE',  ( 198.8752826725510658, 100.3130050945023299, 58.81793774317634416 ) ) ;
#58898=CARTESIAN_POINT ( 'NONE',  ( -154.7998111145352311, 68.80117179139327277, 59.72958456622436785 ) ) ;
#58899=CARTESIAN_POINT ( 'NONE',  ( 22.89270809252618832, 7.840160460323052583, 13.08620663423853436 ) ) ;
#58900=DIRECTION ( 'NONE',  ( -0.000000000000000000, 1.000000000000000000, -0.000000000000000000 ) ) ;
#58901=CARTESIAN_POINT ( 'NONE',  ( -85.46258339457291697, 25.02772366257408621, -45.79754920329482815 ) ) ;
#58903=CARTESIAN_POINT ( 'NONE',  ( 22.80839748737788142, 6.826915557457463812, 61.70818393205063046 ) ) ;
#58906=CARTESIAN_POINT ( 'NONE',  ( 14.80291736570134731, 7.477373894757625372, 18.12158280542935884 ) ) ;
#58909=ADVANCED_FACE ( 'NONE', ( #22636 ), #44795, .F. ) ;
#58911=ORIENTED_EDGE ( 'NONE', *, *, #52494, .T. ) ;
#58914=CARTESIAN_POINT ( 'NONE',  ( -132.0958200534847435, 50.71531800824803327, -46.63840928461922886 ) ) ;
#58915=CARTESIAN_POINT ( 'NONE',  ( -102.7447593990059289, 34.14748189312172144, -50.01457726497595502 ) ) ;
#58916=CARTESIAN_POINT ( 'NONE',  ( 55.91133443650745960, 12.16263767238152127, -72.51936885403362965 ) ) ;
#58919=CARTESIAN_POINT ( 'NONE',  ( -24.18258876560172865, 8.512344710720677554, -17.93097106050854705 ) ) ;
#58920=CARTESIAN_POINT ( 'NONE',  ( 174.6808034781869878, 72.36770494831971234, 86.57635966052535537 ) ) ;
#58923=CARTESIAN_POINT ( 'NONE',  ( 110.7164744784863899, 29.10110206241301967, 71.45576479620105204 ) ) ;
#58925=CARTESIAN_POINT ( 'NONE',  ( 130.7260570116704343, 40.73146260246713268, -63.53671823496143389 ) ) ;
#58930=CARTESIAN_POINT ( 'NONE',  ( 163.5277822717018523, 62.51852278986679323, -92.88600173900509560 ) ) ;
#58936=CARTESIAN_POINT ( 'NONE',  ( -121.1775535805057444, 43.46577565517550568, -9.717201679529251734 ) ) ;
#58939=CARTESIAN_POINT ( 'NONE',  ( -178.2427210808089626, 93.01567669683339545, -20.85170211881552760 ) ) ;
#58940=CARTESIAN_POINT ( 'NONE',  ( -165.7713056973201446, 80.74264649718244868, -67.53382473510175998 ) ) ;
#58942=CARTESIAN_POINT ( 'NONE',  ( -142.9728934044262019, 58.82891228489262403, -46.03245465095029232 ) ) ;
#58943=ORIENTED_EDGE ( 'NONE', *, *, #18055, .T. ) ;
#58948=DIRECTION ( 'NONE',  ( 0.000000000000000000, 0.000000000000000000, 1.000000000000000000 ) ) ;
#58949=FACE_OUTER_BOUND ( 'NONE', #67423, .T. ) ;
#58952=LINE ( 'NONE', #11810, #38796 ) ;
#58953=CARTESIAN_POINT ( 'NONE',  ( -127.6881387055492922, 48.89937523111243678, -76.54403142618212996 ) ) ;
#58957=CARTESIAN_POINT ( 'NONE',  ( -149.5074843970971301, 64.17983161892347255, -88.50193171241930656 ) ) ;
#58959=EDGE_LOOP ( 'NONE', ( #12751, #52963 ) ) ;
#58960=CARTESIAN_POINT ( 'NONE',  ( 184.3941060377212295, 82.01604625189466446, -77.31420240063759763 ) ) ;
#58962=CARTESIAN_POINT ( 'NONE',  ( -165.9111709580270997, 79.44576090485632847, -40.12534605873958071 ) ) ;
#58965=CARTESIAN_POINT ( 'NONE',  ( 103.8055367708241192, 27.11070767929350112, -66.38655192125422388 ) ) ;
#58966=CARTESIAN_POINT ( 'NONE',  ( -77.71801202538873099, 23.03755222122951452, -62.00518611626486631 ) ) ;
#58968=CARTESIAN_POINT ( 'NONE',  ( -124.9970785861867739, 47.10847819093958577, 30.67033377869767818 ) ) ;
#58969=CARTESIAN_POINT ( 'NONE',  ( 212.1983751099433846, 117.2326047784727336, 63.69360226375801659 ) ) ;
#58972=CARTESIAN_POINT ( 'NONE',  ( -109.3432140528234839, 36.51591785955882585, -13.09559261180481116 ) ) ;
#58975=EDGE_CURVE ( 'NONE', #14285, #42689, #50923, .T. ) ;
#58977=CARTESIAN_POINT ( 'NONE',  ( -84.88037603621106086, 24.78657832303205666, -92.09904858809437656 ) ) ;
#58978=CARTESIAN_POINT ( 'NONE',  ( 150.2076397309211586, 52.21780102759852582, -18.67121458051684613 ) ) ;
#58983=CARTESIAN_POINT ( 'NONE',  ( 206.0202013761258115, 108.1716492322431264, 82.99495773477644889 ) ) ;
#58987=CARTESIAN_POINT ( 'NONE',  ( 12.91653440534542341, 7.431946726541410975, -76.80479733579223023 ) ) ;
#58990=ADVANCED_FACE ( 'NONE', ( #51114 ), #3273, .F. ) ;
#58991=CARTESIAN_POINT ( 'NONE',  ( -2.874437057892791803, 6.618922960888052209, 31.96075603522317010 ) ) ;
#58993=CARTESIAN_POINT ( 'NONE',  ( 87.94810462138822515, 20.94053779377377822, 83.51093339085589662 ) ) ;
#58999=CARTESIAN_POINT ( 'NONE',  ( -132.0958200534847435, 50.71531800824803327, 7.050691896308118878 ) ) ;
#59000=CARTESIAN_POINT ( 'NONE',  ( -108.6944271866238978, 37.30738480893074893, 68.78232788442275591 ) ) ;
#59001=CARTESIAN_POINT ( 'NONE',  ( -180.6134399488801705, 95.87473607775544338, 91.62122452033388242 ) ) ;
#59005=VECTOR ( 'NONE', #36100, 1000.000000000000000 ) ;
#59006=CARTESIAN_POINT ( 'NONE',  ( 94.11746922806584337, 22.11341285603780804, 64.54865186196720117 ) ) ;
#59008=CARTESIAN_POINT ( 'NONE',  ( 198.4045886930829283, 99.71425793793710568, -21.07018120517999549 ) ) ;
#59010=CARTESIAN_POINT ( 'NONE',  ( -156.9834569011572682, 70.78920417036412971, 91.28448318999808464 ) ) ;
#59012=CARTESIAN_POINT ( 'NONE',  ( 140.8984307802396643, 45.84194788389002895, 34.37783282223308134 ) ) ;
#59015=CARTESIAN_POINT ( 'NONE',  ( 81.57915404881515542, 18.81499384983929701, 4.817277352176767558 ) ) ;
#59019=EDGE_CURVE ( 'NONE', #61067, #25434, #35969, .T. ) ;
#59022=CARTESIAN_POINT ( 'NONE',  ( -74.19961951691010427, 20.67022044985853313, -21.80058496222482134 ) ) ;
#59023=CARTESIAN_POINT ( 'NONE',  ( 67.55134213333079174, 13.77030723107741395, -76.05851458524612951 ) ) ;
#59024=CARTESIAN_POINT ( 'NONE',  ( -61.51762070241280611, 16.51067482779403406, 41.62754106045760949 ) ) ;
#59027=CARTESIAN_POINT ( 'NONE',  ( 163.1265310614427619, 62.18610413911356005, 31.97814890642583663 ) ) ;
#59029=DIRECTION ( 'NONE',  ( 0.000000000000000000, 0.000000000000000000, 1.000000000000000000 ) ) ;
#59031=CARTESIAN_POINT ( 'NONE',  ( -145.6181732888550471, 62.24768171590013566, -89.57533543414972144 ) ) ;
#59033=CARTESIAN_POINT ( 'NONE',  ( -179.8926034784146282, 96.58272071140105197, 35.08552098014282450 ) ) ;
#59034=CARTESIAN_POINT ( 'NONE',  ( 126.4219470349615904, 38.26519385429185149, 64.87749366262461592 ) ) ;
#59038=EDGE_LOOP ( 'NONE', ( #49073, #8391, #9852, #33191 ) ) ;
#59040=CARTESIAN_POINT ( 'NONE',  ( -104.5740066103012680, 35.09687312794774527, 4.030067934921061301 ) ) ;
#59047=CARTESIAN_POINT ( 'NONE',  ( 110.2429982417149432, 28.88204397445228722, 71.45576479620103783 ) ) ;
#59048=AXIS2_PLACEMENT_3D ( 'NONE', #2911, #66947, #9225 ) ;
#59054=EDGE_CURVE ( 'NONE', #42011, #15039, #60131, .T. ) ;
#59056=CARTESIAN_POINT ( 'NONE',  ( -78.66644367742109978, 23.39876645725289706, 57.26275173013680586 ) ) ;
#59057=CARTESIAN_POINT ( 'NONE',  ( 188.5843222076478014, 86.53342480589844854, 37.10520038439885582 ) ) ;
#59059=CARTESIAN_POINT ( 'NONE',  ( -74.79002408692177539, 20.88280597089420709, 17.49881191264313429 ) ) ;
#59062=CARTESIAN_POINT ( 'NONE',  ( 22.15943197741200876, 7.796127622097904997, 33.55009939024217402 ) ) ;
#59064=CARTESIAN_POINT ( 'NONE',  ( 162.7963212667073378, 63.21900188423069977, -65.18246456083083729 ) ) ;
#59065=VERTEX_POINT ( 'NONE', #52488 ) ;
#59066=DIRECTION ( 'NONE',  ( 0.000000000000000000, 0.000000000000000000, 1.000000000000000000 ) ) ;
#59070=CARTESIAN_POINT ( 'NONE',  ( -29.04400972079232446, 10.22852224114065223, -62.55024186826118893 ) ) ;
#59071=CARTESIAN_POINT ( 'NONE',  ( -190.6985136298601731, 109.1272424661242582, -95.00000000000133582 ) ) ;
#59076=ORIENTED_EDGE ( 'NONE', *, *, #35155, .T. ) ;
#59077=CARTESIAN_POINT ( 'NONE',  ( -131.6399667378751133, 51.62465701391629125, 42.96608471902324311 ) ) ;
#59079=CARTESIAN_POINT ( 'NONE',  ( 181.0840389613909736, 78.60582251573002566, 17.46404351504774510 ) ) ;
#59080=CARTESIAN_POINT ( 'NONE',  ( 182.8317132966081999, 81.83833949797246987, -90.11192720193595562 ) ) ;
#59081=CARTESIAN_POINT ( 'NONE',  ( 60.62939143133407072, 12.13148391928981162, 57.03056178573838508 ) ) ;
#59086=AXIS2_PLACEMENT_3D ( 'NONE', #13394, #34856, #60534 ) ;
#59087=CARTESIAN_POINT ( 'NONE',  ( 86.62931800182293784, 20.48449268398422163, -62.66611478937537782 ) ) ;
#59094=CARTESIAN_POINT ( 'NONE',  ( 70.46452034227868921, 14.52462608639673469, 36.30783829542910013 ) ) ;
#59095=CARTESIAN_POINT ( 'NONE',  ( 9.319975126229035567, 7.386007236262731368, 94.99999999999866418 ) ) ;
#59101=CARTESIAN_POINT ( 'NONE',  ( 86.62931800182293784, 19.42108912189599934, 17.86753698201564688 ) ) ;
#59102=ORIENTED_EDGE ( 'NONE', *, *, #66240, .F. ) ;
#59103=CARTESIAN_POINT ( 'NONE',  ( 15.78827728214693416, -170.0000000000000000, -8.674393508222099314 ) ) ;
#59104=ORIENTED_EDGE ( 'NONE', *, *, #53019, .T. ) ;
#59109=CARTESIAN_POINT ( 'NONE',  ( 129.6961120139403647, 38.96846414226717314, 57.61019598173326273 ) ) ;
#59111=CARTESIAN_POINT ( 'NONE',  ( 153.2384531768735769, 54.43344429203622781, 43.11883740112016739 ) ) ;
#59112=CARTESIAN_POINT ( 'NONE',  ( 64.93224207568367490, 14.16036304753835040, 44.56800710844814972 ) ) ;
#59113=LINE ( 'NONE', #13046, #15688 ) ;
#59116=CARTESIAN_POINT ( 'NONE',  ( -23.99924996210628336, 8.487987924059021694, 38.69610266098428042 ) ) ;
#59117=CARTESIAN_POINT ( 'NONE',  ( -145.9181947914994169, 62.49417193455352759, -62.56801270397023274 ) ) ;
#59118=EDGE_LOOP ( 'NONE', ( #17214, #16446 ) ) ;
#59119=FACE_BOUND ( 'NONE', #9203, .T. ) ;
#59121=CARTESIAN_POINT ( 'NONE',  ( -173.1211646369891355, 88.63826465341152527, 72.66624519710475738 ) ) ;
#59123=CARTESIAN_POINT ( 'NONE',  ( -120.1650841064594033, 44.02024060322521848, -37.56662740794514832 ) ) ;
#59124=CARTESIAN_POINT ( 'NONE',  ( -83.15209219203885027, 25.16621997697721014, 17.10401920708160262 ) ) ;
#59129=CARTESIAN_POINT ( 'NONE',  ( 63.98971758354223027, 12.90030016320050699, 17.92090471930345430 ) ) ;
#59130=CARTESIAN_POINT ( 'NONE',  ( -86.06525741550315445, 26.37048289224654241, 66.01641903232457764 ) ) ;
#59131=CARTESIAN_POINT ( 'NONE',  ( 40.23250010525561748, 9.533837034108117336, -89.34369780650632720 ) ) ;
#59133=AXIS2_PLACEMENT_3D ( 'NONE', #24904, #46001, #66789 ) ;
#59134=CARTESIAN_POINT ( 'NONE',  ( -34.06637338149494809, 11.05895377318622863, 3.842940194179071067 ) ) ;
#59138=CARTESIAN_POINT ( 'NONE',  ( 18.20314211955701822, 7.596739727129573794, -76.98109712673615945 ) ) ;
#59141=CARTESIAN_POINT ( 'NONE',  ( -142.8492950481059154, 60.01492924994603584, 61.60267790966557300 ) ) ;
#59143=CARTESIAN_POINT ( 'NONE',  ( 70.38121440378670002, 14.50253793787158862, -14.89899490779335522 ) ) ;
#59144=CARTESIAN_POINT ( 'NONE',  ( -24.03640295269301319, 9.507963273819775907, -44.04650067501650312 ) ) ;
#59147=AXIS2_PLACEMENT_3D ( 'NONE', #44120, #11776, #60666 ) ;
#59148=CARTESIAN_POINT ( 'NONE',  ( -74.27277138815051671, 21.76582788880764596, -90.22237058240676788 ) ) ;
#59149=CYLINDRICAL_SURFACE ( 'NONE', #67835, 7.500000000000020428 ) ;
#59153=CARTESIAN_POINT ( 'NONE',  ( -166.0012244511291613, 80.97916541034754800, 62.79134880957640519 ) ) ;
#59156=EDGE_CURVE ( 'NONE', #52761, #56686, #20627, .T. ) ;
#59158=CARTESIAN_POINT ( 'NONE',  ( 92.91022130985207639, 21.66059330820416307, 94.99999999999866418 ) ) ;
#59161=CARTESIAN_POINT ( 'NONE',  ( 187.2384682876462136, 86.54721710842896698, -12.56464666103593153 ) ) ;
#59162=CARTESIAN_POINT ( 'NONE',  ( -83.51052366780672287, 24.22613130369188283, -10.03992714516486906 ) ) ;
#59164=CARTESIAN_POINT ( 'NONE',  ( 41.33692564073609077, 8.668977654195479943, -23.52549198662623908 ) ) ;
#59166=CARTESIAN_POINT ( 'NONE',  ( -102.2801239173131194, -170.0000000000000000, 91.70817568734248937 ) ) ;
#59167=CARTESIAN_POINT ( 'NONE',  ( 163.7403496014744064, 64.00600007368872468, 59.63034611569458576 ) ) ;
#59172=CARTESIAN_POINT ( 'NONE',  ( -49.44484229820456278, 14.28460989390478986, 69.66605993095367921 ) ) ;
#59175=CARTESIAN_POINT ( 'NONE',  ( -14.67600935270417928, 8.444777994442205227, 94.42750418574264870 ) ) ;
#59176=ORIENTED_EDGE ( 'NONE', *, *, #52014, .T. ) ;
#59177=DIRECTION ( 'NONE',  ( -0.000000000000000000, 1.000000000000000000, -0.000000000000000000 ) ) ;
#59179=AXIS2_PLACEMENT_3D ( 'NONE', #12714, #49990, #12362 ) ;
#59180=ORIENTED_EDGE ( 'NONE', *, *, #54538, .T. ) ;
#59181=CARTESIAN_POINT ( 'NONE',  ( 35.35682721709835619, 8.930334680552826754, 84.77865436726582971 ) ) ;
#59183=CARTESIAN_POINT ( 'NONE',  ( 92.52113039222224700, 22.58921125235802663, -65.49921141967747928 ) ) ;
#59186=CARTESIAN_POINT ( 'NONE',  ( -59.36813706141739999, 15.88103696331963377, -63.42195766872510632 ) ) ;
#59187=CARTESIAN_POINT ( 'NONE',  ( 38.42384008295177722, 8.283891555743467805, -8.823408633594510775 ) ) ;
#59190=CARTESIAN_POINT ( 'NONE',  ( -152.4930836497867688, 68.09400557494207362, -76.04119844780879589 ) ) ;
#59191=CARTESIAN_POINT ( 'NONE',  ( 94.12988949694081953, 22.11811104795076233, 37.44777776544177073 ) ) ;
#59192=B_SPLINE_CURVE_WITH_KNOTS ( 'NONE', 3,
 ( #4016, #14566, #41644, #20876, #4363, #41306, #69048, #58168, #31777, #37054, #21227, #68046, #46923, #42334, #47938, #31436, #32125, #30750, #63450, #10657 ),
 .UNSPECIFIED., .F., .F.,
 ( 4, 2, 2, 2, 2, 2, 2, 2, 2, 4 ),
 ( 0.01042392800800004925, 0.01174416055531339598, 0.01306439310262674097, 0.01372450937628338051, 0.01438462564994002005, 0.01570485819725330606, 0.01702509074456659555, 0.01834532329187988503, 0.01966555583919317451, 0.02098578838650646053 ),
 .UNSPECIFIED. ) ;
#59196=CARTESIAN_POINT ( 'NONE',  ( -48.70883077256304716, 14.10659259062419224, -46.72446105713036246 ) ) ;
#59197=EDGE_CURVE ( 'NONE', #49097, #32365, #15660, .T. ) ;
#59200=CARTESIAN_POINT ( 'NONE',  ( 10.13563904803030979, 7.391572367417532874, 42.46823125868149873 ) ) ;
#59202=CARTESIAN_POINT ( 'NONE',  ( -85.89736547126425137, 26.29987632947471354, 89.59003780420152907 ) ) ;
#59203=FACE_OUTER_BOUND ( 'NONE', #54062, .T. ) ;
#59205=VERTEX_POINT ( 'NONE', #18322 ) ;
#59207=CARTESIAN_POINT ( 'NONE',  ( -15.27748264047828997, 7.491388194171917370, -15.09317646226059217 ) ) ;
#59208=CARTESIAN_POINT ( 'NONE',  ( -168.6270250298198903, 83.72687254638921672, 85.99976982588017904 ) ) ;
#59212=CARTESIAN_POINT ( 'NONE',  ( -33.85171821065139142, 11.02091558840051455, 71.67896086471448314 ) ) ;
#59214=CARTESIAN_POINT ( 'NONE',  ( -14.84903512415884919, 8.461292896365062433, -13.43169028553783839 ) ) ;
#59215=CARTESIAN_POINT ( 'NONE',  ( -78.66644367742109978, 22.32174330031319442, 3.573650549209446137 ) ) ;
#59216=CARTESIAN_POINT ( 'NONE',  ( 22.52576749827964875, 6.809805260274348626, -19.50566305713887161 ) ) ;
#59217=VERTEX_POINT ( 'NONE', #46089 ) ;
#59218=CARTESIAN_POINT ( 'NONE',  ( 15.78827728214693416, -170.0000000000000000, 37.51470767270523510 ) ) ;
#59221=CARTESIAN_POINT ( 'NONE',  ( 67.93154431625912082, 14.90489441944786897, -22.06196858991532039 ) ) ;
#59222=B_SPLINE_CURVE_WITH_KNOTS ( 'NONE', 3,
 ( #38774, #43329, #11323, #48591, #59164, #5016, #69384, #42980, #10631, #16261, #59856, #58820, #54583, #65153, #60218, #64806, #38410, #59507, #785, #54223, #32792, #6046, #37363, #21534, #27505, #26824, #21205, #12036, #10982, #1134, #64452, #16947, #22585, #32104, #42652, #22238, #11676, #53878, #26483, #33147, #48251, #6408, #27858, #49301, #65504 ),
 .UNSPECIFIED., .F., .F.,
 ( 4, 2, 2, 2, 2, 2, 2, 2, 2, 2, 2, 2, 2, 1, 2, 2, 2, 2, 2, 2, 2, 2, 4 ),
 ( 0.02352719711393055219, 0.02499986300757014307, 0.02573619595438995239, 0.02647252890120975824, 0.02794519479484937341, 0.02941786068848898511, 0.03015419363530879443, 0.03089052658212860722, 0.03236319247576821545, 0.03309952542258803171, 0.03383585836940784103, 0.03530852426304745273, 0.03604485720986726205, 0.03678119015668707831, 0.03751752310350688763, 0.03825385605032669695, 0.03972652194396632253, 0.04119918783760595504, 0.04267185373124557368, 0.04340818667806538300, 0.04414451962488518538, 0.04561718551852481096, 0.04708985141216442960 ),
 .UNSPECIFIED. ) ;
#59224=FACE_OUTER_BOUND ( 'NONE', #63198, .T. ) ;
#59225=EDGE_CURVE ( 'NONE', #46532, #36510, #56784, .T. ) ;
#59226=CARTESIAN_POINT ( 'NONE',  ( -155.5977325361977819, 70.88311713755697951, 15.76059677166101380 ) ) ;
#59228=CARTESIAN_POINT ( 'NONE',  ( 188.4937788906148910, 86.43336847120863808, -42.52624257897028315 ) ) ;
#59229=CARTESIAN_POINT ( 'NONE',  ( 21.75684465274325419, 6.764994602232769161, 42.08264190274187655 ) ) ;
#59230=CARTESIAN_POINT ( 'NONE',  ( -148.5419150567446991, 64.67935585776004359, 84.45219532842064325 ) ) ;
#59235=CARTESIAN_POINT ( 'NONE',  ( 31.91383250562745388, 8.564461488297009595, -42.63145424299220565 ) ) ;
#59240=CARTESIAN_POINT ( 'NONE',  ( -151.6716822472524200, 66.03661194063734285, -22.66300283947714789 ) ) ;
#59246=CARTESIAN_POINT ( 'NONE',  ( -152.5067928559255392, 66.76529500553621688, 58.17683507072492688 ) ) ;
#59248=CARTESIAN_POINT ( 'NONE',  ( -1.862553927312063262, 7.582910205528080816, -47.49339086204825833 ) ) ;
#59249=CARTESIAN_POINT ( 'NONE',  ( 103.9652201950894579, 26.08439499369982428, 14.37774731416467411 ) ) ;
#59254=CARTESIAN_POINT ( 'NONE',  ( 9.058156535714477542, 6.378495712187263855, -73.18255775613405945 ) ) ;
#59259=CARTESIAN_POINT ( 'NONE',  ( 132.9453095272139649, 42.04754713161462831, -36.02331093239565973 ) ) ;
#59260=CARTESIAN_POINT ( 'NONE',  ( -129.4098618459772183, 48.85263848239745244, -49.04253402992481625 ) ) ;
#59262=CARTESIAN_POINT ( 'NONE',  ( 55.77012379229940819, 12.13428856597100669, -68.11229150268280819 ) ) ;
#59266=CARTESIAN_POINT ( 'NONE',  ( 197.1975259970231775, 98.19639476549652102, 10.18970865138460624 ) ) ;
#59270=ORIENTED_EDGE ( 'NONE', *, *, #17637, .F. ) ;
#59271=CARTESIAN_POINT ( 'NONE',  ( 133.8566784816069060, 42.60093787723654657, -62.86786152285933582 ) ) ;
#59273=CARTESIAN_POINT ( 'NONE',  ( 141.0517870458593848, 47.14452711594498879, 65.98772666960701372 ) ) ;
#59275=CARTESIAN_POINT ( 'NONE',  ( -97.85576954355163082, 30.58918648956191788, 44.09425425760385053 ) ) ;
#59276=CARTESIAN_POINT ( 'NONE',  ( 91.67571176799447130, 21.20498955963031307, -48.87521057456431350 ) ) ;
#59279=VERTEX_POINT ( 'NONE', #11875 ) ;
#59283=EDGE_CURVE ( 'NONE', #32318, #28360, #22433, .T. ) ;
#59284=DIRECTION ( 'NONE',  ( 0.000000000000000000, 0.000000000000000000, 1.000000000000000000 ) ) ;
#59289=CARTESIAN_POINT ( 'NONE',  ( -125.8938041572051389, 47.69968343338781125, 72.46449846362081360 ) ) ;
#59291=CARTESIAN_POINT ( 'NONE',  ( 55.99998955208977236, 12.18058389017405041, 13.13159707503299956 ) ) ;
#59292=AXIS2_PLACEMENT_3D ( 'NONE', #22017, #11444, #27984 ) ;
#59294=CARTESIAN_POINT ( 'NONE',  ( -142.2626321327577443, 58.26997216742665131, 63.10616936434193747 ) ) ;
#59298=EDGE_CURVE ( 'NONE', #29569, #5706, #18156, .T. ) ;
#59300=CARTESIAN_POINT ( 'NONE',  ( 136.1081004736420255, 42.80058051492066085, -23.83655509551084961 ) ) ;
#59302=CARTESIAN_POINT ( 'NONE',  ( -102.2801239173131052, 32.78103895658057354, -50.01457726497594081 ) ) ;
#59303=CARTESIAN_POINT ( 'NONE',  ( 197.8572563162090603, 97.41072138832258531, 12.95325563156990789 ) ) ;
#59304=CARTESIAN_POINT ( 'NONE',  ( -96.00016893459647349, 29.70347032303887858, 15.28240503082096069 ) ) ;
#59308=EDGE_CURVE ( 'NONE', #63135, #23015, #4685, .T. ) ;
#59309=CARTESIAN_POINT ( 'NONE',  ( 188.2950202724320548, 86.21411212788221690, -72.65244717427873411 ) ) ;
#59310=CARTESIAN_POINT ( 'NONE',  ( 110.2429982417149574, 29.99119854320843714, 44.61121420573733332 ) ) ;
#59314=CARTESIAN_POINT ( 'NONE',  ( 109.7732660198864494, 29.77277639096406148, -62.76698815611734972 ) ) ;
#59315=CARTESIAN_POINT ( 'NONE',  ( 82.13067365723604496, 17.93447087949267527, 31.19152029446487617 ) ) ;
#59317=CARTESIAN_POINT ( 'NONE',  ( -119.9771613955296772, 43.90337778233485722, 33.50398703533743117 ) ) ;
#59319=B_SPLINE_CURVE_WITH_KNOTS ( 'NONE', 3,
 ( #46723, #22062, #22410, #38236, #27678, #16443, #65684, #26988, #5534, #43850, #26652, #54400, #27328, #21364, #48087, #37897, #250, #59677, #64629, #37543, #6583, #6223, #32963, #49120, #49471, #11849, #58993, #33329, #48768, #44197, #53712, #17471, #959, #43157, #59343, #65327, #17113, #11154, #38590, #16087, #32619, #5197, #1306, #10462, #64982, #60032, #69546, #31934, #54047, #48417, #53361, #605, #42811, #43504, #16777, #64279, #10813, #32281 ),
 .UNSPECIFIED., .F., .F.,
 ( 4, 2, 2, 2, 2, 2, 2, 2, 2, 2, 2, 2, 2, 2, 2, 2, 2, 2, 2, 2, 2, 2, 2, 2, 2, 2, 2, 2, 4 ),
 ( 0.000000000000000000, 0.002051743101817396931, 0.003077614652726094312, 0.004103486203634792127, 0.005129357754543489509, 0.006155229305452186890, 0.007181100856360885139, 0.008206972407269582520, 0.009232843958178280769, 0.01025871550908697902, 0.01128458705999567727, 0.01231045861090437551, 0.01436220171272178416, 0.01538807326363049455, 0.01641394481453920320, 0.01743981636544791186, 0.01846568791635662052, 0.01949155946726532918, 0.02051743101817404130, 0.02256917411999149331, 0.02359504567090022278, 0.02462091722180894879, 0.02564678877271767479, 0.02667266032362640427, 0.02769853187453513027, 0.02872440342544385627, 0.02975027497635258922, 0.03077614652726131522, 0.03282788962907880193 ),
 .UNSPECIFIED. ) ;
#59320=VERTEX_POINT ( 'NONE', #42120 ) ;
#59321=CARTESIAN_POINT ( 'NONE',  ( -24.95029760921699946, 9.631514785009935409, 7.102706412057313123 ) ) ;
#59322=ORIENTED_EDGE ( 'NONE', *, *, #50831, .F. ) ;
#59323=CARTESIAN_POINT ( 'NONE',  ( -14.66033866466834645, 7.432913330382390882, -46.01550798236979034 ) ) ;
#59324=LINE ( 'NONE', #11137, #20597 ) ;
#59325=CARTESIAN_POINT ( 'NONE',  ( 152.6560521232695464, 54.00248515670894278, -22.53561542425598319 ) ) ;
#59326=CARTESIAN_POINT ( 'NONE',  ( 36.98541457540712685, 9.120571655722418569, 17.68600818565902699 ) ) ;
#59327=CARTESIAN_POINT ( 'NONE',  ( -97.48179118242302366, 31.52606332398821820, -75.14452323989597460 ) ) ;
#59328=CARTESIAN_POINT ( 'NONE',  ( 112.1664364330408432, 30.89547116421898565, -89.85190045744435849 ) ) ;
#59330=EDGE_CURVE ( 'NONE', #67718, #31575, #24015, .T. ) ;
#59332=CARTESIAN_POINT ( 'NONE',  ( 212.2009967487813356, 117.2366405038844022, 90.35305982578324802 ) ) ;
#59334=VERTEX_POINT ( 'NONE', #44895 ) ;
#59335=CARTESIAN_POINT ( 'NONE',  ( 56.94505604581135572, 12.37336791557970983, 59.74625065850809591 ) ) ;
#59336=CARTESIAN_POINT ( 'NONE',  ( 15.78827728214693771, 7.507518794609575608, -62.36349468914946925 ) ) ;
#59337=CARTESIAN_POINT ( 'NONE',  ( -29.02794087136070189, 9.207646203414336483, 17.99040909154227919 ) ) ;
#59338=ADVANCED_FACE ( 'NONE', ( #66378 ), #65312, .F. ) ;
#59339=DIRECTION ( 'NONE',  ( -0.000000000000000000, 1.000000000000000000, -0.000000000000000000 ) ) ;
#59340=CARTESIAN_POINT ( 'NONE',  ( -0.3734056954813049778, 6.520221844775925923, 38.59366696979675027 ) ) ;
#59341=CARTESIAN_POINT ( 'NONE',  ( -102.2801239173131052, 32.78103895658057354, -61.85912785543958847 ) ) ;
#59342=VECTOR ( 'NONE', #57644, 1000.000000000000000 ) ;
#59343=CARTESIAN_POINT ( 'NONE',  ( 84.10229504626889252, 19.63355683306561872, 83.83215316015663632 ) ) ;
#59345=ORIENTED_EDGE ( 'NONE', *, *, #68084, .F. ) ;
#59348=CARTESIAN_POINT ( 'NONE',  ( -129.4098618459771899, 48.85263848239743822, 4.646567151002527929 ) ) ;
#59349=CARTESIAN_POINT ( 'NONE',  ( -166.0031475600389115, 80.98114714564766814, -39.83147878504032491 ) ) ;
#59352=EDGE_LOOP ( 'NONE', ( #31017, #36870, #22844, #20019 ) ) ;
#59354=DIRECTION ( 'NONE',  ( -0.000000000000000000, 1.000000000000000000, -0.000000000000000000 ) ) ;
#59355=CARTESIAN_POINT ( 'NONE',  ( 199.7291770695759965, 101.4092159658446803, -11.35800590186485515 ) ) ;
#59356=CARTESIAN_POINT ( 'NONE',  ( -156.2685900000522849, 70.13315996971763866, 88.64677459970704376 ) ) ;
#59357=CARTESIAN_POINT ( 'NONE',  ( 133.8566784816069628, 41.42467568809806977, 44.51034083899536142 ) ) ;
#59360=CARTESIAN_POINT ( 'NONE',  ( 83.59652366361572717, 19.46709838196857234, 17.23118984585019575 ) ) ;
#59361=CARTESIAN_POINT ( 'NONE',  ( 164.9700808964341547, 65.04346068891115351, 10.35365659087820056 ) ) ;
#59363=ORIENTED_EDGE ( 'NONE', *, *, #36825, .T. ) ;
#59366=( BOUNDED_CURVE ( )  B_SPLINE_CURVE ( 3, ( #12283, #23193, #11930, #33402 ),
 .UNSPECIFIED., .F., .F. ) 
 B_SPLINE_CURVE_WITH_KNOTS ( ( 4, 4 ),
 ( 2.746264796135519770, 3.776976132411494103 ),
 .UNSPECIFIED. ) 
 CURVE ( )  GEOMETRIC_REPRESENTATION_ITEM ( )  RATIONAL_B_SPLINE_CURVE ( ( 1.000000000000000000, 0.9134116588687805072, 0.9134116588687805072, 1.000000000000000000 ) ) 
 REPRESENTATION_ITEM ( '' )  );
#59367=CARTESIAN_POINT ( 'NONE',  ( -118.9981077023450666, 42.11809457178108573, -93.14365615247058372 ) ) ;
#59369=B_SPLINE_CURVE_WITH_KNOTS ( 'NONE', 3,
 ( #61668, #39524, #3283, #18413, #12798, #35288, #34947, #45840, #56390, #2248, #14179, #39867, #18765, #30357, #24741, #40908, #67650, #19446, #23695, #66618, #45486, #29660, #56744, #61325, #13486, #51121, #57092, #2934, #8562, #7867, #30013, #62364, #24398, #13150, #8905, #51472, #51809, #67316, #19101, #18074, #40555, #60973, #56049, #3617, #66282, #62008, #50428, #34256 ),
 .UNSPECIFIED., .F., .F.,
 ( 4, 2, 2, 2, 2, 2, 2, 2, 2, 2, 2, 2, 2, 2, 2, 2, 2, 2, 2, 2, 2, 2, 2, 4 ),
 ( 1.387778780781445676E-17, 0.003619254076116648709, 0.004524067595145762205, 0.005428881114174875268, 0.007238508152233127414, 0.008143321671262276906, 0.009048135190291429000, 0.01085776222834966380, 0.01176257574737874824, 0.01266738926640783268, 0.01357220278543691885, 0.01447701630446600329, 0.01538182982349508947, 0.01628664334252417217, 0.01719145686155325661, 0.01809627038058234452, 0.01900108389961142549, 0.01990589741864050993, 0.02171552445669866147, 0.02262033797572774937, 0.02352515149475683728, 0.02533477853281501657, 0.02714440557087319586, 0.02895403260893137515 ),
 .UNSPECIFIED. ) ;
#59372=EDGE_LOOP ( 'NONE', ( #29525, #36225 ) ) ;
#59373=CARTESIAN_POINT ( 'NONE',  ( 160.4963793545269652, 60.04225845346908130, 30.03251751463668029 ) ) ;
#59375=CYLINDRICAL_SURFACE ( 'NONE', #38428, 7.500000000000020428 ) ;
#59377=CARTESIAN_POINT ( 'NONE',  ( -149.5074843970971017, 65.50121172469320641, -88.50193171241930656 ) ) ;
#59379=CARTESIAN_POINT ( 'NONE',  ( -37.38781680082738035, 10.64362327909142358, -20.56642074805881748 ) ) ;
#59380=CARTESIAN_POINT ( 'NONE',  ( -180.6158171975814923, 97.47361786002629458, 37.99731989376397223 ) ) ;
#59381=CARTESIAN_POINT ( 'NONE',  ( -38.93922791710217979, 10.94334660650242341, -69.90365907529749734 ) ) ;
#59391=DIRECTION ( 'NONE',  ( -0.000000000000000000, 1.000000000000000000, -0.000000000000000000 ) ) ;
#59393=CARTESIAN_POINT ( 'NONE',  ( -7.825402957745083654, 7.899365992529244984, -8.573520141480125645 ) ) ;
#59394=CARTESIAN_POINT ( 'NONE',  ( 66.21839516550542726, 13.43774118063817546, 84.18802111937300481 ) ) ;
#59402=CARTESIAN_POINT ( 'NONE',  ( 205.1049299651095623, 106.9023875785546096, -63.17048162308526571 ) ) ;
#59406=CARTESIAN_POINT ( 'NONE',  ( -78.66644367742111399, -170.0000000000000000, -42.61545063171789849 ) ) ;
#59407=CARTESIAN_POINT ( 'NONE',  ( 199.2433808803260717, 99.15270001483533235, 85.23814155805331438 ) ) ;
#59408=CARTESIAN_POINT ( 'NONE',  ( 150.7926588734435711, 52.63999027731880886, -40.19948293293975183 ) ) ;
#59409=CARTESIAN_POINT ( 'NONE',  ( 163.1313205310724754, 63.49733392291055623, -65.54288040409811344 ) ) ;
#59411=CARTESIAN_POINT ( 'NONE',  ( -149.5074843970971301, 64.17983161892347255, -88.50193171241930656 ) ) ;
#59416=CARTESIAN_POINT ( 'NONE',  ( -79.61931371420118353, 22.68640080971622197, 45.37248484975646079 ) ) ;
#59417=CARTESIAN_POINT ( 'NONE',  ( -24.18270484670773968, 9.527492911955594224, -67.70162071242002355 ) ) ;
#59418=CARTESIAN_POINT ( 'NONE',  ( 39.40195752203892710, 9.424259417798134919, 29.91383430596324899 ) ) ;
#59419=CARTESIAN_POINT ( 'NONE',  ( -24.18258876560172865, 8.512344710720679331, 62.60268071088248831 ) ) ;
#59425=ORIENTED_EDGE ( 'NONE', *, *, #9221, .T. ) ;
#59426=CARTESIAN_POINT ( 'NONE',  ( 39.40195752203892710, 9.424259417798131366, -23.77526687496409608 ) ) ;
#59427=CARTESIAN_POINT ( 'NONE',  ( -146.1140637052938871, 62.65471088530799904, 31.51667258806176974 ) ) ;
#59428=CARTESIAN_POINT ( 'NONE',  ( 56.19513604272052731, 11.19349063094195706, 67.28664494194475765 ) ) ;
#59430=CARTESIAN_POINT ( 'NONE',  ( -29.13697796587925026, 10.24294185249329203, -89.36513106409366003 ) ) ;
#59434=VECTOR ( 'NONE', #13869, 1000.000000000000000 ) ;
#59440=CARTESIAN_POINT ( 'NONE',  ( 66.73594759725092729, 13.56641407806656296, 43.82974788099483021 ) ) ;
#59441=EDGE_CURVE ( 'NONE', #61067, #14016, #10669, .T. ) ;
#59442=EDGE_LOOP ( 'NONE', ( #48661, #53472 ) ) ;
#59444=CYLINDRICAL_SURFACE ( 'NONE', #14783, 7.500000000000020428 ) ;
#59445=ADVANCED_FACE ( 'NONE', ( #24146 ), #24829, .F. ) ;
#59447=DIRECTION ( 'NONE',  ( 0.000000000000000000, 0.000000000000000000, 1.000000000000000000 ) ) ;
#59448=ORIENTED_EDGE ( 'NONE', *, *, #35514, .T. ) ;
#59450=VERTEX_POINT ( 'NONE', #19900 ) ;
#59453=CARTESIAN_POINT ( 'NONE',  ( 87.59061758233885087, 19.75077892934020696, 17.82126877942726040 ) ) ;
#59456=B_SPLINE_CURVE_WITH_KNOTS ( 'NONE', 3,
 ( #59341, #49119, #12209, #53710, #11153, #32618, #54045, #5870, #16776, #38235, #59676, #27677, #22409, #65326, #29427, #24514, #50877, #66734, #34015, #7639, #44909, #61769, #12556, #67762, #40324, #67415, #2697, #8327, #40666, #30131, #24160, #55456, #3389, #13595, #29090, #12917, #34372, #13258 ),
 .UNSPECIFIED., .F., .F.,
 ( 4, 2, 2, 2, 2, 2, 2, 2, 2, 2, 2, 2, 2, 2, 2, 2, 2, 2, 4 ),
 ( 0.000000000000000000, 0.001559859933532193633, 0.003119719867064387267, 0.004679579800596567023, 0.006239439734128746778, 0.007799299667660926534, 0.008579229634427035928, 0.009359159601193144454, 0.01091901953472536324, 0.01169894950149148738, 0.01247887946825761325, 0.01403873940178985980, 0.01559859933532211154, 0.01715845926885435982, 0.01871831920238660810, 0.02027817913591885637, 0.02183803906945110812, 0.02339789900298335640, 0.02495775893651560814 ),
 .UNSPECIFIED. ) ;
#59457=DIRECTION ( 'NONE',  ( -0.8160245890732938934, -0.5780171883497599028, 0.000000000000000000 ) ) ;
#59460=CARTESIAN_POINT ( 'NONE',  ( 66.73467315386237431, 14.60276727483218373, 43.84403630633526916 ) ) ;
#59465=EDGE_LOOP ( 'NONE', ( #38356, #56584, #10858, #46875 ) ) ;
#59466=CARTESIAN_POINT ( 'NONE',  ( 137.3861614007144851, 44.78548268714477132, -63.74609645935769464 ) ) ;
#59470=FACE_BOUND ( 'NONE', #10016, .T. ) ;
#59471=CARTESIAN_POINT ( 'NONE',  ( -4.513903087372260536, 6.697902023160579255, -76.49641857693266900 ) ) ;
#59472=CARTESIAN_POINT ( 'NONE',  ( -148.6426892915312692, 64.76241938621078020, -7.968279941028272972 ) ) ;
#59474=CARTESIAN_POINT ( 'NONE',  ( -83.69370847062540975, 25.38703975185374162, 5.502694545838179963 ) ) ;
#59477=CARTESIAN_POINT ( 'NONE',  ( -77.81700272789856854, 21.99959588779042718, -88.84078370873776009 ) ) ;
#59478=CARTESIAN_POINT ( 'NONE',  ( 66.29961816943395547, 13.45804302849873579, 3.708301206476156686 ) ) ;
#59479=CARTESIAN_POINT ( 'NONE',  ( 112.5721302457195776, 29.97407549554797868, 17.41144223022721960 ) ) ;
#59480=CARTESIAN_POINT ( 'NONE',  ( 88.98064924903393091, 21.30386569031178468, -9.351095346740329717 ) ) ;
#59481=ORIENTED_EDGE ( 'NONE', *, *, #24886, .F. ) ;
#59482=CARTESIAN_POINT ( 'NONE',  ( -38.69449158134467837, 11.92067517118076658, 8.909342758798803885 ) ) ;
#59487=CARTESIAN_POINT ( 'NONE',  ( 104.0290905220488469, 27.20720373712009987, 94.99999999999866418 ) ) ;
#59489=CARTESIAN_POINT ( 'NONE',  ( 69.74037587279241279, 14.33355757956374887, -13.01822706347090453 ) ) ;
#59491=CARTESIAN_POINT ( 'NONE',  ( -24.18158274621863768, 9.527343002918316373, -44.77222497198581408 ) ) ;
#59492=CARTESIAN_POINT ( 'NONE',  ( -51.77779688167512262, 14.86590802019196644, -76.31248613329042030 ) ) ;
#59493=LINE ( 'NONE', #27142, #56666 ) ;
#59494=CARTESIAN_POINT ( 'NONE',  ( -122.8011284400168250, 45.68452922414294193, -22.41731093363175020 ) ) ;
#59497=CARTESIAN_POINT ( 'NONE',  ( 31.91383250562745388, 8.564461488296997160, 64.74674811886252712 ) ) ;
#59500=AXIS2_PLACEMENT_3D ( 'NONE', #55686, #50064, #18063 ) ;
#59501=CARTESIAN_POINT ( 'NONE',  ( 63.42451435127777160, 13.80104019830836215, -89.40979201309713176 ) ) ;
#59503=CARTESIAN_POINT ( 'NONE',  ( 88.28889510440058075, 21.05995314109331318, 17.68549489745171854 ) ) ;
#59504=CARTESIAN_POINT ( 'NONE',  ( 184.0001683447903531, 83.06228184427189376, -23.80381492175980895 ) ) ;
#59505=CARTESIAN_POINT ( 'NONE',  ( 211.1046732743772907, 117.3965485104337318, 13.77185182296995158 ) ) ;
#59506=CARTESIAN_POINT ( 'NONE',  ( -80.76613269273198625, 24.21305865109442124, -89.09189068382836751 ) ) ;
#59507=CARTESIAN_POINT ( 'NONE',  ( 46.41758729921146909, 9.425975226414264441, -18.93824580312872996 ) ) ;
#59512=CARTESIAN_POINT ( 'NONE',  ( 132.9453095272139649, 42.04754713161464252, 17.66579024853170665 ) ) ;
#59513=CARTESIAN_POINT ( 'NONE',  ( 93.87111289824407834, 23.09598275302507275, -41.30595271919344214 ) ) ;
#59514=CARTESIAN_POINT ( 'NONE',  ( -47.55316895016326839, 13.83165595246918400, 65.16454658915249354 ) ) ;
#59519=EDGE_LOOP ( 'NONE', ( #67772, #52029, #11366, #44410 ) ) ;
#59522=EDGE_CURVE ( 'NONE', #29948, #8034, #45875, .T. ) ;
#59523=VERTEX_POINT ( 'NONE', #49284 ) ;
#59530=CARTESIAN_POINT ( 'NONE',  ( -62.53989795537027874, 16.81768094534200841, -69.05562491124992164 ) ) ;
#59532=LINE ( 'NONE', #16972, #17269 ) ;
#59533=CARTESIAN_POINT ( 'NONE',  ( 8.000000000000007105, 249.8719672152120381, 94.99999999999866418 ) ) ;
#59535=CARTESIAN_POINT ( 'NONE',  ( -156.6644740249450649, 71.86407434531899696, -71.41639533428784148 ) ) ;
#59539=CARTESIAN_POINT ( 'NONE',  ( -49.44484229820457699, 14.28460989390479519, -37.71214243090105356 ) ) ;
#59541=CARTESIAN_POINT ( 'NONE',  ( -30.46002654261638298, 10.45132580906818021, 30.26469554571997378 ) ) ;
#59544=CARTESIAN_POINT ( 'NONE',  ( -84.19760194758025307, 25.59349365599864257, 86.53227919859817518 ) ) ;
#59547=EDGE_LOOP ( 'NONE', ( #47294, #46889 ) ) ;
#59550=CARTESIAN_POINT ( 'NONE',  ( -13.47230132170245298, 7.324574289401430960, -11.11349493250400577 ) ) ;
#59551=CARTESIAN_POINT ( 'NONE',  ( -48.32993240732255913, 12.98137013984324817, 41.17929439291747684 ) ) ;
#59554=CARTESIAN_POINT ( 'NONE',  ( -38.54237244144231767, 11.89088379031762344, 66.98059792128260881 ) ) ;
#59555=CARTESIAN_POINT ( 'NONE',  ( -14.33060720034883495, 8.412649192293187639, -19.83824270713523319 ) ) ;
#59557=CARTESIAN_POINT ( 'NONE',  ( 23.09541709302173729, 6.844586979481591449, -17.88187169697903656 ) ) ;
#59563=CARTESIAN_POINT ( 'NONE',  ( -60.58154029404758489, 17.28267858483603447, -91.33302142368104626 ) ) ;
#59564=CARTESIAN_POINT ( 'NONE',  ( 117.4400732876363804, 32.35632188881473326, 88.66185363912092043 ) ) ;
#59566=CARTESIAN_POINT ( 'NONE',  ( 116.6681538161788723, 33.09439081574000596, -20.47854696611932468 ) ) ;
#59569=CARTESIAN_POINT ( 'NONE',  ( 140.2058232509808420, 46.59155168125931823, -12.65523780476208238 ) ) ;
#59575=CARTESIAN_POINT ( 'NONE',  ( 39.40195752203891999, 9.424259417798147354, -35.61981746542776506 ) ) ;
#59577=CARTESIAN_POINT ( 'NONE',  ( -149.9449619562961118, 64.55090813009795170, -22.96827994102829607 ) ) ;
#59579=CARTESIAN_POINT ( 'NONE',  ( 181.9295958320008708, 80.90438706151870463, 56.18881794660865125 ) ) ;
#59580=CARTESIAN_POINT ( 'NONE',  ( -151.6716822472524484, 66.03661194063735707, 57.87064893191389814 ) ) ;
#59582=CARTESIAN_POINT ( 'NONE',  ( -5.879983509979056500, 7.779504553499495323, -50.17789015261076457 ) ) ;
#59583=CARTESIAN_POINT ( 'NONE',  ( 104.3931729003987101, 26.26823401847090622, 14.98636371210345963 ) ) ;
#59586=CARTESIAN_POINT ( 'NONE',  ( 22.52576749827963809, 6.809805260274344185, 61.02798871425216731 ) ) ;
#59588=CARTESIAN_POINT ( 'NONE',  ( 15.29305096970402644, 7.491604910111012039, 18.17015708224157322 ) ) ;
#59593=CARTESIAN_POINT ( 'NONE',  ( -131.1078488676298832, 50.02394948559181387, -37.01727943492374351 ) ) ;
#59594=CARTESIAN_POINT ( 'NONE',  ( 45.04360969585142982, 9.210232288266690048, -64.99837574662008421 ) ) ;
#59595=CARTESIAN_POINT ( 'NONE',  ( 58.46823952472683317, 12.69204591816732908, -64.08093776701846878 ) ) ;
#59600=ADVANCED_FACE ( 'NONE', ( #24327 ), #28908, .F. ) ;
#59601=CARTESIAN_POINT ( 'NONE',  ( -190.6985136298602015, 109.1272424661243434, 16.02916387300914280 ) ) ;
#59602=CARTESIAN_POINT ( 'NONE',  ( 188.5939771839741752, 86.54409833618940695, 90.35527049066209315 ) ) ;
#59606=CARTESIAN_POINT ( 'NONE',  ( 185.1660960081723601, 84.30194217633003007, 30.51265424631614920 ) ) ;
#59609=CARTESIAN_POINT ( 'NONE',  ( 129.1052153257903683, 39.78893484542955150, -64.54437869395790983 ) ) ;
#59610=B_SPLINE_CURVE_WITH_KNOTS ( 'NONE', 3,
 ( #5874, #32284, #26992, #27334, #4851, #47749, #21714, #69212, #21036, #50194, #65688, #66397, #65330, #32969, #2362, #22761, #34379, #66743, #34020, #23814, #60036, #17476 ),
 .UNSPECIFIED., .F., .F.,
 ( 4, 2, 2, 2, 2, 2, 2, 2, 2, 2, 4 ),
 ( 7.734610455448194220E-17, 0.001318139496345227578, 0.001977209244517785965, 0.002636278992690344568, 0.003954418489035436621, 0.005272557985380528674, 0.005931627733553080338, 0.006590697481725632002, 0.007908836978070760484, 0.009226976474415886365, 0.01054511597076101224 ),
 .UNSPECIFIED. ) ;
#59611=CARTESIAN_POINT ( 'NONE',  ( 134.7720294983483029, 43.15885542353191084, 71.31265126893414674 ) ) ;
#59612=CARTESIAN_POINT ( 'NONE',  ( -76.32962633615591130, 21.44528079176260249, -49.74613438994566650 ) ) ;
#59615=CARTESIAN_POINT ( 'NONE',  ( 86.62931800182292363, 19.42108912189599224, -89.51066537983906812 ) ) ;
#59616=CARTESIAN_POINT ( 'NONE',  ( 89.87518614971254749, 20.55373388674513535, -50.09968107337091681 ) ) ;
#59617=CARTESIAN_POINT ( 'NONE',  ( -189.5325095384514213, 107.4952257375067433, 40.55217149438323077 ) ) ;
#59619=ORIENTED_EDGE ( 'NONE', *, *, #2104, .T. ) ;
#59620=CARTESIAN_POINT ( 'NONE',  ( 111.1767565371974911, 29.31586421952251698, -50.87893186375811894 ) ) ;
#59625=CARTESIAN_POINT ( 'NONE',  ( -170.2951623264596890, 85.51757001115470302, -62.09646688624404476 ) ) ;
#59628=CARTESIAN_POINT ( 'NONE',  ( 56.29445224195348629, 12.24017809212662122, 7.103959071770647782 ) ) ;
#59632=DIRECTION ( 'NONE',  ( 0.000000000000000000, 0.000000000000000000, 1.000000000000000000 ) ) ;
#59633=CARTESIAN_POINT ( 'NONE',  ( -55.53469534616546355, 14.81076603075805487, -23.37177340799619785 ) ) ;
#59636=CARTESIAN_POINT ( 'NONE',  ( 138.1919700334460686, 44.10401742531043823, -22.81667472755705006 ) ) ;
#59637=CARTESIAN_POINT ( 'NONE',  ( 93.86680996363769225, 22.01878169039501643, -68.18320037815716717 ) ) ;
#59638=CARTESIAN_POINT ( 'NONE',  ( 204.6977192012829789, 106.3443248447423315, 17.36317014830577321 ) ) ;
#59639=CARTESIAN_POINT ( 'NONE',  ( -95.21430597939257723, 29.33390900154318359, 8.609081036463225090 ) ) ;
#59644=CARTESIAN_POINT ( 'NONE',  ( 40.37438610703017616, 8.537526699166106070, 29.96096040500725977 ) ) ;
#59648=CARTESIAN_POINT ( 'NONE',  ( 211.8345664497466885, 118.5225165986914817, -46.15373158227198758 ) ) ;
#59650=CARTESIAN_POINT ( 'NONE',  ( -71.57660578921957040, 20.81129687646280146, -66.96296472413820311 ) ) ;
#59652=CARTESIAN_POINT ( 'NONE',  ( 45.89232972083998874, 10.36128169546909739, -46.88626132967853977 ) ) ;
#59653=CARTESIAN_POINT ( 'NONE',  ( 212.1535111375854967, 117.1635556319084799, 64.38318638549677075 ) ) ;
#59655=CARTESIAN_POINT ( 'NONE',  ( -26.50207385662995918, 9.849226639603646305, 5.204319795929868597 ) ) ;
#59659=CARTESIAN_POINT ( 'NONE',  ( -102.2801239173131052, 33.91021738430207222, 57.36362509687880618 ) ) ;
#59660=CYLINDRICAL_SURFACE ( 'NONE', #40884, 7.500000000000020428 ) ;
#59661=CARTESIAN_POINT ( 'NONE',  ( 93.72687053612526142, 23.04134601640627267, 61.58162035816948077 ) ) ;
#59662=CARTESIAN_POINT ( 'NONE',  ( 152.1327777395850660, 53.61712543276775023, -11.50499121041532469 ) ) ;
#59663=LINE ( 'NONE', #16072, #53462 ) ;
#59667=CARTESIAN_POINT ( 'NONE',  ( 211.9344894260836725, 116.8270173945561510, 88.38486393112469841 ) ) ;
#59669=ADVANCED_FACE ( 'NONE', ( #7090 ), #3215, .F. ) ;
#59671=CARTESIAN_POINT ( 'NONE',  ( 61.08522853873729019, 13.26388801693372343, 71.42126950169983957 ) ) ;
#59672=CARTESIAN_POINT ( 'NONE',  ( -102.2801239173131194, 32.78103895658057354, -8.170026674512225640 ) ) ;
#59673=CARTESIAN_POINT ( 'NONE',  ( -12.39770133248888406, 8.241491894828985920, 4.805493982876364534 ) ) ;
#59674=CARTESIAN_POINT ( 'NONE',  ( 46.65974587859241751, 10.48396258569371398, -71.91825419913200790 ) ) ;
#59675=CARTESIAN_POINT ( 'NONE',  ( -0.3258398948454890864, 6.518608385615800138, 37.11425296739088253 ) ) ;
#59676=CARTESIAN_POINT ( 'NONE',  ( -108.0980548770428129, 35.83569586822709141, -64.60032205779721437 ) ) ;
#59677=CARTESIAN_POINT ( 'NONE',  ( 92.40462699547136083, 22.54601413076274952, 86.10444742709040611 ) ) ;
#59683=CARTESIAN_POINT ( 'NONE',  ( -169.8972248494842745, 85.08697738648012887, -35.42540969111004756 ) ) ;
#59685=CARTESIAN_POINT ( 'NONE',  ( -132.9227230387961072, 52.53474289881230419, -39.78390660009881685 ) ) ;
#59686=ORIENTED_EDGE ( 'NONE', *, *, #61770, .T. ) ;
#59690=CARTESIAN_POINT ( 'NONE',  ( 197.2199163281728147, 98.22431253015349739, -17.64478213631704762 ) ) ;
#59691=CARTESIAN_POINT ( 'NONE',  ( -156.5968336791922582, 70.43374190556866665, 94.38119541604979190 ) ) ;
#59693=DIRECTION ( 'NONE',  ( -0.8160245890732938934, -0.5780171883497599028, 0.000000000000000000 ) ) ;
#59696=FACE_OUTER_BOUND ( 'NONE', #19588, .T. ) ;
#59697=CARTESIAN_POINT ( 'NONE',  ( 79.54836217416615796, 18.17815803851262402, 7.882887560960153195 ) ) ;
#59699=AXIS2_PLACEMENT_3D ( 'NONE', #27511, #48953, #43684 ) ;
#59702=VERTEX_POINT ( 'NONE', #60898 ) ;
#59707=EDGE_LOOP ( 'NONE', ( #69015, #13065 ) ) ;
#59708=CARTESIAN_POINT ( 'NONE',  ( -118.9073340572059863, 42.06264533740859690, -93.36481285813314912 ) ) ;
#59711=VERTEX_POINT ( 'NONE', #12720 ) ;
#59712=DIRECTION ( 'NONE',  ( -0.000000000000000000, 1.000000000000000000, -0.000000000000000000 ) ) ;
#59723=CARTESIAN_POINT ( 'NONE',  ( 127.2107679985236501, 38.70844091144996924, 67.36980645316099015 ) ) ;
#59725=ORIENTED_EDGE ( 'NONE', *, *, #3110, .T. ) ;
#59727=CARTESIAN_POINT ( 'NONE',  ( -47.60267131192345857, 12.80969088899330721, 90.58369976394168077 ) ) ;
#59730=CARTESIAN_POINT ( 'NONE',  ( -109.7865258608846801, 36.76046659111707271, 91.82485696114136431 ) ) ;
#59733=CARTESIAN_POINT ( 'NONE',  ( -48.51071349036728009, 14.05900477738932253, 87.82452332375471826 ) ) ;
#59735=VERTEX_POINT ( 'NONE', #26391 ) ;
#59739=CARTESIAN_POINT ( 'NONE',  ( 212.1707951106657504, 117.1901534358506041, -70.01254296698697033 ) ) ;
#59742=CARTESIAN_POINT ( 'NONE',  ( -38.78626392836186909, 10.91334659013840103, -95.00000000000133582 ) ) ;
#59743=CARTESIAN_POINT ( 'NONE',  ( 23.28845814680232351, 7.864847136539610872, 37.02807486054078367 ) ) ;
#59745=DIRECTION ( 'NONE',  ( -0.000000000000000000, 1.000000000000000000, -0.000000000000000000 ) ) ;
#59747=EDGE_LOOP ( 'NONE', ( #14610, #25675, #12657, #59764 ) ) ;
#59749=CARTESIAN_POINT ( 'NONE',  ( 157.4703587214989398, -170.0000000000000000, 36.90946747225337532 ) ) ;
#59755=CARTESIAN_POINT ( 'NONE',  ( -82.32750425780474757, 23.74963782027935721, 44.48151486517527076 ) ) ;
#59757=CARTESIAN_POINT ( 'NONE',  ( 61.09275639403233527, 12.23448398202909537, -50.48616642848160296 ) ) ;
#59761=CARTESIAN_POINT ( 'NONE',  ( 129.1381264900934411, 38.64720302602604107, -10.82883967016261550 ) ) ;
#59762=CIRCLE ( 'NONE', #29455, 242.4895526022646379 ) ;
#59764=ORIENTED_EDGE ( 'NONE', *, *, #28494, .T. ) ;
#59768=CARTESIAN_POINT ( 'NONE',  ( -147.3669217311067996, 63.69361261596465340, 31.02940414706721128 ) ) ;
#59769=CARTESIAN_POINT ( 'NONE',  ( 60.40277045393653310, 12.08176563382369650, 71.19188811025489372 ) ) ;
#59770=CARTESIAN_POINT ( 'NONE',  ( -5.412684891282531829, 7.753215344827982136, 57.34180824127475518 ) ) ;
#59771=EDGE_CURVE ( 'NONE', #49789, #55679, #20772, .T. ) ;
#59774=ORIENTED_EDGE ( 'NONE', *, *, #30042, .T. ) ;
#59778=EDGE_CURVE ( 'NONE', #26520, #38200, #67764, .T. ) ;
#59782=CARTESIAN_POINT ( 'NONE',  ( -170.2747214445850261, 84.01465441107043830, -8.415621470039866381 ) ) ;
#59786=ORIENTED_EDGE ( 'NONE', *, *, #7256, .T. ) ;
#59787=CARTESIAN_POINT ( 'NONE',  ( 84.28078136020371858, 18.63296074526051527, 17.49438883205864670 ) ) ;
#59789=CARTESIAN_POINT ( 'NONE',  ( -71.17819443284076897, 19.60909329639481058, 38.40917392580900014 ) ) ;
#59793=ORIENTED_EDGE ( 'NONE', *, *, #52182, .T. ) ;
#59794=CARTESIAN_POINT ( 'NONE',  ( -196.7348448768811409, -170.0000000000000000, 11.57801738291933091 ) ) ;
#59795=CARTESIAN_POINT ( 'NONE',  ( 88.98408042523108463, 20.23787745328941767, 3.242737632188622321 ) ) ;
#59801=CARTESIAN_POINT ( 'NONE',  ( 133.8566784816069344, -170.0000000000000000, -77.86786152285937135 ) ) ;
#59805=CARTESIAN_POINT ( 'NONE',  ( -173.1211646369891355, 88.63826465341152527, -34.71195716474998960 ) ) ;
#59806=CARTESIAN_POINT ( 'NONE',  ( -133.3926783185151521, 51.63401075114366279, -15.26785645255982438 ) ) ;
#59808=DIRECTION ( 'NONE',  ( -0.000000000000000000, 0.000000000000000000, -1.000000000000000000 ) ) ;
#59810=CARTESIAN_POINT ( 'NONE',  ( 134.0849965622593913, 42.73957449886184179, -77.86786152285938556 ) ) ;
#59812=ORIENTED_EDGE ( 'NONE', *, *, #32153, .T. ) ;
#59813=VECTOR ( 'NONE', #50071, 1000.000000000000000 ) ;
#59814=FACE_BOUND ( 'NONE', #41607, .T. ) ;
#59815=CARTESIAN_POINT ( 'NONE',  ( -0.8055628312658246193, 6.535476276302841114, -72.41444179526300218 ) ) ;
#59816=CARTESIAN_POINT ( 'NONE',  ( -179.5109681715918271, 96.11572638569522553, 61.20124511069693085 ) ) ;
#59817=CARTESIAN_POINT ( 'NONE',  ( 115.8407534776555252, 31.55877564758569775, -92.10373643822070733 ) ) ;
#59818=CARTESIAN_POINT ( 'NONE',  ( -118.3918229753715252, 42.92682904595257298, -42.92333884901141516 ) ) ;
#59822=CARTESIAN_POINT ( 'NONE',  ( -71.47840469610784453, 19.71248552135259757, -94.11786278736408917 ) ) ;
#59824=CARTESIAN_POINT ( 'NONE',  ( 115.0454575488273434, 31.16784721673997183, 4.500807871381157454 ) ) ;
#59825=CARTESIAN_POINT ( 'NONE',  ( 39.40195752203892710, 9.424259417798138472, -89.30891864635511013 ) ) ;
#59830=DIRECTION ( 'NONE',  ( 0.000000000000000000, -1.000000000000000000, 0.000000000000000000 ) ) ;
#59831=CARTESIAN_POINT ( 'NONE',  ( 106.0076881141067702, 28.07010157927252436, 84.57606687714297777 ) ) ;
#59832=CARTESIAN_POINT ( 'NONE',  ( 110.2429982417149574, -170.0000000000000000, -97.11153874658106133 ) ) ;
#59834=CARTESIAN_POINT ( 'NONE',  ( -30.95341298663138474, 10.53108683215057262, -50.31719736520187070 ) ) ;
#59835=CARTESIAN_POINT ( 'NONE',  ( 211.5787168283555673, 118.1262790876037485, -94.52141717514192010 ) ) ;
#59836=CARTESIAN_POINT ( 'NONE',  ( -78.24445602694504487, 23.23728082089436953, -88.80455181264525777 ) ) ;
#59837=CYLINDRICAL_SURFACE ( 'NONE', #25159, 7.500000000000013323 ) ;
#59839=ORIENTED_EDGE ( 'NONE', *, *, #50105, .F. ) ;
#59841=CARTESIAN_POINT ( 'NONE',  ( 32.66364305947234925, 8.639871491745250154, 67.58839702922695380 ) ) ;
#59842=CARTESIAN_POINT ( 'NONE',  ( 173.5843421840238250, 71.34465141434344559, 63.95638635334570665 ) ) ;
#59843=CARTESIAN_POINT ( 'NONE',  ( -165.6404838346739155, 80.60836113891895138, 65.78406423995896546 ) ) ;
#59844=EDGE_CURVE ( 'NONE', #2040, #65219, #55975, .T. ) ;
#59848=FACE_OUTER_BOUND ( 'NONE', #35067, .T. ) ;
#59851=CARTESIAN_POINT ( 'NONE',  ( -15.07200981767290848, 7.471751903425209562, 66.40871753783480358 ) ) ;
#59852=CARTESIAN_POINT ( 'NONE',  ( 211.4997502125519304, 118.0043045815490501, 6.689424349925599422 ) ) ;
#59856=CARTESIAN_POINT ( 'NONE',  ( 44.34263167748004264, 9.103379693481564061, -21.93902944785204667 ) ) ;
#59858=FACE_BOUND ( 'NONE', #60149, .T. ) ;
#59859=CARTESIAN_POINT ( 'NONE',  ( -61.38706483483509402, 16.47181058798475917, -38.69296264354031223 ) ) ;
#59866=CARTESIAN_POINT ( 'NONE',  ( 87.58754341703158275, 20.81465688423120142, -35.86779864721757605 ) ) ;
#59868=CARTESIAN_POINT ( 'NONE',  ( -49.43836229152578454, 14.28302414152160438, 59.66443661698006906 ) ) ;
#59870=CARTESIAN_POINT ( 'NONE',  ( 151.1873096904021736, 52.92629247302095763, 14.16866593802975949 ) ) ;
#59871=LINE ( 'NONE', #12747, #8620 ) ;
#59873=CARTESIAN_POINT ( 'NONE',  ( 55.76298701799387914, 11.10663440745154240, 12.44327555652177608 ) ) ;
#59874=CARTESIAN_POINT ( 'NONE',  ( -58.32860549785897319, 15.58423118879329294, 57.91070985857294318 ) ) ;
#59876=VERTEX_POINT ( 'NONE', #8052 ) ;
#59879=CARTESIAN_POINT ( 'NONE',  ( 102.8066580714140912, 25.59117171226998977, 36.10287978058507008 ) ) ;
#59882=CARTESIAN_POINT ( 'NONE',  ( 41.80372346091802882, 9.750024116765239057, 71.36764769552664234 ) ) ;
#59884=CARTESIAN_POINT ( 'NONE',  ( -156.9919426121902575, 72.16759471857101005, -68.59451387288930846 ) ) ;
#59885=CARTESIAN_POINT ( 'NONE',  ( 70.12389542974194967, 15.47520081968154315, 8.025324115680595227 ) ) ;
#59887=CARTESIAN_POINT ( 'NONE',  ( -47.55316895016326129, 13.83165595246916801, -42.21365577270224634 ) ) ;
#59890=CARTESIAN_POINT ( 'NONE',  ( -155.3934881382774336, 70.69666961025296814, -91.34784486870364617 ) ) ;
#59892=CARTESIAN_POINT ( 'NONE',  ( 81.09284835776151112, 17.60558077568531132, 85.83069754542404439 ) ) ;
#59894=ORIENTED_EDGE ( 'NONE', *, *, #28499, .F. ) ;
#59895=ORIENTED_EDGE ( 'NONE', *, *, #11472, .F. ) ;
#59898=CARTESIAN_POINT ( 'NONE',  ( -171.5398786593827936, 86.87885897849457706, 84.67500624867942349 ) ) ;
#59902=CARTESIAN_POINT ( 'NONE',  ( -61.53550548562875377, 17.56596194025584978, -38.91274425169289231 ) ) ;
#59903=B_SPLINE_CURVE_WITH_KNOTS ( 'NONE', 3,
 ( #63190, #33616, #22694, #33261, #54695, #59612, #28675, #50130, #1241, #60330, #11091, #7219, #49060, #54336, #895, #39234, #28315, #44131, #545, #59968, #32898, #53984, #43785, #6155, #65622, #32553, #11428, #1957, #12151, #49413, #55042, #6865, #5810, #65259, #27264, #38886, #17409, #21998, #11785, #55390, #49757, #23053, #27969, #17052 ),
 .UNSPECIFIED., .F., .F.,
 ( 4, 2, 2, 2, 2, 2, 2, 2, 2, 2, 2, 2, 2, 2, 2, 2, 2, 2, 2, 2, 2, 4 ),
 ( 0.02432640572110343624, 0.02583721026359364625, 0.02659261253483873391, 0.02734801480608382157, 0.02885881934857402811, 0.02961422161981911577, 0.03036962389106420343, 0.03188042843355436140, 0.03339123297604452978, 0.03414663524728961397, 0.03490203751853471204, 0.03641284206102490123, 0.03716824433226999930, 0.03792364660351509736, 0.03943445114600528656, 0.04094525568849546882, 0.04245606023098566495, 0.04396686477347584721, 0.04472226704472094527, 0.04547766931596604334, 0.04698847385845628111, 0.04849927840094651194 ),
 .UNSPECIFIED. ) ;
#59905=CARTESIAN_POINT ( 'NONE',  ( -10.69547592951790982, 8.103864096836385755, -23.01549004601787729 ) ) ;
#59906=CARTESIAN_POINT ( 'NONE',  ( -71.37402418445425667, 19.67651958824262692, -71.23054666910613264 ) ) ;
#59907=CARTESIAN_POINT ( 'NONE',  ( 21.75684465274325063, 6.764994602232768273, -11.60645927818548451 ) ) ;
#59912=EDGE_LOOP ( 'NONE', ( #59481, #42714 ) ) ;
#59913=CARTESIAN_POINT ( 'NONE',  ( -143.2587158300141823, 60.34092810886538416, 15.53215084215549346 ) ) ;
#59916=CARTESIAN_POINT ( 'NONE',  ( 117.1442106208647971, 32.20759653584552495, 93.81850280107182982 ) ) ;
#59918=EDGE_CURVE ( 'NONE', #19003, #33435, #5611, .T. ) ;
#59920=CARTESIAN_POINT ( 'NONE',  ( -78.66644367742109978, 23.39876645725290061, 45.41820113967312977 ) ) ;
#59921=CARTESIAN_POINT ( 'NONE',  ( 138.5684226926155702, 45.53585076428269218, -10.82367928455951400 ) ) ;
#59927=CARTESIAN_POINT ( 'NONE',  ( -156.9232798886536386, 72.10386843399170687, -16.62516299996477898 ) ) ;
#59930=CARTESIAN_POINT ( 'NONE',  ( 63.01563776193090405, 12.67277567978497643, -8.876140241706053757 ) ) ;
#59932=CARTESIAN_POINT ( 'NONE',  ( -37.07086358537074489, 10.58360809068250141, 69.53818740131970344 ) ) ;
#59934=ORIENTED_EDGE ( 'NONE', *, *, #48505, .T. ) ;
#59936=CARTESIAN_POINT ( 'NONE',  ( -156.6692143066620133, 70.50016761530883969, 62.82118311751774797 ) ) ;
#59942=CARTESIAN_POINT ( 'NONE',  ( 20.74093720376649586, 6.709541214524347374, 58.70593033936504668 ) ) ;
#59943=CARTESIAN_POINT ( 'NONE',  ( -190.0891074294818566, 108.2702128816165583, 88.58129052767998246 ) ) ;
#59944=CARTESIAN_POINT ( 'NONE',  ( 10.83418588031599228, 6.392467435475928994, -75.51611801531713297 ) ) ;
#59946=EDGE_CURVE ( 'NONE', #17554, #60122, #4747, .T. ) ;
#59950=CARTESIAN_POINT ( 'NONE',  ( -133.3149301983942507, 51.57857650535020611, -68.13965555861794599 ) ) ;
#59953=CARTESIAN_POINT ( 'NONE',  ( 59.29474530993687864, 12.86968658439548463, -63.54875636054207888 ) ) ;
#59957=CARTESIAN_POINT ( 'NONE',  ( -131.8293781841207988, 50.52790876176725021, -91.49601856444540715 ) ) ;
#59959=CARTESIAN_POINT ( 'NONE',  ( 187.0823097343935331, 84.88801889414973800, 94.99999999999866418 ) ) ;
#59963=CARTESIAN_POINT ( 'NONE',  ( 177.5945652320814645, 75.14951358071817822, -37.08239668887548390 ) ) ;
#59967=CARTESIAN_POINT ( 'NONE',  ( 141.3586046882815879, 47.34625111366352712, 63.34599527006825070 ) ) ;
#59968=CARTESIAN_POINT ( 'NONE',  ( -71.43874587651170316, 19.69883891272894871, -44.63390031017252824 ) ) ;
#59970=CARTESIAN_POINT ( 'NONE',  ( 79.51684382776136317, 17.11558840174940954, -94.59398989896673982 ) ) ;
#59972=CARTESIAN_POINT ( 'NONE',  ( -190.3061188229048923, 108.5745819235681608, 42.30307631859309225 ) ) ;
#59979=CARTESIAN_POINT ( 'NONE',  ( -133.0156404686407825, 51.36557667666784965, 89.43440121892608374 ) ) ;
#59981=CARTESIAN_POINT ( 'NONE',  ( 56.28782924480457694, 12.23883190161851076, 13.82014511301142967 ) ) ;
#59982=ORIENTED_EDGE ( 'NONE', *, *, #36767, .T. ) ;
#59983=CARTESIAN_POINT ( 'NONE',  ( -132.4951995226844872, 50.99687809989497111, 34.55095761923556097 ) ) ;
#59988=CARTESIAN_POINT ( 'NONE',  ( 79.22946426532584496, 17.02750615740071183, -17.72431334350951104 ) ) ;
#59990=CARTESIAN_POINT ( 'NONE',  ( 93.92910382125423041, 22.04227458821881669, -68.42647781650052252 ) ) ;
#59992=CARTESIAN_POINT ( 'NONE',  ( -24.61452482346733461, 8.570300138934635825, -93.36648426586947380 ) ) ;
#59998=DIRECTION ( 'NONE',  ( 0.000000000000000000, 0.000000000000000000, 1.000000000000000000 ) ) ;
#60002=CARTESIAN_POINT ( 'NONE',  ( 211.5034924207027984, 118.0100795718635140, -40.66011177504395135 ) ) ;
#60006=CARTESIAN_POINT ( 'NONE',  ( 44.34362023773823580, 10.12115849931653599, -48.78329502920555427 ) ) ;
#60007=CARTESIAN_POINT ( 'NONE',  ( 159.6593397521790507, 59.37286298965128140, -77.65605731442671811 ) ) ;
#60010=CARTESIAN_POINT ( 'NONE',  ( -29.04400972079232446, 10.22852224114067354, 17.98340990312981802 ) ) ;
#60011=EDGE_CURVE ( 'NONE', #46836, #57348, #33377, .T. ) ;
#60014=AXIS2_PLACEMENT_3D ( 'NONE', #65981, #60680, #37833 ) ;
#60015=CARTESIAN_POINT ( 'NONE',  ( -85.89966968015255588, 25.20990842792081565, 89.59847398112991357 ) ) ;
#60016=CARTESIAN_POINT ( 'NONE',  ( 93.08174259058945665, 22.79847752828721141, 67.91146075705054841 ) ) ;
#60017=CARTESIAN_POINT ( 'NONE',  ( 126.3732561463888118, 38.23795180971327312, 36.44577969812711160 ) ) ;
#60018=CARTESIAN_POINT ( 'NONE',  ( 32.66364305947235636, 8.639871491745251930, 13.89929584829961229 ) ) ;
#60019=LINE ( 'NONE', #11478, #12110 ) ;
#60023=CARTESIAN_POINT ( 'NONE',  ( 211.6713973331038687, 116.4246122071819229, 87.60636827412143646 ) ) ;
#60032=CARTESIAN_POINT ( 'NONE',  ( 79.53788081641260987, 18.17489638840366695, 88.43542930566641758 ) ) ;
#60036=CARTESIAN_POINT ( 'NONE',  ( -190.4966031023458584, 108.8421921967458701, -11.08920354847794876 ) ) ;
#60037=CARTESIAN_POINT ( 'NONE',  ( -128.9786047358386440, 48.55852351614670681, 18.11557624711077352 ) ) ;
#60039=CARTESIAN_POINT ( 'NONE',  ( -173.1211646369891355, 88.63826465341151106, -49.71195716475001092 ) ) ;
#60040=CARTESIAN_POINT ( 'NONE',  ( -132.5976199670998597, 52.30296609017644016, -45.78660264953770564 ) ) ;
#60041=ORIENTED_EDGE ( 'NONE', *, *, #16200, .F. ) ;
#60042=CARTESIAN_POINT ( 'NONE',  ( -124.1094910780272329, 45.33021696310841975, -49.70193067791534958 ) ) ;
#60044=CARTESIAN_POINT ( 'NONE',  ( -146.1260528621668300, 61.36307454672305539, -22.17874663354146492 ) ) ;
#60045=LINE ( 'NONE', #11867, #57373 ) ;
#60050=CARTESIAN_POINT ( 'NONE',  ( 197.1980152960110217, 96.59350208824301376, -43.48860924640160874 ) ) ;
#60051=CARTESIAN_POINT ( 'NONE',  ( -152.2873556200145515, 67.91256772393730046, 31.25152339806742319 ) ) ;
#60052=CARTESIAN_POINT ( 'NONE',  ( 17.72992212664810907, 6.570588738776105941, -50.26741213039321821 ) ) ;
#60054=CARTESIAN_POINT ( 'NONE',  ( 115.0485321076020568, 32.28990710985445389, 16.04577514241892899 ) ) ;
#60061=CARTESIAN_POINT ( 'NONE',  ( -119.9387902904519763, 42.69579278498642338, -91.52063911540987817 ) ) ;
#60062=AXIS2_PLACEMENT_3D ( 'NONE', #10760, #53307, #38534 ) ;
#60064=CARTESIAN_POINT ( 'NONE',  ( -14.33576511807126863, 8.413127487936190363, -66.00693546820657787 ) ) ;
#60066=CARTESIAN_POINT ( 'NONE',  ( 160.9069879467680835, 60.37290772564308128, 30.22702203457957992 ) ) ;
#60067=CARTESIAN_POINT ( 'NONE',  ( 8.000000000000007105, 249.8719672152120381, 94.99999999999866418 ) ) ;
#60074=CARTESIAN_POINT ( 'NONE',  ( -119.1064753703575718, 42.18441154001784099, 94.99999999999866418 ) ) ;
#60075=CARTESIAN_POINT ( 'NONE',  ( -180.6021503146988891, 97.45669259943416307, 38.94198014546275033 ) ) ;
#60076=CARTESIAN_POINT ( 'NONE',  ( -35.99432170610151616, 10.38324794858010591, -75.63980193136818286 ) ) ;
#60077=CARTESIAN_POINT ( 'NONE',  ( 22.28556289340099283, 7.803548444155005370, 60.60479519626248646 ) ) ;
#60078=ORIENTED_EDGE ( 'NONE', *, *, #48, .T. ) ;
#60081=LINE ( 'NONE', #50241, #66575 ) ;
#60082=CARTESIAN_POINT ( 'NONE',  ( -103.8932886509196436, 34.74144483217662582, 3.846358069395087398 ) ) ;
#60084=CARTESIAN_POINT ( 'NONE',  ( -37.38781680082738035, 10.64362327909143069, -47.41097133852251488 ) ) ;
#60085=CARTESIAN_POINT ( 'NONE',  ( -95.54114085644955878, 29.48728305236672398, 94.99999999999866418 ) ) ;
#60089=CARTESIAN_POINT ( 'NONE',  ( -74.20136529587826146, 21.74007521413449240, -9.739908195685467618 ) ) ;
#60090=CARTESIAN_POINT ( 'NONE',  ( 86.62931800182293784, 19.42108912189596381, 56.55663816294300261 ) ) ;
#60092=VERTEX_POINT ( 'NONE', #18181 ) ;
#60094=CARTESIAN_POINT ( 'NONE',  ( -99.40451658125527956, 32.46531518262781901, -89.26390591963935606 ) ) ;
#60096=CARTESIAN_POINT ( 'NONE',  ( 212.1535111375855251, 117.1635556319084941, -69.83956656682167363 ) ) ;
#60099=LINE ( 'NONE', #33032, #41678 ) ;
#60104=EDGE_CURVE ( 'NONE', #26499, #40777, #23469, .T. ) ;
#60112=CARTESIAN_POINT ( 'NONE',  ( 15.78827728214693416, -170.0000000000000000, 71.85925826316895382 ) ) ;
#60114=CARTESIAN_POINT ( 'NONE',  ( -83.52505811737952968, 24.23179517241433700, 32.18346549745763241 ) ) ;
#60116=CARTESIAN_POINT ( 'NONE',  ( -24.71604178686819964, 9.599501655372948861, -72.99519987063204951 ) ) ;
#60117=CARTESIAN_POINT ( 'NONE',  ( 46.12611922993085756, 10.39838587005582404, 34.08266634447561927 ) ) ;
#60119=CARTESIAN_POINT ( 'NONE',  ( -142.3178993725749137, 58.31327888234797285, 13.58478421935505409 ) ) ;
#60121=EDGE_CURVE ( 'NONE', #41030, #30857, #2356, .T. ) ;
#60122=VERTEX_POINT ( 'NONE', #66733 ) ;
#60126=EDGE_CURVE ( 'NONE', #32549, #20980, #24083, .T. ) ;
#60128=ORIENTED_EDGE ( 'NONE', *, *, #7043, .T. ) ;
#60130=PLANE ( 'NONE',  #16970 ) ;
#60131=B_SPLINE_CURVE_WITH_KNOTS ( 'NONE', 3,
 ( #51801, #61998, #56380, #20133, #18756, #41586, #35279, #56736, #63044, #40212, #30004, #8896, #8201, #46513, #3609, #7859, #29307, #50758, #61660, #29652, #19790, #62709, #14510, #32421, #16577, #15551, #59130, #4640, #31720, #37683, #21174, #4986, #64075, #53847, #64771, #5665, #21504, #31044, #63397, #47889, #9584, #10601, #63743, #58113, #21852, #26452 ),
 .UNSPECIFIED., .F., .F.,
 ( 4, 2, 2, 2, 2, 2, 2, 2, 2, 2, 2, 2, 2, 2, 2, 2, 2, 2, 2, 2, 2, 2, 4 ),
 ( 0.02420077021543440635, 0.02572112563160185161, 0.02648130333968559333, 0.02724148104776933851, 0.02876183646393682541, 0.02952201417202056713, 0.03028219188010430885, 0.03180254729627179228, 0.03332290271243927571, 0.03408308042052300008, 0.03484325812860672444, 0.03636361354477421481, 0.03712379125285794612, 0.03788396896094166355, 0.03864414666902539486, 0.03940432437710911923, 0.04092467979327658878, 0.04244503520944406527, 0.04396539062561152789, 0.04548574604177900438, 0.04624592374986273569, 0.04700610145794646699, 0.04852645687411388797 ),
 .UNSPECIFIED. ) ;
#60132=CARTESIAN_POINT ( 'NONE',  ( -7.825402957745085430, 7.899365992529246761, 18.27103044898354511 ) ) ;
#60133=CARTESIAN_POINT ( 'NONE',  ( 141.0652542208218847, 47.15334271457688686, 92.80065851230959595 ) ) ;
#60137=CARTESIAN_POINT ( 'NONE',  ( -123.6699087229882110, 45.04696784753415528, -76.42458631566876193 ) ) ;
#60142=LINE ( 'NONE', #11959, #11661 ) ;
#60143=CARTESIAN_POINT ( 'NONE',  ( 134.3172730033262781, 41.70277427218488953, -62.86786152285933582 ) ) ;
#60149=EDGE_LOOP ( 'NONE', ( #25351, #49861 ) ) ;
#60151=CARTESIAN_POINT ( 'NONE',  ( 126.6904219525097659, 37.26255867422720058, -95.00000000000133582 ) ) ;
#60154=CARTESIAN_POINT ( 'NONE',  ( -144.2188519266539970, 59.82027639618912218, -74.48106321738612223 ) ) ;
#60162=CARTESIAN_POINT ( 'NONE',  ( 32.37980458033285913, 8.611076697115702672, 40.05964868220856090 ) ) ;
#60164=CARTESIAN_POINT ( 'NONE',  ( -175.9864315813574649, 91.91454246454362931, -49.15589249871932509 ) ) ;
#60170=CARTESIAN_POINT ( 'NONE',  ( -144.2038301586456726, 61.09856042007390897, -74.48259089573751623 ) ) ;
#60172=FACE_BOUND ( 'NONE', #19330, .T. ) ;
#60173=CARTESIAN_POINT ( 'NONE',  ( -0.3734056954813064766, 6.520221844775929476, -68.78453539205794698 ) ) ;
#60174=CARTESIAN_POINT ( 'NONE',  ( -180.5200658187031593, 97.35517482626556784, 63.89930464416294598 ) ) ;
#60176=FACE_OUTER_BOUND ( 'NONE', #24617, .T. ) ;
#60178=DIRECTION ( 'NONE',  ( 0.000000000000000000, -1.000000000000000000, 0.000000000000000000 ) ) ;
#60181=CARTESIAN_POINT ( 'NONE',  ( -76.98209973255083582, 21.68691446935567058, -88.98387085312982947 ) ) ;
#60182=ADVANCED_FACE ( 'NONE', ( #46983 ), #35398, .F. ) ;
#60183=CARTESIAN_POINT ( 'NONE',  ( -15.27594996066617661, 8.502079791899644690, 36.62617975021709071 ) ) ;
#60184=CARTESIAN_POINT ( 'NONE',  ( 115.2288739107204947, 31.25773204386717197, 4.658657091807949513 ) ) ;
#60186=CARTESIAN_POINT ( 'NONE',  ( 93.08073375333748345, 22.79826000593201840, -20.31003796707942044 ) ) ;
#60188=CARTESIAN_POINT ( 'NONE',  ( -38.93847286785603501, 11.96870349976817494, 10.36518148543439821 ) ) ;
#60189=ORIENTED_EDGE ( 'NONE', *, *, #30279, .T. ) ;
#60192=CARTESIAN_POINT ( 'NONE',  ( 79.19119222799089641, 18.06817527909834808, -69.17202811480721891 ) ) ;
#60193=CARTESIAN_POINT ( 'NONE',  ( 103.1614067554331342, 26.83495172254625061, 88.30558029229318606 ) ) ;
#60196=CARTESIAN_POINT ( 'NONE',  ( -28.81071653159242274, 10.19258396314334725, -35.78856510997613327 ) ) ;
#60199=CARTESIAN_POINT ( 'NONE',  ( -190.6985136298602015, 109.1272424661243434, -64.50448789838189612 ) ) ;
#60202=CARTESIAN_POINT ( 'NONE',  ( 32.03384598935270589, 8.576372641736000446, 65.72151599203246519 ) ) ;
#60203=CARTESIAN_POINT ( 'NONE',  ( 177.2011275744679608, 74.76848439756739140, 57.23258176878422887 ) ) ;
#60206=CARTESIAN_POINT ( 'NONE',  ( -166.3205068063721228, 81.30869308872868828, 61.99160270357487690 ) ) ;
#60207=CARTESIAN_POINT ( 'NONE',  ( -167.4844853368929307, 82.52074065752739784, -20.32144448876292842 ) ) ;
#60209=CARTESIAN_POINT ( 'NONE',  ( 181.0840389613909736, -170.0000000000000000, 2.464043515047718014 ) ) ;
#60212=CARTESIAN_POINT ( 'NONE',  ( 106.6322547488295385, 28.34756922280616465, -50.01364319867063557 ) ) ;
#60215=CARTESIAN_POINT ( 'NONE',  ( 185.1660960081723033, 84.30194217633003007, -23.17644693461118877 ) ) ;
#60216=CARTESIAN_POINT ( 'NONE',  ( 10.83521140779424030, 7.398743030771586682, 58.70627392783954690 ) ) ;
#60218=CARTESIAN_POINT ( 'NONE',  ( 45.49006904354233427, 9.279592366778889101, -20.66221359758136344 ) ) ;
#60219=CARTESIAN_POINT ( 'NONE',  ( -125.8938041572051389, 47.69968343338778283, -76.75825448869764500 ) ) ;
#60220=FACE_BOUND ( 'NONE', #61916, .T. ) ;
#60223=CARTESIAN_POINT ( 'NONE',  ( -55.54058841405663571, 14.81234591756537711, -35.21632399845985617 ) ) ;
#60227=ORIENTED_EDGE ( 'NONE', *, *, #54469, .T. ) ;
#60230=CARTESIAN_POINT ( 'NONE',  ( -48.34250119710924309, 14.01879126850790058, 61.30265284070986809 ) ) ;
#60231=CARTESIAN_POINT ( 'NONE',  ( -180.4651598106648294, 97.28730001475651079, 13.02874545039772336 ) ) ;
#60232=CARTESIAN_POINT ( 'NONE',  ( 210.9608386442062624, 117.1762372255316222, 67.68640205245998231 ) ) ;
#60234=ORIENTED_EDGE ( 'NONE', *, *, #14696, .T. ) ;
#60235=CARTESIAN_POINT ( 'NONE',  ( 55.56474667084419394, 11.06706367715631423, 11.46101165398160582 ) ) ;
#60237=ORIENTED_EDGE ( 'NONE', *, *, #7557, .F. ) ;
#60241=CARTESIAN_POINT ( 'NONE',  ( 87.11239765416380010, 20.65008247340817960, -62.66611478937536361 ) ) ;
#60243=B_SPLINE_CURVE_WITH_KNOTS ( 'NONE', 3,
 ( #50481, #1593, #7223, #23056, #44505, #38175, #65984, #17780, #17056, #12501, #22003, #1960, #33266, #64921, #6525, #16717, #59617, #11431, #38527, #59972, #57149, #35699 ),
 .UNSPECIFIED., .F., .F.,
 ( 4, 2, 2, 2, 2, 2, 2, 2, 2, 2, 4 ),
 ( 8.002322828458971877E-17, 0.001318139496345214351, 0.001977209244517765148, 0.002636278992690316379, 0.003954418489035409733, 0.005272557985380503520, 0.005931627733553051715, 0.006590697481725598175, 0.007908836978070736198, 0.009226976474415874221, 0.01054511597076101224 ),
 .UNSPECIFIED. ) ;
#60244=ORIENTED_EDGE ( 'NONE', *, *, #64471, .F. ) ;
#60247=CARTESIAN_POINT ( 'NONE',  ( -156.1477286774993729, 71.38742644140633331, -65.66038772067875584 ) ) ;
#60248=CARTESIAN_POINT ( 'NONE',  ( 68.63585058221465829, 15.08566240483131793, 5.477619919286003558 ) ) ;
#60251=CARTESIAN_POINT ( 'NONE',  ( -47.79955240516188297, 13.88975739862082470, -44.68859367444699160 ) ) ;
#60254=CARTESIAN_POINT ( 'NONE',  ( -47.61402178322637013, 13.84598486314981436, 9.983978065502588706 ) ) ;
#60255=CARTESIAN_POINT ( 'NONE',  ( -131.3096895243911320, 51.39228038925232056, -10.35808099536435556 ) ) ;
#60256=B_SPLINE_CURVE_WITH_KNOTS ( 'NONE', 3,
 ( #15640, #37426, #58878, #65567, #6471, #21943, #33904, #59563, #28261, #33210, #65211, #64864, #32848, #6811, #22998, #43394, #38836, #23360, #49357, #49707, #16667, #1537, #44444, #65933 ),
 .UNSPECIFIED., .F., .F.,
 ( 4, 2, 2, 2, 2, 2, 2, 2, 2, 2, 2, 4 ),
 ( 0.000000000000000000, 0.001318322376542587935, 0.002636644753085175871, 0.003954967129627763589, 0.004614128317899063303, 0.005273289506170363017, 0.006591611882712936424, 0.007250773070984224862, 0.007909934259255513300, 0.009228256635798121402, 0.009887417824069429789, 0.01054657901234073818 ),
 .UNSPECIFIED. ) ;
#60257=CARTESIAN_POINT ( 'NONE',  ( -153.2277253043372696, 68.74531066433421245, -89.48623125317686799 ) ) ;
#60259=CARTESIAN_POINT ( 'NONE',  ( -78.66644367742111399, -170.0000000000000000, 37.91820113967311556 ) ) ;
#60260=AXIS2_PLACEMENT_3D ( 'NONE', #59071, #68272, #31329 ) ;
#60268=CARTESIAN_POINT ( 'NONE',  ( -48.99162761293257518, 13.13973062091724131, -20.29604390856045626 ) ) ;
#60269=CARTESIAN_POINT ( 'NONE',  ( 106.6192711434718348, 27.24117154335862168, -23.14876697959396168 ) ) ;
#60273=CARTESIAN_POINT ( 'NONE',  ( -38.92718193365331558, 11.96647478777219398, 65.05036416477805972 ) ) ;
#60275=CARTESIAN_POINT ( 'NONE',  ( -71.16770070143908811, 19.60548673929830699, -69.98478112900720305 ) ) ;
#60276=CARTESIAN_POINT ( 'NONE',  ( 22.81270948571149404, 6.827178363529887939, -13.53470793533548999 ) ) ;
#60277=VERTEX_POINT ( 'NONE', #53625 ) ;
#60285=CARTESIAN_POINT ( 'NONE',  ( -24.84040467973654742, 9.616437491640137836, 87.82595348829025284 ) ) ;
#60286=CARTESIAN_POINT ( 'NONE',  ( -94.89192151156326815, 29.18342430963128109, -43.83071791538480255 ) ) ;
#60288=CARTESIAN_POINT ( 'NONE',  ( 14.08810621383467421, 7.458732232275138152, -50.32784852290144784 ) ) ;
#60289=CARTESIAN_POINT ( 'NONE',  ( 141.2361973397653685, 47.26569015399785911, -15.31408827969341502 ) ) ;
#60292=VERTEX_POINT ( 'NONE', #69464 ) ;
#60294=CARTESIAN_POINT ( 'NONE',  ( -156.7435307435793845, 71.93726016406967005, -17.46061737335302766 ) ) ;
#60295=CARTESIAN_POINT ( 'NONE',  ( 36.99625334683020128, 8.108440754877207723, -77.08499119840222136 ) ) ;
#60296=CARTESIAN_POINT ( 'NONE',  ( 56.19211641164836379, 11.19288081156168424, -19.49878541329645287 ) ) ;
#60297=CARTESIAN_POINT ( 'NONE',  ( -51.35181696773305760, 13.72007042346227124, 31.27555066828208297 ) ) ;
#60298=LINE ( 'NONE', #50782, #34033 ) ;
#60301=CARTESIAN_POINT ( 'NONE',  ( -155.7433525314459075, 69.65452735858370659, 69.24046085996992872 ) ) ;
#60303=CARTESIAN_POINT ( 'NONE',  ( -165.9992860119575084, 79.53569239468048124, 9.108083402024591990 ) ) ;
#60304=CARTESIAN_POINT ( 'NONE',  ( -83.14462298835725562, 24.07775853418030820, -48.65102209861048976 ) ) ;
#60305=FACE_OUTER_BOUND ( 'NONE', #45093, .T. ) ;
#60312=CARTESIAN_POINT ( 'NONE',  ( -131.7724154034330581, 50.48821165954356616, -64.59405240136965176 ) ) ;
#60313=CARTESIAN_POINT ( 'NONE',  ( -156.3413281584584809, 71.56573911209629557, 94.99999999999866418 ) ) ;
#60314=CARTESIAN_POINT ( 'NONE',  ( 45.02738683369920381, 9.207938468499232698, -74.93078921836432471 ) ) ;
#60315=CARTESIAN_POINT ( 'NONE',  ( 61.08522853873727598, 13.26388801693373232, -62.80148345061859061 ) ) ;
#60321=CARTESIAN_POINT ( 'NONE',  ( 184.2892190079700754, 81.90639475741072317, 83.71060938861219825 ) ) ;
#60324=ORIENTED_EDGE ( 'NONE', *, *, #42321, .F. ) ;
#60328=CARTESIAN_POINT ( 'NONE',  ( 114.6797682035589503, 32.10876583290007602, 57.88993258366536310 ) ) ;
#60329=CARTESIAN_POINT ( 'NONE',  ( 141.2801018238827169, 47.29457739955282847, 64.95722907669554047 ) ) ;
#60330=CARTESIAN_POINT ( 'NONE',  ( -74.40004226286977485, 20.74218500375955543, -48.78853105593013595 ) ) ;
#60332=CARTESIAN_POINT ( 'NONE',  ( 92.53566308513168792, 21.52138666710686010, -38.67290711224870137 ) ) ;
#60334=CARTESIAN_POINT ( 'NONE',  ( -47.61402178322638434, 13.84598486314981614, -16.86057252496108561 ) ) ;
#60337=CARTESIAN_POINT ( 'NONE',  ( 115.2288739107204663, 31.25773204386719684, -49.03044408911942753 ) ) ;
#60339=CARTESIAN_POINT ( 'NONE',  ( 133.8566784816069344, -170.0000000000000000, 17.66579024853170310 ) ) ;
#60340=CARTESIAN_POINT ( 'NONE',  ( -143.8634661037141029, 60.82480701605698670, -47.27825893513519873 ) ) ;
#60344=CARTESIAN_POINT ( 'NONE',  ( 56.52885800925551507, 12.28784885070978916, 6.671513217819436292 ) ) ;
#60347=CARTESIAN_POINT ( 'NONE',  ( -128.1384526288950099, 47.98891607499719925, 30.94904902096297405 ) ) ;
#60353=VECTOR ( 'NONE', #39283, 1000.000000000000000 ) ;
#60355=CARTESIAN_POINT ( 'NONE',  ( 94.12988949694080532, 22.11811104795074812, -69.93042459641294784 ) ) ;
#60358=B_SPLINE_CURVE_WITH_KNOTS ( 'NONE', 3,
 ( #7583, #7918, #12855, #55756, #18471, #39919, #13201, #9294, #41650, #25489, #24103, #30757, #8263, #46929, #35342, #40270, #46575, #68392, #24452, #19155, #20193, #63106, #61718, #52205, #13543, #50821, #56439, #40609, #4021, #57832, #57147, #67705, #62060, #30405, #19498, #51524, #13875, #62419, #62767, #40960, #3329, #9647, #45541, #56801, #8618, #35696 ),
 .UNSPECIFIED., .F., .F.,
 ( 4, 2, 2, 2, 2, 2, 2, 2, 2, 2, 2, 2, 2, 2, 2, 2, 2, 2, 2, 2, 2, 2, 4 ),
 ( 0.02420077021543442022, 0.02572112563160194876, 0.02648130333968569741, 0.02724148104776944260, 0.02876183646393689827, 0.02952201417202062611, 0.03028219188010435742, 0.03180254729627184085, 0.03332290271243932428, 0.03408308042052305559, 0.03484325812860678689, 0.03636361354477425645, 0.03712379125285798775, 0.03788396896094172600, 0.03864414666902546425, 0.03940432437710919555, 0.04092467979327665123, 0.04244503520944410691, 0.04396539062561155564, 0.04548574604177901132, 0.04624592374986272181, 0.04700610145794643924, 0.04852645687411390185 ),
 .UNSPECIFIED. ) ;
#60365=CARTESIAN_POINT ( 'NONE',  ( 41.09671232177015554, 8.635892912882342287, 30.10370141709571712 ) ) ;
#60366=CARTESIAN_POINT ( 'NONE',  ( 201.9777685760379313, 102.6876480786892927, -23.98289206748827951 ) ) ;
#60371=FACE_OUTER_BOUND ( 'NONE', #25260, .T. ) ;
#60374=CARTESIAN_POINT ( 'NONE',  ( -25.98312968277008039, 8.759224980175263298, -47.96912024656418794 ) ) ;
#60377=CARTESIAN_POINT ( 'NONE',  ( -47.68562151781910785, 12.82916850665305475, -95.00000000000133582 ) ) ;
#60380=AXIS2_PLACEMENT_3D ( 'NONE', #6540, #37496, #55062 ) ;
#60381=CARTESIAN_POINT ( 'NONE',  ( -81.95806712579563680, 23.60263724764760696, 84.86105897464825887 ) ) ;
#60382=CARTESIAN_POINT ( 'NONE',  ( -86.06016868996614733, 25.27707703029501118, 66.04626657972286807 ) ) ;
#60383=CARTESIAN_POINT ( 'NONE',  ( 128.0540543950622236, 39.18660671946769014, 41.78878589093363161 ) ) ;
#60384=CARTESIAN_POINT ( 'NONE',  ( 32.29578462738146527, 8.602609172809797755, 12.98030737452486072 ) ) ;
#60386=CARTESIAN_POINT ( 'NONE',  ( -99.98584758882476820, 32.75338129098886952, -22.82608027691124519 ) ) ;
#60388=CARTESIAN_POINT ( 'NONE',  ( 207.5654265768424693, 110.3565116837594076, 83.44490759518619427 ) ) ;
#60390=ORIENTED_EDGE ( 'NONE', *, *, #57432, .T. ) ;
#60393=CARTESIAN_POINT ( 'NONE',  ( -189.4248691432192970, 107.3461292335514656, -43.84368868221933724 ) ) ;
#60401=CARTESIAN_POINT ( 'NONE',  ( -166.7050147108375029, 81.70694330787516435, -38.28854392307332688 ) ) ;
#60402=CARTESIAN_POINT ( 'NONE',  ( -188.6739852773920632, 108.2139733222100517, -40.40546001351593475 ) ) ;
#60403=ORIENTED_EDGE ( 'NONE', *, *, #43755, .T. ) ;
#60404=CARTESIAN_POINT ( 'NONE',  ( -102.2801239173131052, 32.78103895658058065, 3.674523915951417141 ) ) ;
#60407=CARTESIAN_POINT ( 'NONE',  ( -143.8794621588508562, 59.54894433207191184, -20.43180592025295894 ) ) ;
#60408=CARTESIAN_POINT ( 'NONE',  ( -5.417282889646083177, 7.753782747238989970, -62.65547924408967617 ) ) ;
#60413=CARTESIAN_POINT ( 'NONE',  ( -61.10880364359509542, 17.43879918625642844, 6.541553347541163355 ) ) ;
#60414=CARTESIAN_POINT ( 'NONE',  ( 201.5903370237275283, 102.1785392640257868, -50.66542380412518298 ) ) ;
#60415=CARTESIAN_POINT ( 'NONE',  ( -150.5993571094983281, 66.43939758484178526, 30.79752979960735715 ) ) ;
#60416=CARTESIAN_POINT ( 'NONE',  ( 18.66025561752211104, 6.609375019058820300, -49.96014427081493636 ) ) ;
#60422=ORIENTED_EDGE ( 'NONE', *, *, #52864, .F. ) ;
#60425=CARTESIAN_POINT ( 'NONE',  ( 177.0110682437507990, 75.98481089748379702, 30.49479835804475059 ) ) ;
#60428=CARTESIAN_POINT ( 'NONE',  ( -12.78319349481552258, 8.274445259016799170, -64.11374738978491905 ) ) ;
#60434=VERTEX_POINT ( 'NONE', #34641 ) ;
#60436=CARTESIAN_POINT ( 'NONE',  ( -38.69408084385330682, 10.89529537250242974, -14.00704445308265633 ) ) ;
#60438=CARTESIAN_POINT ( 'NONE',  ( 129.1052153257903967, 39.78893484542955150, 69.67837425836049192 ) ) ;
#60440=EDGE_CURVE ( 'NONE', #10658, #26520, #43763, .T. ) ;
#60443=ORIENTED_EDGE ( 'NONE', *, *, #42697, .T. ) ;
#60445=CARTESIAN_POINT ( 'NONE',  ( -105.8683518445188554, 35.77995342500076248, 4.571401378338662447 ) ) ;
#60447=CARTESIAN_POINT ( 'NONE',  ( -36.37663950036512261, 10.45389057208229033, -37.15064349336959282 ) ) ;
#60448=CARTESIAN_POINT ( 'NONE',  ( -94.77657963819960685, 29.12969147113658153, 91.47122548580749424 ) ) ;
#60449=CARTESIAN_POINT ( 'NONE',  ( -143.2471548081022661, 59.04577938365764567, 34.05900480430268829 ) ) ;
#60450=CARTESIAN_POINT ( 'NONE',  ( -131.3154845336012500, 50.16828105866952114, 59.75965407406295782 ) ) ;
#60451=CARTESIAN_POINT ( 'NONE',  ( -72.35078170365746075, 21.08176362823952843, -19.82354011342815880 ) ) ;
#60453=CARTESIAN_POINT ( 'NONE',  ( 82.14449817946436383, 17.93919511903895625, 70.07299682206928537 ) ) ;
#60454=B_SPLINE_CURVE_WITH_KNOTS ( 'NONE', 3,
 ( #50591, #8737, #19978, #20306, #3447, #62180, #47043, #51639, #24909, #3109, #24571, #61826, #15038, #67473, #14000, #52320, #63228, #40722, #57945, #41771, #31227, #41429, #46341, #52658, #57609, #4483, #13650, #30526, #56559, #9420, #9765, #56920, #9073, #36494, #25609, #25941, #36150, #8385, #35104, #47373, #19620, #18934, #40383, #35456, #29829, #62541 ),
 .UNSPECIFIED., .F., .F.,
 ( 4, 2, 2, 2, 2, 2, 2, 2, 2, 2, 2, 2, 2, 2, 2, 2, 2, 2, 2, 2, 2, 2, 4 ),
 ( 0.02989107162308287519, 0.03170280136394029724, 0.03351453110479772624, 0.03532626084565514829, 0.03713799058651257035, 0.03894972032736999934, 0.03985558519779868608, 0.04076145006822737282, 0.04166731493865606650, 0.04257317980908476018, 0.04347904467951344692, 0.04438490954994213367, 0.04529077442037082735, 0.04619663929079951409, 0.04710250416122820777, 0.04800836903165689451, 0.04891423390208558819, 0.04982009877251427493, 0.05163182851337158596, 0.05344355825422892475, 0.05525528799508625660, 0.05706701773594359539, 0.05887874747680092724 ),
 .UNSPECIFIED. ) ;
#60455=ORIENTED_EDGE ( 'NONE', *, *, #23919, .F. ) ;
#60457=CARTESIAN_POINT ( 'NONE',  ( 34.45500533947589616, 7.817363290423890554, 43.07223163450435521 ) ) ;
#60462=CARTESIAN_POINT ( 'NONE',  ( -124.1007047332778228, 46.52282960291165637, 57.66784334201018680 ) ) ;
#60464=CARTESIAN_POINT ( 'NONE',  ( 150.0973882686025433, 52.13852366454153042, -42.22282177753791643 ) ) ;
#60465=AXIS2_PLACEMENT_3D ( 'NONE', #19518, #18139, #67379 ) ;
#60467=ORIENTED_EDGE ( 'NONE', *, *, #46843, .T. ) ;
#60471=CYLINDRICAL_SURFACE ( 'NONE', #65713, 7.500000000000013323 ) ;
#60472=CARTESIAN_POINT ( 'NONE',  ( -149.5074843970971017, 65.50121172469319220, -49.81283053149199702 ) ) ;
#60474=CARTESIAN_POINT ( 'NONE',  ( -85.46258339457286013, 25.02772366257408265, 34.73610256809621433 ) ) ;
#60475=CARTESIAN_POINT ( 'NONE',  ( 152.8672128926848188, 55.41186463791517269, -76.39475647682806425 ) ) ;
#60476=CARTESIAN_POINT ( 'NONE',  ( 43.96062659677686213, 10.06332325923986204, 43.38939548662082046 ) ) ;
#60478=ORIENTED_EDGE ( 'NONE', *, *, #24012, .T. ) ;
#60482=CARTESIAN_POINT ( 'NONE',  ( -189.2776534485022069, 107.1424877329940841, -95.00000000000133582 ) ) ;
#60486=CARTESIAN_POINT ( 'NONE',  ( 138.0620293754376178, 45.21335672767177272, 84.48092758364141730 ) ) ;
#60490=VERTEX_POINT ( 'NONE', #27945 ) ;
#60491=CARTESIAN_POINT ( 'NONE',  ( -120.4816138481825192, 43.03185659245512085, -74.47313363230125560 ) ) ;
#60493=ORIENTED_EDGE ( 'NONE', *, *, #54760, .T. ) ;
#60497=CARTESIAN_POINT ( 'NONE',  ( 139.2794027252094509, 45.99190465195508892, 15.36930535624699523 ) ) ;
#60503=CARTESIAN_POINT ( 'NONE',  ( 15.29293866748104769, 6.484959508098437020, 45.01470767270525641 ) ) ;
#60505=CARTESIAN_POINT ( 'NONE',  ( 133.8566784816069344, 41.42467568809808398, -89.71241211332301191 ) ) ;
#60507=ORIENTED_EDGE ( 'NONE', *, *, #61770, .F. ) ;
#60508=CARTESIAN_POINT ( 'NONE',  ( -124.1007047332778512, 46.52282960291164216, 3.978742161082801321 ) ) ;
#60510=CARTESIAN_POINT ( 'NONE',  ( 88.52345267551652341, 20.07594890262054932, 3.106688155335522339 ) ) ;
#60513=ORIENTED_EDGE ( 'NONE', *, *, #9005, .T. ) ;
#60516=CARTESIAN_POINT ( 'NONE',  ( 156.5977259323288990, 56.97512126940429056, 29.44731887063822739 ) ) ;
#60517=CARTESIAN_POINT ( 'NONE',  ( 65.40383840050414221, 14.27443447873231719, 30.18673279204580595 ) ) ;
#60518=CARTESIAN_POINT ( 'NONE',  ( -126.7989199172159829, 47.09198523267867387, -23.02839162617069491 ) ) ;
#60519=CARTESIAN_POINT ( 'NONE',  ( -142.8209151613836241, 58.70887234856630243, -92.57052796546220463 ) ) ;
#60520=CARTESIAN_POINT ( 'NONE',  ( 126.6395826915640015, 37.23416510613625974, -72.42523722532835961 ) ) ;
#60521=EDGE_CURVE ( 'NONE', #30354, #39251, #7895, .T. ) ;
#60523=CARTESIAN_POINT ( 'NONE',  ( 140.2200249818745021, 46.60103563593128229, -74.34575589100958837 ) ) ;
#60527=EDGE_CURVE ( 'NONE', #57935, #57426, #43302, .T. ) ;
#60528=DIRECTION ( 'NONE',  ( 0.000000000000000000, 0.000000000000000000, 1.000000000000000000 ) ) ;
#60530=FACE_OUTER_BOUND ( 'NONE', #60626, .T. ) ;
#60531=CARTESIAN_POINT ( 'NONE',  ( -34.74023699876256899, 11.17830703027882677, 30.96454232188382605 ) ) ;
#60532=CARTESIAN_POINT ( 'NONE',  ( -142.5087559769085317, 59.74468185400779419, -12.71953806562390810 ) ) ;
#60534=DIRECTION ( 'NONE',  ( 0.000000000000000000, 0.000000000000000000, 1.000000000000000000 ) ) ;
#60537=CARTESIAN_POINT ( 'NONE',  ( -72.09647865251525900, 19.92687487589685702, -92.68025296393560097 ) ) ;
#60539=CARTESIAN_POINT ( 'NONE',  ( 117.6916924104495763, 32.48309187151380684, 11.28248544281732002 ) ) ;
#60542=CARTESIAN_POINT ( 'NONE',  ( -95.63694837622348643, 30.64472169584719907, -39.02429480595472455 ) ) ;
#60546=CARTESIAN_POINT ( 'NONE',  ( 109.6443462180100425, 29.71354171299205049, 83.31739449737001735 ) ) ;
#60547=CARTESIAN_POINT ( 'NONE',  ( 181.0840389613909736, -170.0000000000000000, -16.88050707541594164 ) ) ;
#60551=CARTESIAN_POINT ( 'NONE',  ( -188.6739852773920632, 108.2139733222100375, -70.66125817296374123 ) ) ;
#60553=ORIENTED_EDGE ( 'NONE', *, *, #40963, .F. ) ;
#60555=CARTESIAN_POINT ( 'NONE',  ( 178.4027079424739384, 75.93756746109792743, 70.66078313421148493 ) ) ;
#60557=CARTESIAN_POINT ( 'NONE',  ( -167.6566265204789943, 82.70140535081092992, 70.30913300738275495 ) ) ;
#60560=CARTESIAN_POINT ( 'NONE',  ( -125.8938041572051389, -170.0000000000000000, -69.25825448869763079 ) ) ;
#60561=ORIENTED_EDGE ( 'NONE', *, *, #20097, .T. ) ;
#60563=CARTESIAN_POINT ( 'NONE',  ( 93.87650740736114585, 23.09802612281734469, 8.371155946943980908 ) ) ;
#60564=CARTESIAN_POINT ( 'NONE',  ( 17.48988570800758424, 7.568061572928497682, -35.71044138032643644 ) ) ;
#60567=CARTESIAN_POINT ( 'NONE',  ( 212.1700216741375300, 117.1889356120871639, -17.70906844655045376 ) ) ;
#60569=FACE_BOUND ( 'NONE', #7847, .T. ) ;
#60570=CARTESIAN_POINT ( 'NONE',  ( -58.33245019990695823, 15.58496056636070115, -35.95393952762761813 ) ) ;
#60573=LINE ( 'NONE', #25387, #28932 ) ;
#60574=CARTESIAN_POINT ( 'NONE',  ( 88.98820631332499431, 21.30618275724810218, -50.45717736827222666 ) ) ;
#60575=CARTESIAN_POINT ( 'NONE',  ( -49.12372073857199695, 14.20664392157176437, 60.04245956566853692 ) ) ;
#60576=DIRECTION ( 'NONE',  ( -0.000000000000000000, 1.000000000000000000, -0.000000000000000000 ) ) ;
#60579=CYLINDRICAL_SURFACE ( 'NONE', #22099, 7.500000000000020428 ) ;
#60580=ORIENTED_EDGE ( 'NONE', *, *, #59918, .T. ) ;
#60581=CARTESIAN_POINT ( 'NONE',  ( 55.51597771111714508, 11.05737652677078664, 10.96812083458806697 ) ) ;
#60582=EDGE_CURVE ( 'NONE', #37469, #34631, #33242, .T. ) ;
#60586=CARTESIAN_POINT ( 'NONE',  ( 106.5030061485517763, 28.28936250057212476, -90.56079799092418625 ) ) ;
#60587=ORIENTED_EDGE ( 'NONE', *, *, #26295, .T. ) ;
#60589=CARTESIAN_POINT ( 'NONE',  ( -58.75378739419586793, 16.75118858561006974, -22.41342698957060620 ) ) ;
#60591=ORIENTED_EDGE ( 'NONE', *, *, #63859, .F. ) ;
#60596=CARTESIAN_POINT ( 'NONE',  ( 164.6598737201888127, 64.78038692612518901, 34.70323317510625571 ) ) ;
#60597=CARTESIAN_POINT ( 'NONE',  ( 106.6322547488295527, 28.34756922280617530, 3.675457982256730372 ) ) ;
#60598=CARTESIAN_POINT ( 'NONE',  ( 69.83617901654358207, 15.39919709983077389, 7.339238517795263483 ) ) ;
#60602=CARTESIAN_POINT ( 'NONE',  ( -14.65000983264446788, 8.442132792737769620, -93.38135813376521810 ) ) ;
#60606=CARTESIAN_POINT ( 'NONE',  ( 93.32455161385975373, 21.81511294875801710, 87.50465937977445208 ) ) ;
#60613=ORIENTED_EDGE ( 'NONE', *, *, #63779, .F. ) ;
#60614=CARTESIAN_POINT ( 'NONE',  ( -7.825402957745083654, 6.891034867348163395, -23.57352014148015584 ) ) ;
#60615=CARTESIAN_POINT ( 'NONE',  ( -167.1306301799594110, 82.15042288607379817, 87.48651795901140815 ) ) ;
#60616=CARTESIAN_POINT ( 'NONE',  ( -47.55360235114366674, 12.79819361309568926, -16.38438511314839374 ) ) ;
#60619=CARTESIAN_POINT ( 'NONE',  ( -56.97556689808915564, 16.24958672959845885, -35.46295881559763075 ) ) ;
#60622=CARTESIAN_POINT ( 'NONE',  ( -14.32241591711282247, 7.401556312061832621, 41.37047100563557933 ) ) ;
#60625=ORIENTED_EDGE ( 'NONE', *, *, #20097, .F. ) ;
#60626=EDGE_LOOP ( 'NONE', ( #33679, #29352, #67828, #41258 ) ) ;
#60627=CARTESIAN_POINT ( 'NONE',  ( -142.8556048422594813, 60.01994222009839319, 14.85110067941132961 ) ) ;
#60629=CARTESIAN_POINT ( 'NONE',  ( -32.72965438883313993, 10.82661681132672093, 83.98928369309581399 ) ) ;
#60633=CARTESIAN_POINT ( 'NONE',  ( -190.6985136298601731, 109.1272424661242582, 94.99999999999866418 ) ) ;
#60634=CARTESIAN_POINT ( 'NONE',  ( 138.5943620234099001, 45.55242290395134575, -22.51329138269814578 ) ) ;
#60637=EDGE_LOOP ( 'NONE', ( #40975, #40629, #9708, #13277 ) ) ;
#60639=CARTESIAN_POINT ( 'NONE',  ( -11.57808265946730231, 7.164483090579921054, 4.272735484984936605 ) ) ;
#60640=CARTESIAN_POINT ( 'NONE',  ( 33.44983424733139543, 7.709709042132400825, -65.37461540421082873 ) ) ;
#60649=CARTESIAN_POINT ( 'NONE',  ( 198.8732368717151644, 100.3103976497390590, -65.93875134692073914 ) ) ;
#60651=CARTESIAN_POINT ( 'NONE',  ( -5.183193881612056408, 7.740932022135016410, -35.89460273968080628 ) ) ;
#60652=CARTESIAN_POINT ( 'NONE',  ( 110.2429982417149290, 28.88204397445231209, 2.766663615273646570 ) ) ;
#60655=FACE_BOUND ( 'NONE', #14101, .T. ) ;
#60666=DIRECTION ( 'NONE',  ( 0.000000000000000000, 0.000000000000000000, 1.000000000000000000 ) ) ;
#60668=CARTESIAN_POINT ( 'NONE',  ( 186.2914852210160461, 84.03335794683924576, 85.09093861525570901 ) ) ;
#60671=B_SPLINE_CURVE_WITH_KNOTS ( 'NONE', 3,
 ( #1406, #27789, #1063, #43953, #17224, #33433, #54859, #6685, #17589, #28131, #39054, #60497, #20024, #30575, #3840, #14046, #3488, #35505, #62930, #40773, #40089, #45713, #41478, #52025, #4187, #56966, #30233, #61544, #62590, #24267, #61872, #25310, #51682, #41126, #8074, #40429, #19318, #29523, #14403, #13700, #35152, #9117, #13363, #50990, #2805, #67190, #8786, #24960 ),
 .UNSPECIFIED., .F., .F.,
 ( 4, 2, 2, 2, 2, 2, 2, 2, 2, 2, 2, 2, 2, 2, 2, 2, 2, 2, 2, 2, 2, 2, 2, 4 ),
 ( 0.000000000000000000, 0.001591515129442203210, 0.003183030258884406421, 0.003978787823605504231, 0.004774545388326602476, 0.006366060517768851006, 0.007957575647211098668, 0.009549090776653347198, 0.01034484834137447580, 0.01114060590609560440, 0.01193636347081673300, 0.01273212103553786334, 0.01432363616498011881, 0.01591515129442237775, 0.01671090885914350288, 0.01750666642386462801, 0.01830242398858576008, 0.01909818155330688522, 0.02068969668274918405, 0.02148545424747034041, 0.02228121181219149330, 0.02387272694163372622, 0.02466848450635488951, 0.02546424207107604240 ),
 .UNSPECIFIED. ) ;
#60672=FACE_OUTER_BOUND ( 'NONE', #27584, .T. ) ;
#60673=CARTESIAN_POINT ( 'NONE',  ( -176.3791001330698975, 90.82833141237287577, -62.28654758217901843 ) ) ;
#60674=EDGE_CURVE ( 'NONE', #27330, #31531, #31756, .T. ) ;
#60676=ORIENTED_EDGE ( 'NONE', *, *, #51937, .F. ) ;
#60680=DIRECTION ( 'NONE',  ( 0.000000000000000000, 0.000000000000000000, 1.000000000000000000 ) ) ;
#60684=CARTESIAN_POINT ( 'NONE',  ( -49.12372073857197563, 14.20664392157176259, -20.49119220572248423 ) ) ;
#60686=CARTESIAN_POINT ( 'NONE',  ( -124.3250225421925848, 45.46958056770282752, -8.231571376810528307 ) ) ;
#60688=CARTESIAN_POINT ( 'NONE',  ( -149.5074843970971017, 65.50121172469319220, -49.81283053149199702 ) ) ;
#60690=CARTESIAN_POINT ( 'NONE',  ( -130.2601666248127401, 49.43645820311487427, 85.70393383863903125 ) ) ;
#60691=ORIENTED_EDGE ( 'NONE', *, *, #18986, .F. ) ;
#60692=CARTESIAN_POINT ( 'NONE',  ( 86.14852828165525978, 19.25704475759650336, -35.82156419891170884 ) ) ;
#60693=AXIS2_PLACEMENT_3D ( 'NONE', #46611, #19890, #68748 ) ;
#60695=B_SPLINE_CURVE_WITH_KNOTS ( 'NONE', 3,
 ( #68487, #37501, #16399, #57931, #47030, #210, #20292, #47704, #69505, #69165, #4126, #53674, #41757, #37855, #30862, #42096, #42772, #63214, #20991, #15366 ),
 .UNSPECIFIED., .F., .F.,
 ( 4, 2, 2, 2, 2, 2, 2, 2, 2, 4 ),
 ( 0.009977836299145791815, 0.01121959191743023346, 0.01246134753571467683, 0.01308222534485689766, 0.01370310315399911848, 0.01494485877228356185, 0.01618661439056800350, 0.01742837000885244861, 0.01867012562713689372, 0.01991188124542133536 ),
 .UNSPECIFIED. ) ;
#60696=CARTESIAN_POINT ( 'NONE',  ( -132.6161619568759136, 51.08240647571224002, 34.78398694684950243 ) ) ;
#60697=CARTESIAN_POINT ( 'NONE',  ( 82.94816950786172072, 19.25538918181909054, 43.75103483649611036 ) ) ;
#60699=EDGE_CURVE ( 'NONE', #34184, #32490, #22392, .T. ) ;
#60700=CARTESIAN_POINT ( 'NONE',  ( 187.8959968237854241, 85.77553094678179946, -20.03028080268358835 ) ) ;
#60701=CARTESIAN_POINT ( 'NONE',  ( 141.0645618855931218, 45.95036951196543384, -18.81836596334719047 ) ) ;
#60703=CARTESIAN_POINT ( 'NONE',  ( 93.85846834761629509, 22.01563781856519952, -72.17934525255718370 ) ) ;
#60707=CARTESIAN_POINT ( 'NONE',  ( 39.40195752203892710, 8.409560354027400209, 29.91383430596324899 ) ) ;
#60709=DIRECTION ( 'NONE',  ( -0.000000000000000000, 1.000000000000000000, -0.000000000000000000 ) ) ;
#60712=CARTESIAN_POINT ( 'NONE',  ( 208.5884523568771840, 113.6152425727544824, -37.40009660611077891 ) ) ;
#60713=CARTESIAN_POINT ( 'NONE',  ( -71.26746920569853216, 20.70422440535243069, -70.71288310661476828 ) ) ;
#60714=CARTESIAN_POINT ( 'NONE',  ( -78.66644367742111399, 22.32174330031318377, -76.96000122218160300 ) ) ;
#60715=CARTESIAN_POINT ( 'NONE',  ( -26.50364027666004318, 8.832969329054181529, -48.48556182960913219 ) ) ;
#60719=CARTESIAN_POINT ( 'NONE',  ( -9.771516655894561865, 7.025139475821124080, -50.17770668640199716 ) ) ;
#60720=FACE_OUTER_BOUND ( 'NONE', #68243, .T. ) ;
#60722=CARTESIAN_POINT ( 'NONE',  ( 126.4318266066171645, 38.27072266789463839, 35.91859280786284359 ) ) ;
#60727=CARTESIAN_POINT ( 'NONE',  ( 61.09977118998601497, 13.26754120022605932, 30.05771525600105321 ) ) ;
#60731=CARTESIAN_POINT ( 'NONE',  ( 63.01563776193090405, 13.70579113808098271, 71.65751152968501003 ) ) ;
#60733=CARTESIAN_POINT ( 'NONE',  ( -189.8071159312682710, 107.8771087123620163, -44.99094141979524863 ) ) ;
#60736=CARTESIAN_POINT ( 'NONE',  ( 204.6977192012829789, 106.3443248447423315, 71.05227132923315025 ) ) ;
#60737=CARTESIAN_POINT ( 'NONE',  ( 132.0249343950657135, 41.49728247212332377, -9.346915333156639250 ) ) ;
#60738=EDGE_CURVE ( 'NONE', #16384, #9825, #21511, .T. ) ;
#60743=CARTESIAN_POINT ( 'NONE',  ( -36.38071096718370256, 11.47804921491337637, -37.15419882060332668 ) ) ;
#60746=CARTESIAN_POINT ( 'NONE',  ( -173.7825098940164992, 87.86624138172392406, 84.52333946395306441 ) ) ;
#60748=CARTESIAN_POINT ( 'NONE',  ( -121.2008155373973750, 43.48033530165983507, -48.28419163247083645 ) ) ;
#60750=CARTESIAN_POINT ( 'NONE',  ( 140.0012045870120687, -170.0000000000000000, 94.99999999999866418 ) ) ;
#60751=CARTESIAN_POINT ( 'NONE',  ( -5.412684891282534494, 7.753215344827985689, -76.88094471104368210 ) ) ;
#60755=CARTESIAN_POINT ( 'NONE',  ( 162.2792973920977317, 62.79117098392629259, -91.54424637048310842 ) ) ;
#60756=CARTESIAN_POINT ( 'NONE',  ( 197.2200752504832053, 96.62072041958364821, -43.16169500306578044 ) ) ;
#60757=ADVANCED_FACE ( 'NONE', ( #56952 ), #52010, .F. ) ;
#60761=VERTEX_POINT ( 'NONE', #9107 ) ;
#60762=CARTESIAN_POINT ( 'NONE',  ( 55.90536342106781120, 11.13510150712953717, 34.87586743684235557 ) ) ;
#60765=CARTESIAN_POINT ( 'NONE',  ( -73.09185868250601459, 20.27574131633382848, -10.72959749028603049 ) ) ;
#60766=CARTESIAN_POINT ( 'NONE',  ( -38.57591613063113556, 11.89740419135774196, -94.16128332851744176 ) ) ;
#60767=CARTESIAN_POINT ( 'NONE',  ( -9.765753193741732119, 8.033970690975921869, -77.01142990352218476 ) ) ;
#60768=VERTEX_POINT ( 'NONE', #4173 ) ;
#60769=CARTESIAN_POINT ( 'NONE',  ( -101.1578861705715724, 33.34056307617599657, 84.28663787432705590 ) ) ;
#60772=ORIENTED_EDGE ( 'NONE', *, *, #34254, .F. ) ;
#60774=CARTESIAN_POINT ( 'NONE',  ( 208.0306608271317259, 112.7988899307264887, -77.39258503760095209 ) ) ;
#60775=AXIS2_PLACEMENT_3D ( 'NONE', #65718, #55134, #43535 ) ;
#60776=CARTESIAN_POINT ( 'NONE',  ( -38.87848244732137459, 10.93141945332450504, -16.95606301243583758 ) ) ;
#60777=CARTESIAN_POINT ( 'NONE',  ( 156.0322512485978450, 56.54107760830848406, -89.94358864157470634 ) ) ;
#60778=CARTESIAN_POINT ( 'NONE',  ( -131.6253556217204732, 51.61436399519942597, 6.412036120678384243 ) ) ;
#60779=CARTESIAN_POINT ( 'NONE',  ( 17.73567516211397432, 7.577454475141602863, 57.09994424157939363 ) ) ;
#60782=ORIENTED_EDGE ( 'NONE', *, *, #69174, .T. ) ;
#60784=CARTESIAN_POINT ( 'NONE',  ( 204.6977192012829789, 106.3443248447423315, -90.01503221354893469 ) ) ;
#60785=CARTESIAN_POINT ( 'NONE',  ( -108.9145525555662033, 37.42858360505776005, 7.667561549411721522 ) ) ;
#60787=CARTESIAN_POINT ( 'NONE',  ( -37.07602570886410120, 10.58457435034603300, -47.78910661960291861 ) ) ;
#60788=CARTESIAN_POINT ( 'NONE',  ( -97.82004213277211591, 30.57222530530879823, 85.67048935340082494 ) ) ;
#60791=CARTESIAN_POINT ( 'NONE',  ( -77.71490760329790248, 23.03637365463982434, -23.22547527094106812 ) ) ;
#60793=CARTESIAN_POINT ( 'NONE',  ( 79.11678589158262298, 16.99307320450158443, 64.06522735529883050 ) ) ;
#60795=CARTESIAN_POINT ( 'NONE',  ( 39.40195752203892710, 8.409560354027400209, 29.91383430596324899 ) ) ;
#60796=B_SPLINE_CURVE_WITH_KNOTS ( 'NONE', 3,
 ( #14299, #57207, #25211, #46642, #68118, #41379, #62834, #14635, #9360, #30825, #6505, #59593, #11413, #54677, #27599, #5795, #37122, #53965, #5110, #32535, #49040, #43424, #881, #16698, #6141, #64549, #22329, #53281, #26912, #32884, #22678, #26571, #58914, #37813, #48009, #54318, #10727, #32201, #59260, #27249, #44115, #69472, #48684, #49394, #11072, #5456 ),
 .UNSPECIFIED., .F., .F.,
 ( 4, 2, 2, 2, 2, 2, 2, 2, 2, 2, 2, 2, 2, 2, 2, 2, 2, 2, 2, 2, 2, 2, 4 ),
 ( 0.000000000000000000, 0.001615199098318927107, 0.003230398196637854213, 0.004037997745797326440, 0.004845597294956798667, 0.006460796393275733580, 0.007268395942435232696, 0.008075995491594732678, 0.009691194589913694479, 0.01049879413907319099, 0.01130639368823268751, 0.01211399323739218402, 0.01292159278655168227, 0.01453679188487069784, 0.01615199098318971516, 0.01695959053234921340, 0.01776719008150871512, 0.01938238917982775325, 0.02099758827814678791, 0.02180518782730633820, 0.02261278737646588849, 0.02422798647478491274, 0.02584318557310393699 ),
 .UNSPECIFIED. ) ;
#60801=CARTESIAN_POINT ( 'NONE',  ( -48.32993240732255913, 12.98137013984325350, 14.33474380245380431 ) ) ;
#60805=ORIENTED_EDGE ( 'NONE', *, *, #27524, .T. ) ;
#60807=CARTESIAN_POINT ( 'NONE',  ( -152.9121563765243650, 67.12206067149027433, -8.781803752322767664 ) ) ;
#60814=CARTESIAN_POINT ( 'NONE',  ( 150.5744176759382924, 53.72473166688033075, -73.42946358852339017 ) ) ;
#60816=CARTESIAN_POINT ( 'NONE',  ( 42.71247067544612719, 9.879726907348450382, 30.67953867783917232 ) ) ;
#60818=CARTESIAN_POINT ( 'NONE',  ( 138.1919700334460401, 44.10401742531044533, -49.66122531802075457 ) ) ;
#60820=ORIENTED_EDGE ( 'NONE', *, *, #41787, .T. ) ;
#60825=CARTESIAN_POINT ( 'NONE',  ( 33.77444274891858811, 8.756048688386680823, -21.23933397304090676 ) ) ;
#60829=CARTESIAN_POINT ( 'NONE',  ( 139.3117261255414121, 46.01296213310618555, 85.54168116855211679 ) ) ;
#60839=CARTESIAN_POINT ( 'NONE',  ( 163.7464701930789204, 62.69993100427426214, -20.91664329413919887 ) ) ;
#60842=CARTESIAN_POINT ( 'NONE',  ( -129.1212007313910988, 49.87404947283614121, -89.31921607445420364 ) ) ;
#60846=DIRECTION ( 'NONE',  ( -0.000000000000000000, 1.000000000000000000, -0.000000000000000000 ) ) ;
#60847=CARTESIAN_POINT ( 'NONE',  ( 12.03194517566456234, 6.409266703743585758, 44.02472010739144537 ) ) ;
#60849=CARTESIAN_POINT ( 'NONE',  ( -59.57733000654214095, 15.94108165424591661, -75.56201074176625809 ) ) ;
#60850=CARTESIAN_POINT ( 'NONE',  ( 63.01563776193091826, -170.0000000000000000, 2.968410348757589023 ) ) ;
#60852=CARTESIAN_POINT ( 'NONE',  ( -142.3393481102175429, 58.33014244976923379, -71.38071900410970727 ) ) ;
#60853=CARTESIAN_POINT ( 'NONE',  ( 93.71772995179817656, 21.96265635001559957, 12.83079813077724118 ) ) ;
#60855=ORIENTED_EDGE ( 'NONE', *, *, #34158, .F. ) ;
#60857=CARTESIAN_POINT ( 'NONE',  ( 56.32277010625402625, 12.24595634619651641, 87.60108806781256874 ) ) ;
#60858=CARTESIAN_POINT ( 'NONE',  ( 38.43102714813441878, 9.298961820315049920, 29.96078491149901524 ) ) ;
#60859=CARTESIAN_POINT ( 'NONE',  ( 63.49941241090382960, 13.81848793187417535, 29.81296093922127000 ) ) ;
#60860=CARTESIAN_POINT ( 'NONE',  ( -131.6133495896317243, 50.37677745548732133, -10.71135871446110954 ) ) ;
#60861=CARTESIAN_POINT ( 'NONE',  ( 154.6667526376337207, 55.50347409140649546, 70.71395942990847061 ) ) ;
#60862=CARTESIAN_POINT ( 'NONE',  ( 128.0568017572568635, 38.03085713813909052, -75.14985521657804668 ) ) ;
#60864=CARTESIAN_POINT ( 'NONE',  ( 141.3400002717723396, 47.33399859146519617, -69.80018433290322832 ) ) ;
#60865=CARTESIAN_POINT ( 'NONE',  ( -145.5195986658808920, 62.16746116576787529, -75.51344088246251829 ) ) ;
#60868=CARTESIAN_POINT ( 'NONE',  ( -150.3850953947692233, 66.25368649589884740, -34.85138302416307710 ) ) ;
#60869=CARTESIAN_POINT ( 'NONE',  ( 205.5130322755755117, 109.1888880665735684, -9.481380442157899324 ) ) ;
#60870=CARTESIAN_POINT ( 'NONE',  ( -37.05762690088740641, 11.60527003175541338, 32.74225044994760481 ) ) ;
#60874=CARTESIAN_POINT ( 'NONE',  ( -5.888165822225389867, 7.780336669456523246, 44.86524469126863579 ) ) ;
#60876=CARTESIAN_POINT ( 'NONE',  ( -48.04019567818505010, 12.91272349839804789, -66.88950554398400072 ) ) ;
#60877=CARTESIAN_POINT ( 'NONE',  ( -5.412684891282529165, 7.753215344827987465, -23.19184353011629796 ) ) ;
#60879=CARTESIAN_POINT ( 'NONE',  ( -8.314488422519703548, 7.931352979988681717, 30.11558103944717857 ) ) ;
#60881=CARTESIAN_POINT ( 'NONE',  ( 115.7746371641014775, 31.52600568297706118, 15.35476345625890460 ) ) ;
#60882=CARTESIAN_POINT ( 'NONE',  ( 46.10482416129922001, 10.39500475043931083, -93.43768358713884936 ) ) ;
#60883=ORIENTED_EDGE ( 'NONE', *, *, #25985, .T. ) ;
#60885=ORIENTED_EDGE ( 'NONE', *, *, #59522, .T. ) ;
#60888=CARTESIAN_POINT ( 'NONE',  ( 82.12277968641505765, 18.98848723477810907, -64.15117521669343148 ) ) ;
#60891=CARTESIAN_POINT ( 'NONE',  ( -55.05276343752909440, 14.68156374112637508, 18.47277718246750311 ) ) ;
#60892=CLOSED_SHELL ( 'NONE', ( #15598, #9796, #39080, #22866, #42316, #39159, #217, #9886, #64903, #7204, #41636, #37066, #14669, #19672, #20710, #39939, #35019, #52790, #11668, #7698, #41625, #38406, #60182, #48025, #23904, #5956, #32236, #55659, #46880, #40279, #39969, #7341, #42719, #39163, #7880, #25575, #37787, #20619, #59669, #63463, #21646, #65018, #62342, #2973, #2384, #28111, #37958, #46289, #30093, #50661, #15639, #36170, #25411, #9913, #26120, #7136, #26375, #25206, #49943, #57521, #36466, #21839, #34239, #9090, #44048, #25096, #11082, #34409, #67664, #4291, #6162, #25570, #32948, #33055, #11512, #51327, #49078, #26847, #23756, #17511, #38990, #4009, #19272, #57989, #2158, #13734, #9456, #50244, #45652, #45192, #58990, #48707, #34642, #34228, #38917, #45503, #27447, #4707, #65246, #54026, #55363, #53843, #14309, #10147, #46744, #39323, #21259, #8576, #2630, #50687, #64409, #37564, #14157, #57273, #31512, #49512, #4535, #2784, #25262, #14378, #8922, #38672, #45091, #11410, #47631, #55453, #48962, #51444, #34518, #22687, #35600, #37932, #48242, #64467, #23817, #29001, #57208, #36925, #54523, #61853, #6765, #5094, #56815, #20933, #63306, #61407, #49881, #46053, #48162, #12322, #40243, #46775, #42913, #4207, #23293, #23539, #6940, #24934, #17539, #65421, #10730, #49748, #45501, #42249, #43416, #27541, #28095, #25495, #57903, #55106, #67661, #28322, #29535, #11345, #23586, #42557, #13105, #45526, #50301, #59338, #62247, #53284, #63444, #25466, #8501, #30987, #61554, #46453, #59600, #21444, #24413, #26833, #42010, #1205, #18907, #63520, #55414, #10247, #8533, #8186, #2623, #51296, #54771, #42504, #31536, #40499, #59445, #44216, #50637, #9768, #19298, #19434, #69351, #52787, #2136, #40326, #44943, #39869, #24158, #40181, #54153, #20492, #58422, #4056, #45925, #7958, #68323, #32069, #42484, #35377, #56415, #3404, #42647, #33548, #27610, #61408, #57183, #48423, #58909, #2966, #51530, #40317, #53484, #46844, #65362, #60757, #8100, #4615, #29944, #68731, #69080, #25739, #58427, #58047, #57794, #61617, #52956, #2244, #62160, #39618, #4068, #10, #5306, #56002, #43262, #32719, #12985, #40339, #23620, #16036, #20380, #14751, #24797, #14548, #8820, #68751, #13031, #21655, #24387, #64160, #9878, #20032, #43106, #685, #11108, #28922, #48405, #25185, #57190, #1179, #56082, #21622, #67377, #8276, #51954, #8180, #36281, #57662, #17724, #58592, #40064, #33506, #61012 ) ) ;
#60894=CARTESIAN_POINT ( 'NONE',  ( -7.825402957745087207, -170.0000000000000000, 10.77103044898353090 ) ) ;
#60895=CARTESIAN_POINT ( 'NONE',  ( -118.5151419614604436, 43.00218563933585614, -14.19961787797135422 ) ) ;
#60898=CARTESIAN_POINT ( 'NONE',  ( 39.40195752203892710, 8.409560354027387774, -89.30891864635511013 ) ) ;
#60900=CARTESIAN_POINT ( 'NONE',  ( 173.6012773665504483, 71.36035397668607061, 63.06485450500365175 ) ) ;
#60902=CARTESIAN_POINT ( 'NONE',  ( -169.1122507277982550, 84.24359299875004581, 58.81210775617142872 ) ) ;
#60904=B_SPLINE_CURVE_WITH_KNOTS ( 'NONE', 3,
 ( #29116, #3083, #62515, #3421, #35082, #35785, #24197, #8360, #40695, #45640, #30163, #56533, #24881, #46318, #51272, #56895, #18216, #13623, #56185, #66767, #67794, #29810, #39666, #51612, #23845, #67118, #7671, #8710, #50566, #19241, #45982, #45285, #19592, #2385, #40357, #61120, #57234, #41056, #18910, #67450, #34408, #9049, #62153, #55851, #61805 ),
 .UNSPECIFIED., .F., .F.,
 ( 4, 2, 2, 1, 2, 2, 2, 2, 2, 2, 2, 2, 2, 2, 2, 2, 2, 2, 2, 2, 2, 2, 4 ),
 ( 0.02345095402629350165, 0.02491692321306680433, 0.02564990780645345914, 0.02638289239984011048, 0.02711587699322676182, 0.02784886158661341315, 0.02931483077338671930, 0.03004781536677335330, 0.03078079996015998382, 0.03224676914693325180, 0.03297975374031988927, 0.03371273833370651979, 0.03517870752047982941, 0.03664467670725313903, 0.03737766130063981118, 0.03811064589402649028, 0.03957661508079979990, 0.04104258426757310951, 0.04250855345434641913, 0.04324153804773307741, 0.04397452264111972875, 0.04544049182789304531, 0.04690646101466636186 ),
 .UNSPECIFIED. ) ;
#60908=CARTESIAN_POINT ( 'NONE',  ( 102.7446498997620097, 26.65764321315730356, -43.95904520983128094 ) ) ;
#60909=CARTESIAN_POINT ( 'NONE',  ( 173.9832054143776077, 71.71542822834034325, -95.00000000000133582 ) ) ;
#60910=CARTESIAN_POINT ( 'NONE',  ( -78.66644367742111399, 22.32174330031318021, -23.27090004125422595 ) ) ;
#60912=CARTESIAN_POINT ( 'NONE',  ( 212.0850679406004247, 117.0583048437722056, -15.64194342746143640 ) ) ;
#60913=FACE_BOUND ( 'NONE', #29133, .T. ) ;
#60917=ORIENTED_EDGE ( 'NONE', *, *, #65, .F. ) ;
#60919=CARTESIAN_POINT ( 'NONE',  ( 87.59078297315397776, 20.81577753000345510, -50.77505834181354061 ) ) ;
#60922=CARTESIAN_POINT ( 'NONE',  ( -174.7817412490652771, 90.52199442492062076, 4.151215324986693211 ) ) ;
#60923=CARTESIAN_POINT ( 'NONE',  ( 207.4566510040494620, 111.9649643341356011, 56.57504234372401442 ) ) ;
#60924=EDGE_CURVE ( 'NONE', #19164, #31197, #8950, .T. ) ;
#60926=FACE_OUTER_BOUND ( 'NONE', #65170, .T. ) ;
#60930=CARTESIAN_POINT ( 'NONE',  ( -62.54085973597666026, 16.81797209566546769, 64.17062851049894334 ) ) ;
#60932=VECTOR ( 'NONE', #52319, 1000.000000000000000 ) ;
#60934=ORIENTED_EDGE ( 'NONE', *, *, #42307, .T. ) ;
#60937=CARTESIAN_POINT ( 'NONE',  ( 93.32228019177716760, 22.88890999585039410, -73.55979981550770219 ) ) ;
#60940=VERTEX_POINT ( 'NONE', #22071 ) ;
#60941=CARTESIAN_POINT ( 'NONE',  ( 41.09759788073309039, 9.651672055033845510, 71.56824425796526157 ) ) ;
#60942=CARTESIAN_POINT ( 'NONE',  ( 158.3516718297675823, 59.61984652322053080, 29.44820441190890037 ) ) ;
#60943=CARTESIAN_POINT ( 'NONE',  ( -152.9143627383494959, 68.46626892668652431, -62.46033273451909196 ) ) ;
#60944=CARTESIAN_POINT ( 'NONE',  ( 65.40383840050414221, 14.27443447873230120, 3.342182201582107659 ) ) ;
#60947=CARTESIAN_POINT ( 'NONE',  ( -54.08488990389049889, 15.46443908526321742, -50.16924448875967357 ) ) ;
#60948=CARTESIAN_POINT ( 'NONE',  ( 60.61895554631703220, 13.15982272268128384, -36.09744376541886623 ) ) ;
#60949=CARTESIAN_POINT ( 'NONE',  ( -133.3944793432480083, 52.87251459353621641, -15.31422958618754748 ) ) ;
#60951=CARTESIAN_POINT ( 'NONE',  ( 116.9200705848630548, 32.09536795999726166, -13.12392903560524005 ) ) ;
#60952=CARTESIAN_POINT ( 'NONE',  ( 83.49107459963974520, 18.37327588711363191, 84.05685319569637670 ) ) ;
#60957=CARTESIAN_POINT ( 'NONE',  ( 45.49006904354232006, 9.279592366778883772, 6.182336992882302873 ) ) ;
#60958=CARTESIAN_POINT ( 'NONE',  ( -180.4741487479101352, 97.29837986977219089, 93.66950218727245669 ) ) ;
#60960=EDGE_CURVE ( 'NONE', #56594, #14354, #50929, .T. ) ;
#60961=CARTESIAN_POINT ( 'NONE',  ( 103.0103829243728910, 25.67737053862327556, -14.52816394246318055 ) ) ;
#60962=CARTESIAN_POINT ( 'NONE',  ( 198.8687991397275994, 98.67887821384411495, 5.136872697827199019 ) ) ;
#60964=DIRECTION ( 'NONE',  ( 0.000000000000000000, -1.000000000000000000, 0.000000000000000000 ) ) ;
#60966=CARTESIAN_POINT ( 'NONE',  ( -14.55390976651257162, 7.422979442794212623, 34.29323620107704329 ) ) ;
#60969=LINE ( 'NONE', #22292, #59813 ) ;
#60972=CARTESIAN_POINT ( 'NONE',  ( -149.5074843970971017, 64.17983161892348676, 3.876270649435373361 ) ) ;
#60973=CARTESIAN_POINT ( 'NONE',  ( 184.3966782763552033, 83.48172388049823667, -77.31299941553588440 ) ) ;
#60974=CARTESIAN_POINT ( 'NONE',  ( -169.1116812882275724, 84.24296059722693997, 44.67583165595225125 ) ) ;
#60975=CARTESIAN_POINT ( 'NONE',  ( -101.8191498210054675, 32.54686850610960391, -50.01457726497592660 ) ) ;
#60978=DIRECTION ( 'NONE',  ( 0.000000000000000000, -1.000000000000000000, 0.000000000000000000 ) ) ;
#60979=CARTESIAN_POINT ( 'NONE',  ( 136.1037846510193106, 43.98155406734452555, -9.508421591050250754 ) ) ;
#60987=CARTESIAN_POINT ( 'NONE',  ( -14.55390976651258050, 7.422979442794215288, 7.448685610613371644 ) ) ;
#60990=CARTESIAN_POINT ( 'NONE',  ( 60.62939143133410624, 12.13148391928980807, -23.50308998565268936 ) ) ;
#60991=EDGE_CURVE ( 'NONE', #26264, #32665, #61102, .T. ) ;
#60994=CARTESIAN_POINT ( 'NONE',  ( -48.99162761293256807, 13.13973062091723776, 33.39305727236687460 ) ) ;
#60996=EDGE_LOOP ( 'NONE', ( #53644, #63651, #33250, #5849 ) ) ;
#60997=CARTESIAN_POINT ( 'NONE',  ( -55.05276343752909440, 15.72344139423348786, -77.06087458892358200 ) ) ;
#61002=CARTESIAN_POINT ( 'NONE',  ( -173.1211646369891639, 87.12891641440852197, -88.40105834567665966 ) ) ;
#61004=FACE_BOUND ( 'NONE', #14272, .T. ) ;
#61006=EDGE_CURVE ( 'NONE', #10264, #52549, #58150, .T. ) ;
#61007=CARTESIAN_POINT ( 'NONE',  ( -4.504169684898452708, 6.697401007565304099, 71.18915580831600209 ) ) ;
#61010=CARTESIAN_POINT ( 'NONE',  ( 180.6710448012268841, 78.18844465372406205, 29.30859410551140698 ) ) ;
#61012=ADVANCED_FACE ( 'NONE', ( #50887 ), #28746, .F. ) ;
#61015=CARTESIAN_POINT ( 'NONE',  ( 110.2429982417149574, -170.0000000000000000, 17.76666361527367499 ) ) ;
#61017=CARTESIAN_POINT ( 'NONE',  ( 39.40195752203891999, 9.424259417798147354, -35.61981746542776506 ) ) ;
#61018=CARTESIAN_POINT ( 'NONE',  ( 187.7243171268374056, 85.58745653499732953, 86.99151838653519064 ) ) ;
#61020=VERTEX_POINT ( 'NONE', #51591 ) ;
#61021=CARTESIAN_POINT ( 'NONE',  ( 177.0075766083211875, 74.58167636505947939, -50.02476627610127480 ) ) ;
#61022=CARTESIAN_POINT ( 'NONE',  ( -180.2252811616041868, 95.40045830523435200, -66.63472952968756147 ) ) ;
#61025=CARTESIAN_POINT ( 'NONE',  ( 117.7442255600442849, 33.63739995216996448, 63.45684847541002682 ) ) ;
#61027=CARTESIAN_POINT ( 'NONE',  ( -3.868882431147346868, 6.665575841812235502, 4.394750620680583530 ) ) ;
#61029=DIRECTION ( 'NONE',  ( -0.000000000000000000, 1.000000000000000000, -0.000000000000000000 ) ) ;
#61030=CARTESIAN_POINT ( 'NONE',  ( 22.89837001126011984, 6.832355714161187699, -94.17556532809329894 ) ) ;
#61031=VECTOR ( 'NONE', #56392, 1000.000000000000000 ) ;
#61032=CARTESIAN_POINT ( 'NONE',  ( -47.56466076048272384, 13.83435953640667293, -16.36260880930676720 ) ) ;
#61035=AXIS2_PLACEMENT_3D ( 'NONE', #68534, #18963, #40757 ) ;
#61037=CARTESIAN_POINT ( 'NONE',  ( -72.77296415263758433, 21.23032531836538084, 6.408587851164161187 ) ) ;
#61039=CARTESIAN_POINT ( 'NONE',  ( -173.1211646369891355, 88.63826465341151106, -76.55650775521370122 ) ) ;
#61040=CARTESIAN_POINT ( 'NONE',  ( -123.7039169285859828, 45.06792368978931052, 84.61315978542810967 ) ) ;
#61042=CARTESIAN_POINT ( 'NONE',  ( 80.73012746365749592, 17.49169339352364361, -38.66384684947503558 ) ) ;
#61044=ORIENTED_EDGE ( 'NONE', *, *, #51765, .F. ) ;
#61046=CARTESIAN_POINT ( 'NONE',  ( 79.14113188808480004, 18.05280674635442750, 37.70299700396097364 ) ) ;
#61049=CARTESIAN_POINT ( 'NONE',  ( 140.5781926063689298, 45.63383190293698988, -20.01610080164386929 ) ) ;
#61051=CARTESIAN_POINT ( 'NONE',  ( -173.1211646369891355, 88.63826465341152527, -7.867406574286299303 ) ) ;
#61062=CARTESIAN_POINT ( 'NONE',  ( -102.7502407665687230, 33.01985383847077316, 72.36362509687882039 ) ) ;
#61063=CARTESIAN_POINT ( 'NONE',  ( -24.41864932425148282, 8.543938959778818898, -40.16677908042758105 ) ) ;
#61064=CARTESIAN_POINT ( 'NONE',  ( 164.8407099662995279, 63.61629583487390960, -71.88438285980473097 ) ) ;
#61067=VERTEX_POINT ( 'NONE', #35761 ) ;
#61068=B_SPLINE_CURVE_WITH_KNOTS ( 'NONE', 3,
 ( #20087, #3557, #25028, #41542, #8148, #40497, #56682, #67943, #62995, #29952, #62659, #36264, #57722, #2528, #45432, #66912, #18707, #61613 ),
 .UNSPECIFIED., .F., .F.,
 ( 4, 2, 2, 2, 2, 2, 2, 2, 4 ),
 ( 0.01001677236965714708, 0.01126784864425927138, 0.01251892491886139568, 0.01377000119346351997, 0.01502107746806564254, 0.01627215374266776857, 0.01752323001726989113, 0.01877430629187201716, 0.02002538256647413972 ),
 .UNSPECIFIED. ) ;
#61072=CARTESIAN_POINT ( 'NONE',  ( -77.47632222052990869, 21.87111359341350791, 84.17632590412091531 ) ) ;
#61073=CARTESIAN_POINT ( 'NONE',  ( -79.61931371420115511, 22.68640080971621487, 72.21703544022015819 ) ) ;
#61079=CARTESIAN_POINT ( 'NONE',  ( -95.05323930133207000, 30.36974142673411237, -13.59935561858418396 ) ) ;
#61081=CARTESIAN_POINT ( 'NONE',  ( 55.76255201544533691, 12.13275766515751997, 35.34123246681144082 ) ) ;
#61082=CARTESIAN_POINT ( 'NONE',  ( 35.34747263975754805, 7.916651221204775268, 84.78471632296681548 ) ) ;
#61085=CARTESIAN_POINT ( 'NONE',  ( 197.6319840686292082, 97.13072366387987699, -95.00000000000133582 ) ) ;
#61087=CARTESIAN_POINT ( 'NONE',  ( -14.92860730136983705, 8.468845235798738713, 8.351230680223016734 ) ) ;
#61090=CARTESIAN_POINT ( 'NONE',  ( 197.6316695787931508, 97.13022718399028577, 66.08436601712787706 ) ) ;
#61092=CARTESIAN_POINT ( 'NONE',  ( 133.4058733589413350, 42.32720528873925758, -24.17876034193200852 ) ) ;
#61095=PRODUCT_CONTEXT ( 'NONE', #46670, 'mechanical' ) ;
#61098=CARTESIAN_POINT ( 'NONE',  ( -32.41898580403142205, 10.77423026598439471, -35.36526679678951979 ) ) ;
#61099=EDGE_CURVE ( 'NONE', #67205, #17944, #12306, .T. ) ;
#61102=LINE ( 'NONE', #61448, #67024 ) ;
#61104=CARTESIAN_POINT ( 'NONE',  ( -118.5043919384111604, 41.81711884544880320, -41.10325547692050918 ) ) ;
#61106=CARTESIAN_POINT ( 'NONE',  ( -142.0902782307735208, 58.13494170556001706, -16.61472388644448372 ) ) ;
#61107=CARTESIAN_POINT ( 'NONE',  ( -1.862553927312061042, 7.582910205528087033, -74.33794145251196994 ) ) ;
#61111=CARTESIAN_POINT ( 'NONE',  ( 203.9181091394787586, 105.2759068139671115, -36.32593103262158252 ) ) ;
#61113=CARTESIAN_POINT ( 'NONE',  ( 23.09541709302173018, 6.844586979481618982, -44.72642228744273041 ) ) ;
#61114=CARTESIAN_POINT ( 'NONE',  ( -55.05276343752910151, 14.68156374112636620, 3.472777182467474244 ) ) ;
#61119=CARTESIAN_POINT ( 'NONE',  ( -173.1211646369891071, 88.63826465341152527, 18.97714401617737323 ) ) ;
#61120=CARTESIAN_POINT ( 'NONE',  ( 20.37135563017390893, 6.690359945346061821, -63.90633550731507029 ) ) ;
#61122=CARTESIAN_POINT ( 'NONE',  ( -15.32495246574475090, 8.506829480038508251, -70.26458035401391555 ) ) ;
#61123=ORIENTED_EDGE ( 'NONE', *, *, #43505, .F. ) ;
#61124=CARTESIAN_POINT ( 'NONE',  ( -94.85411614066488539, 30.27638713119805303, 92.81031322454776955 ) ) ;
#61125=CARTESIAN_POINT ( 'NONE',  ( -23.93933407965395332, 9.495050561681672718, 38.21205357566448413 ) ) ;
#61126=CARTESIAN_POINT ( 'NONE',  ( -78.66644367742111399, 23.39876645725287219, -50.11545063171791270 ) ) ;
#61129=ORIENTED_EDGE ( 'NONE', *, *, #7474, .F. ) ;
#61130=CARTESIAN_POINT ( 'NONE',  ( 212.0803491126036988, 118.9047894217573287, -69.30594524286756553 ) ) ;
#61134=CARTESIAN_POINT ( 'NONE',  ( 140.4641697461912884, 46.75994457266055093, 40.59688181447199185 ) ) ;
#61136=CARTESIAN_POINT ( 'NONE',  ( -173.5422248620772052, 89.11126078969412845, 45.82169460664104577 ) ) ;
#61138=CARTESIAN_POINT ( 'NONE',  ( 110.2429982417149574, -170.0000000000000000, -43.42243756565370205 ) ) ;
#61140=ORIENTED_EDGE ( 'NONE', *, *, #58570, .F. ) ;
#61145=CARTESIAN_POINT ( 'NONE',  ( -33.37566357177429666, 9.916833145467597532, -50.07922491613769012 ) ) ;
#61147=CARTESIAN_POINT ( 'NONE',  ( -142.3178993725749137, 58.31327888234797285, 40.42933480981873373 ) ) ;
#61154=CARTESIAN_POINT ( 'NONE',  ( 38.42384008295177722, 8.283891555743464252, 44.86569254733282008 ) ) ;
#61156=EDGE_CURVE ( 'NONE', #5523, #56201, #64551, .T. ) ;
#61157=CARTESIAN_POINT ( 'NONE',  ( 133.8566784816069060, 42.60093787723655367, 17.66579024853170310 ) ) ;
#61159=EDGE_CURVE ( 'NONE', #33533, #60292, #2223, .T. ) ;
#61161=CARTESIAN_POINT ( 'NONE',  ( -118.4709174626548531, 42.97515378817185194, 66.07066160974568447 ) ) ;
#61162=CARTESIAN_POINT ( 'NONE',  ( -102.2801239173131194, -170.0000000000000000, 3.674523915951417141 ) ) ;
#61167=CARTESIAN_POINT ( 'NONE',  ( -149.5074843970971017, 64.17983161892347255, -7.968279941028269420 ) ) ;
#61170=CARTESIAN_POINT ( 'NONE',  ( -62.54086041493280135, 17.86944394914988976, 65.15299748377630351 ) ) ;
#61171=CARTESIAN_POINT ( 'NONE',  ( 86.62931800182293784, -170.0000000000000000, -62.66611478937537782 ) ) ;
#61174=CARTESIAN_POINT ( 'NONE',  ( 150.5538013146980347, 53.70974888488127874, -67.55639953143700893 ) ) ;
#61175=CARTESIAN_POINT ( 'NONE',  ( -38.93922791710217979, 10.94334660650242341, 37.47454328655717148 ) ) ;
#61176=CARTESIAN_POINT ( 'NONE',  ( 140.4586216751745269, 45.55624550472995793, -47.09120538612899765 ) ) ;
#61178=ORIENTED_EDGE ( 'NONE', *, *, #11347, .F. ) ;
#61180=CARTESIAN_POINT ( 'NONE',  ( -122.7930600691577752, 44.48546375740916403, 44.96461390212944309 ) ) ;
#61182=CARTESIAN_POINT ( 'NONE',  ( 38.90907126433565111, 9.359889524363177671, -8.775266874964067654 ) ) ;
#61186=CARTESIAN_POINT ( 'NONE',  ( 127.3308700373269886, 38.77640327688543209, 86.99888605803015196 ) ) ;
#61189=CARTESIAN_POINT ( 'NONE',  ( 199.6029099983328479, 101.2457601186893612, -91.99728860495294214 ) ) ;
#61194=EDGE_LOOP ( 'NONE', ( #48299, #55966, #68599, #45605 ) ) ;
#61195=CARTESIAN_POINT ( 'NONE',  ( 160.9069879467681403, 60.37290772564308128, -23.46207914634777936 ) ) ;
#61196=CARTESIAN_POINT ( 'NONE',  ( -31.43908319763709969, 10.61114334766716638, -77.16174795566554678 ) ) ;
#61198=CARTESIAN_POINT ( 'NONE',  ( -133.3122825023497171, 52.81354457049841500, -95.00000000000133582 ) ) ;
#61199=PLANE ( 'NONE',  #35282 ) ;
#61200=ORIENTED_EDGE ( 'NONE', *, *, #16818, .F. ) ;
#61201=CARTESIAN_POINT ( 'NONE',  ( 164.1338586910085837, 64.33646242148854810, -13.32728364527724807 ) ) ;
#61204=CARTESIAN_POINT ( 'NONE',  ( -61.39252081892700375, 16.47343302442957835, -73.57560269778032591 ) ) ;
#61205=CARTESIAN_POINT ( 'NONE',  ( 133.4819570657469683, 41.19842572144921178, -89.71241211332299770 ) ) ;
#61206=ORIENTED_EDGE ( 'NONE', *, *, #50686, .F. ) ;
#61207=CARTESIAN_POINT ( 'NONE',  ( -142.0251973982164486, 58.08401473564114070, -69.74446058856305797 ) ) ;
#61210=CARTESIAN_POINT ( 'NONE',  ( 164.3577270662354124, 63.21061577643033758, -46.60488526209466187 ) ) ;
#61212=ORIENTED_EDGE ( 'NONE', *, *, #19516, .F. ) ;
#61214=EDGE_CURVE ( 'NONE', #36547, #18072, #49741, .T. ) ;
#61215=CARTESIAN_POINT ( 'NONE',  ( -102.2801239173131194, 33.91021738430207932, 45.51907450641513009 ) ) ;
#61217=CARTESIAN_POINT ( 'NONE',  ( 79.54836217416615796, 18.17815803851261336, -18.96166302950352645 ) ) ;
#61219=CARTESIAN_POINT ( 'NONE',  ( -132.0958200534848004, 50.71531800824801195, -19.79385869415553856 ) ) ;
#61220=CARTESIAN_POINT ( 'NONE',  ( 39.40195752203892710, 9.424259417798138472, -89.30891864635511013 ) ) ;
#61224=FACE_OUTER_BOUND ( 'NONE', #8999, .T. ) ;
#61225=VERTEX_POINT ( 'NONE', #65965 ) ;
#61228=CARTESIAN_POINT ( 'NONE',  ( -149.9475539515598257, 65.87716206616009629, -34.81283053149195439 ) ) ;
#61234=DIRECTION ( 'NONE',  ( -0.000000000000000000, 1.000000000000000000, -0.000000000000000000 ) ) ;
#61235=CARTESIAN_POINT ( 'NONE',  ( -49.11825192196926793, 13.17012322555987858, -64.94842763682078157 ) ) ;
#61238=CARTESIAN_POINT ( 'NONE',  ( -14.92860730136983882, 8.468845235798742266, 35.19578127068669460 ) ) ;
#61239=CARTESIAN_POINT ( 'NONE',  ( -59.94781924509479865, 16.04872117907065032, 16.66037302724637925 ) ) ;
#61246=CARTESIAN_POINT ( 'NONE',  ( 42.71680114082826663, 9.880016734137544887, -9.529744981248345681 ) ) ;
#61252=CARTESIAN_POINT ( 'NONE',  ( -77.02372450489328060, 21.70271995013164101, 57.44099635086979561 ) ) ;
#61253=CARTESIAN_POINT ( 'NONE',  ( -169.1005390226460179, 82.76152663947084420, 71.51309903033511262 ) ) ;
#61259=CARTESIAN_POINT ( 'NONE',  ( 105.4134760436918583, 27.80903124201758558, 69.71480060533734502 ) ) ;
#61263=CARTESIAN_POINT ( 'NONE',  ( 88.53025347111699261, 21.14438024052373422, 3.096674985598131258 ) ) ;
#61264=CARTESIAN_POINT ( 'NONE',  ( 22.15926701483428474, 7.796117250416237709, -39.05393624471034286 ) ) ;
#61267=CARTESIAN_POINT ( 'NONE',  ( 210.9747454890631388, 115.3673079504856105, -12.86836890806030276 ) ) ;
#61268=FACE_BOUND ( 'NONE', #14442, .T. ) ;
#61272=CARTESIAN_POINT ( 'NONE',  ( 86.62931800182293784, 20.48449268398422873, -50.82156419891174437 ) ) ;
#61273=CARTESIAN_POINT ( 'NONE',  ( 38.91512155099545112, 9.360679678889628264, -77.46436805589146957 ) ) ;
#61275=CARTESIAN_POINT ( 'NONE',  ( 211.8382652195005846, 118.5282575235989384, 65.86877708187445535 ) ) ;
#61286=EDGE_LOOP ( 'NONE', ( #27092, #60591 ) ) ;
#61288=CARTESIAN_POINT ( 'NONE',  ( -83.52505811737952968, 24.23179517241435832, -75.19473686439705773 ) ) ;
#61289=CARTESIAN_POINT ( 'NONE',  ( -62.55184817504198946, 17.87278652436698323, -16.38738335002791047 ) ) ;
#61290=CARTESIAN_POINT ( 'NONE',  ( 93.43270425363547815, 22.93046121381055968, -73.33260761053102783 ) ) ;
#61292=ORIENTED_EDGE ( 'NONE', *, *, #66988, .F. ) ;
#61293=CARTESIAN_POINT ( 'NONE',  ( 8.683531412707429453, 6.377173148747127485, -40.60382404160758796 ) ) ;
#61294=CARTESIAN_POINT ( 'NONE',  ( -105.7402726937670678, 35.71226297334109034, -89.54607016031067701 ) ) ;
#61295=CARTESIAN_POINT ( 'NONE',  ( 19.10216788411014122, 6.629360741291161041, 3.937534161706087943 ) ) ;
#61297=B_SPLINE_CURVE_WITH_KNOTS ( 'NONE', 3,
 ( #58812, #422, #5008, #20491, #26473, #10623, #11312, #41959, #31409, #52838, #4662, #7095, #6744, #48935, #28555, #49289, #39805, #27496, #23632, #17655, #39454, #50362, #28193, #16939, #49642, #50000, #45070, #43665, #65856, #34193, #12028, #6036, #1470, #60207, #2177, #32784, #1833, #6400, #66555, #44018, #18342, #22930, #23291, #54573, #44736, #12725 ),
 .UNSPECIFIED., .F., .F.,
 ( 4, 2, 2, 2, 2, 2, 2, 2, 2, 2, 2, 2, 2, 2, 2, 2, 2, 2, 2, 2, 2, 2, 4 ),
 ( 1.398578778534940505E-17, 0.003635178948345853429, 0.005452768422518746751, 0.007270357896691640072, 0.008179152633778073722, 0.009087947370864508240, 0.01090553684503742064, 0.01181433158212388812, 0.01272312631921035907, 0.01363192105629682828, 0.01454071579338329749, 0.01544951053046976670, 0.01635830526755623418, 0.01726710000464270686, 0.01817589474172917607, 0.01908468947881564529, 0.01999348421590211450, 0.02090227895298858718, 0.02181107369007505639, 0.02362866316424793930, 0.02544625263842082916, 0.02726384211259371554, 0.02908143158676660192 ),
 .UNSPECIFIED. ) ;
#61300=DIRECTION ( 'NONE',  ( 0.000000000000000000, 0.000000000000000000, 1.000000000000000000 ) ) ;
#61301=CARTESIAN_POINT ( 'NONE',  ( -132.9126122820979390, 52.52752252041129566, -18.22572883211020311 ) ) ;
#61302=CARTESIAN_POINT ( 'NONE',  ( 110.2429982417149290, 28.88204397445231209, -24.07788697519002596 ) ) ;
#61303=CARTESIAN_POINT ( 'NONE',  ( 86.01819737891891293, 19.21322810362191902, 83.41904106266301255 ) ) ;
#61305=ORIENTED_EDGE ( 'NONE', *, *, #64499, .F. ) ;
#61306=ORIENTED_EDGE ( 'NONE', *, *, #63510, .T. ) ;
#61309=CARTESIAN_POINT ( 'NONE',  ( 45.02738683369921802, 9.207938468499234475, 5.602862553026719539 ) ) ;
#61310=CARTESIAN_POINT ( 'NONE',  ( -180.3444197309645176, 97.13822914721130530, 89.96127970653128614 ) ) ;
#61312=CARTESIAN_POINT ( 'NONE',  ( 104.7034219878851928, 26.40210929103715642, -21.65807146565094143 ) ) ;
#61313=CARTESIAN_POINT ( 'NONE',  ( 203.9181091394787870, 105.2759068139671257, 17.36317014830576611 ) ) ;
#61314=CARTESIAN_POINT ( 'NONE',  ( 198.5841913839438746, 99.94205862921178607, 86.03763448066921171 ) ) ;
#61315=CYLINDRICAL_SURFACE ( 'NONE', #13044, 7.500000000000020428 ) ;
#61316=CARTESIAN_POINT ( 'NONE',  ( -71.59086462055189770, 19.75139532313339430, -71.95998834529184762 ) ) ;
#61319=AXIS2_PLACEMENT_3D ( 'NONE', #835, #33195, #125 ) ;
#61320=CARTESIAN_POINT ( 'NONE',  ( 10.31616749326173554, 7.393414706728908214, -21.30915619223937085 ) ) ;
#61322=ORIENTED_EDGE ( 'NONE', *, *, #67591, .F. ) ;
#61325=CARTESIAN_POINT ( 'NONE',  ( 188.5842358232185916, 88.03712271786932320, -70.86903138220263543 ) ) ;
#61326=CARTESIAN_POINT ( 'NONE',  ( -37.51960690572916235, 11.69306339258380056, 87.00308991710100770 ) ) ;
#61327=CARTESIAN_POINT ( 'NONE',  ( 207.8484262634767390, 110.7633525054913974, -77.48949184225725162 ) ) ;
#61333=CARTESIAN_POINT ( 'NONE',  ( 128.4224537826254107, 38.23837035195744960, -38.33144164633024076 ) ) ;
#61334=VERTEX_POINT ( 'NONE', #66319 ) ;
#61335=ORIENTED_EDGE ( 'NONE', *, *, #50020, .F. ) ;
#61336=VECTOR ( 'NONE', #21834, 1000.000000000000114 ) ;
#61338=VECTOR ( 'NONE', #51462, 1000.000000000000000 ) ;
#61341=CARTESIAN_POINT ( 'NONE',  ( 58.48209831743720599, 11.66636741727081628, -10.38159958421693574 ) ) ;
#61343=CARTESIAN_POINT ( 'NONE',  ( -50.14771795543006050, 13.42081263859820872, 32.12267660860144503 ) ) ;
#61346=CYLINDRICAL_SURFACE ( 'NONE', #44652, 7.500000000000020428 ) ;
#61348=CARTESIAN_POINT ( 'NONE',  ( 198.4059165548112560, 99.71594270191990006, -66.57968520498842224 ) ) ;
#61350=CARTESIAN_POINT ( 'NONE',  ( 107.9301116202192077, 27.82606182274595596, 3.116396251667963746 ) ) ;
#61351=CARTESIAN_POINT ( 'NONE',  ( -169.8842709557924593, 83.59602878049473418, 4.696942425479066152 ) ) ;
#61353=FACE_BOUND ( 'NONE', #40396, .T. ) ;
#61355=CARTESIAN_POINT ( 'NONE',  ( -101.2355754230665781, 32.25344808697845167, -88.77378729876801344 ) ) ;
#61356=ORIENTED_EDGE ( 'NONE', *, *, #9778, .F. ) ;
#61358=CARTESIAN_POINT ( 'NONE',  ( 153.2523375521184050, 55.69936538551846894, 57.54797417081107369 ) ) ;
#61362=EDGE_CURVE ( 'NONE', #32365, #29569, #18106, .T. ) ;
#61368=CARTESIAN_POINT ( 'NONE',  ( -177.5271152834791337, 92.16916858125017598, -62.96948660494962269 ) ) ;
#61373=CARTESIAN_POINT ( 'NONE',  ( -180.0175713311536754, 95.14770835574076102, 8.515290778967939289 ) ) ;
#61374=CARTESIAN_POINT ( 'NONE',  ( -0.5751131641471384226, 6.527254166626918597, 12.70591576700029890 ) ) ;
#61375=LINE ( 'NONE', #18127, #34871 ) ;
#61378=CARTESIAN_POINT ( 'NONE',  ( 139.7928618793172859, 45.12615179300589574, 14.75651092525571784 ) ) ;
#61379=CARTESIAN_POINT ( 'NONE',  ( -180.6209440844957896, 95.88392769199009535, 38.64167446930188987 ) ) ;
#61385=CARTESIAN_POINT ( 'NONE',  ( -74.20136529587826146, 21.74007521413449950, 17.10464239477820669 ) ) ;
#61386=CARTESIAN_POINT ( 'NONE',  ( 46.90222083990963853, 9.503928413859233260, -42.87962864881881586 ) ) ;
#61387=CARTESIAN_POINT ( 'NONE',  ( -172.3127615181935539, 87.73358064377643473, -76.52411096701514737 ) ) ;
#61388=CARTESIAN_POINT ( 'NONE',  ( -120.0202139357153186, 42.74628011209018297, 87.13439761332067235 ) ) ;
#61389=ORIENTED_EDGE ( 'NONE', *, *, #38208, .F. ) ;
#61390=CARTESIAN_POINT ( 'NONE',  ( 79.93126905972556528, 17.24332478304277316, -46.70519100763757336 ) ) ;
#61394=CARTESIAN_POINT ( 'NONE',  ( 79.12879321038292346, 18.04902206524926811, 37.44799338594253868 ) ) ;
#61396=CARTESIAN_POINT ( 'NONE',  ( 39.40195752203892710, -170.0000000000000000, -50.61981746542779348 ) ) ;
#61397=CARTESIAN_POINT ( 'NONE',  ( 139.3067271572849677, 44.81402783181197691, -11.52040805170238791 ) ) ;
#61399=CARTESIAN_POINT ( 'NONE',  ( -180.4614954900547161, 97.28277348252829881, -16.93614783883196750 ) ) ;
#61400=CARTESIAN_POINT ( 'NONE',  ( -153.7005182577090068, 67.81869626254727734, -36.07780814487768595 ) ) ;
#61401=VERTEX_POINT ( 'NONE', #25813 ) ;
#61404=CARTESIAN_POINT ( 'NONE',  ( 105.2506154496929582, 26.63995206619729927, 69.55816789470473793 ) ) ;
#61405=CARTESIAN_POINT ( 'NONE',  ( 164.7167608259061637, 63.51199216609071385, 61.80061252660392057 ) ) ;
#61407=ADVANCED_FACE ( 'NONE', ( #40943 ), #62753, .T. ) ;
#61408=ADVANCED_FACE ( 'NONE', ( #51511 ), #8245, .F. ) ;
#61411=CARTESIAN_POINT ( 'NONE',  ( 186.2651679807462415, 84.00458780104320056, -49.16829926748396673 ) ) ;
#61412=CARTESIAN_POINT ( 'NONE',  ( -105.4589068214114178, 34.42476264325677704, 58.05430461866929903 ) ) ;
#61413=CARTESIAN_POINT ( 'NONE',  ( -31.43908319763709258, 9.591432048623767415, -35.31719736520183517 ) ) ;
#61426=CARTESIAN_POINT ( 'NONE',  ( -62.06231780744545290, 17.72446026058426938, 40.49660573368029048 ) ) ;
#61427=CARTESIAN_POINT ( 'NONE',  ( -96.77705718164442317, 31.18700926299570853, -10.55039380601694710 ) ) ;
#61428=AXIS2_PLACEMENT_3D ( 'NONE', #35818, #15047, #57616 ) ;
#61429=CARTESIAN_POINT ( 'NONE',  ( 57.07246224906425880, 12.39953617563783084, 41.91415364038640945 ) ) ;
#61430=CARTESIAN_POINT ( 'NONE',  ( 31.90811916295598039, 7.552800146120133284, 91.55187592262117846 ) ) ;
#61434=CARTESIAN_POINT ( 'NONE',  ( -7.825402957745083654, 6.891034867348166060, -50.41807073194384259 ) ) ;
#61436=CARTESIAN_POINT ( 'NONE',  ( -14.84903512415885274, 8.461292896365064209, 13.41286030492582348 ) ) ;
#61437=CARTESIAN_POINT ( 'NONE',  ( -142.4991775570125583, 58.45550857435405590, 14.10091869410458010 ) ) ;
#61439=CARTESIAN_POINT ( 'NONE',  ( 197.3054165770396366, 96.72615186924561215, 62.24439187461354095 ) ) ;
#61440=CARTESIAN_POINT ( 'NONE',  ( 128.0882145863933772, 39.20607399008168414, -21.49800594817171273 ) ) ;
#61441=AXIS2_PLACEMENT_3D ( 'NONE', #37232, #58342, #9831 ) ;
#61445=CARTESIAN_POINT ( 'NONE',  ( -35.17296606710973350, 11.25626711331309515, -49.34029585684413632 ) ) ;
#61448=CARTESIAN_POINT ( 'NONE',  ( 39.40195752203892710, -170.0000000000000000, -77.46436805589148378 ) ) ;
#61450=CARTESIAN_POINT ( 'NONE',  ( -122.7930600691578036, 44.48546375740917114, -35.56903786926160649 ) ) ;
#61454=CARTESIAN_POINT ( 'NONE',  ( 150.3392635816054508, 53.55403001380570771, 88.24482449747890200 ) ) ;
#61458=CARTESIAN_POINT ( 'NONE',  ( -154.7826623253029936, 70.14150242829515491, 32.88389497768243075 ) ) ;
#61460=CARTESIAN_POINT ( 'NONE',  ( 79.82127737190243977, 17.20935440217364487, 7.211099181453766604 ) ) ;
#61463=AXIS2_PLACEMENT_3D ( 'NONE', #87, #32454, #21887 ) ;
#61465=CARTESIAN_POINT ( 'NONE',  ( -1.928775478690862188, 7.585606196872214824, -91.95340218108046315 ) ) ;
#61471=CARTESIAN_POINT ( 'NONE',  ( 173.5836858989432301, 72.71885240881778145, 37.09537031985573208 ) ) ;
#61472=CARTESIAN_POINT ( 'NONE',  ( -31.65307660562752901, 10.64641742089424703, -89.00629854612921577 ) ) ;
#61475=CARTESIAN_POINT ( 'NONE',  ( -10.69547592951790804, 8.103864096836391084, -76.70459122694524012 ) ) ;
#61477=CYLINDRICAL_SURFACE ( 'NONE', #63376, 7.500000000000013323 ) ;
#61478=CARTESIAN_POINT ( 'NONE',  ( -25.07735481787161902, 9.648965052008779963, 33.73669382820916951 ) ) ;
#61479=CARTESIAN_POINT ( 'NONE',  ( -72.35078170365747496, 21.08176362823951777, -46.66809070389184200 ) ) ;
#61482=CARTESIAN_POINT ( 'NONE',  ( 175.1380114663270149, 74.18445479419006006, -92.83823291830314872 ) ) ;
#61484=CARTESIAN_POINT ( 'NONE',  ( 141.0792860804899647, 47.16255757051796138, 34.91922768290986312 ) ) ;
#61486=CARTESIAN_POINT ( 'NONE',  ( -130.1938957973835613, 50.61368074696266461, 5.112861415500842277 ) ) ;
#61487=LINE ( 'NONE', #23858, #55356 ) ;
#61488=EDGE_LOOP ( 'NONE', ( #9283, #38846 ) ) ;
#61500=CARTESIAN_POINT ( 'NONE',  ( -74.39861643904067989, 21.81123504700006777, -9.598885444783787690 ) ) ;
#61501=ORIENTED_EDGE ( 'NONE', *, *, #23437, .F. ) ;
#61502=CARTESIAN_POINT ( 'NONE',  ( -105.4642082819536029, 35.56541171990216554, 44.82579570833843974 ) ) ;
#61507=CARTESIAN_POINT ( 'NONE',  ( 110.2429982417149574, -170.0000000000000000, 37.11121420573731911 ) ) ;
#61510=CARTESIAN_POINT ( 'NONE',  ( -54.56693200831794144, 14.55131601960339083, 18.47277718246750666 ) ) ;
#61515=CARTESIAN_POINT ( 'NONE',  ( -155.5978531700836527, 69.52241200678679434, -11.08417929211540276 ) ) ;
#61516=ORIENTED_EDGE ( 'NONE', *, *, #63282, .T. ) ;
#61517=CARTESIAN_POINT ( 'NONE',  ( -55.53469534616547776, 14.81076603075804066, 30.31732777293112946 ) ) ;
#61518=CARTESIAN_POINT ( 'NONE',  ( -56.72676045871357786, 16.18052435693488533, 57.34706834696837774 ) ) ;
#61522=CARTESIAN_POINT ( 'NONE',  ( 154.0281735872262061, 56.28213428456459155, -63.80132600415307564 ) ) ;
#61523=CARTESIAN_POINT ( 'NONE',  ( -35.38560449531986052, 10.27249159032102277, 31.33411146270130487 ) ) ;
#61524=AXIS2_PLACEMENT_3D ( 'NONE', #45937, #19548, #41010 ) ;
#61525=CARTESIAN_POINT ( 'NONE',  ( 140.2332932573541484, 45.41010019581506185, -39.54326788570185869 ) ) ;
#61528=DIRECTION ( 'NONE',  ( -0.000000000000000000, 1.000000000000000000, -0.000000000000000000 ) ) ;
#61531=ORIENTED_EDGE ( 'NONE', *, *, #6542, .F. ) ;
#61532=CARTESIAN_POINT ( 'NONE',  ( 31.95163392065795804, 8.568192436298479819, -17.26688347263179679 ) ) ;
#61534=CARTESIAN_POINT ( 'NONE',  ( 91.11342358617750392, 21.00000175105271083, 58.03984230042496506 ) ) ;
#61536=( NAMED_UNIT ( * ) SI_UNIT ( $, .STERADIAN. ) SOLID_ANGLE_UNIT ( ) );
#61538=EDGE_CURVE ( 'NONE', #51139, #41326, #56655, .T. ) ;
#61541=CARTESIAN_POINT ( 'NONE',  ( 158.3604774538084712, 58.34594647925810307, -9.319281447646249106 ) ) ;
#61542=DIRECTION ( 'NONE',  ( 0.000000000000000000, -1.000000000000000000, 0.000000000000000000 ) ) ;
#61543=CARTESIAN_POINT ( 'NONE',  ( 63.98971758354224448, 12.90030016320051232, 71.61000590023084555 ) ) ;
#61544=CARTESIAN_POINT ( 'NONE',  ( 140.5958192060901695, 46.84598876498518649, 6.864059862099193055 ) ) ;
#61548=CARTESIAN_POINT ( 'NONE',  ( 158.3516718297676107, 59.61984652322050948, -24.24089676901845536 ) ) ;
#61554=ADVANCED_FACE ( 'NONE', ( #52857 ), #53892, .F. ) ;
#61556=CARTESIAN_POINT ( 'NONE',  ( -149.2910611247327779, 63.99625741915658494, -61.65738112195566600 ) ) ;
#61563=CARTESIAN_POINT ( 'NONE',  ( -100.4347360276018861, 32.97716872911836816, 3.890190775139684476 ) ) ;
#61564=B_SPLINE_CURVE_WITH_KNOTS ( 'NONE', 3,
 ( #9213, #67966, #24013, #19767, #24713, #3937, #61641, #61295, #30326, #29625, #25058, #51779, #2905, #34586, #46147, #2557, #19074, #3585, #46488, #56023, #66939, #50733, #45456, #18730, #24365, #45810, #67289, #13457, #34917, #56356, #20796, #20115, #53482, #68637, #63019, #64050, #15530, #4618, #31362, #58419, #42923, #16206, #58089, #69330, #23 ),
 .UNSPECIFIED., .F., .F.,
 ( 4, 2, 2, 1, 2, 2, 2, 2, 2, 2, 2, 2, 2, 2, 2, 2, 2, 2, 2, 2, 2, 2, 4 ),
 ( 0.02345095402629350512, 0.02491692321306682861, 0.02564990780645348689, 0.02638289239984014517, 0.02711587699322680345, 0.02784886158661346173, 0.02931483077338677828, 0.03004781536677343309, 0.03078079996016008790, 0.03224676914693340446, 0.03297975374032005580, 0.03371273833370671408, 0.03517870752048002370, 0.03664467670725333331, 0.03737766130063998465, 0.03811064589402663599, 0.03957661508079993173, 0.04104258426757322747, 0.04250855345434652321, 0.04324153804773317455, 0.04397452264111981202, 0.04544049182789309388, 0.04690646101466637574 ),
 .UNSPECIFIED. ) ;
#61565=CARTESIAN_POINT ( 'NONE',  ( 61.73284572609541954, 13.41039274811037352, 83.60527669376516258 ) ) ;
#61568=CARTESIAN_POINT ( 'NONE',  ( 81.57915404881515542, 18.81499384983930767, -22.02727323828690231 ) ) ;
#61569=CARTESIAN_POINT ( 'NONE',  ( -170.2801941679960009, 84.02053682015869640, 31.36767604865260850 ) ) ;
#61570=CARTESIAN_POINT ( 'NONE',  ( 32.32614265053613423, 8.605592782137726715, -94.18410555706600462 ) ) ;
#61575=CARTESIAN_POINT ( 'NONE',  ( -12.78319349481552081, 8.274445259016799170, 70.10900556253349691 ) ) ;
#61577=CARTESIAN_POINT ( 'NONE',  ( 39.40195752203892710, -170.0000000000000000, 37.41383430596326320 ) ) ;
#61579=CARTESIAN_POINT ( 'NONE',  ( 211.1046732743772907, 117.3965485104337461, -13.07269876749372628 ) ) ;
#61581=CARTESIAN_POINT ( 'NONE',  ( -0.3732240621745024356, 7.527003275829099671, 38.59489257713590149 ) ) ;
#61582=CARTESIAN_POINT ( 'NONE',  ( -12.19213298737871298, 7.214665545688172976, -90.49457743040542823 ) ) ;
#61584=CARTESIAN_POINT ( 'NONE',  ( -53.13004807512038496, 14.17398740785106526, -62.29520437222935669 ) ) ;
#61585=CARTESIAN_POINT ( 'NONE',  ( -5.879983509979051171, 7.779504553499513975, -23.33333956214708493 ) ) ;
#61587=CARTESIAN_POINT ( 'NONE',  ( -60.97011009284709360, 16.34812508431679490, 15.60724065707690755 ) ) ;
#61589=VECTOR ( 'NONE', #11650, 1000.000000000000000 ) ;
#61594=CARTESIAN_POINT ( 'NONE',  ( 39.40195752203892710, 8.409560354027384221, 71.75838489642698903 ) ) ;
#61599=CARTESIAN_POINT ( 'NONE',  ( -165.7689197919845014, 79.30072199592275695, 66.67702330705374436 ) ) ;
#61600=VERTEX_POINT ( 'NONE', #23995 ) ;
#61601=ORIENTED_EDGE ( 'NONE', *, *, #51085, .T. ) ;
#61605=CARTESIAN_POINT ( 'NONE',  ( -171.0950923142953854, 86.38958441093224394, 57.93243116198902243 ) ) ;
#61607=CARTESIAN_POINT ( 'NONE',  ( 61.08522853873726177, 13.26388801693370922, -9.112382269691240211 ) ) ;
#61610=DIRECTION ( 'NONE',  ( 1.000000000000000000, 0.000000000000000000, -0.000000000000000000 ) ) ;
#61613=CARTESIAN_POINT ( 'NONE',  ( 8.485361335568063268, 6.376707943524878353, -95.00000000000133582 ) ) ;
#61617=ADVANCED_FACE ( 'NONE', ( #60926 ), #60579, .F. ) ;
#61621=CARTESIAN_POINT ( 'NONE',  ( 110.2429982417149574, -170.0000000000000000, 63.95576479620102361 ) ) ;
#61623=CARTESIAN_POINT ( 'NONE',  ( -180.5954680880247167, 97.44843622358463620, 10.83696913367529646 ) ) ;
#61624=CARTESIAN_POINT ( 'NONE',  ( 212.1734186221016216, 119.0499290057855575, 64.24444335267637030 ) ) ;
#61625=CARTESIAN_POINT ( 'NONE',  ( 80.17205177205137545, 17.31791394718354837, -73.98926831092168754 ) ) ;
#61627=DIRECTION ( 'NONE',  ( 0.000000000000000000, 0.000000000000000000, 1.000000000000000000 ) ) ;
#61632=CARTESIAN_POINT ( 'NONE',  ( -85.34215807311491631, 24.97769003780924280, -66.03245772043236173 ) ) ;
#61634=CARTESIAN_POINT ( 'NONE',  ( 15.78827728214693416, 6.500811158483284835, -77.36349468914950478 ) ) ;
#61635=EDGE_CURVE ( 'NONE', #31528, #66072, #49314, .T. ) ;
#61638=ORIENTED_EDGE ( 'NONE', *, *, #24858, .T. ) ;
#61640=CARTESIAN_POINT ( 'NONE',  ( -108.2447486367085929, 37.06113128159649506, -91.63506942693179269 ) ) ;
#61641=CARTESIAN_POINT ( 'NONE',  ( 18.66025561752211104, 6.609375019058820300, 3.728956910112429579 ) ) ;
#61644=CARTESIAN_POINT ( 'NONE',  ( 59.94652978725885362, 13.01168383647462434, -36.37311755078323472 ) ) ;
#61646=CARTESIAN_POINT ( 'NONE',  ( 112.5721302457195350, 29.97407549554797868, -9.433108360236460044 ) ) ;
#61647=CARTESIAN_POINT ( 'NONE',  ( 81.57915404881515542, 18.81499384983930412, -48.87182382875059261 ) ) ;
#61648=CARTESIAN_POINT ( 'NONE',  ( -170.4689427914638031, 85.70641121003137641, -88.87457044037061848 ) ) ;
#61652=CARTESIAN_POINT ( 'NONE',  ( 46.13320811200731697, 9.380653113584052960, 7.225283526527610967 ) ) ;
#61654=CARTESIAN_POINT ( 'NONE',  ( -47.80193682758674356, 12.85650137125657544, -17.85234014397047275 ) ) ;
#61655=CARTESIAN_POINT ( 'NONE',  ( 110.2429982417149290, 28.88204397445231209, -24.07788697519002596 ) ) ;
#61657=CARTESIAN_POINT ( 'NONE',  ( -24.30174763577181096, 8.528231305356500869, -94.16290959115248427 ) ) ;
#61658=CARTESIAN_POINT ( 'NONE',  ( 212.2010424008437894, 119.0930793856250887, 90.34093224311959602 ) ) ;
#61660=CARTESIAN_POINT ( 'NONE',  ( -85.73740570227381852, 26.23277384689413694, 62.24966593035414064 ) ) ;
#61661=CARTESIAN_POINT ( 'NONE',  ( -13.47230132170245653, 7.324574289401433624, 42.57560624842334107 ) ) ;
#61663=CARTESIAN_POINT ( 'NONE',  ( 8.763528846667103522, 7.383598436776580343, -13.53555138396326996 ) ) ;
#61667=CARTESIAN_POINT ( 'NONE',  ( -143.8634661037141029, 60.82480701605699380, 6.410842245792165883 ) ) ;
#61668=CARTESIAN_POINT ( 'NONE',  ( 181.0840389613909736, 80.03940679743418229, -63.06960825634327961 ) ) ;
#61669=CARTESIAN_POINT ( 'NONE',  ( -32.09642077712169339, 10.71953907670691919, 83.90686141431137912 ) ) ;
#61670=CARTESIAN_POINT ( 'NONE',  ( 208.9507214515059843, 112.3605999017434698, -76.86410794482465292 ) ) ;
#61674=CARTESIAN_POINT ( 'NONE',  ( 8.480977594057451441, 7.382886909400596664, -44.72572676602403874 ) ) ;
#61675=CARTESIAN_POINT ( 'NONE',  ( 126.4083787442699673, 37.10531539900949127, -44.54862598322278444 ) ) ;
#61679=FACE_OUTER_BOUND ( 'NONE', #55537, .T. ) ;
#61681=CARTESIAN_POINT ( 'NONE',  ( -26.87327614295026024, 8.886070347947315540, -63.69140009212348730 ) ) ;
#61682=CARTESIAN_POINT ( 'NONE',  ( 11.82322073186613132, 6.406156243758798219, 4.299284300909138601 ) ) ;
#61687=CARTESIAN_POINT ( 'NONE',  ( 197.4121679705847896, 98.46451029407251099, -72.45810111998113712 ) ) ;
#61690=CARTESIAN_POINT ( 'NONE',  ( -166.1495968531527581, 79.68938347407072342, -93.12242192314892009 ) ) ;
#61695=CARTESIAN_POINT ( 'NONE',  ( -2.174378755909786687, 6.588636630831476104, 69.41550620898735247 ) ) ;
#61699=CARTESIAN_POINT ( 'NONE',  ( 154.0515132159917471, 56.29926936869307497, 57.06238980954113771 ) ) ;
#61700=LINE ( 'NONE', #13525, #14129 ) ;
#61708=CARTESIAN_POINT ( 'NONE',  ( 179.0096185093688064, 76.53352131383245194, -50.94553233058115893 ) ) ;
#61709=CARTESIAN_POINT ( 'NONE',  ( 156.5890478960376413, 58.24007662587946044, 44.37067197906655736 ) ) ;
#61714=AXIS2_PLACEMENT_3D ( 'NONE', #42673, #9287, #68712 ) ;
#61715=CARTESIAN_POINT ( 'NONE',  ( -177.5271152834791621, 92.16916858125016176, 17.56416516644142334 ) ) ;
#61716=CARTESIAN_POINT ( 'NONE',  ( -2.866724795119729219, 6.618578306599218308, 16.41915603436029514 ) ) ;
#61718=CARTESIAN_POINT ( 'NONE',  ( -86.16504208171677703, 26.41251233979373936, 37.38851751404891388 ) ) ;
#61719=CARTESIAN_POINT ( 'NONE',  ( -23.99957301099517437, 9.503061049698496632, -16.95513486474544251 ) ) ;
#61720=CARTESIAN_POINT ( 'NONE',  ( 139.6203063421347679, 45.01495791936839908, 5.340914006301072270 ) ) ;
#61728=CARTESIAN_POINT ( 'NONE',  ( 82.74007713545066167, 18.13042311233564163, -49.73892840124477743 ) ) ;
#61731=CARTESIAN_POINT ( 'NONE',  ( -148.6409722988649662, 63.44808865916662199, 72.51830521237032201 ) ) ;
#61734=CARTESIAN_POINT ( 'NONE',  ( 185.5572090022886016, 83.24697331286184010, -10.84236386202956304 ) ) ;
#61736=CARTESIAN_POINT ( 'NONE',  ( -79.62207341875655686, 23.76621716825509978, -8.316621442820189003 ) ) ;
#61738=CARTESIAN_POINT ( 'NONE',  ( -48.58011387679029269, 14.07568064779664674, 34.02037858821316973 ) ) ;
#61745=EDGE_CURVE ( 'NONE', #49052, #33190, #59871, .T. ) ;
#61746=CARTESIAN_POINT ( 'NONE',  ( 181.0840389613909736, 78.60582251573005408, -51.22505766587963905 ) ) ;
#61749=CARTESIAN_POINT ( 'NONE',  ( 164.9559213734325169, 63.71338633026441300, -69.92522862138935125 ) ) ;
#61754=CARTESIAN_POINT ( 'NONE',  ( -71.97767679134960872, 19.88555875055813971, 94.99999999999866418 ) ) ;
#61755=CARTESIAN_POINT ( 'NONE',  ( 37.70910994512001224, 9.209110272746713122, -50.43038720028041411 ) ) ;
#61756=CARTESIAN_POINT ( 'NONE',  ( 63.01563776193091826, 12.67277567978498531, -50.72069083216976537 ) ) ;
#61761=CARTESIAN_POINT ( 'NONE',  ( 60.63380853769238854, 13.16344960520421736, 30.19706154477051285 ) ) ;
#61763=ORIENTED_EDGE ( 'NONE', *, *, #6819, .F. ) ;
#61764=FACE_OUTER_BOUND ( 'NONE', #44517, .T. ) ;
#61766=CARTESIAN_POINT ( 'NONE',  ( -189.9638655956219964, 108.0957249433520673, -45.34231387932501178 ) ) ;
#61767=CARTESIAN_POINT ( 'NONE',  ( -144.2029146819478740, 59.80706661873671948, 16.70020471700040332 ) ) ;
#61768=CARTESIAN_POINT ( 'NONE',  ( 19.54452863209719382, 7.657034792877148277, -9.664348475683180340 ) ) ;
#61769=CARTESIAN_POINT ( 'NONE',  ( -109.7816385129979153, 36.75776661907243437, -69.85981554950058126 ) ) ;
#61770=EDGE_CURVE ( 'NONE', #52584, #63745, #32363, .T. ) ;
#61771=CARTESIAN_POINT ( 'NONE',  ( 126.6464677212869816, 38.39096133771045061, -18.81003903715838987 ) ) ;
#61777=CARTESIAN_POINT ( 'NONE',  ( -34.06637338149495520, 11.05895377318623574, -49.84616098674828777 ) ) ;
#61780=CARTESIAN_POINT ( 'NONE',  ( -169.7991992212453738, 83.50566726453351407, 85.28103951956639150 ) ) ;
#61782=CARTESIAN_POINT ( 'NONE',  ( 126.4757069339777473, 38.29528077539267628, 8.808907411169407453 ) ) ;
#61785=CARTESIAN_POINT ( 'NONE',  ( -143.2464978228199186, 59.04559547356112148, -11.33080930835344624 ) ) ;
#61787=ORIENTED_EDGE ( 'NONE', *, *, #6348, .F. ) ;
#61788=CARTESIAN_POINT ( 'NONE',  ( 152.1975304496806700, 54.91466247927352384, 85.25451727479598674 ) ) ;
#61791=CARTESIAN_POINT ( 'NONE',  ( -59.96408504033279740, 17.10126854471816316, 16.66205370559185539 ) ) ;
#61792=CARTESIAN_POINT ( 'NONE',  ( 127.2202105166096402, 37.55913282978156786, 33.50704232745487587 ) ) ;
#61793=CARTESIAN_POINT ( 'NONE',  ( -156.7435307435794130, 71.93726016406968427, 36.22848380757431386 ) ) ;
#61796=EDGE_CURVE ( 'NONE', #27866, #18637, #68293, .T. ) ;
#61801=CARTESIAN_POINT ( 'NONE',  ( -3.791772492091277424, 7.668372357990064891, -90.22677180356119209 ) ) ;
#61802=ORIENTED_EDGE ( 'NONE', *, *, #7656, .F. ) ;
#61804=CARTESIAN_POINT ( 'NONE',  ( 173.6737675136087660, 72.80308721038095143, 35.61421337580090807 ) ) ;
#61805=CARTESIAN_POINT ( 'NONE',  ( 15.78827728214693416, 6.500811158483329244, -62.36349468914946925 ) ) ;
#61806=CARTESIAN_POINT ( 'NONE',  ( -132.6092625803567273, 52.31125232006263559, 68.31422680659306934 ) ) ;
#61808=CARTESIAN_POINT ( 'NONE',  ( -96.26864862082260288, 30.94441745358434304, 87.21210164009336552 ) ) ;
#61810=CARTESIAN_POINT ( 'NONE',  ( -71.42007367207959589, 20.75704712149296682, -44.61501727073203938 ) ) ;
#61811=ORIENTED_EDGE ( 'NONE', *, *, #40051, .T. ) ;
#61813=DIRECTION ( 'NONE',  ( 0.000000000000000000, 0.000000000000000000, 1.000000000000000000 ) ) ;
#61815=CARTESIAN_POINT ( 'NONE',  ( -133.3944793432480367, 52.87251459353622352, 11.53032100427611795 ) ) ;
#61816=CARTESIAN_POINT ( 'NONE',  ( 70.51583798635766698, 15.57951509147423330, -70.30715017899500197 ) ) ;
#61817=VERTEX_POINT ( 'NONE', #52106 ) ;
#61819=CARTESIAN_POINT ( 'NONE',  ( -142.5042386072304055, 59.74110826975218203, -18.20533799458240409 ) ) ;
#61826=CARTESIAN_POINT ( 'NONE',  ( -167.1540252468942356, 80.72321878831101571, -73.60722793262152663 ) ) ;
#61830=EDGE_CURVE ( 'NONE', #62112, #27226, #19776, .T. ) ;
#61831=CARTESIAN_POINT ( 'NONE',  ( 33.03722315490661998, 7.666819786578626506, 41.38888860195424968 ) ) ;
#61835=CYLINDRICAL_SURFACE ( 'NONE', #47846, 7.500000000000013323 ) ;
#61837=CARTESIAN_POINT ( 'NONE',  ( 32.14349651933086705, 7.576119504381665593, 8.618131405027169123 ) ) ;
#61840=CARTESIAN_POINT ( 'NONE',  ( 150.4544126017350720, 52.39556706174411005, -46.28865209072233000 ) ) ;
#61841=B_SPLINE_CURVE_WITH_KNOTS ( 'NONE', 3,
 ( #39257, #50843, #2661, #35016, #24121, #45216, #56461, #55417, #8288, #28702, #51198, #24474, #38909, #12173, #50150, #1975, #62083, #51877, #68076, #25853, #14931, #63474, #4046, #51546, #41335, #14257, #9671, #52565, #30779, #46246, #3689, #35715, #19878, #67383, #41671, #46594, #40980, #13900, #25165, #67725, #58190, #68413, #3351, #62788, #36746, #36398 ),
 .UNSPECIFIED., .F., .F.,
 ( 4, 2, 2, 2, 2, 2, 2, 2, 2, 2, 2, 2, 2, 2, 2, 2, 2, 2, 2, 2, 2, 2, 4 ),
 ( 0.02584318557310391617, 0.02743529570732761852, 0.02823135077443945928, 0.02902740584155130005, 0.03061951597577497464, 0.03221162610999864923, 0.03380373624422232381, 0.03459979131133418540, 0.03539584637844603310, 0.03619190144555788774, 0.03698795651266974238, 0.03858006664689345167, 0.03937612171400529937, 0.04017217678111716095, 0.04096823184822900865, 0.04176428691534087023, 0.04335639704956461421, 0.04494850718378835819, 0.04654061731801210910, 0.04813272745223585308, 0.04892878251934774936, 0.04972483758645964563, 0.05131694772068339655 ),
 .UNSPECIFIED. ) ;
#61842=EDGE_LOOP ( 'NONE', ( #64061, #8437, #59786, #41739 ) ) ;
#61843=CARTESIAN_POINT ( 'NONE',  ( -103.1191803759318191, 33.20880928687111577, -88.73880487180355203 ) ) ;
#61846=CARTESIAN_POINT ( 'NONE',  ( -58.76099769480629931, 16.75353773354893860, 71.18551801496039388 ) ) ;
#61849=EDGE_CURVE ( 'NONE', #36237, #1174, #33983, .T. ) ;
#61851=CARTESIAN_POINT ( 'NONE',  ( -9.763294602873862971, 7.024900256480052896, -62.51313501726206567 ) ) ;
#61853=ADVANCED_FACE ( 'NONE', ( #63235 ), #35465, .T. ) ;
#61854=CARTESIAN_POINT ( 'NONE',  ( 134.7770330630253284, 41.98246829846537054, -36.06570861580060949 ) ) ;
#61858=CARTESIAN_POINT ( 'NONE',  ( -156.4966862384869160, 71.70877417666515896, 67.83814759271207606 ) ) ;
#61859=CARTESIAN_POINT ( 'NONE',  ( -118.6288898061518893, 41.89286798341292695, 36.23774008308858186 ) ) ;
#61860=CARTESIAN_POINT ( 'NONE',  ( -57.42615654242919732, 15.33060010148603780, -35.59764363562960199 ) ) ;
#61863=CARTESIAN_POINT ( 'NONE',  ( 126.4143409752912817, 38.26092613416376764, 91.69694997615445686 ) ) ;
#61864=CARTESIAN_POINT ( 'NONE',  ( 113.8748103246145575, 30.59837980920001854, 43.69098323372512738 ) ) ;
#61865=CARTESIAN_POINT ( 'NONE',  ( 93.27435913120712030, 21.79585130525710568, -93.43499286684529181 ) ) ;
#61866=B_SPLINE_CURVE_WITH_KNOTS ( 'NONE', 3,
 ( #47817, #68591, #69277, #20065, #21104, #64002, #8829, #46438, #67919, #41518, #11215, #11555, #28093, #26720, #48831, #17184, #64695, #58708, #32682, #43217, #54823, #33394, #6295, #54107, #15813, #5933, #53430, #11921, #10525, #22827, #48149, #65396, #16502, #31998, #37256, #59059, #38657, #6644, #27745, #21430, #27393, #29953, #5259, #37960 ),
 .UNSPECIFIED., .F., .F.,
 ( 4, 2, 2, 2, 2, 2, 2, 2, 2, 2, 2, 2, 2, 2, 2, 2, 2, 2, 2, 2, 2, 4 ),
 ( 0.02432640572110344318, 0.02583721026359364972, 0.02659261253483873391, 0.02734801480608381810, 0.02885881934857401770, 0.02961422161981914006, 0.03036962389106425894, 0.03188042843355446548, 0.03339123297604467550, 0.03414663524728978050, 0.03490203751853487857, 0.03641284206102507470, 0.03716824433227017277, 0.03792364660351526390, 0.03943445114600544615, 0.04094525568849563535, 0.04245606023098581067, 0.04396686477347599292, 0.04472226704472108405, 0.04547766931596616824, 0.04698847385845635050, 0.04849927840094651887 ),
 .UNSPECIFIED. ) ;
#61869=CARTESIAN_POINT ( 'NONE',  ( 159.6725804802005939, 59.38339663535512614, -9.596184105213222182 ) ) ;
#61870=CARTESIAN_POINT ( 'NONE',  ( 115.2288739107204947, 31.25773204386717197, -75.87499467958308230 ) ) ;
#61871=CARTESIAN_POINT ( 'NONE',  ( 67.56108154898467433, 13.77276756375644950, 70.14326033379539638 ) ) ;
#61872=CARTESIAN_POINT ( 'NONE',  ( 140.0820590176526252, 46.51134312115247127, 5.975627082199469697 ) ) ;
#61885=CARTESIAN_POINT ( 'NONE',  ( 127.7862882585783808, 37.87790449424836936, 86.28152948240347087 ) ) ;
#61887=CARTESIAN_POINT ( 'NONE',  ( 164.6561571795774626, 64.77723933022092240, -41.40462224256973656 ) ) ;
#61889=AXIS2_PLACEMENT_3D ( 'NONE', #18747, #55683, #34600 ) ;
#61891=CARTESIAN_POINT ( 'NONE',  ( 164.7167608259061353, 63.51199216609071385, -45.57758983525081220 ) ) ;
#61894=CARTESIAN_POINT ( 'NONE',  ( 61.40555507485842668, 13.33627009881806558, 83.66953863785889212 ) ) ;
#61895=CARTESIAN_POINT ( 'NONE',  ( 154.9766071814075588, 57.00087550806519232, -90.23040783010065979 ) ) ;
#61896=CARTESIAN_POINT ( 'NONE',  ( -190.6985136298601731, 109.1272424661242582, 94.99999999999866418 ) ) ;
#61898=CARTESIAN_POINT ( 'NONE',  ( 36.17848201055296897, 9.023908545482070664, -89.98582735140863065 ) ) ;
#61899=CARTESIAN_POINT ( 'NONE',  ( 132.7179291807800325, 40.74118679001687582, -77.78442630836887872 ) ) ;
#61902=CARTESIAN_POINT ( 'NONE',  ( -8.314488422519710653, 7.931352979988687935, 56.96013162991090439 ) ) ;
#61904=CARTESIAN_POINT ( 'NONE',  ( -156.6644740249450649, 71.86407434531901117, -44.57184474382414408 ) ) ;
#61905=CARTESIAN_POINT ( 'NONE',  ( 210.5008983495072243, 116.4753531594351159, -12.22384055568752892 ) ) ;
#61907=CARTESIAN_POINT ( 'NONE',  ( -3.862560291631543574, 7.672660553664872651, 31.24333188717660192 ) ) ;
#61908=CARTESIAN_POINT ( 'NONE',  ( 57.45325234994688657, 11.45088831722005906, 85.96000542775017550 ) ) ;
#61909=CARTESIAN_POINT ( 'NONE',  ( -49.43915770973592316, 13.24768844696975378, -64.56308494239007700 ) ) ;
#61910=CARTESIAN_POINT ( 'NONE',  ( 206.6955592216990851, 109.1214665502618146, -51.06646129112117904 ) ) ;
#61911=CARTESIAN_POINT ( 'NONE',  ( 178.1903523079566298, 75.72906488635186406, 3.031147140003530804 ) ) ;
#61912=CARTESIAN_POINT ( 'NONE',  ( -58.96922974609610435, 15.76655591015166102, 4.571986130225868195 ) ) ;
#61916=EDGE_LOOP ( 'NONE', ( #51975, #41978 ) ) ;
#61919=CARTESIAN_POINT ( 'NONE',  ( 45.49006904354232717, 9.279592366778889101, 59.87143817380967192 ) ) ;
#61921=CARTESIAN_POINT ( 'NONE',  ( -4.675860265596308629, 6.706201026861161374, 84.49030423809293211 ) ) ;
#61925=FACE_OUTER_BOUND ( 'NONE', #54160, .T. ) ;
#61926=CARTESIAN_POINT ( 'NONE',  ( -165.7138623879809529, 79.24467249981145756, 66.38117368143906560 ) ) ;
#61927=ORIENTED_EDGE ( 'NONE', *, *, #47825, .T. ) ;
#61932=B_SPLINE_CURVE_WITH_KNOTS ( 'NONE', 3,
 ( #27725, #45297, #23159, #12962, #66439, #65375, #28071, #2059, #17161, #6268, #50579, #55868, #66783, #2400, #49875, #1701, #40028, #49163, #33718, #1002, #22454, #6974, #43893, #38635, #18227, #54802, #44608, #1350, #60077, #12255, #55504, #11895, #33375, #22803, #6623, #44248, #17878, #65729, #39336, #60779, #12603, #34062, #7331 ),
 .UNSPECIFIED., .F., .F.,
 ( 4, 2, 2, 2, 2, 2, 2, 2, 1, 2, 2, 2, 2, 2, 2, 2, 2, 2, 2, 2, 2, 4 ),
 ( 3.469446951953614189E-18, 0.001466285743483492117, 0.002199428615225232538, 0.002932571486966972958, 0.004398857230450428646, 0.005865142973933883466, 0.007331428717417340021, 0.008064571589159083911, 0.008797714460900827801, 0.009530857332642571692, 0.01026400020438431732, 0.01173028594786780857, 0.01319657169135129808, 0.01466285743483479106, 0.01539600030657653496, 0.01612914317831827885, 0.01759542892180177009, 0.01906171466528526134, 0.01979485753702700870, 0.02052800040876874912, 0.02199428615225223343, 0.02346057189573571775 ),
 .UNSPECIFIED. ) ;
#61942=CARTESIAN_POINT ( 'NONE',  ( 56.52205390515081262, 12.28646189164059344, -12.59121248216328581 ) ) ;
#61943=EDGE_LOOP ( 'NONE', ( #56137, #50435, #6820, #26864 ) ) ;
#61944=CARTESIAN_POINT ( 'NONE',  ( 204.6977192012829789, 106.3443248447423457, -63.17048162308526571 ) ) ;
#61945=CARTESIAN_POINT ( 'NONE',  ( 21.44191228441539465, 7.755009954762289937, -47.97187036235548163 ) ) ;
#61946=CARTESIAN_POINT ( 'NONE',  ( 9.280894575734579988, 7.385644305345136829, 60.59831840680561044 ) ) ;
#61948=FACE_BOUND ( 'NONE', #18286, .T. ) ;
#61949=EDGE_LOOP ( 'NONE', ( #31481, #22260 ) ) ;
#61952=CARTESIAN_POINT ( 'NONE',  ( 89.87840278991589571, 21.62393877508910478, -50.08560210100184662 ) ) ;
#61954=CARTESIAN_POINT ( 'NONE',  ( -177.5288247523079121, 93.72924674643515175, 17.56298962112507667 ) ) ;
#61955=CARTESIAN_POINT ( 'NONE',  ( 12.60449501160847774, 6.419572319999807597, 84.40508385186305418 ) ) ;
#61956=EDGE_CURVE ( 'NONE', #18072, #60434, #3832, .T. ) ;
#61957=CARTESIAN_POINT ( 'NONE',  ( 79.38020582286198135, 17.07365509555548400, -72.15476770513920712 ) ) ;
#61960=CYLINDRICAL_SURFACE ( 'NONE', #34824, 7.500000000000020428 ) ;
#61961=CARTESIAN_POINT ( 'NONE',  ( 198.4059165548111991, 99.71594270191987164, -39.73513461452476037 ) ) ;
#61967=CARTESIAN_POINT ( 'NONE',  ( 89.65730223173022750, 21.54473673261222189, -77.03190999791871718 ) ) ;
#61969=VERTEX_POINT ( 'NONE', #27968 ) ;
#61972=CARTESIAN_POINT ( 'NONE',  ( 46.84154678921880333, 10.51341196666389344, 63.27653607351307841 ) ) ;
#61974=CARTESIAN_POINT ( 'NONE',  ( 102.7983318509014765, 26.68040613344513190, 9.220450153127773163 ) ) ;
#61980=CARTESIAN_POINT ( 'NONE',  ( 174.1422537179815038, 73.24254491731257133, -73.42316486936464059 ) ) ;
#61982=CARTESIAN_POINT ( 'NONE',  ( 117.4696399285658686, 32.37118663718647582, -18.65062314217833617 ) ) ;
#61984=CARTESIAN_POINT ( 'NONE',  ( 83.37782009939536465, 19.39546426214657870, -36.55869151441629583 ) ) ;
#61990=CARTESIAN_POINT ( 'NONE',  ( 179.4227152810058215, 78.36166152262364903, 2.638148450095675557 ) ) ;
#61993=CARTESIAN_POINT ( 'NONE',  ( 126.4083787442700242, 37.10531539900949127, 9.140475197704560628 ) ) ;
#61995=CARTESIAN_POINT ( 'NONE',  ( 202.8553521992888307, 105.5342351882353142, 83.10660119179087246 ) ) ;
#61997=CARTESIAN_POINT ( 'NONE',  ( 210.5008983495071675, 116.4753531594350875, 41.46526062523980727 ) ) ;
#61998=CARTESIAN_POINT ( 'NONE',  ( -79.14094329813313777, 23.58034730000056811, 57.26275173013680586 ) ) ;
#61999=CARTESIAN_POINT ( 'NONE',  ( -14.32120159453989672, 7.401444311907543927, 33.85853709894156793 ) ) ;
#62004=FACE_OUTER_BOUND ( 'NONE', #60996, .T. ) ;
#62005=B_SPLINE_CURVE_WITH_KNOTS ( 'NONE', 3,
 ( #64067, #59472, #15879, #48552, #27823, #746, #49260, #22200, #43638, #33470, #65467, #17259, #6715, #14345, #62170, #22896, #40713, #60532, #19970, #17620, #30868, #57250, #3436, #62531, #51288, #52311, #61819, #40376, #9065, #12346, #19612, #13992, #55243, #33802, #3102, #35098, #24900, #7066, #18925, #36140, #41072, #24563, #13642, #45996, #41421, #62875 ),
 .UNSPECIFIED., .F., .F.,
 ( 4, 2, 2, 2, 2, 2, 2, 2, 2, 2, 2, 2, 2, 2, 2, 2, 2, 2, 2, 2, 2, 2, 4 ),
 ( 0.000000000000000000, 0.003373244802897266970, 0.004216556003621581977, 0.005059867204345896985, 0.006746489605794529602, 0.007589800806518840273, 0.008433112007243148342, 0.009276423207967458145, 0.01011973440869176621, 0.01180635681014038582, 0.01349297921158900196, 0.01433629041231331176, 0.01517960161303762504, 0.01686622401448622730, 0.01770953521521050761, 0.01855284641593478792, 0.02023946881738338324, 0.02108278001810766356, 0.02192609121883194040, 0.02361271362028050450, 0.02445602482100478481, 0.02529933602172906165, 0.02698595842317762575 ),
 .UNSPECIFIED. ) ;
#62007=CARTESIAN_POINT ( 'NONE',  ( -31.43908319763710679, -170.0000000000000000, -15.97264677473816974 ) ) ;
#62008=CARTESIAN_POINT ( 'NONE',  ( 181.9295958320008424, 80.90438706151871884, -78.03393500570973629 ) ) ;
#62009=CARTESIAN_POINT ( 'NONE',  ( -38.85841857822266121, 11.95291994873726971, 92.55007051657004524 ) ) ;
#62010=CARTESIAN_POINT ( 'NONE',  ( -78.66644367742111399, 22.32174330031318732, -88.80455181264524356 ) ) ;
#62011=CARTESIAN_POINT ( 'NONE',  ( 35.65775178405255730, 7.951994368745585184, -49.62299231391522625 ) ) ;
#62012=CARTESIAN_POINT ( 'NONE',  ( -109.3553681454883844, 36.52260784104395697, 8.634393988911380546 ) ) ;
#62013=CARTESIAN_POINT ( 'NONE',  ( 10.83521140779424030, 7.398743030771589346, -48.67192843401519298 ) ) ;
#62014=CARTESIAN_POINT ( 'NONE',  ( 133.3990214534116774, 41.14886683286417934, -51.01281999844796644 ) ) ;
#62018=CARTESIAN_POINT ( 'NONE',  ( 186.2922852436126959, 85.51514452367332808, 85.09180308946348248 ) ) ;
#62021=CARTESIAN_POINT ( 'NONE',  ( -27.70005010046228122, 9.007417901453017350, -63.15562276199040781 ) ) ;
#62022=EDGE_CURVE ( 'NONE', #11917, #11797, #29876, .T. ) ;
#62026=CARTESIAN_POINT ( 'NONE',  ( 8.540853903193186270, 6.376814430361481101, 12.61568352143839533 ) ) ;
#62029=CARTESIAN_POINT ( 'NONE',  ( -61.52761555060400411, 17.56359742150277725, -73.37817215718246189 ) ) ;
#62030=CARTESIAN_POINT ( 'NONE',  ( 198.7129816317746247, 100.1061386900356069, -66.14231288720782231 ) ) ;
#62031=VECTOR ( 'NONE', #31969, 1000.000000000000000 ) ;
#62032=CARTESIAN_POINT ( 'NONE',  ( -180.5231752320737257, 95.76423526868921954, -40.96427428279935157 ) ) ;
#62034=CARTESIAN_POINT ( 'NONE',  ( -23.99957301099517437, 9.503061049698491303, 63.57851690664559641 ) ) ;
#62036=CARTESIAN_POINT ( 'NONE',  ( -51.13073217147959326, 13.66490163179658879, 71.05935392568744646 ) ) ;
#62037=AXIS2_PLACEMENT_3D ( 'NONE', #33303, #66707, #44539 ) ;
#62038=CARTESIAN_POINT ( 'NONE',  ( -1.314022807222069877, 6.554273999800678929, 68.21404729449294280 ) ) ;
#62039=ORIENTED_EDGE ( 'NONE', *, *, #49593, .F. ) ;
#62042=CARTESIAN_POINT ( 'NONE',  ( -108.9444157621017979, 37.44493815491209432, -65.88002215714232079 ) ) ;
#62045=DIRECTION ( 'NONE',  ( -0.000000000000000000, 1.000000000000000000, -0.000000000000000000 ) ) ;
#62049=CARTESIAN_POINT ( 'NONE',  ( -173.1211646369891355, 88.63826465341151106, 3.977144016177345254 ) ) ;
#62053=CARTESIAN_POINT ( 'NONE',  ( 155.2870855780215038, 57.23765125306422163, 44.09879959064866028 ) ) ;
#62054=LINE ( 'NONE', #18809, #59434 ) ;
#62056=DIRECTION ( 'NONE',  ( -0.000000000000000000, 1.000000000000000000, -0.000000000000000000 ) ) ;
#62057=CARTESIAN_POINT ( 'NONE',  ( -173.5394735271662228, 87.59446374803708579, 3.977144016177343477 ) ) ;
#62060=CARTESIAN_POINT ( 'NONE',  ( -85.12122836439577611, 25.97531040437158367, 41.76940575333474470 ) ) ;
#62061=CARTESIAN_POINT ( 'NONE',  ( -24.18158274621862702, 9.527343002918316373, -17.92767438152212023 ) ) ;
#62062=CARTESIAN_POINT ( 'NONE',  ( 141.2894128405439176, 46.09731134920846074, 11.20330446142119207 ) ) ;
#62064=B_SPLINE_CURVE_WITH_KNOTS ( 'NONE', 3,
 ( #9867, #30630, #4246, #41526, #36940, #52076, #58380, #62978, #31325, #3893, #10189, #31654, #25364, #4576, #53090, #68268, #20073, #14785 ),
 .UNSPECIFIED., .F., .F.,
 ( 4, 2, 2, 2, 2, 2, 2, 2, 4 ),
 ( 0.01384554320395945531, 0.01548911742118727966, 0.01713269163841510401, 0.02041984007287080127, 0.02206341429009864297, 0.02370698850732648119, 0.02452877561594040551, 0.02535056272455432289, 0.02699413694178218540 ),
 .UNSPECIFIED. ) ;
#62065=CARTESIAN_POINT ( 'NONE',  ( 116.8937673311172603, 32.08228998570057655, -46.89815673556866216 ) ) ;
#62067=CARTESIAN_POINT ( 'NONE',  ( 42.49453823366106064, 8.831814337191470798, -36.28277223276639063 ) ) ;
#62068=CARTESIAN_POINT ( 'NONE',  ( -73.37451557318128437, 21.44378618812643467, 86.28309517344128210 ) ) ;
#62071=CARTESIAN_POINT ( 'NONE',  ( 79.11678624235125312, 16.99307331934756604, -43.31297501014353202 ) ) ;
#62076=VECTOR ( 'NONE', #40033, 1000.000000000000000 ) ;
#62078=CARTESIAN_POINT ( 'NONE',  ( 80.16761386260780853, 18.37011649821943848, 33.37197744852545611 ) ) ;
#62083=CARTESIAN_POINT ( 'NONE',  ( -119.1795380580999648, 42.22910606512927956, 61.61258993744711177 ) ) ;
#62084=CARTESIAN_POINT ( 'NONE',  ( -83.15209219203882185, 25.16621997697718882, -9.740531383382071695 ) ) ;
#62085=CARTESIAN_POINT ( 'NONE',  ( -179.5186635612084274, 96.12511541314945873, -11.41482807252975462 ) ) ;
#62088=CARTESIAN_POINT ( 'NONE',  ( -54.08488990389049889, 15.46443908526321209, 30.36440728263135469 ) ) ;
#62090=ORIENTED_EDGE ( 'NONE', *, *, #30117, .T. ) ;
#62096=FACE_OUTER_BOUND ( 'NONE', #34509, .T. ) ;
#62097=CARTESIAN_POINT ( 'NONE',  ( 188.5843222076478582, 86.53342480589839170, -43.42845138699213692 ) ) ;
#62098=CARTESIAN_POINT ( 'NONE',  ( 18.19980344696536889, 6.589834367837007711, 30.40873729102910517 ) ) ;
#62099=CARTESIAN_POINT ( 'NONE',  ( 157.4703587214989113, 57.65129005721576050, -62.96873488960130771 ) ) ;
#62103=DIRECTION ( 'NONE',  ( 0.000000000000000000, 0.000000000000000000, 1.000000000000000000 ) ) ;
#62104=CARTESIAN_POINT ( 'NONE',  ( 180.4006926312003714, 77.91522284673895626, -89.91415884680702675 ) ) ;
#62106=CARTESIAN_POINT ( 'NONE',  ( 70.25990036603481315, 14.47042233282420476, -41.26302775415978630 ) ) ;
#62107=LINE ( 'NONE', #13246, #14231 ) ;
#62108=CARTESIAN_POINT ( 'NONE',  ( -57.42826130032240428, 16.37596353166460261, 30.69935087320815015 ) ) ;
#62109=CARTESIAN_POINT ( 'NONE',  ( -38.45778834351241215, 11.87434869453508135, -67.00674613719260719 ) ) ;
#62110=CARTESIAN_POINT ( 'NONE',  ( 59.30258796551117939, 12.87111270082601067, 30.77794280086910206 ) ) ;
#62112=VERTEX_POINT ( 'NONE', #36724 ) ;
#62113=CARTESIAN_POINT ( 'NONE',  ( -4.955782654901476292, 6.720825733572403315, -49.86023888739470067 ) ) ;
#62114=CARTESIAN_POINT ( 'NONE',  ( 39.40195752203892710, -170.0000000000000000, -35.61981746542776506 ) ) ;
#62117=CARTESIAN_POINT ( 'NONE',  ( 126.6395826915640015, 37.23416510613628105, -18.73613604440101454 ) ) ;
#62119=FACE_OUTER_BOUND ( 'NONE', #23584, .T. ) ;
#62125=CARTESIAN_POINT ( 'NONE',  ( 133.8566784816069344, 42.60093787723652525, -51.02331093239568816 ) ) ;
#62126=CARTESIAN_POINT ( 'NONE',  ( -33.36965723649377225, 10.93726715887724055, -50.06857660072027727 ) ) ;
#62129=CARTESIAN_POINT ( 'NONE',  ( 181.0840389613909451, 80.03940679743416808, -36.22505766587961062 ) ) ;
#62133=CARTESIAN_POINT ( 'NONE',  ( -30.47069031368415182, 9.433993659086596040, -23.42594627002974050 ) ) ;
#62137=AXIS2_PLACEMENT_3D ( 'NONE', #62391, #57119, #36006 ) ;
#62138=CARTESIAN_POINT ( 'NONE',  ( 150.1388893866326555, 53.40890567970688352, 88.97308815910281510 ) ) ;
#62140=CARTESIAN_POINT ( 'NONE',  ( 127.2358066117906787, 38.72257733469223950, -73.92861135475047263 ) ) ;
#62142=CARTESIAN_POINT ( 'NONE',  ( -152.5101325120252795, 68.10842280990928543, 45.10774975830220512 ) ) ;
#62147=EDGE_LOOP ( 'NONE', ( #10053, #55661 ) ) ;
#62149=CARTESIAN_POINT ( 'NONE',  ( -7.825402957745085430, 7.899365992529253866, -89.10717191287116634 ) ) ;
#62150=ORIENTED_EDGE ( 'NONE', *, *, #6413, .F. ) ;
#62151=ORIENTED_EDGE ( 'NONE', *, *, #48372, .F. ) ;
#62152=CARTESIAN_POINT ( 'NONE',  ( -168.7314919967217861, 83.83749564070828342, 17.57661599061045976 ) ) ;
#62153=CARTESIAN_POINT ( 'NONE',  ( 16.77391662606471101, 6.533867394142991891, -62.41210858207633549 ) ) ;
#62154=CARTESIAN_POINT ( 'NONE',  ( -132.2161740628506550, 52.03204870034955576, 60.92179302142604769 ) ) ;
#62155=VERTEX_POINT ( 'NONE', #41646 ) ;
#62156=DIRECTION ( 'NONE',  ( -0.000000000000000000, 1.000000000000000000, -0.000000000000000000 ) ) ;
#62158=VERTEX_POINT ( 'NONE', #37056 ) ;
#62159=CARTESIAN_POINT ( 'NONE',  ( 178.3500803230180907, 77.29460076174662220, -90.39474168206896820 ) ) ;
#62160=ADVANCED_FACE ( 'NONE', ( #68388 ), #47591, .F. ) ;
#62161=CARTESIAN_POINT ( 'NONE',  ( 138.2136629441929472, 45.30947856186676859, 30.88737808275690355 ) ) ;
#62163=CARTESIAN_POINT ( 'NONE',  ( 115.7731501832035832, 32.64791439093733061, 32.02106840025158618 ) ) ;
#62165=CARTESIAN_POINT ( 'NONE',  ( 63.98689050258322908, 13.93365232918667651, -62.61274692488039051 ) ) ;
#62170=CARTESIAN_POINT ( 'NONE',  ( -143.2587158300142107, 60.34092810886538416, -11.31239974830817374 ) ) ;
#62171=CARTESIAN_POINT ( 'NONE',  ( -124.1007047332777802, 46.52282960291164216, -49.71035901984455307 ) ) ;
#62172=CARTESIAN_POINT ( 'NONE',  ( 63.01563776193091826, -170.0000000000000000, -62.56524142263340593 ) ) ;
#62174=B_SPLINE_CURVE_WITH_KNOTS ( 'NONE', 3,
 ( #52158, #11218, #27396, #3975, #64344, #32349, #58712, #46884, #10528, #53775, #37260, #43576, #21775, #69280, #16844, #48152, #21107, #42549, #27672, #64698, #10879, #62721, #64006, #32002, #59407, #53433, #14526, #32685, #48834, #5262, #681, #35985, #54747, #49463, #58983, #16767, #60388, #596, #33667, #28019, #48760, #43840, #12202, #55095, #64269, #27317, #60023, #59667, #37888, #43148, #22750, #28371, #59332, #38226, #1642, #49818, #11480, #32952, #10802, #38943, #32272, #21699, #65674, #53702, #54391, #37532 ),
 .UNSPECIFIED., .F., .F.,
 ( 4, 2, 2, 2, 2, 2, 2, 2, 2, 2, 2, 2, 2, 2, 2, 2, 2, 2, 2, 2, 2, 2, 2, 2, 2, 2, 2, 2, 2, 2, 2, 2, 4 ),
 ( 0.000000000000000000, 0.001357572341309158485, 0.002036358511963770688, 0.002715144682618383324, 0.004072717023927597754, 0.005430289365236812618, 0.006109075535891419183, 0.006787861706546025747, 0.008145434047855280510, 0.009503006389164535272, 0.01018179255981917393, 0.01086057873047381259, 0.01221815107178313153, 0.01357572341309244701, 0.01629086809571106409, 0.01900601277832967770, 0.02172115746094829478, 0.02443630214356691185, 0.02715144682618552546, 0.02986659150880414254, 0.03122416385011346496, 0.03258173619142278737, 0.03393930853273210979, 0.03529688087404143221, 0.03665445321535075462, 0.03733323938600540542, 0.03801202555666004929, 0.03869081172731469315, 0.03936959789796934395, 0.04004838406862398781, 0.04072717023927863861, 0.04208474258058787082, 0.04344231492189710303 ),
 .UNSPECIFIED. ) ;
#62175=CARTESIAN_POINT ( 'NONE',  ( -51.00284195030131684, 13.63270405836958155, -90.07839450250217794 ) ) ;
#62176=CARTESIAN_POINT ( 'NONE',  ( -48.20191234209509901, 13.98522789163153135, -93.32217931443403813 ) ) ;
#62178=CARTESIAN_POINT ( 'NONE',  ( -144.2029146819477887, 59.80706661873674079, 43.54475530746405809 ) ) ;
#62180=CARTESIAN_POINT ( 'NONE',  ( -170.2801941679960294, 84.02053682015868219, -76.01052631320209230 ) ) ;
#62183=CARTESIAN_POINT ( 'NONE',  ( -105.8683518445188412, 35.77995342500074827, 31.41595196880235008 ) ) ;
#62185=CARTESIAN_POINT ( 'NONE',  ( -174.6805680479237424, 88.88026187971797754, -88.55446335397090252 ) ) ;
#62187=CARTESIAN_POINT ( 'NONE',  ( 81.05403189674304087, 18.64820877954959499, 59.01636669307008276 ) ) ;
#62194=CARTESIAN_POINT ( 'NONE',  ( 32.90878072717891456, 7.653588083204819092, 14.33083675908082988 ) ) ;
#62203=DIRECTION ( 'NONE',  ( 0.000000000000000000, 0.000000000000000000, 1.000000000000000000 ) ) ;
#62204=VERTEX_POINT ( 'NONE', #4365 ) ;
#62206=CARTESIAN_POINT ( 'NONE',  ( -14.19493007850032740, 7.389842975086044596, -73.72984886113263769 ) ) ;
#62207=CARTESIAN_POINT ( 'NONE',  ( -34.51918258780366244, 10.11719938103012595, 30.87373719683911588 ) ) ;
#62208=CARTESIAN_POINT ( 'NONE',  ( -24.93568128341083678, 8.613819379861709535, 68.32887008604041057 ) ) ;
#62211=CARTESIAN_POINT ( 'NONE',  ( -152.4930836497867119, 68.09400557494207362, 58.18155450450962007 ) ) ;
#62215=CARTESIAN_POINT ( 'NONE',  ( -179.5186635612084558, 96.12511541314940189, -65.10392925345711035 ) ) ;
#62216=CARTESIAN_POINT ( 'NONE',  ( 130.0051068477732485, 40.31041537049797086, 84.25595455720329596 ) ) ;
#62217=CARTESIAN_POINT ( 'NONE',  ( 114.6890011751076202, 30.99337387307411262, 43.17062650260461254 ) ) ;
#62218=CARTESIAN_POINT ( 'NONE',  ( 90.45368079632972069, 20.76052788962625328, -90.50765348280665989 ) ) ;
#62224=CARTESIAN_POINT ( 'NONE',  ( 66.29961816943399810, 13.45804302849873224, 57.39740238740354528 ) ) ;
#62231=CARTESIAN_POINT ( 'NONE',  ( 164.9540180502650628, 65.02981548735056094, -16.21117244928680989 ) ) ;
#62235=CARTESIAN_POINT ( 'NONE',  ( 66.73431804020509617, 14.60294556126671672, 57.63975947924529208 ) ) ;
#62241=CARTESIAN_POINT ( 'NONE',  ( 164.6598737201887559, 64.78038692612517480, -45.83041859628480097 ) ) ;
#62243=CARTESIAN_POINT ( 'NONE',  ( 164.9697211531229755, 63.72502658717166213, -43.92099099202817314 ) ) ;
#62245=DIRECTION ( 'NONE',  ( 0.000000000000000000, 0.000000000000000000, -1.000000000000000000 ) ) ;
#62247=ADVANCED_FACE ( 'NONE', ( #58494 ), #25486, .F. ) ;
#62249=CARTESIAN_POINT ( 'NONE',  ( 157.4703587214989113, 58.92748579479259519, -89.81328548006499091 ) ) ;
#62250=CARTESIAN_POINT ( 'NONE',  ( 81.05403189674299824, 18.64820877954959499, -21.51728507832098103 ) ) ;
#62251=CARTESIAN_POINT ( 'NONE',  ( -173.9107726370295381, 89.52858981106767544, -88.43244303168964393 ) ) ;
#62252=CARTESIAN_POINT ( 'NONE',  ( 150.4550062612853480, 52.39582885725847916, 66.45880062188886939 ) ) ;
#62253=CARTESIAN_POINT ( 'NONE',  ( 93.72059824125564376, 23.03897520779757713, 39.70469307016926308 ) ) ;
#62256=CARTESIAN_POINT ( 'NONE',  ( -96.76336539645312484, 31.18045094643429493, 59.75870862236858017 ) ) ;
#62257=CARTESIAN_POINT ( 'NONE',  ( -11.79249160485394299, 8.191429102467033374, 70.82980661725612492 ) ) ;
#62259=EDGE_CURVE ( 'NONE', #37698, #34548, #31357, .T. ) ;
#62260=CARTESIAN_POINT ( 'NONE',  ( 150.9128604434957595, 53.97103482421773180, -20.45779706337464887 ) ) ;
#62262=CARTESIAN_POINT ( 'NONE',  ( 109.3154830994003390, 29.56170298203815605, 29.65404401712086013 ) ) ;
#62263=CARTESIAN_POINT ( 'NONE',  ( -1.096061481932295356, 7.553048580900439291, 34.29492952217174206 ) ) ;
#62266=CARTESIAN_POINT ( 'NONE',  ( 210.1954643503416094, 114.1986276268024056, -38.71856909762487930 ) ) ;
#62267=CARTESIAN_POINT ( 'NONE',  ( 177.7889574972181777, 75.33777460203559428, 3.211639890609760517 ) ) ;
#62268=CARTESIAN_POINT ( 'NONE',  ( -55.54058841405665703, 14.81234591756537355, 18.47277718246749956 ) ) ;
#62273=CARTESIAN_POINT ( 'NONE',  ( 104.3931729003987101, 26.26823401847089201, -65.54728805928756685 ) ) ;
#62275=CARTESIAN_POINT ( 'NONE',  ( 46.89016064832838993, 10.52130577388959054, -16.76345691462488929 ) ) ;
#62276=CARTESIAN_POINT ( 'NONE',  ( 44.86216938219161676, 9.182565662897493652, 59.11098717133123870 ) ) ;
#62278=CARTESIAN_POINT ( 'NONE',  ( -10.07658142808628199, 7.047931155041471385, 84.14318101103907566 ) ) ;
#62280=EDGE_CURVE ( 'NONE', #12765, #14559, #49020, .T. ) ;
#62282=CARTESIAN_POINT ( 'NONE',  ( -109.7811201291769834, 37.90784085457606523, -15.43969849781013259 ) ) ;
#62285=CARTESIAN_POINT ( 'NONE',  ( 55.97663400285460256, 12.17578876026178669, -94.18817934799618286 ) ) ;
#62287=ORIENTED_EDGE ( 'NONE', *, *, #62829, .F. ) ;
#62291=CARTESIAN_POINT ( 'NONE',  ( -156.0300823189602681, 69.91528270335483342, 34.48016162486435832 ) ) ;
#62293=CARTESIAN_POINT ( 'NONE',  ( 173.6020601204682237, 71.36108012062133810, -16.28340663019495338 ) ) ;
#62294=CARTESIAN_POINT ( 'NONE',  ( -172.7173255566596879, 88.18461381371093921, 57.66624519710471475 ) ) ;
#62295=VECTOR ( 'NONE', #19152, 1000.000000000000000 ) ;
#62297=CARTESIAN_POINT ( 'NONE',  ( 56.94505604581134861, 12.37336791557970805, -20.78740111288298564 ) ) ;
#62301=CARTESIAN_POINT ( 'NONE',  ( 208.9507214515059559, 112.3605999017435124, 3.669543826566413980 ) ) ;
#62302=CARTESIAN_POINT ( 'NONE',  ( -142.5087559769085033, 59.74468185400777998, 40.96956311530343697 ) ) ;
#62304=FACE_BOUND ( 'NONE', #59912, .T. ) ;
#62308=CARTESIAN_POINT ( 'NONE',  ( -118.4647292297932495, 42.97137042695754161, 90.72527677266357671 ) ) ;
#62309=CARTESIAN_POINT ( 'NONE',  ( 33.77444274891860942, 8.756048688386677270, -74.92843515396829446 ) ) ;
#62310=CARTESIAN_POINT ( 'NONE',  ( -179.2210908201800237, 95.76260491022608790, 15.86921790254495335 ) ) ;
#62311=CARTESIAN_POINT ( 'NONE',  ( 205.5049354810107047, 109.1776577097391652, 56.05227132923312894 ) ) ;
#62312=CARTESIAN_POINT ( 'NONE',  ( 79.52861599156693728, 17.11914630560287875, -72.63190030141871034 ) ) ;
#62313=VERTEX_POINT ( 'NONE', #40778 ) ;
#62315=CARTESIAN_POINT ( 'NONE',  ( 198.2588776805010298, 99.52972231602373654, -47.68225496974167754 ) ) ;
#62317=CARTESIAN_POINT ( 'NONE',  ( -86.09999398724995956, 25.29376521564874380, 12.10207219235686793 ) ) ;
#62321=CARTESIAN_POINT ( 'NONE',  ( -86.09999398724994535, 25.29376521564874025, -68.43157957903414967 ) ) ;
#62326=CARTESIAN_POINT ( 'NONE',  ( 15.78827728214693416, 6.500811158483327468, -35.51894409868578606 ) ) ;
#62328=CARTESIAN_POINT ( 'NONE',  ( 103.1534365798308812, 26.83148826706847601, 12.76670356914313942 ) ) ;
#62337=CARTESIAN_POINT ( 'NONE',  ( -26.19968929187003326, 8.789572452951027515, 86.01030072649960800 ) ) ;
#62338=CARTESIAN_POINT ( 'NONE',  ( -52.00092620775819796, 14.92276858858357258, 4.117465040003481569 ) ) ;
#62342=ADVANCED_FACE ( 'NONE', ( #8438 ), #35512, .F. ) ;
#62343=CARTESIAN_POINT ( 'NONE',  ( 86.62931800182293784, 20.48449268398423584, -35.82156419891171595 ) ) ;
#62344=CARTESIAN_POINT ( 'NONE',  ( -172.3565569771572257, 87.77934603007950898, -88.40105834567737020 ) ) ;
#62345=VERTEX_POINT ( 'NONE', #55931 ) ;
#62346=EDGE_CURVE ( 'NONE', #58885, #19257, #45766, .T. ) ;
#62348=CARTESIAN_POINT ( 'NONE',  ( 46.50704915687943242, 9.440294391580041022, 12.98352632930303407 ) ) ;
#62352=CARTESIAN_POINT ( 'NONE',  ( 129.1381264900934696, 38.64720302602603397, 16.01571092030106414 ) ) ;
#62353=CARTESIAN_POINT ( 'NONE',  ( 38.57272366894952853, 8.302820907903958769, -89.34357163266685120 ) ) ;
#62354=CARTESIAN_POINT ( 'NONE',  ( 201.5359545986093508, 103.7719700437703949, 83.58986283284697549 ) ) ;
#62357=CARTESIAN_POINT ( 'NONE',  ( -106.6940984894958149, 35.07986071359380986, 31.93677410839523034 ) ) ;
#62359=CARTESIAN_POINT ( 'NONE',  ( 12.47451846520756646, 7.423604437114562415, -22.90708336615600160 ) ) ;
#62360=ORIENTED_EDGE ( 'NONE', *, *, #11347, .T. ) ;
#62361=CARTESIAN_POINT ( 'NONE',  ( 203.9181091394787018, 105.2759068139671115, -9.481380442157897548 ) ) ;
#62362=ORIENTED_EDGE ( 'NONE', *, *, #43724, .T. ) ;
#62364=CARTESIAN_POINT ( 'NONE',  ( 187.6511924654682559, 87.00187850361888309, -74.20232582961776302 ) ) ;
#62365=CARTESIAN_POINT ( 'NONE',  ( -144.2155061717025717, 61.10843690942978412, 70.38575101539866807 ) ) ;
#62366=DIRECTION ( 'NONE',  ( -0.000000000000000000, 1.000000000000000000, -0.000000000000000000 ) ) ;
#62368=EDGE_CURVE ( 'NONE', #31528, #43301, #33097, .T. ) ;
#62369=CARTESIAN_POINT ( 'NONE',  ( 36.09137906183516264, 8.001963043161762101, -49.85409025298285712 ) ) ;
#62370=B_SPLINE_CURVE_WITH_KNOTS ( 'NONE', 3,
 ( #45916, #13224, #8290, #13563, #18839, #39945, #7244, #24123, #40294, #45218, #23436, #18490, #29058, #29736, #1978, #50500, #51200, #61399, #28704, #56463, #45565, #34686, #40982, #3013, #44875, #24477, #67385, #19174, #40627, #66358, #12878, #62085, #3353, #56121, #18146, #13902, #39601, #24813, #35365, #23771, #50152, #56827, #7938, #61051 ),
 .UNSPECIFIED., .F., .F.,
 ( 4, 2, 2, 2, 2, 2, 2, 2, 2, 2, 2, 2, 2, 2, 2, 2, 2, 2, 2, 2, 2, 4 ),
 ( 0.02908143158676660192, 0.03095422299093867138, 0.03282701439511073738, 0.03469980579928280684, 0.03657259720345487630, 0.03844538860762694577, 0.04031818001179900829, 0.04125457571388502914, 0.04219097141597105693, 0.04312736711805707779, 0.04359556496910008128, 0.04406376282014309864, 0.04500015852222911256, 0.04593655422431514035, 0.04687294992640116120, 0.04780934562848718206, 0.04968213703265925846, 0.05155492843683133486, 0.05342771984100341126, 0.05530051124517548766, 0.05717330264934757100, 0.05904609405351964740 ),
 .UNSPECIFIED. ) ;
#62372=CARTESIAN_POINT ( 'NONE',  ( 15.78827728214693416, 7.507518794609576496, -35.51894409868578606 ) ) ;
#62374=CARTESIAN_POINT ( 'NONE',  ( 132.0440382699655117, 40.34028297386451811, -50.81529750769279730 ) ) ;
#62377=AXIS2_PLACEMENT_3D ( 'NONE', #22186, #47871, #5646 ) ;
#62380=CARTESIAN_POINT ( 'NONE',  ( -24.41864932425148282, 8.543938959778817122, -67.01132967089127135 ) ) ;
#62381=AXIS2_PLACEMENT_3D ( 'NONE', #49966, #16567, #64410 ) ;
#62382=CARTESIAN_POINT ( 'NONE',  ( 8.336882341125875229, 6.376438415325264231, 9.686664293182547070 ) ) ;
#62383=CARTESIAN_POINT ( 'NONE',  ( 40.38495044702530379, 9.554194848483440694, -77.41568337247169040 ) ) ;
#62388=CARTESIAN_POINT ( 'NONE',  ( -180.6009936245623066, 95.85948119829087943, -41.58058426359100679 ) ) ;
#62390=CARTESIAN_POINT ( 'NONE',  ( -169.1005390226458758, 82.76152663947081578, 17.82399784940768228 ) ) ;
#62391=CARTESIAN_POINT ( 'NONE',  ( -55.05276343752910151, -170.0000000000000000, -96.40542517938723677 ) ) ;
#62392=CARTESIAN_POINT ( 'NONE',  ( -47.56463531432803649, 12.80077789972090052, 65.15204238671329051 ) ) ;
#62395=CARTESIAN_POINT ( 'NONE',  ( -6.851003965218991354, 6.829052369041588300, 57.00742815665407903 ) ) ;
#62398=CARTESIAN_POINT ( 'NONE',  ( 150.9128604434957595, 53.97103482421773180, 60.07585470801640781 ) ) ;
#62399=CARTESIAN_POINT ( 'NONE',  ( -105.8879245385188597, 35.79035667534149923, -62.76632112264718444 ) ) ;
#62400=CARTESIAN_POINT ( 'NONE',  ( -51.35181696773307181, 13.72007042346227657, -49.25810110310893464 ) ) ;
#62402=DIRECTION ( 'NONE',  ( 0.000000000000000000, 0.000000000000000000, 1.000000000000000000 ) ) ;
#62406=ORIENTED_EDGE ( 'NONE', *, *, #68835, .F. ) ;
#62410=DIRECTION ( 'NONE',  ( -0.000000000000000000, 1.000000000000000000, -0.000000000000000000 ) ) ;
#62412=B_SPLINE_CURVE_WITH_KNOTS ( 'NONE', 3,
 ( #48482, #65044, #317, #43218, #58371, #10184, #64003, #31646, #4913, #69278, #10526, #31999, #53431, #26721, #48150, #28852, #6997, #11922, #28094, #44269, #61161, #39357, #38658, #2421, #33395, #65397, #54824, #12982, #44974, #55525, #1370, #13328, #39017, #7705, #12626, #44632, #29151, #49539, #7356, #34785, #60462, #50601, #28811, #1725, #23876, #22828 ),
 .UNSPECIFIED., .F., .F.,
 ( 4, 2, 2, 2, 2, 2, 2, 2, 2, 2, 2, 2, 2, 2, 2, 2, 2, 2, 2, 2, 2, 2, 4 ),
 ( 6.938893903907228378E-18, 0.003192770216278338277, 0.003990962770347912004, 0.004789155324417485732, 0.006385540432556642727, 0.007183732986626235537, 0.007981925540695827478, 0.009578310648835042587, 0.01037650320290463973, 0.01117469575697423514, 0.01197288831104383056, 0.01277108086511342597, 0.01436746597325257689, 0.01596385108139172782, 0.01676204363546130241, 0.01756023618953087700, 0.01835842874360045160, 0.01915662129767002619, 0.02075300640580919273, 0.02234939151394836274, 0.02394577662208753274, 0.02474396917615711428, 0.02554216173022670275 ),
 .UNSPECIFIED. ) ;
#62415=CARTESIAN_POINT ( 'NONE',  ( -125.8938041572051389, -170.0000000000000000, 18.77539728269342945 ) ) ;
#62419=CARTESIAN_POINT ( 'NONE',  ( -82.33596576276352152, 24.83688096733769513, 44.47724042997496952 ) ) ;
#62420=CARTESIAN_POINT ( 'NONE',  ( 150.6448088972535402, 52.53284510403385354, 93.79555634108432116 ) ) ;
#62421=LINE ( 'NONE', #67366, #25302 ) ;
#62422=EDGE_CURVE ( 'NONE', #32318, #5211, #41458, .T. ) ;
#62424=CARTESIAN_POINT ( 'NONE',  ( 117.0065308422768453, 32.13872219870569324, -46.67330633784816740 ) ) ;
#62428=CARTESIAN_POINT ( 'NONE',  ( 44.86216938219162387, 9.182565662897474112, -48.26721519052350828 ) ) ;
#62433=CARTESIAN_POINT ( 'NONE',  ( 68.94309019697860208, 15.16533147648755175, 41.93448570448100554 ) ) ;
#62446=CARTESIAN_POINT ( 'NONE',  ( -55.05276343752909440, 15.72344139423348430, 30.31732777293113301 ) ) ;
#62448=EDGE_LOOP ( 'NONE', ( #29281, #33231 ) ) ;
#62449=CARTESIAN_POINT ( 'NONE',  ( -109.7790042512817621, 37.90666514836943435, 10.88333844894347457 ) ) ;
#62450=CARTESIAN_POINT ( 'NONE',  ( 106.4107271020440209, 27.14892220304138704, 57.50428525336668173 ) ) ;
#62451=CARTESIAN_POINT ( 'NONE',  ( 164.4728833318992542, 63.30716077995683833, 66.45373925860369013 ) ) ;
#62452=FACE_OUTER_BOUND ( 'NONE', #41033, .T. ) ;
#62454=CARTESIAN_POINT ( 'NONE',  ( 16.76400266940279593, 6.533513613209220416, 30.06214509688793157 ) ) ;
#62455=EDGE_CURVE ( 'NONE', #28945, #37023, #35599, .T. ) ;
#62461=CARTESIAN_POINT ( 'NONE',  ( 175.8197560646975717, 73.44385669436823605, -92.05716592950678034 ) ) ;
#62462=DIRECTION ( 'NONE',  ( 0.000000000000000000, 0.000000000000000000, 1.000000000000000000 ) ) ;
#62465=CARTESIAN_POINT ( 'NONE',  ( -37.39246151129641049, 11.66872370876246201, -65.07389322207556859 ) ) ;
#62466=CARTESIAN_POINT ( 'NONE',  ( 187.2384682876462421, 86.54721710842893856, 67.96900511035511272 ) ) ;
#62467=CARTESIAN_POINT ( 'NONE',  ( 12.03317402819681803, 6.409531826169462931, -22.67129521315044727 ) ) ;
#62469=EDGE_LOOP ( 'NONE', ( #60883, #5899, #50119, #7040 ) ) ;
#62470=CARTESIAN_POINT ( 'NONE',  ( -1.083610669212422550, 6.545642299653468221, -39.59529283513472819 ) ) ;
#62474=CARTESIAN_POINT ( 'NONE',  ( 127.2202105166096686, 37.55913282978156786, -20.18205885347246920 ) ) ;
#62476=CARTESIAN_POINT ( 'NONE',  ( 10.15118267943872254, 7.391905976536035539, 5.716968369951990425 ) ) ;
#62481=CARTESIAN_POINT ( 'NONE',  ( 126.6266894765173703, 38.37986986668738609, -41.46026502974351047 ) ) ;
#62486=ORIENTED_EDGE ( 'NONE', *, *, #57328, .F. ) ;
#62488=AXIS2_PLACEMENT_3D ( 'NONE', #20520, #46220, #67698 ) ;
#62489=EDGE_CURVE ( 'NONE', #47113, #51654, #313, .T. ) ;
#62493=CARTESIAN_POINT ( 'NONE',  ( -146.7345109736526467, 61.86270848728295846, -8.496187606269963055 ) ) ;
#62495=EDGE_CURVE ( 'NONE', #51047, #18819, #22123, .T. ) ;
#62497=ORIENTED_EDGE ( 'NONE', *, *, #814, .T. ) ;
#62500=CARTESIAN_POINT ( 'NONE',  ( 159.6439063569485199, 60.64869340040664980, 83.41414359430092418 ) ) ;
#62502=CARTESIAN_POINT ( 'NONE',  ( 132.2818448028689033, 41.65267246304673421, -77.70421314065404772 ) ) ;
#62513=CARTESIAN_POINT ( 'NONE',  ( 173.6007744016332310, 72.73482010729016167, 37.39045840423305833 ) ) ;
#62514=EDGE_CURVE ( 'NONE', #8866, #3372, #26377, .T. ) ;
#62515=CARTESIAN_POINT ( 'NONE',  ( 16.76400266940279238, 6.533513613209218640, -77.31605726496678699 ) ) ;
#62517=CARTESIAN_POINT ( 'NONE',  ( -128.1267916618074594, 49.19573276651586724, 72.13916297000683642 ) ) ;
#62519=CARTESIAN_POINT ( 'NONE',  ( 59.73312635112155533, 12.96464920523511211, 3.707537953021396326 ) ) ;
#62520=DIRECTION ( 'NONE',  ( 0.000000000000000000, 0.000000000000000000, 1.000000000000000000 ) ) ;
#62522=CARTESIAN_POINT ( 'NONE',  ( -61.38706483483510823, 16.47181058798476272, -11.84841205307662371 ) ) ;
#62524=CARTESIAN_POINT ( 'NONE',  ( 141.3556389957210513, 47.34429831367557284, 37.30624493767670913 ) ) ;
#62525=CARTESIAN_POINT ( 'NONE',  ( 110.2429982417149574, 29.99119854320846201, 29.61121420573730489 ) ) ;
#62527=CARTESIAN_POINT ( 'NONE',  ( -100.4466073551323149, 31.85873123265079698, -76.64638814016929302 ) ) ;
#62529=EDGE_LOOP ( 'NONE', ( #464, #52616, #38159, #6518 ) ) ;
#62531=CARTESIAN_POINT ( 'NONE',  ( -142.0860844253783171, 59.41107357617634932, -16.58767256066205675 ) ) ;
#62532=DIRECTION ( 'NONE',  ( -0.000000000000000000, 1.000000000000000000, -0.000000000000000000 ) ) ;
#62539=CARTESIAN_POINT ( 'NONE',  ( 70.41705859591010608, 15.55317472777718102, -44.45805487547348633 ) ) ;
#62540=CARTESIAN_POINT ( 'NONE',  ( -118.4470345550925572, 42.96051736048242731, 37.07762135854807894 ) ) ;
#62541=CARTESIAN_POINT ( 'NONE',  ( -173.1211646369891355, 87.12891641440857882, -61.55650775521367279 ) ) ;
#62544=CARTESIAN_POINT ( 'NONE',  ( -104.5916564445180228, 35.10571011602408475, 45.16936569891448983 ) ) ;
#62546=CARTESIAN_POINT ( 'NONE',  ( -37.92542950990691253, 10.74638084523341952, 7.098505947254272641 ) ) ;
#62548=CARTESIAN_POINT ( 'NONE',  ( 79.54836217416615796, 18.17815803851261691, 61.57198874188753024 ) ) ;
#62554=CARTESIAN_POINT ( 'NONE',  ( 33.44527180510248598, 7.709232309484696621, 5.985868913544964087 ) ) ;
#62555=CARTESIAN_POINT ( 'NONE',  ( -12.77550690612891948, 8.273784096785062658, -48.57362545616927463 ) ) ;
#62556=CARTESIAN_POINT ( 'NONE',  ( -31.43908319763710679, 10.61114334766716283, -8.472646774738153752 ) ) ;
#62558=CARTESIAN_POINT ( 'NONE',  ( -120.5470175916968714, 44.25832081621095426, -90.82375973165250116 ) ) ;
#62561=CARTESIAN_POINT ( 'NONE',  ( -61.77164219855451677, 17.63686644795249592, 68.03177444750755853 ) ) ;
#62562=CARTESIAN_POINT ( 'NONE',  ( -24.32937228292060894, 8.531905774118433428, 8.433788283749800385 ) ) ;
#62565=CARTESIAN_POINT ( 'NONE',  ( -59.45032975077103998, 15.90473825383027418, -90.32613011058693075 ) ) ;
#62566=CARTESIAN_POINT ( 'NONE',  ( -101.8191498210054817, 32.54686850610963234, -23.17002667451226117 ) ) ;
#62567=B_SPLINE_CURVE_WITH_KNOTS ( 'NONE', 3,
 ( #8860, #29605, #19396, #35589, #63005, #52105, #2883, #40507, #24350, #30654, #30310, #45792, #67269, #14126, #46129, #14476, #19055, #8512, #25731, #3919, #67951, #29962, #61955, #40859, #13776, #47161, #4268, #35236, #51424, #3568, #68624, #57046, #41551, #46472, #51759, #20429, #9544, #19747, #56691, #68292, #41209, #67600, #3235, #25039, #57733, #46825, #62669, #41894, #34899, #35931, #57383, #25392, #20098, #14807, #36272, #31004 ),
 .UNSPECIFIED., .F., .F.,
 ( 4, 2, 2, 2, 2, 2, 2, 2, 2, 2, 2, 2, 2, 2, 2, 2, 2, 2, 2, 2, 2, 2, 2, 2, 2, 2, 2, 4 ),
 ( 0.000000000000000000, 0.001960808883428094649, 0.002941213325142143058, 0.003921617766856191033, 0.004902022208570239008, 0.005882426650284287850, 0.006862831091998335825, 0.007843235533712383800, 0.009804044417140516179, 0.01078444885885456589, 0.01176485330056861733, 0.01274525774228266704, 0.01372566218399671849, 0.01470606662571076993, 0.01568647106742481964, 0.01764727995085291212, 0.01960808883428100113, 0.02058849327599503176, 0.02156889771770906239, 0.02254930215942309302, 0.02352970660113712364, 0.02451011104285115080, 0.02549051548456518143, 0.02745132436799324616, 0.02843172880970725944, 0.02941213325142126925, 0.03039253769313528253, 0.03137294213484929234 ),
 .UNSPECIFIED. ) ;
#62568=CARTESIAN_POINT ( 'NONE',  ( 157.4703587214989113, 58.92748579479260229, -36.12418429913763163 ) ) ;
#62569=ORIENTED_EDGE ( 'NONE', *, *, #65655, .F. ) ;
#62571=CARTESIAN_POINT ( 'NONE',  ( -157.0079874970172966, 72.18249880494042259, 65.33901375635429076 ) ) ;
#62573=CARTESIAN_POINT ( 'NONE',  ( -123.4531143159639299, 44.90777521523904880, 31.02450779894023469 ) ) ;
#62576=CARTESIAN_POINT ( 'NONE',  ( 32.99392442438140449, -170.0000000000000000, 94.99999999999866418 ) ) ;
#62577=CARTESIAN_POINT ( 'NONE',  ( 136.3620490432820418, 44.14280731999023288, 83.62320897871926206 ) ) ;
#62579=CARTESIAN_POINT ( 'NONE',  ( 112.1164716692773169, 29.75790342121399590, 44.38885595698212683 ) ) ;
#62582=AXIS2_PLACEMENT_3D ( 'NONE', #21774, #43219, #64697 ) ;
#62586=DIRECTION ( 'NONE',  ( -0.000000000000000000, 1.000000000000000000, -0.000000000000000000 ) ) ;
#62589=CYLINDRICAL_SURFACE ( 'NONE', #39799, 7.500000000000013323 ) ;
#62590=CARTESIAN_POINT ( 'NONE',  ( 140.4769819293526893, 46.76840769395177944, 6.632038057673795173 ) ) ;
#62594=VERTEX_POINT ( 'NONE', #53991 ) ;
#62597=CARTESIAN_POINT ( 'NONE',  ( 159.2258951716709134, 60.31399909112330704, -24.08478607002721006 ) ) ;
#62600=DIRECTION ( 'NONE',  ( -0.8118923937861950435, -0.5838071093367415143, 0.000000000000000000 ) ) ;
#62601=CARTESIAN_POINT ( 'NONE',  ( 141.2703093103738468, 46.08481602256642873, 89.55010852364083007 ) ) ;
#62605=CARTESIAN_POINT ( 'NONE',  ( 160.2883311361769643, 61.16711613734478448, -36.67006685438227720 ) ) ;
#62607=CARTESIAN_POINT ( 'NONE',  ( 160.9241720448058857, 60.38677655937336652, -36.95059568240409931 ) ) ;
#62609=CARTESIAN_POINT ( 'NONE',  ( -61.68940124183720286, 16.56194981783060172, 94.99999999999866418 ) ) ;
#62610=CARTESIAN_POINT ( 'NONE',  ( -131.6133495896317527, 50.37677745548732844, 42.97774246646625329 ) ) ;
#62613=CARTESIAN_POINT ( 'NONE',  ( -166.9982296371934467, 80.56207291422407479, 33.98233018829063923 ) ) ;
#62614=CARTESIAN_POINT ( 'NONE',  ( 150.2809931605061990, 52.27058242113235309, 61.60090139188071845 ) ) ;
#62616=ORIENTED_EDGE ( 'NONE', *, *, #67667, .F. ) ;
#62617=CARTESIAN_POINT ( 'NONE',  ( -99.98584758882475398, 32.75338129098884110, 57.70757149447982215 ) ) ;
#62618=CARTESIAN_POINT ( 'NONE',  ( -9.524904342798462764, 8.016391612076533946, 57.15107637743524549 ) ) ;
#62621=CARTESIAN_POINT ( 'NONE',  ( -55.70465171559254003, 14.85707552169330015, 84.02815862627096521 ) ) ;
#62626=CARTESIAN_POINT ( 'NONE',  ( 185.5412249395996582, 84.70425786166001103, 3.927857500730326912 ) ) ;
#62627=CARTESIAN_POINT ( 'NONE',  ( 210.0292194063021896, 113.9511645670926470, -38.54573400340662914 ) ) ;
#62628=CYLINDRICAL_SURFACE ( 'NONE', #17489, 7.500000000000013323 ) ;
#62634=CARTESIAN_POINT ( 'NONE',  ( 46.90170507415071910, 10.52318308703817884, -15.77993614618464591 ) ) ;
#62638=DIRECTION ( 'NONE',  ( -0.000000000000000000, 1.000000000000000000, -0.000000000000000000 ) ) ;
#62639=CARTESIAN_POINT ( 'NONE',  ( -103.8932886509196720, 34.74144483217663293, -22.99819252106857803 ) ) ;
#62647=CARTESIAN_POINT ( 'NONE',  ( -152.9121563765244503, 67.12206067149024591, 44.90729742860457208 ) ) ;
#62649=CARTESIAN_POINT ( 'NONE',  ( 173.6718135456487460, 71.42581476597410983, -15.69921511153743765 ) ) ;
#62655=ORIENTED_EDGE ( 'NONE', *, *, #63973, .F. ) ;
#62656=CARTESIAN_POINT ( 'NONE',  ( 208.5889601154908917, 111.8333159387241551, 3.437899764226651111 ) ) ;
#62657=CARTESIAN_POINT ( 'NONE',  ( 12.68603346975296198, 7.427591953486040843, 71.19195324979203576 ) ) ;
#62658=CARTESIAN_POINT ( 'NONE',  ( 211.3917124729449881, 115.9987099435923170, 40.10166218625693801 ) ) ;
#62659=CARTESIAN_POINT ( 'NONE',  ( 10.49251118870545874, 6.388821808438093441, -91.38086936670454463 ) ) ;
#62660=EDGE_CURVE ( 'NONE', #57612, #44678, #13185, .T. ) ;
#62665=CARTESIAN_POINT ( 'NONE',  ( -130.9554073334018938, 51.14437639132944469, 86.26655013740494837 ) ) ;
#62666=CARTESIAN_POINT ( 'NONE',  ( -171.0814041607220020, 84.88598211196838861, -22.59712748936987481 ) ) ;
#62667=CARTESIAN_POINT ( 'NONE',  ( -175.1968289912784087, 90.99944698359487916, 18.69656961583812915 ) ) ;
#62668=EDGE_CURVE ( 'NONE', #5375, #38218, #43912, .T. ) ;
#62669=CARTESIAN_POINT ( 'NONE',  ( 23.29087563001241179, 6.856811323692250326, 90.57454065962596701 ) ) ;
#62670=CARTESIAN_POINT ( 'NONE',  ( 81.74909803672913711, 17.81295302817863302, -75.88269741394819334 ) ) ;
#62674=CARTESIAN_POINT ( 'NONE',  ( 204.3091227790962705, 107.5190503136782638, -36.32593103262159673 ) ) ;
#62678=CARTESIAN_POINT ( 'NONE',  ( -31.43908319763710679, -170.0000000000000000, -96.50629854612921577 ) ) ;
#62680=CARTESIAN_POINT ( 'NONE',  ( -58.76099769480629220, 16.75353773354893860, -9.348133756430646812 ) ) ;
#62684=ORIENTED_EDGE ( 'NONE', *, *, #11025, .F. ) ;
#62689=CARTESIAN_POINT ( 'NONE',  ( 103.4725384926516654, 26.96797537091728003, 7.030248456595348472 ) ) ;
#62693=CARTESIAN_POINT ( 'NONE',  ( 174.2468109002382732, 73.34092405459593067, -67.47484041734936966 ) ) ;
#62695=CARTESIAN_POINT ( 'NONE',  ( 102.7571040248401459, 25.57023079238896557, -42.89496695998435172 ) ) ;
#62698=VERTEX_POINT ( 'NONE', #67030 ) ;
#62701=CARTESIAN_POINT ( 'NONE',  ( -86.06525741550316866, 26.37048289224656372, -68.20633391999385253 ) ) ;
#62702=CARTESIAN_POINT ( 'NONE',  ( 173.6700117628887483, 72.79957362875124716, 11.13452001345382314 ) ) ;
#62705=CARTESIAN_POINT ( 'NONE',  ( 136.4532421912245468, 43.01422451910222833, -90.16584641462647198 ) ) ;
#62706=CARTESIAN_POINT ( 'NONE',  ( 33.59857101126895174, 7.725381174399810646, -92.04009980661062684 ) ) ;
#62708=CARTESIAN_POINT ( 'NONE',  ( 210.6592759200687510, 116.7161312026394029, 41.26595981562259396 ) ) ;
#62709=CARTESIAN_POINT ( 'NONE',  ( -86.11230725916333029, 26.39026888680172434, 63.72904867199921597 ) ) ;
#62710=CARTESIAN_POINT ( 'NONE',  ( -102.7502407665687798, 33.01985383847078026, 45.51907450641513719 ) ) ;
#62714=CARTESIAN_POINT ( 'NONE',  ( 203.1420903260745661, 104.2307086582026869, -9.599904899726423579 ) ) ;
#62718=DIRECTION ( 'NONE',  ( -1.000000000000000000, 0.000000000000000000, 0.000000000000000000 ) ) ;
#62720=CARTESIAN_POINT ( 'NONE',  ( 32.90878072717890745, 7.653588083204843073, -39.35826442184654894 ) ) ;
#62721=CARTESIAN_POINT ( 'NONE',  ( 198.5761553035918894, 98.31031792041292761, 86.05966332576983291 ) ) ;
#62723=CARTESIAN_POINT ( 'NONE',  ( 10.13563904803030979, 7.391572367417537315, -38.06542051270953664 ) ) ;
#62724=CARTESIAN_POINT ( 'NONE',  ( 133.3996297101684263, 41.14871796345732236, -36.02331093239567394 ) ) ;
#62729=CARTESIAN_POINT ( 'NONE',  ( -125.8938041572051389, 47.69968343338780414, -8.069153307770243089 ) ) ;
#62730=CARTESIAN_POINT ( 'NONE',  ( -149.5074843970971017, 65.50121172469319220, 18.87627064943540134 ) ) ;
#62731=CARTESIAN_POINT ( 'NONE',  ( -28.13266652174641180, 9.071935854491414375, -62.92545503574774557 ) ) ;
#62734=CARTESIAN_POINT ( 'NONE',  ( 8.951900209438536038, 6.378066731449593796, 7.575917132388738651 ) ) ;
#62738=CARTESIAN_POINT ( 'NONE',  ( 173.5843421840238250, 71.34465141434344559, -70.26636659897270931 ) ) ;
#62739=CARTESIAN_POINT ( 'NONE',  ( -173.1211646369891355, 87.12891641440857882, -49.71195716475001092 ) ) ;
#62740=CARTESIAN_POINT ( 'NONE',  ( 93.92280655489128094, 22.03989931749466180, -18.24301154267179825 ) ) ;
#62741=CARTESIAN_POINT ( 'NONE',  ( -28.13527276074848160, 10.08983026464524357, 57.82341847530290835 ) ) ;
#62750=CARTESIAN_POINT ( 'NONE',  ( -109.7811201291770118, 37.90784085457603680, -69.12879967873752207 ) ) ;
#62751=CARTESIAN_POINT ( 'NONE',  ( -47.80896875121164413, 12.85816703949531181, -40.75691379661022751 ) ) ;
#62753=PLANE ( 'NONE',  #38986 ) ;
#62757=VERTEX_POINT ( 'NONE', #28682 ) ;
#62763=DIRECTION ( 'NONE',  ( -0.000000000000000000, 1.000000000000000000, -0.000000000000000000 ) ) ;
#62767=CARTESIAN_POINT ( 'NONE',  ( -81.90760111942958588, 24.66532273091448246, 44.69847146411395755 ) ) ;
#62770=CARTESIAN_POINT ( 'NONE',  ( 204.6977192012829789, -170.0000000000000000, -63.17048162308526571 ) ) ;
#62772=ORIENTED_EDGE ( 'NONE', *, *, #26494, .F. ) ;
#62774=CARTESIAN_POINT ( 'NONE',  ( 11.82322073186613487, 6.406156243758798219, 57.98838548183650232 ) ) ;
#62776=CARTESIAN_POINT ( 'NONE',  ( 199.7286177451875915, 101.4075663537892069, 31.07105176568274629 ) ) ;
#62777=CARTESIAN_POINT ( 'NONE',  ( -81.12211859130741232, 24.35291027093249383, 84.49380358467659846 ) ) ;
#62784=CARTESIAN_POINT ( 'NONE',  ( 115.7731501832036400, 32.64791439093733061, -75.35713396160309685 ) ) ;
#62786=CARTESIAN_POINT ( 'NONE',  ( 198.2545923567585646, 97.90679023593577313, -74.51984543740591960 ) ) ;
#62787=CARTESIAN_POINT ( 'NONE',  ( -38.54712373114178092, 11.89174538567466932, 62.11797067184914312 ) ) ;
#62788=CARTESIAN_POINT ( 'NONE',  ( -124.9927180788553756, 45.90286323198617424, 72.42390737291080427 ) ) ;
#62789=CARTESIAN_POINT ( 'NONE',  ( -85.89078989036967471, 26.29712602777651398, -17.80139899211184940 ) ) ;
#62791=CARTESIAN_POINT ( 'NONE',  ( -48.58279704072702998, 14.07632445131079635, 41.61883750805020554 ) ) ;
#62796=CARTESIAN_POINT ( 'NONE',  ( 103.1653143050726271, 25.74301230421576747, 66.48834995395209546 ) ) ;
#62797=CARTESIAN_POINT ( 'NONE',  ( 113.6936194768560853, 30.51122948389054201, 84.13335573343988472 ) ) ;
#62808=CARTESIAN_POINT ( 'NONE',  ( -83.14462298835724141, 24.07775853418029754, 58.72718026324421459 ) ) ;
#62810=CARTESIAN_POINT ( 'NONE',  ( 107.5866342775021849, 27.67195717782396969, -90.08692006097672333 ) ) ;
#62811=CARTESIAN_POINT ( 'NONE',  ( -55.54036735998995766, 15.85474597822063991, 45.31732777293116499 ) ) ;
#62813=CARTESIAN_POINT ( 'NONE',  ( -31.93169728792084783, 10.69234447276977562, -62.16174795566553257 ) ) ;
#62815=CARTESIAN_POINT ( 'NONE',  ( -156.6692143066620702, 70.50016761530885390, -17.71246865387325897 ) ) ;
#62816=CARTESIAN_POINT ( 'NONE',  ( 186.5979919519638202, 85.84756789133376742, 68.74285688226639479 ) ) ;
#62817=CARTESIAN_POINT ( 'NONE',  ( 14.80582440982707482, 6.470883766728821485, -8.722983937927098808 ) ) ;
#62819=CARTESIAN_POINT ( 'NONE',  ( -1.314022807222076761, 6.554273999800675377, -39.16415506736178287 ) ) ;
#62820=CARTESIAN_POINT ( 'NONE',  ( 188.4937788906148910, 86.43336847120860966, 64.85195978288442120 ) ) ;
#62822=CARTESIAN_POINT ( 'NONE',  ( 66.30567821786755189, 13.45988234822863205, -63.32099564467209518 ) ) ;
#62823=CARTESIAN_POINT ( 'NONE',  ( 126.8015497489690659, 37.32461426945043570, -19.23696772009197176 ) ) ;
#62825=CARTESIAN_POINT ( 'NONE',  ( 22.28556289340099639, 7.803548444155008035, -19.92885657512854536 ) ) ;
#62826=CARTESIAN_POINT ( 'NONE',  ( 8.679939806240508204, 7.383357464882123189, 13.07472991024607190 ) ) ;
#62829=EDGE_CURVE ( 'NONE', #10603, #67718, #47269, .T. ) ;
#62831=CARTESIAN_POINT ( 'NONE',  ( 185.1647878987785987, 82.82967084668429436, 3.655828051775791288 ) ) ;
#62833=CARTESIAN_POINT ( 'NONE',  ( 127.4669243510812890, 38.85312661085429653, -39.56414112603825117 ) ) ;
#62834=CARTESIAN_POINT ( 'NONE',  ( -128.9786047358386725, 48.55852351614670681, -35.57352493381657865 ) ) ;
#62835=CARTESIAN_POINT ( 'NONE',  ( -107.2385267828037314, 36.51474259889400287, -48.14687793975550534 ) ) ;
#62838=CARTESIAN_POINT ( 'NONE',  ( 186.6075385349484463, 85.85749512876283518, -48.82324223727037804 ) ) ;
#62841=CARTESIAN_POINT ( 'NONE',  ( -142.3178993725748569, 58.31327888234796575, -13.25976637110863443 ) ) ;
#62844=CARTESIAN_POINT ( 'NONE',  ( 151.9622908680735520, 54.74094082471709299, 85.49672239616074876 ) ) ;
#62846=CARTESIAN_POINT ( 'NONE',  ( 133.4058733589413634, 42.32720528873925758, -77.86786152285935714 ) ) ;
#62847=CARTESIAN_POINT ( 'NONE',  ( 126.4083787442699958, 37.10531539900949127, 35.98502578816821540 ) ) ;
#62852=B_SPLINE_CURVE_WITH_KNOTS ( 'NONE', 3,
 ( #34707, #19903, #30118, #50866, #13582, #62108, #67071, #13247, #41359, #8312, #3712, #18865, #7961, #14280, #13924, #40313, #56846, #3039, #39967, #46624, #29415, #51569, #8663, #68099, #3377, #51222, #40653, #61426, #2682, #24500, #67402, #24148, #45590, #9006, #19193, #25189, #35044, #24831, #56486, #35740, #46273, #67749, #62811, #29760 ),
 .UNSPECIFIED., .F., .F.,
 ( 4, 2, 2, 2, 2, 2, 2, 2, 2, 2, 2, 2, 1, 2, 2, 2, 2, 2, 2, 1, 2, 2, 4 ),
 ( 0.02381751147647563974, 0.02531129726520769258, 0.02605819015957371726, 0.02680508305393974541, 0.02829886884267179131, 0.02979265463140384068, 0.03053954752576986884, 0.03128644042013589699, 0.03278022620886796024, 0.03427401199760002348, 0.03576779778633208673, 0.03651469068069810447, 0.03726158357506412222, 0.03800847646943014690, 0.03875536936379617159, 0.04024915515252819320, 0.04174294094126021482, 0.04323672672999225031, 0.04398361962435826111, 0.04473051251872428580, 0.04547740541309029660, 0.04622429830745632129, 0.04771808409618833596 ),
 .UNSPECIFIED. ) ;
#62855=EDGE_CURVE ( 'NONE', #564, #27576, #30621, .T. ) ;
#62858=ORIENTED_EDGE ( 'NONE', *, *, #66176, .F. ) ;
#62859=CARTESIAN_POINT ( 'NONE',  ( -169.8885678771097787, 85.07765565657315676, 4.695052042634683787 ) ) ;
#62860=CARTESIAN_POINT ( 'NONE',  ( -177.1539090641757639, 91.73101548694630480, -9.028362732657411627 ) ) ;
#62863=CARTESIAN_POINT ( 'NONE',  ( -108.8469686167213837, 37.39105600699775778, 88.02876656477920392 ) ) ;
#62866=ORIENTED_EDGE ( 'NONE', *, *, #1181, .F. ) ;
#62867=DIRECTION ( 'NONE',  ( 0.000000000000000000, 0.000000000000000000, 1.000000000000000000 ) ) ;
#62868=CARTESIAN_POINT ( 'NONE',  ( -132.4776673493543058, 52.21763813822162348, -72.85944512281113816 ) ) ;
#62871=CARTESIAN_POINT ( 'NONE',  ( 69.83260694998129736, 15.39825517924929343, -66.92839821032720238 ) ) ;
#62872=ORIENTED_EDGE ( 'NONE', *, *, #47877, .T. ) ;
#62875=CARTESIAN_POINT ( 'NONE',  ( -149.5074843970971017, 65.50121172469319220, -22.96827994102830317 ) ) ;
#62878=CARTESIAN_POINT ( 'NONE',  ( -47.68562151781910785, 12.82916850665305475, -95.00000000000133582 ) ) ;
#62879=CARTESIAN_POINT ( 'NONE',  ( -53.57849794046929759, 15.33131313570892829, -89.04869412804561080 ) ) ;
#62881=CARTESIAN_POINT ( 'NONE',  ( -147.7845268487069177, 62.73119438705055018, 45.53313422460936266 ) ) ;
#62883=CARTESIAN_POINT ( 'NONE',  ( 205.5004956747122549, 107.4493581495447927, 56.08442209846073467 ) ) ;
#62886=CARTESIAN_POINT ( 'NONE',  ( -108.6944271866238978, 37.30738480893074183, 41.93777729395904430 ) ) ;
#62888=CARTESIAN_POINT ( 'NONE',  ( -33.13098007862451055, 9.875138601866705557, 18.18261215273323472 ) ) ;
#62890=CARTESIAN_POINT ( 'NONE',  ( 79.14113188808478583, 18.05280674635441684, 64.54754759442464263 ) ) ;
#62895=CARTESIAN_POINT ( 'NONE',  ( 31.96227686234411181, 7.558148489540048587, 9.588200182408197492 ) ) ;
#62902=CARTESIAN_POINT ( 'NONE',  ( -58.10608953386395825, 15.52134062643866486, 30.96269639377317517 ) ) ;
#62903=CARTESIAN_POINT ( 'NONE',  ( -31.43908319763710679, 9.591432048623756756, -8.472646774738153752 ) ) ;
#62904=CARTESIAN_POINT ( 'NONE',  ( -189.7987719395348734, 107.8653664616570609, 14.45894391646097077 ) ) ;
#62905=DIRECTION ( 'NONE',  ( 0.000000000000000000, 0.000000000000000000, 1.000000000000000000 ) ) ;
#62906=CARTESIAN_POINT ( 'NONE',  ( -55.48029021084977330, 14.79618042659997634, -88.90542517938726519 ) ) ;
#62907=CARTESIAN_POINT ( 'NONE',  ( -101.8145602049405625, 32.54453702486149780, -8.170026674512225640 ) ) ;
#62908=CARTESIAN_POINT ( 'NONE',  ( 149.9883446984744921, 53.30011109831376359, -44.21193250460613910 ) ) ;
#62910=EDGE_CURVE ( 'NONE', #21098, #52425, #43172, .T. ) ;
#62912=ORIENTED_EDGE ( 'NONE', *, *, #9627, .F. ) ;
#62914=AXIS2_PLACEMENT_3D ( 'NONE', #6476, #50433, #1911 ) ;
#62916=CARTESIAN_POINT ( 'NONE',  ( 173.5844030397475706, 72.71952271766126330, -17.18546232013203934 ) ) ;
#62918=CARTESIAN_POINT ( 'NONE',  ( -108.9444157621018405, 37.44493815491210853, 68.34273079517608096 ) ) ;
#62921=CARTESIAN_POINT ( 'NONE',  ( -173.1211646369891071, 88.63826465341152527, -61.55650775521367279 ) ) ;
#62922=CARTESIAN_POINT ( 'NONE',  ( -0.5183605925911975998, 6.525266619725953454, -17.78142633563535213 ) ) ;
#62923=CARTESIAN_POINT ( 'NONE',  ( 110.7114632166112358, 29.09878355652111992, 29.61121420573730134 ) ) ;
#62927=CARTESIAN_POINT ( 'NONE',  ( 201.9869293910475392, 102.6997661182767274, 43.71240911156287012 ) ) ;
#62928=CARTESIAN_POINT ( 'NONE',  ( 113.8568724296587789, 30.58972477291341363, -76.85635754368730943 ) ) ;
#62930=CARTESIAN_POINT ( 'NONE',  ( 141.1220430186942281, 47.19066702031171445, 12.04571220398737452 ) ) ;
#62935=CARTESIAN_POINT ( 'NONE',  ( 70.51583798635768119, 15.57951509147424041, 63.91560277332340689 ) ) ;
#62936=CARTESIAN_POINT ( 'NONE',  ( 129.1909336867078935, 38.67767333518755635, 84.81811994820998279 ) ) ;
#62937=CARTESIAN_POINT ( 'NONE',  ( 152.1381498073140790, 54.87048121475570639, 4.768634089295844980 ) ) ;
#62939=CARTESIAN_POINT ( 'NONE',  ( 159.6614743841974473, 60.66237087206235401, -50.81097292345923222 ) ) ;
#62942=CARTESIAN_POINT ( 'NONE',  ( 112.5537757279407316, 31.07998172410697180, -36.27139529453720712 ) ) ;
#62947=CARTESIAN_POINT ( 'NONE',  ( 136.3292018078239494, 42.93753790426542594, 56.77035877741786862 ) ) ;
#62948=CARTESIAN_POINT ( 'NONE',  ( -165.7143741370936709, 79.24519349471955820, 37.10392210004761893 ) ) ;
#62950=DIRECTION ( 'NONE',  ( -0.000000000000000000, 1.000000000000000000, -0.000000000000000000 ) ) ;
#62955=CARTESIAN_POINT ( 'NONE',  ( 151.3136733342016953, 54.26417151662140981, -12.48898785249184407 ) ) ;
#62957=CARTESIAN_POINT ( 'NONE',  ( -49.88515215727291263, 13.35630923481828169, 86.04290591518972064 ) ) ;
#62958=CARTESIAN_POINT ( 'NONE',  ( 107.2614272668149340, 28.62909081796205513, 43.99715716284213585 ) ) ;
#62959=CARTESIAN_POINT ( 'NONE',  ( -151.2497169612549328, 65.66843968092751993, -61.80823754933450687 ) ) ;
#62961=CARTESIAN_POINT ( 'NONE',  ( 188.4374648754671284, 87.87346242052440459, 8.459214379405038287 ) ) ;
#62962=CARTESIAN_POINT ( 'NONE',  ( 208.9781236209186090, 112.4006213943319636, -37.65073565875546535 ) ) ;
#62964=CARTESIAN_POINT ( 'NONE',  ( 176.0745160362857860, 73.68684431790050837, 15.55076182205331570 ) ) ;
#62965=VERTEX_POINT ( 'NONE', #19076 ) ;
#62966=LINE ( 'NONE', #19710, #45308 ) ;
#62967=EDGE_CURVE ( 'NONE', #18071, #63625, #55670, .T. ) ;
#62969=CARTESIAN_POINT ( 'NONE',  ( -77.71801202538871678, 23.03755222122951452, 72.21756683605353544 ) ) ;
#62974=CARTESIAN_POINT ( 'NONE',  ( -118.4753258120605324, -170.0000000000000000, -95.00000000000133582 ) ) ;
#62975=CARTESIAN_POINT ( 'NONE',  ( -105.8879245385188455, 35.79035667534149212, -9.077219941719809171 ) ) ;
#62978=CARTESIAN_POINT ( 'NONE',  ( 200.5226609475754458, 100.7898801217142051, -91.27370320419781535 ) ) ;
#62980=ORIENTED_EDGE ( 'NONE', *, *, #1755, .F. ) ;
#62981=CARTESIAN_POINT ( 'NONE',  ( -153.5002794404625774, 67.64160439471096709, 31.86792471940524152 ) ) ;
#62982=CARTESIAN_POINT ( 'NONE',  ( 59.29615173875419742, 11.84060224810188622, -49.73800052251814208 ) ) ;
#62983=CARTESIAN_POINT ( 'NONE',  ( 175.8855729601531550, 73.50624012737692681, -22.30791473185340834 ) ) ;
#62989=CARTESIAN_POINT ( 'NONE',  ( -31.43908319763709969, 9.591432048623767415, -50.31719736520186359 ) ) ;
#62991=CARTESIAN_POINT ( 'NONE',  ( 20.74185656603722450, 7.717159106492252896, -48.67200694907381120 ) ) ;
#62992=CARTESIAN_POINT ( 'NONE',  ( -147.7895256390024485, 64.04409735547017135, 45.57579272523850022 ) ) ;
#62994=CARTESIAN_POINT ( 'NONE',  ( 212.0739503583954217, 117.0412199804969759, 35.30913288153361407 ) ) ;
#62995=CARTESIAN_POINT ( 'NONE',  ( 11.46041170590452296, 6.400589304860417883, -90.56819552826038944 ) ) ;
#62999=B_SPLINE_CURVE_WITH_KNOTS ( 'NONE', 3,
 ( #13026, #39745, #34828, #45011, #46054, #24619, #19325, #55928, #7745, #18982, #8436, #2121, #19670, #51349, #24270, #14406, #61201, #35509, #45718, #40776, #29885, #62231, #34488, #14049, #56971, #18287, #28853, #30236, #35857, #56612, #8789, #51687, #29194, #8079, #18635, #3494, #50304, #46395, #67874, #41129, #62597, #61548, #57311, #23573 ),
 .UNSPECIFIED., .F., .F.,
 ( 4, 2, 2, 2, 2, 2, 2, 2, 2, 2, 2, 2, 2, 2, 2, 2, 2, 2, 2, 2, 2, 4 ),
 ( 0.000000000000000000, 0.003360573201437662503, 0.004200716501797043326, 0.005040859802156424582, 0.006721146402875118574, 0.007561289703234486820, 0.008401433003593854199, 0.009241576303953223312, 0.01008171960431258896, 0.01176200620503132545, 0.01260214950539068415, 0.01344229280575004286, 0.01428243610610940330, 0.01512257940646876200, 0.01680286600718750023, 0.01764300930754687455, 0.01848315260790624887, 0.02016343920862501138, 0.02184372580934377736, 0.02352401241006254334, 0.02520429901078130933, 0.02688458561150007531 ),
 .UNSPECIFIED. ) ;
#63002=CARTESIAN_POINT ( 'NONE',  ( -131.5919238272131508, 51.59099727820048997, 86.92280933128381548 ) ) ;
#63003=CARTESIAN_POINT ( 'NONE',  ( 35.65622260226240314, 8.964590916200311455, -63.46208756248341842 ) ) ;
#63004=CARTESIAN_POINT ( 'NONE',  ( -178.5848962563133568, 94.99295350784004199, 16.63922201400802692 ) ) ;
#63005=CARTESIAN_POINT ( 'NONE',  ( 8.402653425627045536, 6.376553021891479212, 92.54943276849337508 ) ) ;
#63007=CARTESIAN_POINT ( 'NONE',  ( 84.73231936899554739, 18.78199960571075877, -77.43798840702864084 ) ) ;
#63010=CARTESIAN_POINT ( 'NONE',  ( -102.2801239173131052, 32.78103895658058065, 72.36362509687883460 ) ) ;
#63011=ORIENTED_EDGE ( 'NONE', *, *, #63696, .F. ) ;
#63012=CARTESIAN_POINT ( 'NONE',  ( -83.51052366780672287, 24.22613130369188639, 16.80462344529878749 ) ) ;
#63014=CARTESIAN_POINT ( 'NONE',  ( -55.54036735998997898, 15.85474597822064702, -8.371773407996174754 ) ) ;
#63017=CARTESIAN_POINT ( 'NONE',  ( 12.46704290855393182, 6.417105965824391411, -49.74798076428597682 ) ) ;
#63018=CARTESIAN_POINT ( 'NONE',  ( -178.5835577246388084, 93.42126246260829703, 60.02133511208158012 ) ) ;
#63019=CARTESIAN_POINT ( 'NONE',  ( 20.74852474914887779, 6.709938988646747760, 16.31688092656622757 ) ) ;
#63022=LINE ( 'NONE', #41913, #64885 ) ;
#63023=CARTESIAN_POINT ( 'NONE',  ( 178.1888264190354789, 77.13727704498029425, -63.63756854808438845 ) ) ;
#63024=LINE ( 'NONE', #14831, #41534 ) ;
#63025=CARTESIAN_POINT ( 'NONE',  ( 102.8111940033034415, 25.59308899183601582, -42.38074508319384393 ) ) ;
#63032=CARTESIAN_POINT ( 'NONE',  ( 39.40195752203892710, 8.409560354027389550, 18.06928371549960133 ) ) ;
#63034=CARTESIAN_POINT ( 'NONE',  ( 173.6007744016332595, 72.73482010729023273, 10.54590781376938580 ) ) ;
#63037=CARTESIAN_POINT ( 'NONE',  ( 137.8342272233871881, 43.87828770902297748, -90.84184450531311938 ) ) ;
#63038=CARTESIAN_POINT ( 'NONE',  ( -157.0077369422018023, 70.81157624963285002, 11.09516931919394978 ) ) ;
#63042=CARTESIAN_POINT ( 'NONE',  ( 207.8407634284390895, 112.5209879629464211, 43.53050796622361673 ) ) ;
#63044=CARTESIAN_POINT ( 'NONE',  ( -82.32006615997346444, 24.83050031643766431, 58.19495574293904383 ) ) ;
#63045=CARTESIAN_POINT ( 'NONE',  ( -109.7647482398635361, 36.74843029291201191, 38.56660667589553526 ) ) ;
#63048=CARTESIAN_POINT ( 'NONE',  ( -47.55539076061677406, 13.83217677045059268, 91.88810249661966623 ) ) ;
#63051=VERTEX_POINT ( 'NONE', #56026 ) ;
#63052=CARTESIAN_POINT ( 'NONE',  ( 21.75198946226450758, 7.772524967554916842, -74.43766794452670865 ) ) ;
#63058=CARTESIAN_POINT ( 'NONE',  ( 140.0820590176526252, 46.51134312115247837, -47.71347409872789314 ) ) ;
#63059=CARTESIAN_POINT ( 'NONE',  ( 207.0312524359575832, 111.3509507522488917, -90.37915150709905276 ) ) ;
#63060=CARTESIAN_POINT ( 'NONE',  ( 12.03162622199373111, 7.415834979634797541, -36.52294849145773270 ) ) ;
#63062=CARTESIAN_POINT ( 'NONE',  ( -122.1940143064357187, 45.29738883755585732, -9.041013927513500192 ) ) ;
#63065=CARTESIAN_POINT ( 'NONE',  ( 173.9599793006471486, 73.07129831195001657, 92.85047428432565653 ) ) ;
#63067=CARTESIAN_POINT ( 'NONE',  ( -25.50312845906833559, 8.692070753302667541, -74.25253205409154589 ) ) ;
#63070=CARTESIAN_POINT ( 'NONE',  ( 13.37366753069833258, 6.435102282077985514, 3.552458417556365156 ) ) ;
#63073=CARTESIAN_POINT ( 'NONE',  ( 208.5884523568772693, 113.6152425727545250, 16.28900457481658393 ) ) ;
#63075=CARTESIAN_POINT ( 'NONE',  ( -175.9970298498767534, 90.38640259140139221, -49.15178234214096875 ) ) ;
#63077=CARTESIAN_POINT ( 'NONE',  ( -24.18270484670773612, 9.527492911955590671, 66.52113223989842083 ) ) ;
#63086=CARTESIAN_POINT ( 'NONE',  ( -106.4728934171454284, 36.10295170132727804, -75.58225694355543567 ) ) ;
#63088=DIRECTION ( 'NONE',  ( -0.000000000000000000, 1.000000000000000000, -0.000000000000000000 ) ) ;
#63089=CARTESIAN_POINT ( 'NONE',  ( -102.2801239173131194, -170.0000000000000000, -69.35912785543959558 ) ) ;
#63092=CARTESIAN_POINT ( 'NONE',  ( 59.29597493004737174, 11.84030339376940688, 16.99923005275914534 ) ) ;
#63093=CARTESIAN_POINT ( 'NONE',  ( -61.75629144857965258, 16.58190704077737720, 68.03453561796777649 ) ) ;
#63098=CARTESIAN_POINT ( 'NONE',  ( 46.48565096083556369, 10.45589966334459575, 88.61677544424188113 ) ) ;
#63099=CARTESIAN_POINT ( 'NONE',  ( -177.1540936177023013, 91.73126115633630207, -75.39503670027723103 ) ) ;
#63101=EDGE_LOOP ( 'NONE', ( #3600, #3826, #5879, #64424 ) ) ;
#63105=CARTESIAN_POINT ( 'NONE',  ( 55.51637278631174155, 12.08345311280959855, -43.73033833359424705 ) ) ;
#63106=CARTESIAN_POINT ( 'NONE',  ( -86.11230725916333029, 26.39026888680170657, 36.88449808153552567 ) ) ;
#63107=CARTESIAN_POINT ( 'NONE',  ( -24.71604178686819253, 9.599501655372943532, -19.30609868970467957 ) ) ;
#63108=CARTESIAN_POINT ( 'NONE',  ( 92.19920907511536257, 21.39700525884453342, 32.16603705074736297 ) ) ;
#63110=EDGE_CURVE ( 'NONE', #18323, #564, #63022, .T. ) ;
#63113=EDGE_CURVE ( 'NONE', #44678, #5653, #8693, .T. ) ;
#63114=CARTESIAN_POINT ( 'NONE',  ( 8.288104306525687193, 6.376394648992965486, 63.87267987369663302 ) ) ;
#63115=B_SPLINE_CURVE_WITH_KNOTS ( 'NONE', 3,
 ( #13691, #62923, #56598, #40766, #14724, #4517, #51675, #20344, #52015, #30225, #15073, #25647, #57299, #30564, #25301, #3829, #24946, #36187, #41120, #46382, #57646, #14037, #35495, #52692, #3152, #67861, #47077, #67183, #41810, #9455, #56957, #30916, #62217, #61864, #8421, #35145, #62579, #19657, #14395, #36533 ),
 .UNSPECIFIED., .F., .F.,
 ( 4, 2, 2, 2, 2, 2, 2, 2, 2, 2, 2, 2, 2, 2, 2, 2, 2, 2, 2, 4 ),
 ( 0.02454308262169000582, 0.02608670964102885112, 0.02685852315069829285, 0.02763033666036773459, 0.02917396367970661458, 0.02994577718937605978, 0.03071759069904549458, 0.03226121771838433294, 0.03303303122805375386, 0.03380484473772318171, 0.03534847175706200967, 0.03689209877640083068, 0.03843572579573965864, 0.03997935281507848659, 0.04152297983441731455, 0.04306660685375614250, 0.04461023387309497046, 0.04615386089243379841, 0.04769748791177262637, 0.04924111493111145432 ),
 .UNSPECIFIED. ) ;
#63116=CARTESIAN_POINT ( 'NONE',  ( -27.49195330402089255, 9.993776132065303131, 31.33447323685886587 ) ) ;
#63117=CARTESIAN_POINT ( 'NONE',  ( 203.1423857108907782, 105.9238244286949850, 29.36013609250961309 ) ) ;
#63118=CARTESIAN_POINT ( 'NONE',  ( -72.54813618488350357, 21.15114325868153244, 87.25760088006373394 ) ) ;
#63121=DIRECTION ( 'NONE',  ( 0.000000000000000000, 0.000000000000000000, 1.000000000000000000 ) ) ;
#63124=CARTESIAN_POINT ( 'NONE',  ( 117.6924004117966689, 33.61107268965020722, -71.28084340972505117 ) ) ;
#63125=DIRECTION ( 'NONE',  ( -0.8118923937861950435, -0.5838071093367415143, 0.000000000000000000 ) ) ;
#63126=CARTESIAN_POINT ( 'NONE',  ( 197.5334904971816172, 97.00846725096926093, -68.42925186292004014 ) ) ;
#63128=CARTESIAN_POINT ( 'NONE',  ( -38.93847286785603501, 11.96870349976817494, 64.05428266636177170 ) ) ;
#63130=CARTESIAN_POINT ( 'NONE',  ( -38.78626392836186909, -170.0000000000000000, -95.00000000000133582 ) ) ;
#63131=CARTESIAN_POINT ( 'NONE',  ( -85.35172689181706573, 26.07142112926218047, -19.20697335453129284 ) ) ;
#63134=ORIENTED_EDGE ( 'NONE', *, *, #34722, .F. ) ;
#63135=VERTEX_POINT ( 'NONE', #32400 ) ;
#63137=CARTESIAN_POINT ( 'NONE',  ( -108.1180879163843116, 36.99199941971030370, 15.90925667645064578 ) ) ;
#63139=CARTESIAN_POINT ( 'NONE',  ( -85.96384504792885650, 26.32782846176032621, -40.86557644392104294 ) ) ;
#63140=CARTESIAN_POINT ( 'NONE',  ( 164.6499013411308283, 63.45576988183551492, 65.93988476214543937 ) ) ;
#63146=CARTESIAN_POINT ( 'NONE',  ( 159.2389084450350367, 59.03884018680375334, -63.16658458358803330 ) ) ;
#63148=ORIENTED_EDGE ( 'NONE', *, *, #2462, .T. ) ;
#63151=STYLED_ITEM ( 'NONE', ( #29183 ), #18150 ) ;
#63153=CARTESIAN_POINT ( 'NONE',  ( 38.43102714813442589, 9.298961820315049920, -50.57286685989200947 ) ) ;
#63159=CARTESIAN_POINT ( 'NONE',  ( -31.92572261726340344, 10.69135962481465540, -77.16174795566556099 ) ) ;
#63164=CARTESIAN_POINT ( 'NONE',  ( 36.31593203568480988, 8.028139509847024513, 57.41831045774998188 ) ) ;
#63165=CARTESIAN_POINT ( 'NONE',  ( 8.670103207226935282, 6.377073801252348240, -18.58750088859477856 ) ) ;
#63166=CARTESIAN_POINT ( 'NONE',  ( 22.15926701483429895, 7.796117250416237709, 14.63516493621701642 ) ) ;
#63168=CARTESIAN_POINT ( 'NONE',  ( -122.3963566076408114, 44.23346594671846788, 4.624121492655477894 ) ) ;
#63169=CARTESIAN_POINT ( 'NONE',  ( 39.40195752203892710, 8.409560354027385998, -8.775266874964067654 ) ) ;
#63170=CARTESIAN_POINT ( 'NONE',  ( 126.3580543567275072, 37.07735301062816546, -16.37485516677961073 ) ) ;
#63171=CARTESIAN_POINT ( 'NONE',  ( 18.43272992546528855, 7.606837839440253823, -9.151768092893727058 ) ) ;
#63172=CARTESIAN_POINT ( 'NONE',  ( 11.81843724556921060, 7.412394300769732602, 17.03812180473721938 ) ) ;
#63173=VERTEX_POINT ( 'NONE', #21157 ) ;
#63174=DIRECTION ( 'NONE',  ( 0.000000000000000000, 0.000000000000000000, 1.000000000000000000 ) ) ;
#63176=DIRECTION ( 'NONE',  ( -0.000000000000000000, 1.000000000000000000, -0.000000000000000000 ) ) ;
#63177=LINE ( 'NONE', #68451, #59005 ) ;
#63178=CARTESIAN_POINT ( 'NONE',  ( -109.6752351740181695, 37.84903014964773860, -41.23783467770100941 ) ) ;
#63179=CARTESIAN_POINT ( 'NONE',  ( 188.2962140587030149, 87.71627202537843004, -45.80397896477450814 ) ) ;
#63182=B_SPLINE_CURVE_WITH_KNOTS ( 'NONE', 3,
 ( #28521, #55595, #29558, #49965, #1801, #23942, #29219, #66870, #67223, #51022, #23256, #2832, #18313, #13728, #2146, #65823, #7769, #39419, #8107, #13391, #12693, #61904, #35187, #34513, #18669, #44336, #40460, #34159, #17974, #49607, #45039, #24300, #7426, #28878, #50329, #17617, #56640, #66182, #23601, #22893, #56289, #66521, #39769, #12343, #19008, #60868, #61228, #13055 ),
 .UNSPECIFIED., .F., .F.,
 ( 4, 2, 2, 2, 2, 2, 2, 2, 2, 2, 2, 2, 2, 2, 2, 2, 2, 2, 2, 2, 2, 2, 2, 4 ),
 ( 0.02698595842317763269, 0.02784423243973405820, 0.02870250645629048025, 0.03041905448940323414, 0.03127732850595960762, 0.03213560252251598803, 0.03385215055562873498, 0.03471042457218508070, 0.03556869858874141949, 0.03728524662185411093, 0.03814352063841044971, 0.03900179465496678849, 0.03986006867152312727, 0.04071834268807946605, 0.04157661670463580483, 0.04243489072119214361, 0.04415143875430481424, 0.04500971277086115996, 0.04586798678741749180, 0.04758453482053018324, 0.04930108285364286774, 0.05101763088675554531, 0.05273417891986822981, 0.05445072695298091431 ),
 .UNSPECIFIED. ) ;
#63183=CARTESIAN_POINT ( 'NONE',  ( -142.0685766576042397, 58.11789490499572963, -14.35908353972402551 ) ) ;
#63184=CARTESIAN_POINT ( 'NONE',  ( 199.3764470687682433, 100.9548044849099142, 15.15399381071274831 ) ) ;
#63186=CARTESIAN_POINT ( 'NONE',  ( 113.8568724296587789, 30.58972477291343850, 57.36639540863109232 ) ) ;
#63188=CARTESIAN_POINT ( 'NONE',  ( -61.77164219855450966, 17.63686644795249592, 14.34267326658022235 ) ) ;
#63189=CARTESIAN_POINT ( 'NONE',  ( 126.9201538765324386, 37.39093565120715112, 39.87409765458102129 ) ) ;
#63190=CARTESIAN_POINT ( 'NONE',  ( -78.66644367742109978, 22.32174330031318732, -50.11545063171791270 ) ) ;
#63192=CARTESIAN_POINT ( 'NONE',  ( -95.88718821240196633, 29.65015105908826953, 34.08905749573029453 ) ) ;
#63195=DIRECTION ( 'NONE',  ( -0.000000000000000000, 1.000000000000000000, -0.000000000000000000 ) ) ;
#63196=ORIENTED_EDGE ( 'NONE', *, *, #50688, .T. ) ;
#63198=EDGE_LOOP ( 'NONE', ( #18741, #15984, #59076, #40007 ) ) ;
#63201=CARTESIAN_POINT ( 'NONE',  ( -167.4844853368928739, 82.52074065752738363, 6.523106101700750337 ) ) ;
#63202=EDGE_CURVE ( 'NONE', #14330, #9201, #54169, .T. ) ;
#63203=CARTESIAN_POINT ( 'NONE',  ( 133.8566784816069344, -170.0000000000000000, -97.21241211332302612 ) ) ;
#63204=CARTESIAN_POINT ( 'NONE',  ( -175.9970298498766965, 90.38640259140137800, -22.30723175167727490 ) ) ;
#63205=CARTESIAN_POINT ( 'NONE',  ( -131.3096895243910751, 51.39228038925231346, 70.17557077602670290 ) ) ;
#63207=CARTESIAN_POINT ( 'NONE',  ( -109.5800870510459646, 37.79624625667730697, 93.46020534934932300 ) ) ;
#63210=ORIENTED_EDGE ( 'NONE', *, *, #69545, .F. ) ;
#63211=CARTESIAN_POINT ( 'NONE',  ( -60.97011009284708649, 16.34812508431679490, -11.23730993338677031 ) ) ;
#63214=CARTESIAN_POINT ( 'NONE',  ( 56.00903540737504471, 11.15594382527104500, -94.20234774883739703 ) ) ;
#63216=CARTESIAN_POINT ( 'NONE',  ( 69.83617901654359628, 15.39919709983075613, -73.19441325359579764 ) ) ;
#63224=CARTESIAN_POINT ( 'NONE',  ( -71.22896441287284119, 20.69091426169410042, 36.91910425864390533 ) ) ;
#63228=CARTESIAN_POINT ( 'NONE',  ( -166.2028193222418793, 79.74385139484276408, -71.96685162649892220 ) ) ;
#63229=EDGE_LOOP ( 'NONE', ( #65148, #3579, #22027, #58635 ) ) ;
#63230=CARTESIAN_POINT ( 'NONE',  ( -109.0297561673456102, 36.34391931706016976, -12.38998052533776040 ) ) ;
#63232=CARTESIAN_POINT ( 'NONE',  ( -37.79823708645146496, 10.72197716414928692, 6.888035153445309255 ) ) ;
#63235=FACE_OUTER_BOUND ( 'NONE', #13130, .T. ) ;
#63236=CARTESIAN_POINT ( 'NONE',  ( 110.2429982417149574, -170.0000000000000000, 90.80031538666469260 ) ) ;
#63239=CARTESIAN_POINT ( 'NONE',  ( -13.45956523846224506, 8.333781915634244086, -47.87459002919935358 ) ) ;
#63245=CARTESIAN_POINT ( 'NONE',  ( -121.5684475810873266, 44.90063534192884731, -89.97182396522346437 ) ) ;
#63247=CARTESIAN_POINT ( 'NONE',  ( 58.09877917144279280, 12.61383386832655340, 58.47304198809774078 ) ) ;
#63249=CARTESIAN_POINT ( 'NONE',  ( -25.81763596640060499, 8.735969132042864516, 5.900969464607853432 ) ) ;
#63251=CARTESIAN_POINT ( 'NONE',  ( 39.40195752203892710, -170.0000000000000000, 3.069283715499574239 ) ) ;
#63252=CARTESIAN_POINT ( 'NONE',  ( -14.94265033805046095, 7.459411036484912216, -72.17853611393870494 ) ) ;
#63253=CARTESIAN_POINT ( 'NONE',  ( -102.2801239173131194, 32.78103895658057354, -8.170026674512225640 ) ) ;
#63255=CARTESIAN_POINT ( 'NONE',  ( 154.6530827109542940, 56.75509330623209792, -36.66977919429117350 ) ) ;
#63257=ORIENTED_EDGE ( 'NONE', *, *, #60582, .F. ) ;
#63260=CARTESIAN_POINT ( 'NONE',  ( -153.6946616617038615, 69.16142959008686830, 58.82626357113776550 ) ) ;
#63261=CARTESIAN_POINT ( 'NONE',  ( 177.0110682437507705, 75.98481089748382544, -23.19430282288263356 ) ) ;
#63262=CARTESIAN_POINT ( 'NONE',  ( -109.7079446832838698, 37.86719386855315150, 63.79328878868093256 ) ) ;
#63264=ORIENTED_EDGE ( 'NONE', *, *, #35186, .T. ) ;
#63266=CARTESIAN_POINT ( 'NONE',  ( 87.11228333101210808, 19.58587579906928156, 71.55663816294303103 ) ) ;
#63267=CARTESIAN_POINT ( 'NONE',  ( 201.9822477997853980, 104.3642793804900037, -23.98431144848092345 ) ) ;
#63268=CARTESIAN_POINT ( 'NONE',  ( 133.8566784816069628, 41.42467568809806977, 44.51034083899536142 ) ) ;
#63271=DIRECTION ( 'NONE',  ( 0.000000000000000000, 0.000000000000000000, 1.000000000000000000 ) ) ;
#63272=CARTESIAN_POINT ( 'NONE',  ( 113.4493678088378346, 30.39339414805072437, -63.47052499151446625 ) ) ;
#63274=CARTESIAN_POINT ( 'NONE',  ( 163.2911130186310800, 63.63047778106597718, 14.80112738755994428 ) ) ;
#63280=VERTEX_POINT ( 'NONE', #17606 ) ;
#63281=CARTESIAN_POINT ( 'NONE',  ( -103.2169245450825343, 33.25885825286820108, -49.97046926489813501 ) ) ;
#63282=EDGE_CURVE ( 'NONE', #56227, #52276, #29207, .T. ) ;
#63283=CARTESIAN_POINT ( 'NONE',  ( 126.3770099964006732, 37.08789675649202167, 91.36094124151978235 ) ) ;
#63284=CARTESIAN_POINT ( 'NONE',  ( -62.54085973597666026, 16.81797209566547124, 37.32607792003522462 ) ) ;
#63286=CARTESIAN_POINT ( 'NONE',  ( 150.5744176759382640, 53.72473166688032364, 7.104188182867663848 ) ) ;
#63288=CARTESIAN_POINT ( 'NONE',  ( -180.6009936245623066, 95.85948119829087943, 38.95306750779999305 ) ) ;
#63290=CARTESIAN_POINT ( 'NONE',  ( 112.1100957124161397, 30.86846953551571104, -50.70151326046267570 ) ) ;
#63292=VERTEX_POINT ( 'NONE', #61215 ) ;
#63298=CARTESIAN_POINT ( 'NONE',  ( 141.2894128405440028, 46.09731134920848916, 64.89240564234853537 ) ) ;
#63299=CARTESIAN_POINT ( 'NONE',  ( -169.1005390226459326, 82.76152663947085841, 44.66854843987135837 ) ) ;
#63300=CIRCLE ( 'NONE', #58811, 243.4957430088094839 ) ;
#63302=EDGE_CURVE ( 'NONE', #29554, #57393, #69078, .T. ) ;
#63303=CARTESIAN_POINT ( 'NONE',  ( 89.20981392318257974, 21.38519354635263170, 44.25831453610486221 ) ) ;
#63306=ADVANCED_FACE ( 'NONE', ( #48045 ), #8800, .T. ) ;
#63309=CARTESIAN_POINT ( 'NONE',  ( -54.44503425861569923, 14.51857899460407708, 84.00475665173640039 ) ) ;
#63310=CARTESIAN_POINT ( 'NONE',  ( 108.3753929817421664, 29.13179266688724312, 44.39034800661560354 ) ) ;
#63312=CARTESIAN_POINT ( 'NONE',  ( 55.66333002014489750, 11.08673571569896943, 92.52088922431616425 ) ) ;
#63313=CARTESIAN_POINT ( 'NONE',  ( 188.4365915667138438, 87.87248959723055464, 11.47310305952803056 ) ) ;
#63314=CARTESIAN_POINT ( 'NONE',  ( 210.9506883977751954, 115.3310071214937267, -47.97542656608541733 ) ) ;
#63318=DIRECTION ( 'NONE',  ( 0.000000000000000000, 0.000000000000000000, 1.000000000000000000 ) ) ;
#63324=LINE ( 'NONE', #58040, #42330 ) ;
#63325=CARTESIAN_POINT ( 'NONE',  ( -105.4642082819536313, 35.56541171990216554, -8.863305472588931977 ) ) ;
#63330=EDGE_CURVE ( 'NONE', #45231, #20757, #43114, .T. ) ;
#63333=CARTESIAN_POINT ( 'NONE',  ( 56.30011474572734187, 11.21470186335419505, -46.56933648099417411 ) ) ;
#63334=CARTESIAN_POINT ( 'NONE',  ( 174.1251613516844543, 71.84747073139210727, -14.02940449773612208 ) ) ;
#63338=CARTESIAN_POINT ( 'NONE',  ( -133.3799602664182089, 52.86209125874979975, 38.65010449165978201 ) ) ;
#63340=CARTESIAN_POINT ( 'NONE',  ( 19.54326199789021956, 7.657220834818549093, -49.51591199172310809 ) ) ;
#63341=CARTESIAN_POINT ( 'NONE',  ( -142.0084862216822330, 59.34995487985344909, 38.79924527383067101 ) ) ;
#63350=CARTESIAN_POINT ( 'NONE',  ( -118.8238520964533507, 43.19104454097361412, 94.39884469698169767 ) ) ;
#63352=FACE_OUTER_BOUND ( 'NONE', #38256, .T. ) ;
#63353=CARTESIAN_POINT ( 'NONE',  ( -62.41990535723909517, -170.0000000000000000, -95.00000000000133582 ) ) ;
#63354=CARTESIAN_POINT ( 'NONE',  ( 67.93926590385568431, 13.86859831467922710, 42.99160110879589780 ) ) ;
#63355=CARTESIAN_POINT ( 'NONE',  ( 8.976513922597330719, 7.384348797512408247, 88.04828221664904220 ) ) ;
#63363=CARTESIAN_POINT ( 'NONE',  ( -82.32750425780476178, 23.74963782027935721, 17.63696427471160888 ) ) ;
#63371=CARTESIAN_POINT ( 'NONE',  ( -180.2244609727085276, 95.39945930389644957, 62.74216164717486066 ) ) ;
#63372=CARTESIAN_POINT ( 'NONE',  ( 130.7531879853686405, 39.58149302537893988, 70.69835057338305262 ) ) ;
#63373=ORIENTED_EDGE ( 'NONE', *, *, #5396, .T. ) ;
#63374=CARTESIAN_POINT ( 'NONE',  ( -38.02163356681019479, 10.76490728754187032, 94.99999999999866418 ) ) ;
#63376=AXIS2_PLACEMENT_3D ( 'NONE', #8714, #62156, #29459 ) ;
#63378=EDGE_CURVE ( 'NONE', #27549, #33732, #68239, .T. ) ;
#63379=CARTESIAN_POINT ( 'NONE',  ( 103.8093541423579325, 26.01745837747062851, -47.30919203401695228 ) ) ;
#63380=CARTESIAN_POINT ( 'NONE',  ( -25.80058235236790054, 8.733375263008323230, 42.68610631600346039 ) ) ;
#63381=CARTESIAN_POINT ( 'NONE',  ( -144.9412191745148277, 61.69548892475970803, -63.18798172190984275 ) ) ;
#63386=AXIS2_PLACEMENT_3D ( 'NONE', #49207, #67085, #16519 ) ;
#63387=CARTESIAN_POINT ( 'NONE',  ( -84.23336401058612921, 25.60798568215576054, -64.41046605635534661 ) ) ;
#63388=CARTESIAN_POINT ( 'NONE',  ( -6.140867422161948141, 6.785844475553973965, -89.24911309443601226 ) ) ;
#63391=CARTESIAN_POINT ( 'NONE',  ( 126.8015497489690375, 37.32461426945043570, 7.607582870371705219 ) ) ;
#63393=CARTESIAN_POINT ( 'NONE',  ( -153.1121305730337099, 67.29834700374524914, 17.95717372012110502 ) ) ;
#63395=AXIS2_PLACEMENT_3D ( 'NONE', #17404, #27611, #38881 ) ;
#63396=CARTESIAN_POINT ( 'NONE',  ( 211.1046732743772338, 117.3965485104337176, 40.61640241343361168 ) ) ;
#63397=CARTESIAN_POINT ( 'NONE',  ( -81.90760111942955746, 24.66532273091451088, 71.54302205457766206 ) ) ;
#63398=CARTESIAN_POINT ( 'NONE',  ( -103.2169245450825343, 33.25885825286820108, 30.56318250649291457 ) ) ;
#63406=DIRECTION ( 'NONE',  ( -0.000000000000000000, 1.000000000000000000, -0.000000000000000000 ) ) ;
#63408=CARTESIAN_POINT ( 'NONE',  ( -169.8885678771098640, 85.07765565657317097, 31.53960263309836520 ) ) ;
#63409=FACE_OUTER_BOUND ( 'NONE', #12341, .T. ) ;
#63410=CARTESIAN_POINT ( 'NONE',  ( 136.7690435008551049, 44.39743995805024213, -50.43862942802062577 ) ) ;
#63411=CARTESIAN_POINT ( 'NONE',  ( 32.29989959354727347, 7.591763852038295290, -40.69674924162746521 ) ) ;
#63412=CARTESIAN_POINT ( 'NONE',  ( 149.9552318559266837, 52.03645904563050095, -43.60103139574965780 ) ) ;
#63414=CARTESIAN_POINT ( 'NONE',  ( -123.0348077379026819, 45.83489305753317211, -8.631653705166407065 ) ) ;
#63416=ADVANCED_BREP_SHAPE_REPRESENTATION ( '', ( #18150, #66832 ), #5131 ) ;
#63417=EDGE_LOOP ( 'NONE', ( #49129, #69391 ) ) ;
#63418=CARTESIAN_POINT ( 'NONE',  ( 182.3755817553430063, 81.36527810436713537, 83.10424013160293555 ) ) ;
#63419=CARTESIAN_POINT ( 'NONE',  ( -165.6754884515988522, 80.64428675972324356, -95.00000000000133582 ) ) ;
#63422=CARTESIAN_POINT ( 'NONE',  ( 64.63121951458684578, 14.08762381031449351, -89.57469566860601162 ) ) ;
#63423=CARTESIAN_POINT ( 'NONE',  ( 90.30732934992393268, 21.77797012484618122, 16.92149306509885776 ) ) ;
#63425=CARTESIAN_POINT ( 'NONE',  ( 173.6012773665504199, 71.36035397668607061, -71.15789844731480684 ) ) ;
#63427=CARTESIAN_POINT ( 'NONE',  ( 93.86680996363766383, 22.01878169039503774, -14.49409919722980256 ) ) ;
#63428=CARTESIAN_POINT ( 'NONE',  ( -27.70115495247213033, 10.02455692117576191, 71.08150156007859266 ) ) ;
#63429=DIRECTION ( 'NONE',  ( 0.000000000000000000, 0.000000000000000000, 1.000000000000000000 ) ) ;
#63435=CARTESIAN_POINT ( 'NONE',  ( 154.6530827109543509, 56.75509330623210502, 70.70842316756356638 ) ) ;
#63436=CARTESIAN_POINT ( 'NONE',  ( -104.5916564445180512, 35.10571011602409186, -62.20883666294024295 ) ) ;
#63437=DIRECTION ( 'NONE',  ( 0.000000000000000000, 0.000000000000000000, 1.000000000000000000 ) ) ;
#63438=CARTESIAN_POINT ( 'NONE',  ( -0.3276879771421796761, 7.525453440574858988, 90.93095886057497523 ) ) ;
#63440=ORIENTED_EDGE ( 'NONE', *, *, #56195, .T. ) ;
#63444=ADVANCED_FACE ( 'NONE', ( #5825 ), #49428, .F. ) ;
#63448=CARTESIAN_POINT ( 'NONE',  ( 46.42183744180581328, 10.44561024203780875, 93.82526922102383082 ) ) ;
#63449=CARTESIAN_POINT ( 'NONE',  ( -179.6470915626257465, 94.69856161161352759, -72.76301568367956918 ) ) ;
#63450=CARTESIAN_POINT ( 'NONE',  ( 140.8933556880726030, 47.04060091794853804, -94.58027771532738370 ) ) ;
#63451=ORIENTED_EDGE ( 'NONE', *, *, #7147, .F. ) ;
#63452=DIRECTION ( 'NONE',  ( 0.000000000000000000, 0.000000000000000000, 1.000000000000000000 ) ) ;
#63455=CARTESIAN_POINT ( 'NONE',  ( -0.9897066053608921665, 7.549089325901768177, 7.675277931132895581 ) ) ;
#63456=CARTESIAN_POINT ( 'NONE',  ( 174.9099402067543565, 73.96774984027639732, -39.45882913571559669 ) ) ;
#63457=CARTESIAN_POINT ( 'NONE',  ( -153.6946616617039183, 69.16142959008689672, -75.39648938118064336 ) ) ;
#63459=EDGE_LOOP ( 'NONE', ( #10028, #13785, #6394, #21471 ) ) ;
#63461=CARTESIAN_POINT ( 'NONE',  ( 8.336031647119270360, 6.376437040857335425, 65.33787955784195844 ) ) ;
#63463=ADVANCED_FACE ( 'NONE', ( #43457 ), #55411, .F. ) ;
#63464=CARTESIAN_POINT ( 'NONE',  ( 202.7506655727289342, 105.3943386412348815, 43.96215325962744913 ) ) ;
#63465=CARTESIAN_POINT ( 'NONE',  ( 79.20784687562183990, 17.02089708476972874, 89.76511234889541413 ) ) ;
#63467=ORIENTED_EDGE ( 'NONE', *, *, #728, .T. ) ;
#63470=CARTESIAN_POINT ( 'NONE',  ( 117.4711568421289911, 33.49899443629669804, -68.20117326592374241 ) ) ;
#63471=DIRECTION ( 'NONE',  ( -0.8160245890732938934, -0.5780171883497599028, 0.000000000000000000 ) ) ;
#63472=CARTESIAN_POINT ( 'NONE',  ( 199.3743599161303450, 99.31857334527873604, -65.36260388931131615 ) ) ;
#63474=CARTESIAN_POINT ( 'NONE',  ( -118.4553071845214873, 41.78724769484929880, 63.86654146996676218 ) ) ;
#63475=CARTESIAN_POINT ( 'NONE',  ( 151.6351261592329251, 53.25263237790402115, -65.75027802898746643 ) ) ;
#63476=CARTESIAN_POINT ( 'NONE',  ( 22.54170116539453161, 7.818774103032803069, -93.41931582978958204 ) ) ;
#63477=VECTOR ( 'NONE', #25079, 1000.000000000000000 ) ;
#63481=CARTESIAN_POINT ( 'NONE',  ( 68.94309019697858787, 15.16533147648755175, -11.75461547644634841 ) ) ;
#63482=VECTOR ( 'NONE', #46139, 1000.000000000000000 ) ;
#63483=CARTESIAN_POINT ( 'NONE',  ( -85.90077524418995836, 26.30132018890135726, -40.62086469904666330 ) ) ;
#63484=CARTESIAN_POINT ( 'NONE',  ( 117.3330559693645938, 32.30248182301458115, 88.32983765503517759 ) ) ;
#63485=CARTESIAN_POINT ( 'NONE',  ( 114.6659427952414632, 32.10199811723105512, -10.50219939888065745 ) ) ;
#63490=CARTESIAN_POINT ( 'NONE',  ( -149.8802420082118374, 65.81997532648824745, 84.41443440944620136 ) ) ;
#63494=ORIENTED_EDGE ( 'NONE', *, *, #15624, .F. ) ;
#63496=CARTESIAN_POINT ( 'NONE',  ( 32.37980458033285203, 8.611076697115699119, -40.47400308918246736 ) ) ;
#63499=CARTESIAN_POINT ( 'NONE',  ( 199.3764173596862292, 100.9540560740992419, 58.24261284197358890 ) ) ;
#63501=CARTESIAN_POINT ( 'NONE',  ( 46.91100451385224801, 9.505349959559994844, 90.54425985225793738 ) ) ;
#63507=CARTESIAN_POINT ( 'NONE',  ( 126.5710838895482198, 37.19597237024179037, -18.47868295772153502 ) ) ;
#63510=EDGE_CURVE ( 'NONE', #15369, #66651, #19508, .T. ) ;
#63514=FACE_OUTER_BOUND ( 'NONE', #23161, .T. ) ;
#63516=CARTESIAN_POINT ( 'NONE',  ( -108.9145525555662459, 37.42858360505776005, -46.02153963151565108 ) ) ;
#63517=CARTESIAN_POINT ( 'NONE',  ( 183.1873354889583254, 82.20882912211250471, -50.93700232963676200 ) ) ;
#63518=ORIENTED_EDGE ( 'NONE', *, *, #12907, .F. ) ;
#63519=ORIENTED_EDGE ( 'NONE', *, *, #17946, .T. ) ;
#63520=ADVANCED_FACE ( 'NONE', ( #23765 ), #67040, .F. ) ;
#63522=CARTESIAN_POINT ( 'NONE',  ( 173.6502905022586560, 71.40583870588187665, 91.51296465151303039 ) ) ;
#63524=EDGE_LOOP ( 'NONE', ( #51596, #19038, #20514, #23764 ) ) ;
#63526=CARTESIAN_POINT ( 'NONE',  ( 117.0065308422768595, 32.13872219870570035, 60.70489602400656537 ) ) ;
#63529=CARTESIAN_POINT ( 'NONE',  ( 129.4987365823221808, 38.85470922756777412, 30.90157705602048921 ) ) ;
#63530=AXIS2_PLACEMENT_3D ( 'NONE', #47896, #53515, #31392 ) ;
#63533=CARTESIAN_POINT ( 'NONE',  ( -95.19652294162978023, 29.32558722310179178, 40.53639674485660294 ) ) ;
#63535=AXIS2_PLACEMENT_3D ( 'NONE', #12836, #13182, #67005 ) ;
#63536=CARTESIAN_POINT ( 'NONE',  ( 91.49345572560145001, 21.13836538408682131, -49.03551200642353081 ) ) ;
#63541=VECTOR ( 'NONE', #52214, 1000.000000000000000 ) ;
#63550=CARTESIAN_POINT ( 'NONE',  ( 61.09977118998600076, 13.26754120022606109, 3.213164665537364684 ) ) ;
#63556=CARTESIAN_POINT ( 'NONE',  ( -132.5976199670998597, 52.30296609017644016, -72.63115324000138173 ) ) ;
#63558=CARTESIAN_POINT ( 'NONE',  ( -94.78109144324893975, 29.13179392050638583, 10.88929637896141855 ) ) ;
#63559=CARTESIAN_POINT ( 'NONE',  ( -94.84390436305042726, 29.16104988397311715, -68.34880207487753978 ) ) ;
#63561=ORIENTED_EDGE ( 'NONE', *, *, #54208, .F. ) ;
#63562=CARTESIAN_POINT ( 'NONE',  ( 187.2354698746857480, 85.05376776489251256, -74.88949992417202850 ) ) ;
#63563=CARTESIAN_POINT ( 'NONE',  ( -165.6212796729685692, 79.15047440262054579, -42.51887467077794014 ) ) ;
#63565=CARTESIAN_POINT ( 'NONE',  ( 107.9213359589208494, 28.92595015506873324, -63.11969581620832770 ) ) ;
#63566=CARTESIAN_POINT ( 'NONE',  ( -73.09214866197369531, 21.34321757515763451, 32.87608688857182671 ) ) ;
#63567=CARTESIAN_POINT ( 'NONE',  ( 80.17205177205137545, 17.31791394718354482, 33.38893405093305944 ) ) ;
#63568=CARTESIAN_POINT ( 'NONE',  ( 64.93224207568367490, 14.16036304753835040, -35.96564466294290696 ) ) ;
#63571=EDGE_LOOP ( 'NONE', ( #16801, #39351, #51790, #32222 ) ) ;
#63572=CARTESIAN_POINT ( 'NONE',  ( -104.5827168854524700, 33.96561401163045701, -22.82331764786334816 ) ) ;
#63575=CARTESIAN_POINT ( 'NONE',  ( -38.69408084385329971, 10.89529537250243152, 12.83750613738102153 ) ) ;
#63576=CARTESIAN_POINT ( 'NONE',  ( 82.94816950786170651, 19.25538918181906922, 70.59558542695980066 ) ) ;
#63577=CARTESIAN_POINT ( 'NONE',  ( -78.66644367742111399, 22.32174330031318732, -88.80455181264524356 ) ) ;
#63578=CARTESIAN_POINT ( 'NONE',  ( 151.1873096904021452, 52.92629247302094342, -12.67588465243391127 ) ) ;
#63580=AXIS2_PLACEMENT_3D ( 'NONE', #41090, #57272, #31236 ) ;
#63582=CARTESIAN_POINT ( 'NONE',  ( 37.47081272996199885, 8.166145978397521432, -62.71310258412169958 ) ) ;
#63583=CARTESIAN_POINT ( 'NONE',  ( -95.05323930133205579, 30.36974142673410526, -67.28845679951155034 ) ) ;
#63584=CARTESIAN_POINT ( 'NONE',  ( -36.89224332184166855, 11.57404295377975956, -21.12750825744156913 ) ) ;
#63587=ORIENTED_EDGE ( 'NONE', *, *, #54919, .F. ) ;
#63594=CARTESIAN_POINT ( 'NONE',  ( -24.33435124463266419, 8.532637995283112176, 13.28721146798333841 ) ) ;
#63596=CIRCLE ( 'NONE', #59048, 242.4895526022646379 ) ;
#63597=CARTESIAN_POINT ( 'NONE',  ( -7.825402957745083654, 6.891034867348166948, -77.26262132240753999 ) ) ;
#63599=CARTESIAN_POINT ( 'NONE',  ( 155.7265855639938650, 57.57443315515123317, -50.93204425173435368 ) ) ;
#63601=AXIS2_PLACEMENT_3D ( 'NONE', #21764, #68914, #16494 ) ;
#63604=CARTESIAN_POINT ( 'NONE',  ( -152.9143627383494959, 68.46626892668655273, 71.76242021779931690 ) ) ;
#63606=CARTESIAN_POINT ( 'NONE',  ( -102.7494334820057276, 34.14986869751101040, 72.36362509687886302 ) ) ;
#63610=CARTESIAN_POINT ( 'NONE',  ( -2.874437057892792247, 6.618922960888032669, -21.72834514570417497 ) ) ;
#63613=CARTESIAN_POINT ( 'NONE',  ( -142.9185165087913845, 58.78605825417614739, 88.31239537911277182 ) ) ;
#63614=EDGE_CURVE ( 'NONE', #29355, #5954, #13659, .T. ) ;
#63620=CARTESIAN_POINT ( 'NONE',  ( 188.0103583326377930, 87.39896620268125105, 39.69940583340289919 ) ) ;
#63622=CARTESIAN_POINT ( 'NONE',  ( 157.0357419681844533, 58.58786672900118475, 29.41886851933077196 ) ) ;
#63625=VERTEX_POINT ( 'NONE', #26526 ) ;
#63626=CARTESIAN_POINT ( 'NONE',  ( 173.6737675136086523, 72.80308721038092301, 62.45876396626458416 ) ) ;
#63627=ORIENTED_EDGE ( 'NONE', *, *, #8704, .T. ) ;
#63628=AXIS2_PLACEMENT_3D ( 'NONE', #69365, #15899, #10612 ) ;
#63629=CARTESIAN_POINT ( 'NONE',  ( -71.59086462055191191, 19.75139532313339075, -18.27088716436448479 ) ) ;
#63633=CARTESIAN_POINT ( 'NONE',  ( 150.0278556977734752, 53.32860603304212788, 11.14328715965509176 ) ) ;
#63635=CARTESIAN_POINT ( 'NONE',  ( -177.1539090641757923, 91.73101548694627638, 44.66073844826994588 ) ) ;
#63639=CARTESIAN_POINT ( 'NONE',  ( 116.5100763992442836, 33.01539745157280237, -39.29511836571368377 ) ) ;
#63647=CARTESIAN_POINT ( 'NONE',  ( 135.6651581599209919, 42.52720121194705172, 56.57256158429925819 ) ) ;
#63648=CARTESIAN_POINT ( 'NONE',  ( 204.6977192012829789, -170.0000000000000000, -43.82593103262159673 ) ) ;
#63651=ORIENTED_EDGE ( 'NONE', *, *, #65922, .T. ) ;
#63652=CARTESIAN_POINT ( 'NONE',  ( 46.51679720856117228, 10.46086439153923742, 8.146061147039359795 ) ) ;
#63653=EDGE_LOOP ( 'NONE', ( #60443, #32539, #18392, #41987 ) ) ;
#63654=CARTESIAN_POINT ( 'NONE',  ( 150.4722669492348643, 53.65054032737658929, -19.49086022515975358 ) ) ;
#63655=CARTESIAN_POINT ( 'NONE',  ( -61.68940124183720286, 16.56194981783060172, 94.99999999999866418 ) ) ;
#63657=CARTESIAN_POINT ( 'NONE',  ( -151.6716822472524484, 66.03661194063732864, -76.35210402040455335 ) ) ;
#63658=CARTESIAN_POINT ( 'NONE',  ( -109.5542371224815810, 36.63223321375210162, 89.85165753065791705 ) ) ;
#63659=B_SPLINE_CURVE_WITH_KNOTS ( 'NONE', 3,
 ( #15587, #21206, #36700, #15921, #58821, #27159, #53540, #26825, #48252, #32450, #27506, #64807, #16607, #32793, #54224, #6047, #50709, #39129, #33148, #44745, #6754, #60567, #13090, #49302, #29260, #2526, #1843, #60912, #11677, #7809, #49650, #54933, #16948, #12384, #61267, #22939, #1478, #44381, #54584, #23980, #33505, #50008, #6409, #1135, #65870, #17665, #22586, #34555, #12037, #44026 ),
 .UNSPECIFIED., .F., .F.,
 ( 4, 2, 2, 2, 2, 2, 2, 2, 2, 2, 2, 2, 2, 2, 2, 2, 2, 2, 2, 2, 2, 2, 2, 2, 4 ),
 ( 0.03126542424884329319, 0.03330676804260272739, 0.03534811183636216853, 0.03738945563012160966, 0.03943079942388104386, 0.04045147132076077484, 0.04147214321764051276, 0.04249281511452024374, 0.04351348701139998165, 0.04555483080515944361, 0.04657550270203918152, 0.04759617459891891944, 0.04810651054735878146, 0.04861684649579864348, 0.04963751839267835364, 0.05065819028955807768, 0.05167886218643778784, 0.05269953408331751188, 0.05372020598019722204, 0.05474087787707693220, 0.05576154977395665624, 0.05780289356771613207, 0.05984423736147560791, 0.06188558115523508374, 0.06392692494899455957 ),
 .UNSPECIFIED. ) ;
#63661=CARTESIAN_POINT ( 'NONE',  ( 205.1049299651095907, 106.9023875785546238, -36.32593103262159673 ) ) ;
#63666=CARTESIAN_POINT ( 'NONE',  ( -72.21947956767111521, 21.03570528348188873, 60.92218443414460438 ) ) ;
#63667=CARTESIAN_POINT ( 'NONE',  ( -102.2801239173131194, 32.78103895658057354, -35.01457726497591239 ) ) ;
#63668=CARTESIAN_POINT ( 'NONE',  ( 55.51547041749727640, 11.05727559334827070, -70.30740390392726624 ) ) ;
#63670=CARTESIAN_POINT ( 'NONE',  ( 21.74799039132244260, 7.772294950329607488, 42.09455586677241001 ) ) ;
#63671=CARTESIAN_POINT ( 'NONE',  ( 160.2883311361769643, 61.16711613734476316, -63.51461744484596039 ) ) ;
#63677=CARTESIAN_POINT ( 'NONE',  ( -149.5074843970971017, 64.17983161892347255, 45.72082123989907387 ) ) ;
#63678=CARTESIAN_POINT ( 'NONE',  ( 61.33627421985469397, 12.28939706835343237, -35.90714437952212990 ) ) ;
#63679=DIRECTION ( 'NONE',  ( -1.000000000000000000, 0.000000000000000000, 0.000000000000000000 ) ) ;
#63680=CIRCLE ( 'NONE', #63628, 243.4957430088094839 ) ;
#63682=EDGE_CURVE ( 'NONE', #61969, #67011, #26243, .T. ) ;
#63683=CARTESIAN_POINT ( 'NONE',  ( -145.5261806899006842, 60.87473129144527917, 5.016016613215474429 ) ) ;
#63684=VERTEX_POINT ( 'NONE', #22280 ) ;
#63685=CARTESIAN_POINT ( 'NONE',  ( -130.5811943660945076, 50.88295841537572528, 32.24531123205569827 ) ) ;
#63687=EDGE_LOOP ( 'NONE', ( #16290, #24344 ) ) ;
#63688=CARTESIAN_POINT ( 'NONE',  ( 34.45972925205163762, 8.830088223935252500, -21.93772383615038635 ) ) ;
#63690=CARTESIAN_POINT ( 'NONE',  ( 205.5004956747123117, 107.4493581495447927, 29.23987150799703727 ) ) ;
#63691=CARTESIAN_POINT ( 'NONE',  ( -2.869721780807583666, 7.625909776230887616, 70.11086547301624705 ) ) ;
#63694=B_SPLINE_CURVE_WITH_KNOTS ( 'NONE', 3,
 ( #3332, #40272, #8266, #30073, #3671, #13203, #29718, #18817, #67707, #51180, #29370, #40611, #61720, #35000, #19157, #24793, #40962, #56104, #19501, #35344, #46231, #56441, #2995, #36031, #62062, #2301, #30759, #45543, #8622, #51526, #61378, #7920, #50823, #14238, #8960, #24454, #25146, #45895, #2642, #30407, #56803, #51861, #46577 ),
 .UNSPECIFIED., .F., .F.,
 ( 4, 2, 2, 2, 2, 2, 2, 2, 2, 2, 2, 1, 2, 2, 2, 2, 2, 2, 2, 2, 2, 4 ),
 ( 0.02515559250233026511, 0.02674001423437957076, 0.02753222510040422011, 0.02832443596642887293, 0.02990885769847824449, 0.03149327943052761258, 0.03307770116257698761, 0.03386991202860167860, 0.03466212289462636265, 0.03624654462667570298, 0.03703875549270038009, 0.03783096635872505720, 0.03862317722474973430, 0.03941538809077441141, 0.04099980982282376563, 0.04258423155487311290, 0.04337644242089779001, 0.04416865328692246712, 0.04575307501897181439, 0.04733749675102115473, 0.04892191848307049507, 0.05050634021511984234 ),
 .UNSPECIFIED. ) ;
#63696=EDGE_CURVE ( 'NONE', #61334, #52913, #6795, .T. ) ;
#63699=ORIENTED_EDGE ( 'NONE', *, *, #62346, .F. ) ;
#63701=CARTESIAN_POINT ( 'NONE',  ( -125.4034380163612212, 47.37464824346550074, 84.30384953410292326 ) ) ;
#63702=CARTESIAN_POINT ( 'NONE',  ( -125.8938041572051389, -170.0000000000000000, -49.91370389823397602 ) ) ;
#63704=CARTESIAN_POINT ( 'NONE',  ( 70.25990036603481315, 14.47042233282420298, 39.27062401723128460 ) ) ;
#63705=CARTESIAN_POINT ( 'NONE',  ( 8.285723989432073111, 7.382582932371003714, 90.57384125127391883 ) ) ;
#63707=VERTEX_POINT ( 'NONE', #40537 ) ;
#63709=CARTESIAN_POINT ( 'NONE',  ( -94.88380767928867954, 29.17964217339916644, 66.13299744995647700 ) ) ;
#63711=CARTESIAN_POINT ( 'NONE',  ( -84.23431294393863311, 24.52078568147204507, 6.024674515077490078 ) ) ;
#63715=CARTESIAN_POINT ( 'NONE',  ( -120.0051930351106506, 43.92079660368832350, 15.92705009691551865 ) ) ;
#63716=CARTESIAN_POINT ( 'NONE',  ( -176.3791001330698975, 90.82833141237288999, 71.93620537013939042 ) ) ;
#63717=CARTESIAN_POINT ( 'NONE',  ( 130.3245512970360664, 39.33195360491890824, 70.48796868334781607 ) ) ;
#63720=B_SPLINE_CURVE_WITH_KNOTS ( 'NONE', 3,
 ( #60736, #18183, #50187, #55819, #35055, #39980, #23470, #56497, #29772, #8678, #51235, #51582, #39634, #61090, #3052, #24846, #46285, #50537, #23809, #56155, #45251, #61439, #34717, #7972, #35753, #14966, #47313, #30816, #57203, #52262, #68772, #36092, #53277, #42050, #25203, #48002, #41709, #46637 ),
 .UNSPECIFIED., .F., .F.,
 ( 4, 2, 2, 2, 2, 2, 2, 2, 2, 2, 2, 2, 2, 2, 2, 2, 2, 2, 4 ),
 ( 1.387778780781445676E-17, 0.003908178031105413383, 0.005862267046658129616, 0.007816356062210845848, 0.009770445077763562081, 0.01172453409331627831, 0.01270157860109262862, 0.01367862310886898240, 0.01465566761664533271, 0.01563271212442168476, 0.01660975663219804027, 0.01758680113997438538, 0.01954089015552708253, 0.02051793466330342416, 0.02149497917107976580, 0.02344906818663246642, 0.02540315720218516357, 0.02735724621773786766, 0.03126542424884323768 ),
 .UNSPECIFIED. ) ;
#63722=CARTESIAN_POINT ( 'NONE',  ( -38.94401347518159895, 10.94428672445531348, 91.58116192842672376 ) ) ;
#63724=CARTESIAN_POINT ( 'NONE',  ( 149.9872551245000807, 52.05943539582076340, 37.48403949321973982 ) ) ;
#63727=CARTESIAN_POINT ( 'NONE',  ( 103.1653143050726271, 25.74301230421576747, -40.88985240790263020 ) ) ;
#63728=CARTESIAN_POINT ( 'NONE',  ( -30.94753041835915752, 9.510749728915508072, 45.21645440618920020 ) ) ;
#63736=CARTESIAN_POINT ( 'NONE',  ( -118.8392474096541918, 43.20060570451233417, -45.01293686198101796 ) ) ;
#63737=CARTESIAN_POINT ( 'NONE',  ( -82.93126516400698733, 25.07709093823495650, 4.899509067904407544 ) ) ;
#63740=CARTESIAN_POINT ( 'NONE',  ( 34.47024887486590217, 7.819232357299694236, -91.15458136497296948 ) ) ;
#63742=CARTESIAN_POINT ( 'NONE',  ( 70.50372867914781239, 14.53505678900966380, 10.95890223166102118 ) ) ;
#63743=CARTESIAN_POINT ( 'NONE',  ( -80.32755469740935439, 24.04130076192508270, 72.08040740567068383 ) ) ;
#63744=CARTESIAN_POINT ( 'NONE',  ( -109.7078892845591582, 36.71702188566216307, 39.09037949355451502 ) ) ;
#63745=VERTEX_POINT ( 'NONE', #13805 ) ;
#63747=CARTESIAN_POINT ( 'NONE',  ( -56.32964631401103617, 16.07016196819930087, 84.08885397732279898 ) ) ;
#63751=CARTESIAN_POINT ( 'NONE',  ( 22.90619343622340764, 7.840927939412484449, -72.27737759400322659 ) ) ;
#63755=CARTESIAN_POINT ( 'NONE',  ( 140.4641697461912884, 46.75994457266055804, -39.93676995691901510 ) ) ;
#63756=CARTESIAN_POINT ( 'NONE',  ( -51.77431913897919458, 14.86466849149170777, -62.79783711398949464 ) ) ;
#63757=CARTESIAN_POINT ( 'NONE',  ( 151.6351261592328683, 53.25263237790398563, -38.90572743852373350 ) ) ;
#63760=ORIENTED_EDGE ( 'NONE', *, *, #19931, .T. ) ;
#63763=EDGE_CURVE ( 'NONE', #27226, #52905, #66604, .T. ) ;
#63766=EDGE_CURVE ( 'NONE', #43079, #14540, #3561, .T. ) ;
#63767=CARTESIAN_POINT ( 'NONE',  ( 131.2739575565289272, 41.05411765250562439, -90.16079167367058744 ) ) ;
#63771=CARTESIAN_POINT ( 'NONE',  ( 176.4367926094704728, 74.03315361639846515, -76.46119564883423436 ) ) ;
#63774=CARTESIAN_POINT ( 'NONE',  ( 89.21005684773500377, 20.31770592753387916, -23.52307059860430627 ) ) ;
#63775=CYLINDRICAL_SURFACE ( 'NONE', #48788, 7.500000000000013323 ) ;
#63776=DIRECTION ( 'NONE',  ( 0.000000000000000000, 0.000000000000000000, 1.000000000000000000 ) ) ;
#63779=EDGE_CURVE ( 'NONE', #53742, #28520, #57270, .T. ) ;
#63788=CARTESIAN_POINT ( 'NONE',  ( -5.583677117989181760, 7.762972448524147140, 84.14020024624272764 ) ) ;
#63792=DIRECTION ( 'NONE',  ( 0.000000000000000000, 0.000000000000000000, 1.000000000000000000 ) ) ;
#63795=CARTESIAN_POINT ( 'NONE',  ( 39.08704187494956983, 9.383114233299528095, 83.60237209767953459 ) ) ;
#63797=CARTESIAN_POINT ( 'NONE',  ( 110.2429982417149574, -170.0000000000000000, 63.95576479620102361 ) ) ;
#63800=CARTESIAN_POINT ( 'NONE',  ( -6.840981040171510763, 6.828436339979224279, 18.22255534678397026 ) ) ;
#63801=CARTESIAN_POINT ( 'NONE',  ( 32.90878072717890745, 7.653588083204842185, -12.51371383138284443 ) ) ;
#63802=CARTESIAN_POINT ( 'NONE',  ( 159.2325040199866635, 60.31699144791972600, 44.25496482726027381 ) ) ;
#63803=CARTESIAN_POINT ( 'NONE',  ( 164.0443904173016847, 62.94849960635616526, 86.97141621194363381 ) ) ;
#63806=CARTESIAN_POINT ( 'NONE',  ( 103.1695711638930959, 26.83837309506523638, -19.12163667725788940 ) ) ;
#63809=CARTESIAN_POINT ( 'NONE',  ( 204.3129818922372749, 107.5244029525887868, 29.20772073876942443 ) ) ;
#63815=CARTESIAN_POINT ( 'NONE',  ( 112.1100957124161539, 30.86846953551572525, -77.54606385092635890 ) ) ;
#63816=DIRECTION ( 'NONE',  ( -0.000000000000000000, 1.000000000000000000, -0.000000000000000000 ) ) ;
#63817=CARTESIAN_POINT ( 'NONE',  ( 197.8572563162090319, 97.41072138832259952, -67.58039613982114702 ) ) ;
#63818=CARTESIAN_POINT ( 'NONE',  ( -31.92572261726339633, 10.69135962481465008, 57.06100499665285497 ) ) ;
#63819=CARTESIAN_POINT ( 'NONE',  ( -14.56151485655250788, 8.434196591921333308, -19.40760647807576333 ) ) ;
#63821=CARTESIAN_POINT ( 'NONE',  ( 155.2910738464913720, 55.97560547655807284, -77.65936666156605384 ) ) ;
#63822=CARTESIAN_POINT ( 'NONE',  ( 17.48889770758267304, 6.561062909825354339, -23.48319453253814260 ) ) ;
#63823=CARTESIAN_POINT ( 'NONE',  ( -155.5978531700835958, 69.52241200678682276, -37.92872988257907707 ) ) ;
#63828=CARTESIAN_POINT ( 'NONE',  ( -84.55783695959763691, 25.74181993349145614, -37.94774160841574684 ) ) ;
#63829=CARTESIAN_POINT ( 'NONE',  ( 106.0226973295788468, 26.97779350220217154, 84.59144110998217059 ) ) ;
#63830=CARTESIAN_POINT ( 'NONE',  ( -154.8006992380338716, 70.15733562427989511, 16.71094074788830497 ) ) ;
#63834=CARTESIAN_POINT ( 'NONE',  ( 23.28785143291466397, 6.856621069835718174, 37.01352062635557161 ) ) ;
#63835=CARTESIAN_POINT ( 'NONE',  ( -156.9646383917485650, 72.14225053943575006, 91.09065068128420251 ) ) ;
#63836=EDGE_LOOP ( 'NONE', ( #60580, #68505, #55270, #67981 ) ) ;
#63837=ORIENTED_EDGE ( 'NONE', *, *, #13025, .F. ) ;
#63842=EDGE_CURVE ( 'NONE', #66387, #39196, #20252, .T. ) ;
#63843=CARTESIAN_POINT ( 'NONE',  ( 91.42704446803595886, 22.18527496519091713, -91.23189972359006106 ) ) ;
#63844=CARTESIAN_POINT ( 'NONE',  ( 103.1665074762347700, 25.74358939450902639, -94.59055577750497434 ) ) ;
#63847=CARTESIAN_POINT ( 'NONE',  ( -31.43908319763709969, 9.591432048623765638, 57.06100499665286208 ) ) ;
#63848=CARTESIAN_POINT ( 'NONE',  ( -154.2585856850054995, 68.31650218414620213, -21.27640989008226313 ) ) ;
#63849=ORIENTED_EDGE ( 'NONE', *, *, #40424, .T. ) ;
#63850=CARTESIAN_POINT ( 'NONE',  ( 184.5867277229703802, 83.68414666546580349, 70.28875302066492736 ) ) ;
#63851=CARTESIAN_POINT ( 'NONE',  ( 10.13405324523498408, 6.385324379632245417, -21.12665790197542037 ) ) ;
#63852=CARTESIAN_POINT ( 'NONE',  ( 21.74799039132244260, 7.772294950329608376, 15.25000527630873393 ) ) ;
#63853=CARTESIAN_POINT ( 'NONE',  ( 188.0141161196705752, 85.90515114331884661, 66.53510735707675394 ) ) ;
#63855=CARTESIAN_POINT ( 'NONE',  ( -78.66644367742111399, 22.32174330031317311, -35.11545063171788428 ) ) ;
#63856=CARTESIAN_POINT ( 'NONE',  ( 21.44031696305384571, 6.747195267824411147, 69.31344765735015301 ) ) ;
#63858=CARTESIAN_POINT ( 'NONE',  ( 8.480977594057446112, 7.382886909400592224, 8.963374414903345411 ) ) ;
#63859=EDGE_CURVE ( 'NONE', #64139, #51909, #29470, .T. ) ;
#63861=CARTESIAN_POINT ( 'NONE',  ( 184.3994103300443896, 82.02159554764426730, 16.70644533388108144 ) ) ;
#63863=PLANE ( 'NONE',  #24035 ) ;
#63865=CARTESIAN_POINT ( 'NONE',  ( -107.0544991134679265, 36.41543129049374983, -48.30370310564277503 ) ) ;
#63866=CARTESIAN_POINT ( 'NONE',  ( 181.5079096844946491, 80.47139261082473638, -51.22505766587965326 ) ) ;
#63867=ORIENTED_EDGE ( 'NONE', *, *, #51765, .T. ) ;
#63871=VERTEX_POINT ( 'NONE', #23944 ) ;
#63873=CARTESIAN_POINT ( 'NONE',  ( 110.2429982417149290, 28.88204397445231209, 56.45576479620100940 ) ) ;
#63876=CARTESIAN_POINT ( 'NONE',  ( 132.9440032680862771, 40.87616997986732059, 29.56257473360772892 ) ) ;
#63878=CARTESIAN_POINT ( 'NONE',  ( -99.97541017369786687, 31.62502926470687470, 45.17167492092433179 ) ) ;
#63880=CARTESIAN_POINT ( 'NONE',  ( 93.92280655489132357, 22.03989931749466535, -45.08756213313548500 ) ) ;
#63886=CARTESIAN_POINT ( 'NONE',  ( -31.43908319763710679, -170.0000000000000000, -23.47264677473818395 ) ) ;
#63887=CARTESIAN_POINT ( 'NONE',  ( -180.6011569556094969, 95.85968111394262792, -15.99745918700219072 ) ) ;
#63888=CARTESIAN_POINT ( 'NONE',  ( -172.3038663181179970, 87.72015621195184565, -61.55650775521367990 ) ) ;
#63889=CARTESIAN_POINT ( 'NONE',  ( -146.1260528621667731, 61.36307454672302697, -49.02329722400514811 ) ) ;
#63893=CARTESIAN_POINT ( 'NONE',  ( -133.1527834403230486, 51.46311219732123732, 40.02479403497597588 ) ) ;
#63895=CARTESIAN_POINT ( 'NONE',  ( -61.86403937395562025, 16.61416349803656800, -12.72252382116044522 ) ) ;
#63896=CARTESIAN_POINT ( 'NONE',  ( -96.43817545481738307, 31.02509717589733640, 60.13372018734977331 ) ) ;
#63897=CARTESIAN_POINT ( 'NONE',  ( -132.2161740628506550, 52.03204870034954865, -73.30095993089241801 ) ) ;
#63898=CARTESIAN_POINT ( 'NONE',  ( -55.05276343752909440, 14.68156374112638929, -77.06087458892358200 ) ) ;
#63900=CARTESIAN_POINT ( 'NONE',  ( -100.4262673593280368, 31.84860241619272969, -62.07669865031897416 ) ) ;
#63902=ORIENTED_EDGE ( 'NONE', *, *, #12389, .T. ) ;
#63906=CARTESIAN_POINT ( 'NONE',  ( 103.5849290181279088, 27.01613348792540847, -73.72874238742858211 ) ) ;
#63907=CARTESIAN_POINT ( 'NONE',  ( -71.17984086584779391, 20.67393782512344558, 38.43314760115057993 ) ) ;
#63908=CARTESIAN_POINT ( 'NONE',  ( 81.03898448521319153, 17.58847173596443270, 32.18774333821972533 ) ) ;
#63909=CARTESIAN_POINT ( 'NONE',  ( 69.36287815987334682, 15.27486453472191208, -47.22355319605652824 ) ) ;
#63910=CARTESIAN_POINT ( 'NONE',  ( -122.8011284400168108, 45.68452922414294193, 31.27179024729560908 ) ) ;
#63912=ORIENTED_EDGE ( 'NONE', *, *, #16588, .T. ) ;
#63913=CARTESIAN_POINT ( 'NONE',  ( -104.1244073710070239, 33.72720758483612258, -8.385545890535196278 ) ) ;
#63916=CARTESIAN_POINT ( 'NONE',  ( -11.14880195267006968, 7.129907723790826601, -36.17668213044176184 ) ) ;
#63918=CARTESIAN_POINT ( 'NONE',  ( 88.98820631332498010, 21.30618275724810573, 56.92102499358249901 ) ) ;
#63919=CARTESIAN_POINT ( 'NONE',  ( 150.9184679586219033, 52.73111408630722963, -13.12037300805640783 ) ) ;
#63923=CARTESIAN_POINT ( 'NONE',  ( 31.96227686234409759, 7.558148489540045034, -70.94545158898284853 ) ) ;
#63924=CARTESIAN_POINT ( 'NONE',  ( -95.60805465865863084, 30.63099276904602419, -72.82232827928781660 ) ) ;
#63926=CARTESIAN_POINT ( 'NONE',  ( -31.93169728792082651, 10.69234447276976852, -8.472646774738153752 ) ) ;
#63927=AXIS2_PLACEMENT_3D ( 'NONE', #23561, #7730, #12655 ) ;
#63931=DIRECTION ( 'NONE',  ( 0.000000000000000000, 0.000000000000000000, 1.000000000000000000 ) ) ;
#63932=CARTESIAN_POINT ( 'NONE',  ( 10.83521140779422609, 7.398743030771587570, -75.51647902447882643 ) ) ;
#63933=CARTESIAN_POINT ( 'NONE',  ( -27.70005010046227412, 9.007417901453017350, 17.37802900940060624 ) ) ;
#63935=CARTESIAN_POINT ( 'NONE',  ( -6.840981040171507210, 6.828436339979226055, 45.06710593724763214 ) ) ;
#63937=CARTESIAN_POINT ( 'NONE',  ( 150.0980941434704903, 53.37942190380065455, -45.02911393569248588 ) ) ;
#63939=ORIENTED_EDGE ( 'NONE', *, *, #43807, .T. ) ;
#63941=CARTESIAN_POINT ( 'NONE',  ( -152.5101325120252795, 68.10842280990928543, 71.95230034876590253 ) ) ;
#63945=CARTESIAN_POINT ( 'NONE',  ( -109.0291978193666438, 37.49173305805086898, 61.58271146452185718 ) ) ;
#63946=CARTESIAN_POINT ( 'NONE',  ( -129.4036885357273832, 50.06837984316182144, -35.78160727525695961 ) ) ;
#63949=CARTESIAN_POINT ( 'NONE',  ( 92.53566308513175898, 21.52138666710688142, 68.70529524960606693 ) ) ;
#63950=CARTESIAN_POINT ( 'NONE',  ( 197.6329787101074658, 98.74106466892200729, -19.51727163173970681 ) ) ;
#63951=CARTESIAN_POINT ( 'NONE',  ( -142.0117116388610157, 58.07347023268670227, 91.60223103192235783 ) ) ;
#63952=CARTESIAN_POINT ( 'NONE',  ( 140.4586216751744701, 45.55624550472996503, 33.44244638526205193 ) ) ;
#63956=CARTESIAN_POINT ( 'NONE',  ( 163.1313205310724186, 63.49733392291055623, 14.99077136729292015 ) ) ;
#63957=CYLINDRICAL_SURFACE ( 'NONE', #57774, 7.500000000000020428 ) ;
#63960=CARTESIAN_POINT ( 'NONE',  ( 173.9405361758639117, 73.05302209498822208, 65.95550401125700546 ) ) ;
#63962=CARTESIAN_POINT ( 'NONE',  ( -106.6781182590523400, 35.07133425426479079, -36.42098577216694366 ) ) ;
#63963=CARTESIAN_POINT ( 'NONE',  ( 63.01563776193091826, 12.67277567978498176, -77.56524142263344856 ) ) ;
#63966=CARTESIAN_POINT ( 'NONE',  ( 155.2870855780214754, 57.23765125306422163, 17.25424900018499486 ) ) ;
#63968=CARTESIAN_POINT ( 'NONE',  ( 160.5018603162735076, 61.33906090758085838, -50.49884186580090528 ) ) ;
#63973=EDGE_CURVE ( 'NONE', #62155, #18800, #56009, .T. ) ;
#63975=EDGE_CURVE ( 'NONE', #30581, #39218, #56386, .T. ) ;
#63976=CARTESIAN_POINT ( 'NONE',  ( 138.6020257460769756, 44.36414356192208430, 69.68300242728969351 ) ) ;
#63977=DIRECTION ( 'NONE',  ( -0.000000000000000000, 1.000000000000000000, -0.000000000000000000 ) ) ;
#63978=CARTESIAN_POINT ( 'NONE',  ( -38.69408084385329971, 10.89529537250242974, -67.69614563400999430 ) ) ;
#63980=CARTESIAN_POINT ( 'NONE',  ( 42.71680114082826663, 9.880016734137541334, 17.31480560921531975 ) ) ;
#63985=CARTESIAN_POINT ( 'NONE',  ( -62.21707580470530274, 16.72016638215685447, 93.81846384057118371 ) ) ;
#63987=CARTESIAN_POINT ( 'NONE',  ( -152.5067928559255392, 66.76529500553621688, -76.04591788159349619 ) ) ;
#63988=CARTESIAN_POINT ( 'NONE',  ( -108.8294929810133880, 36.23425003200458860, 88.03925474513930283 ) ) ;
#63989=CARTESIAN_POINT ( 'NONE',  ( 188.2950976467627413, 87.71503060978560029, 12.04681166319859997 ) ) ;
#63990=EDGE_CURVE ( 'NONE', #53396, #57040, #15117, .T. ) ;
#63991=CARTESIAN_POINT ( 'NONE',  ( -131.1078488676298832, 50.02394948559179255, 70.36092292693098216 ) ) ;
#63994=ORIENTED_EDGE ( 'NONE', *, *, #8680, .F. ) ;
#63997=CARTESIAN_POINT ( 'NONE',  ( -75.00452312211128003, 22.03104735285382887, 58.21301458073671142 ) ) ;
#63998=CARTESIAN_POINT ( 'NONE',  ( 182.5617509987552864, 80.11195108039726165, 29.45250294282221404 ) ) ;
#64000=CARTESIAN_POINT ( 'NONE',  ( 57.08336938683661543, 11.37442068895389191, -65.44980484747004823 ) ) ;
#64001=B_SPLINE_CURVE_WITH_KNOTS ( 'NONE', 3,
 ( #15903, #15213, #41599, #5000, #69009, #9943, #58127, #32083, #42293, #52156, #31399, #35983, #42632, #25786, #63755, #46882, #64089, #52830, #47212, #57782, #42962, #9249, #68344, #20147, #37344, #53519, #20482, #30706, #41946, #58456, #63058, #3973, #14862, #10271, #58797, #48233, #10613, #36327, #5351, #4652, #63410, #9596, #58, #21518, #31058, #26114, #52502, #12016 ),
 .UNSPECIFIED., .F., .F.,
 ( 4, 2, 2, 2, 2, 2, 2, 2, 2, 2, 2, 2, 2, 2, 2, 2, 2, 2, 2, 2, 2, 2, 2, 4 ),
 ( 6.938893903907228378E-18, 0.001591515129442207981, 0.003183030258884409023, 0.003978787823605504231, 0.004774545388326600741, 0.006366060517768843199, 0.007957575647211086525, 0.009549090776653329851, 0.01034484834137445845, 0.01114060590609558532, 0.01193636347081671219, 0.01273212103553784079, 0.01432363616498011881, 0.01591515129442239510, 0.01671090885914353064, 0.01750666642386466271, 0.01830242398858579825, 0.01909818155330693379, 0.02068969668274925344, 0.02148545424747042021, 0.02228121181219158697, 0.02387272694163384071, 0.02466848450635493462, 0.02546424207107603199 ),
 .UNSPECIFIED. ) ;
#64002=CARTESIAN_POINT ( 'NONE',  ( -76.32962633615586867, 21.44528079176259538, 3.942966790981714098 ) ) ;
#64003=CARTESIAN_POINT ( 'NONE',  ( -122.1940143064357187, 45.29738883755586443, 71.49263784387757426 ) ) ;
#64004=CARTESIAN_POINT ( 'NONE',  ( 23.24047374271773592, 7.861801299833796719, 38.49384045076077143 ) ) ;
#64006=CARTESIAN_POINT ( 'NONE',  ( 198.6830395803476108, 98.44480157511503648, 85.91292533661551545 ) ) ;
#64011=CARTESIAN_POINT ( 'NONE',  ( -172.7116702014379825, 86.67317892691258407, 72.66624519710477159 ) ) ;
#64012=ORIENTED_EDGE ( 'NONE', *, *, #26494, .T. ) ;
#64013=EDGE_LOOP ( 'NONE', ( #18952, #16279, #61927, #27914 ) ) ;
#64014=CARTESIAN_POINT ( 'NONE',  ( -25.79929641484369185, 9.749255553662443674, -74.63048772539220010 ) ) ;
#64018=CARTESIAN_POINT ( 'NONE',  ( -149.0782809666403921, 63.81577337591404131, 3.876270649435374693 ) ) ;
#64025=CARTESIAN_POINT ( 'NONE',  ( -133.1640943168118838, 52.70734926280005794, 39.98146393653333064 ) ) ;
#64029=CARTESIAN_POINT ( 'NONE',  ( 58.47673920847985585, 11.66523265296355305, 58.16705259761723568 ) ) ;
#64037=CARTESIAN_POINT ( 'NONE',  ( -165.7689197919845014, 79.30072199592279958, -13.85662846433732831 ) ) ;
#64038=CARTESIAN_POINT ( 'NONE',  ( 137.3958226571046737, 43.60243650158410134, -76.99682858792697004 ) ) ;
#64040=VECTOR ( 'NONE', #60178, 1000.000000000000000 ) ;
#64041=CARTESIAN_POINT ( 'NONE',  ( -189.4248691432192402, 107.3461292335514514, -70.68823927268300622 ) ) ;
#64043=CARTESIAN_POINT ( 'NONE',  ( -95.19652294162979445, 29.32558722310179888, 67.38094733532032876 ) ) ;
#64044=ORIENTED_EDGE ( 'NONE', *, *, #65765, .F. ) ;
#64048=CARTESIAN_POINT ( 'NONE',  ( -120.1346137380981958, 44.00127440773565723, 6.464595127001305563 ) ) ;
#64049=CARTESIAN_POINT ( 'NONE',  ( -179.6470915626256613, 94.69856161161349917, 61.45973726863883968 ) ) ;
#64050=CARTESIAN_POINT ( 'NONE',  ( 20.37135563017390183, 6.690359945346087578, 16.62731626407598640 ) ) ;
#64052=B_SPLINE_CURVE_WITH_KNOTS ( 'NONE', 3,
 ( #21407, #36908, #37234, #58346, #47790, #53059, #4887, #58685, #53402, #27028, #32662, #16131, #5908, #59033, #10855, #21749, #27370, #43196, #64673, #16480, #37935, #59380, #68571, #20373, #60075, #18225, #48810, #23157, #28419, #65021, #16816, #39334, #34060, #66437, #2057, #50235, #44950, #54800, #39676, #12601, #33373, #49872, #61136, #12959 ),
 .UNSPECIFIED., .F., .F.,
 ( 4, 2, 2, 2, 2, 2, 2, 2, 2, 2, 2, 2, 2, 2, 2, 2, 2, 2, 2, 2, 2, 4 ),
 ( 0.02908143158676661927, 0.03095422299093867138, 0.03282701439511072350, 0.03469980579928277908, 0.03657259720345483467, 0.03844538860762689025, 0.04031818001179893890, 0.04125457571388495281, 0.04219097141597095979, 0.04312736711805697370, 0.04359556496909998413, 0.04406376282014300150, 0.04500015852222903623, 0.04593655422431506402, 0.04687294992640109181, 0.04780934562848712654, 0.04968213703265919601, 0.05155492843683127935, 0.05342771984100334881, 0.05530051124517543215, 0.05717330264934750855, 0.05904609405351958495 ),
 .UNSPECIFIED. ) ;
#64055=CARTESIAN_POINT ( 'NONE',  ( 150.7926588734435427, 52.63999027731880176, 40.33416883845127643 ) ) ;
#64057=CARTESIAN_POINT ( 'NONE',  ( 63.01563776193090405, 13.70579113808098271, 71.65751152968501003 ) ) ;
#64059=CARTESIAN_POINT ( 'NONE',  ( -23.93965512371325133, 8.480096402797091315, 37.21140884057258802 ) ) ;
#64061=ORIENTED_EDGE ( 'NONE', *, *, #46932, .F. ) ;
#64064=FACE_BOUND ( 'NONE', #29196, .T. ) ;
#64066=CARTESIAN_POINT ( 'NONE',  ( -85.66184035008927822, 26.20110535976566979, -66.74364312913436947 ) ) ;
#64067=CARTESIAN_POINT ( 'NONE',  ( -149.5074843970971017, 65.50121172469319220, -7.968279941028269420 ) ) ;
#64069=CARTESIAN_POINT ( 'NONE',  ( -80.31482177285911916, 24.03632224640839610, 3.753151970507568436 ) ) ;
#64073=CARTESIAN_POINT ( 'NONE',  ( -118.4106078162223525, 42.93830006159887347, -68.68850339543098471 ) ) ;
#64074=CARTESIAN_POINT ( 'NONE',  ( 67.93926590385571274, 13.86859831467923065, 16.14705051833222171 ) ) ;
#64075=CARTESIAN_POINT ( 'NONE',  ( -85.12122836439576190, 25.97531040437156591, 68.61395634379843500 ) ) ;
#64076=CARTESIAN_POINT ( 'NONE',  ( 41.44377882552309700, 9.699415982225042754, -89.58024731985329936 ) ) ;
#64077=EDGE_LOOP ( 'NONE', ( #11178, #45614 ) ) ;
#64081=LINE ( 'NONE', #37338, #350 ) ;
#64084=CARTESIAN_POINT ( 'NONE',  ( 20.35964562795319921, 7.697260051881319676, -63.89753274017193263 ) ) ;
#64086=CARTESIAN_POINT ( 'NONE',  ( -146.1140637052939155, 62.65471088530802035, 58.36122317852547070 ) ) ;
#64089=CARTESIAN_POINT ( 'NONE',  ( 140.8855094313933023, 47.03549517811089231, -40.89384161477261870 ) ) ;
#64090=CARTESIAN_POINT ( 'NONE',  ( 209.8197250501989970, 115.4463023161200823, -92.02305923795135811 ) ) ;
#64092=CYLINDRICAL_SURFACE ( 'NONE', #14993, 7.500000000000020428 ) ;
#64094=ORIENTED_EDGE ( 'NONE', *, *, #30263, .F. ) ;
#64095=CARTESIAN_POINT ( 'NONE',  ( 70.51601918574517924, 14.53832276813547431, -42.98226787025442519 ) ) ;
#64097=CARTESIAN_POINT ( 'NONE',  ( -55.05276343752910151, 14.68156374112637330, -88.90542517938719413 ) ) ;
#64104=CARTESIAN_POINT ( 'NONE',  ( 88.52077179907877280, 21.14145351760140557, 17.62907072079950410 ) ) ;
#64105=CARTESIAN_POINT ( 'NONE',  ( 188.0094179620990928, 87.39792407168452826, -19.77360373632219392 ) ) ;
#64106=CARTESIAN_POINT ( 'NONE',  ( 212.1913428512246753, 119.0779339498137688, 9.508615975002843612 ) ) ;
#64108=CARTESIAN_POINT ( 'NONE',  ( -180.3158531669106708, 95.51092859788505507, -44.35178396430072922 ) ) ;
#64110=DIRECTION ( 'NONE',  ( -0.000000000000000000, 1.000000000000000000, -0.000000000000000000 ) ) ;
#64113=CARTESIAN_POINT ( 'NONE',  ( 164.8908506817023181, 64.97619709085121542, 64.87856429165069017 ) ) ;
#64117=CARTESIAN_POINT ( 'NONE',  ( 155.2870855780215891, 57.23765125306421453, 70.94335018111237900 ) ) ;
#64119=CARTESIAN_POINT ( 'NONE',  ( 150.8925291903904053, 52.71218673668931842, 6.422435693488909969 ) ) ;
#64126=CARTESIAN_POINT ( 'NONE',  ( 33.04185335729066253, 8.678858904955234266, 87.11446200076579771 ) ) ;
#64130=CARTESIAN_POINT ( 'NONE',  ( -62.49130718206700408, 16.80297926264070796, -70.55131870819045048 ) ) ;
#64132=CARTESIAN_POINT ( 'NONE',  ( -5.412684891282530053, 7.753215344827987465, 3.652707060347378576 ) ) ;
#64133=CARTESIAN_POINT ( 'NONE',  ( 174.9161599490640810, 73.97365196673304411, -48.00021783180836366 ) ) ;
#64139=VERTEX_POINT ( 'NONE', #28431 ) ;
#64143=CARTESIAN_POINT ( 'NONE',  ( 10.15118267943872432, 7.391905976536037315, 32.56151896041566118 ) ) ;
#64144=CARTESIAN_POINT ( 'NONE',  ( 201.9721407532274782, 104.3507814346147597, 43.70693720603514265 ) ) ;
#64154=CARTESIAN_POINT ( 'NONE',  ( -37.52119286077852678, 11.69341290629619756, 60.16572187417437334 ) ) ;
#64155=CARTESIAN_POINT ( 'NONE',  ( -15.07533778868020669, 8.482826962130836534, -14.13728325526587781 ) ) ;
#64156=CARTESIAN_POINT ( 'NONE',  ( 149.9872551245001375, 52.05943539582077051, -69.89416286863497874 ) ) ;
#64160=ADVANCED_FACE ( 'NONE', ( #39343 ), #13312, .F. ) ;
#64161=ORIENTED_EDGE ( 'NONE', *, *, #20549, .F. ) ;
#64163=CARTESIAN_POINT ( 'NONE',  ( 63.50537371531942199, 13.81987663608982331, -8.876140241706055534 ) ) ;
#64164=CARTESIAN_POINT ( 'NONE',  ( -80.32755469740935439, 24.04130076192510046, -35.29779495618403473 ) ) ;
#64166=CARTESIAN_POINT ( 'NONE',  ( 116.6436511186860656, 33.08230081168870385, -12.66062602132463866 ) ) ;
#64169=CARTESIAN_POINT ( 'NONE',  ( -156.6359381387761118, 71.83770944710386175, 89.57239090401904491 ) ) ;
#64170=ORIENTED_EDGE ( 'NONE', *, *, #1847, .T. ) ;
#64173=CARTESIAN_POINT ( 'NONE',  ( -156.1477286774994298, 71.38742644140637594, -11.97128653975141965 ) ) ;
#64174=CARTESIAN_POINT ( 'NONE',  ( 37.45439421541016145, 9.177432671831375899, -35.86035370546551349 ) ) ;
#64177=CARTESIAN_POINT ( 'NONE',  ( -35.17600017528511103, 10.23461991275926586, 58.05366031714377328 ) ) ;
#64178=CARTESIAN_POINT ( 'NONE',  ( 198.7123879174244223, 100.1053816708572697, 59.02484461029090568 ) ) ;
#64181=CARTESIAN_POINT ( 'NONE',  ( -156.9910258076866398, 70.79617246506501260, 64.49172258714661154 ) ) ;
#64183=CARTESIAN_POINT ( 'NONE',  ( 18.19858669090299230, 7.596860100017451600, 17.77656158943756992 ) ) ;
#64186=CARTESIAN_POINT ( 'NONE',  ( -85.75947274862032543, 25.15128705015478516, -45.10382441638937934 ) ) ;
#64187=CARTESIAN_POINT ( 'NONE',  ( 23.09784929786603058, 6.844738137842329984, 66.05627411941513571 ) ) ;
#64190=CARTESIAN_POINT ( 'NONE',  ( 12.03317402819681980, 6.409531826169462043, -76.36039639407782431 ) ) ;
#64192=EDGE_LOOP ( 'NONE', ( #66964, #47922 ) ) ;
#64193=CARTESIAN_POINT ( 'NONE',  ( -102.2801239173131194, -170.0000000000000000, -61.85912785543958847 ) ) ;
#64196=CARTESIAN_POINT ( 'NONE',  ( 173.6718135456486607, 71.42581476597409562, 37.98988606938989676 ) ) ;
#64198=CARTESIAN_POINT ( 'NONE',  ( -109.3585523124447434, 37.67345343047318096, -39.98222387189748162 ) ) ;
#64199=CARTESIAN_POINT ( 'NONE',  ( 62.53356220515465935, 13.59349015304565000, -77.56524142263343435 ) ) ;
#64202=CARTESIAN_POINT ( 'NONE',  ( -23.95096213915837069, 8.481591526885939203, -15.48390114642075588 ) ) ;
#64203=CARTESIAN_POINT ( 'NONE',  ( 197.2199163281727863, 98.22431253015351160, 9.199768454146621366 ) ) ;
#64204=VERTEX_POINT ( 'NONE', #65735 ) ;
#64209=DIRECTION ( 'NONE',  ( -0.000000000000000000, 0.000000000000000000, -1.000000000000000000 ) ) ;
#64210=B_SPLINE_CURVE_WITH_KNOTS ( 'NONE', 3,
 ( #55223, #38353, #28504, #39064, #34139, #22523, #12324, #49239, #44319, #49587, #1419, #38710, #60154, #22877, #65806, #49947, #1778, #17952, #39404, #60852, #48531, #21819, #46403, #61207, #45019, #18991, #13709, #34835, #57317, #56621, #13035, #8443, #29892, #24628, #3168, #34497, #29200, #35162, #19677, #8086, #39754, #51694, #40440, #55934, #51356, #14056, #61556, #30243 ),
 .UNSPECIFIED., .F., .F.,
 ( 4, 2, 2, 2, 2, 2, 2, 2, 2, 2, 2, 2, 2, 2, 2, 2, 2, 2, 2, 2, 2, 2, 2, 4 ),
 ( 0.02746511744866865501, 0.02914922134997097181, 0.03083332525127328513, 0.03251742915257559846, 0.03335948110322677768, 0.03420153305387795689, 0.03504358500452913611, 0.03588563695518031532, 0.03756974085648259742, 0.03841179280713374194, 0.03925384475778488647, 0.04009589670843603099, 0.04093794865908717551, 0.04262205256038942291, 0.04430615646169167032, 0.04514820841234279403, 0.04599026036299390385, 0.04767436426429618596, 0.04935846816559846806, 0.05020052011624961258, 0.05104257206690077098, 0.05272667596820312941, 0.05356872791885428781, 0.05441077986950545314 ),
 .UNSPECIFIED. ) ;
#64211=CARTESIAN_POINT ( 'NONE',  ( -173.1211646369891071, 87.12891641440859303, 18.97714401617737678 ) ) ;
#64212=CARTESIAN_POINT ( 'NONE',  ( -7.825402957745081878, 7.899365992529268965, -23.57352014148015584 ) ) ;
#64213=CARTESIAN_POINT ( 'NONE',  ( 82.82003103503667774, 18.15602011327363385, -90.53761154839286007 ) ) ;
#64215=CARTESIAN_POINT ( 'NONE',  ( 87.10668362745099103, 19.58396519288864113, -50.82156419891175858 ) ) ;
#64220=CARTESIAN_POINT ( 'NONE',  ( -118.6157340058430094, 41.88485941274768010, -13.73874819522372981 ) ) ;
#64224=CARTESIAN_POINT ( 'NONE',  ( -179.5178913137217194, 94.54206947403388028, -11.41325856914813208 ) ) ;
#64226=CARTESIAN_POINT ( 'NONE',  ( -142.0902782307735492, 58.13494170556000995, -43.45927447690819179 ) ) ;
#64227=EDGE_LOOP ( 'NONE', ( #1155, #45656 ) ) ;
#64228=CARTESIAN_POINT ( 'NONE',  ( 55.57634120535662703, 12.09544293553732608, 11.45258174193541656 ) ) ;
#64234=CARTESIAN_POINT ( 'NONE',  ( 15.78827728214693416, -170.0000000000000000, 64.35925826316893961 ) ) ;
#64236=VECTOR ( 'NONE', #54839, 1000.000000000000000 ) ;
#64237=CARTESIAN_POINT ( 'NONE',  ( 83.60262962804351616, 18.41036205028015615, -23.34340396361722725 ) ) ;
#64239=CARTESIAN_POINT ( 'NONE',  ( 63.01563776193091826, -170.0000000000000000, -35.72069083216973695 ) ) ;
#64240=CARTESIAN_POINT ( 'NONE',  ( -94.88380767928866533, 29.17964217339915933, 12.44389626902909640 ) ) ;
#64241=CARTESIAN_POINT ( 'NONE',  ( -95.61819996182568104, 29.52346081122274768, -65.90474338168506563 ) ) ;
#64246=CARTESIAN_POINT ( 'NONE',  ( 181.9295719569813912, 79.46350097013163349, -78.03405158388139284 ) ) ;
#64249=CARTESIAN_POINT ( 'NONE',  ( -168.7150276173047700, 82.35404041280327192, -36.12430427854839365 ) ) ;
#64251=CARTESIAN_POINT ( 'NONE',  ( 106.0228389049370463, 28.07756796303167945, -76.47167350182498069 ) ) ;
#64252=CARTESIAN_POINT ( 'NONE',  ( -76.79042791651913547, 22.68960395613480685, 45.18370245349827741 ) ) ;
#64253=CARTESIAN_POINT ( 'NONE',  ( 82.95057496836383848, 18.19812356106674400, 43.76578103429130806 ) ) ;
#64254=CARTESIAN_POINT ( 'NONE',  ( 64.94098077424388293, 14.16208887966256924, -50.48552314904699756 ) ) ;
#64255=CARTESIAN_POINT ( 'NONE',  ( 40.38132770291767315, 9.553709436640060559, -35.66812004169860018 ) ) ;
#64256=CARTESIAN_POINT ( 'NONE',  ( 212.0180052085437694, 116.9552462415715439, 65.21599223484632546 ) ) ;
#64260=CARTESIAN_POINT ( 'NONE',  ( -13.47230132170245653, 7.324574289401434513, -37.95804552296768719 ) ) ;
#64261=CARTESIAN_POINT ( 'NONE',  ( -85.14310402784583687, 24.89513709528457142, 87.81192798829980006 ) ) ;
#64262=CARTESIAN_POINT ( 'NONE',  ( 88.52077179907880122, 21.14145351760140912, 71.31817190172689891 ) ) ;
#64263=CARTESIAN_POINT ( 'NONE',  ( 150.0973882686025149, 52.13852366454153042, -15.37827118707424567 ) ) ;
#64264=CARTESIAN_POINT ( 'NONE',  ( 33.44035656425386804, 8.720466003183661385, 15.14638828237973556 ) ) ;
#64265=CARTESIAN_POINT ( 'NONE',  ( 33.76124497394583557, 7.742545529019360551, -64.99726042931528980 ) ) ;
#64269=CARTESIAN_POINT ( 'NONE',  ( 211.1750821748527187, 115.6700317698878564, 86.59810276603568013 ) ) ;
#64270=LINE ( 'NONE', #16079, #46560 ) ;
#64273=CARTESIAN_POINT ( 'NONE',  ( 9.280894575734579988, 7.385644305345137717, -73.62443454551277000 ) ) ;
#64277=CARTESIAN_POINT ( 'NONE',  ( -3.252497086158843143, 6.636017118948017490, 31.65047178693046348 ) ) ;
#64278=CARTESIAN_POINT ( 'NONE',  ( -94.84390436305044148, 29.16104988397310649, -14.65970089395015208 ) ) ;
#64279=CARTESIAN_POINT ( 'NONE',  ( 79.68347087906724369, 18.21983559625775939, 93.81314209895157319 ) ) ;
#64284=CARTESIAN_POINT ( 'NONE',  ( -155.1359377029286293, 70.46175948311802983, 70.04776735375013175 ) ) ;
#64285=CARTESIAN_POINT ( 'NONE',  ( -132.6161619568759704, 51.08240647571221160, 7.939436356385802362 ) ) ;
#64286=CARTESIAN_POINT ( 'NONE',  ( -109.3585523124447860, 37.67345343047320227, 67.39597848995725826 ) ) ;
#64287=CARTESIAN_POINT ( 'NONE',  ( -180.4445711980297915, 95.66806589453305776, 93.66785953383893570 ) ) ;
#64292=CARTESIAN_POINT ( 'NONE',  ( 93.92280655489126673, 22.03989931749464404, 62.29064022871924777 ) ) ;
#64293=CARTESIAN_POINT ( 'NONE',  ( 197.5344630110112689, 98.61758706718745771, -19.22573370218078281 ) ) ;
#64295=CARTESIAN_POINT ( 'NONE',  ( 88.21404966472069020, 19.96646357304423347, -89.63590846026569636 ) ) ;
#64297=EDGE_LOOP ( 'NONE', ( #26223, #722 ) ) ;
#64299=CARTESIAN_POINT ( 'NONE',  ( 85.68197636629476222, 20.16141071296263831, 2.912210986997132878 ) ) ;
#64304=ORIENTED_EDGE ( 'NONE', *, *, #8248, .T. ) ;
#64305=CARTESIAN_POINT ( 'NONE',  ( 180.2565361171340612, 79.19912802278402353, 56.18695598174853956 ) ) ;
#64307=EDGE_LOOP ( 'NONE', ( #30592, #31874, #4110, #41269 ) ) ;
#64308=CARTESIAN_POINT ( 'NONE',  ( -76.10397364431024414, 21.36211154336728768, -22.82360444498405272 ) ) ;
#64311=CARTESIAN_POINT ( 'NONE',  ( 152.2924710224604894, 54.98503313872888754, 15.49619585574763647 ) ) ;
#64313=CARTESIAN_POINT ( 'NONE',  ( -173.9548930713591233, 88.06040582145364226, 30.85644618464981903 ) ) ;
#64320=CARTESIAN_POINT ( 'NONE',  ( -167.1534554062404254, 80.72263015867909530, 42.87160806905835386 ) ) ;
#64321=CARTESIAN_POINT ( 'NONE',  ( 126.3580464630938707, 38.22944795020838171, 63.55427522717772604 ) ) ;
#64324=ORIENTED_EDGE ( 'NONE', *, *, #21899, .F. ) ;
#64326=AXIS2_PLACEMENT_3D ( 'NONE', #69484, #64209, #15685 ) ;
#64327=CARTESIAN_POINT ( 'NONE',  ( -47.56977615209015653, 12.80198389319791019, 90.90604448902824686 ) ) ;
#64331=CARTESIAN_POINT ( 'NONE',  ( 68.80232419139076683, 14.08965771880099993, 86.21917338003288478 ) ) ;
#64333=CARTESIAN_POINT ( 'NONE',  ( -132.8123438040340147, 51.22132183644642112, 67.87186335099937651 ) ) ;
#64336=CARTESIAN_POINT ( 'NONE',  ( -96.46212652430689616, 31.03670207994726837, -91.46549339891737418 ) ) ;
#64338=CARTESIAN_POINT ( 'NONE',  ( -71.42007367207963853, 20.75704712149298103, 62.76318509112267918 ) ) ;
#64339=CARTESIAN_POINT ( 'NONE',  ( 188.4904153916303642, 86.42965364612514634, 35.58917660675626848 ) ) ;
#64340=CARTESIAN_POINT ( 'NONE',  ( 55.51597771111714508, 11.05737652677076355, -69.56553093680295774 ) ) ;
#64341=CARTESIAN_POINT ( 'NONE',  ( -35.82706824995756278, 10.35287135866583164, -90.42014361026066638 ) ) ;
#64342=FACE_OUTER_BOUND ( 'NONE', #33621, .T. ) ;
#64343=AXIS2_PLACEMENT_3D ( 'NONE', #32500, #36401, #58873 ) ;
#64344=CARTESIAN_POINT ( 'NONE',  ( 197.9740529046198390, 97.55632647424226889, 93.72595611219642819 ) ) ;
#64349=ORIENTED_EDGE ( 'NONE', *, *, #66343, .T. ) ;
#64351=CARTESIAN_POINT ( 'NONE',  ( -23.99957301099517437, 9.503061049698468210, -70.64423604567282666 ) ) ;
#64352=PLANE ( 'NONE',  #60260 ) ;
#64353=CARTESIAN_POINT ( 'NONE',  ( -24.70911172866235006, 8.583078995053028848, 61.21438271965689637 ) ) ;
#64354=CARTESIAN_POINT ( 'NONE',  ( -144.9439644317224349, 60.40328483334189968, 5.419750871863752373 ) ) ;
#64361=CARTESIAN_POINT ( 'NONE',  ( 56.53776994993149430, 11.26292242501182628, 67.94548126311852343 ) ) ;
#64362=EDGE_CURVE ( 'NONE', #36151, #43433, #42051, .T. ) ;
#64376=CARTESIAN_POINT ( 'NONE',  ( 18.05623392574862862, 7.590818816530167545, 84.04748085494549059 ) ) ;
#64381=CARTESIAN_POINT ( 'NONE',  ( 84.74140601443110654, 18.78541996275572146, 17.63000419208631087 ) ) ;
#64386=ORIENTED_EDGE ( 'NONE', *, *, #38935, .F. ) ;
#64390=CARTESIAN_POINT ( 'NONE',  ( -120.6420427933462065, 44.31795133507804252, 5.915438131401089095 ) ) ;
#64393=CARTESIAN_POINT ( 'NONE',  ( 126.5880720616305837, 37.20544379858412043, 65.72198726327758322 ) ) ;
#64395=B_SPLINE_CURVE_WITH_KNOTS ( 'NONE', 3,
 ( #50352, #23624, #45060, #61252, #13072, #57358, #21111, #15485, #15821, #47135, #52075, #67924, #25363, #26385, #31653, #25705, #68597, #3539, #36939, #35905, #4918, #58043, #30285, #36247, #68267, #47822, #69283, #46443, #42552, #19723, #10188, #41181, #8835, #14450, #20072, #53089, #37263, #15136, #30629, #51733, #57704, #9515, #46798, #20403 ),
 .UNSPECIFIED., .F., .F.,
 ( 4, 2, 2, 2, 2, 2, 2, 2, 2, 2, 2, 2, 2, 2, 2, 2, 2, 2, 2, 2, 2, 4 ),
 ( 0.02432640572110344665, 0.02583721026359363238, 0.02659261253483874432, 0.02734801480608385627, 0.02885881934857403852, 0.02961422161981911577, 0.03036962389106419302, 0.03188042843355437528, 0.03339123297604455753, 0.03414663524728962785, 0.03490203751853469816, 0.03641284206102485266, 0.03716824433226995766, 0.03792364660351505573, 0.03943445114600528656, 0.04094525568849551045, 0.04245606023098574822, 0.04396686477347597211, 0.04472226704472107711, 0.04547766931596618212, 0.04698847385845637825, 0.04849927840094656745 ),
 .UNSPECIFIED. ) ;
#64397=CARTESIAN_POINT ( 'NONE',  ( 150.2794558856211040, 52.26944788078747450, 39.10923047536901720 ) ) ;
#64403=CARTESIAN_POINT ( 'NONE',  ( -24.32937228292060539, 8.531905774118435204, 35.27833887421346759 ) ) ;
#64404=CARTESIAN_POINT ( 'NONE',  ( -142.0227972901369071, 59.36121938936274489, -69.71386678037109164 ) ) ;
#64409=ADVANCED_FACE ( 'NONE', ( #23216 ), #50625, .F. ) ;
#64410=DIRECTION ( 'NONE',  ( 0.000000000000000000, 0.000000000000000000, 1.000000000000000000 ) ) ;
#64411=CARTESIAN_POINT ( 'NONE',  ( -174.7817412490652487, 90.52199442492059234, 57.84031650591408180 ) ) ;
#64414=CARTESIAN_POINT ( 'NONE',  ( -85.64924756730680144, 26.19583280090850153, 8.325405162945308746 ) ) ;
#64417=CARTESIAN_POINT ( 'NONE',  ( -125.4463376280758951, 47.40387005565909817, -76.74829057748890193 ) ) ;
#64418=CARTESIAN_POINT ( 'NONE',  ( 70.51601918574516503, 14.53832276813546542, 10.70683331067295008 ) ) ;
#64419=CARTESIAN_POINT ( 'NONE',  ( 163.1265310614426767, 62.18610413911356005, 5.133598315962148106 ) ) ;
#64420=CARTESIAN_POINT ( 'NONE',  ( 92.20490818459946070, 22.47175429302964034, -11.43690497573547660 ) ) ;
#64422=VECTOR ( 'NONE', #44906, 1000.000000000000000 ) ;
#64423=CARTESIAN_POINT ( 'NONE',  ( -31.92572261726341054, 10.69135962481464119, 3.371903815725487252 ) ) ;
#64424=ORIENTED_EDGE ( 'NONE', *, *, #25831, .T. ) ;
#64426=VERTEX_POINT ( 'NONE', #29516 ) ;
#64427=CARTESIAN_POINT ( 'NONE',  ( 23.04797191264876233, 7.849755664016355716, -71.80966863344457352 ) ) ;
#64428=CARTESIAN_POINT ( 'NONE',  ( 102.8221746832285675, 26.69056128693217289, 89.65735780395625909 ) ) ;
#64429=CARTESIAN_POINT ( 'NONE',  ( -147.1538409485623049, 63.51600817366542628, 57.94073712792580011 ) ) ;
#64430=CARTESIAN_POINT ( 'NONE',  ( 63.50528314073025626, 12.78634332146812547, -8.876140241706053757 ) ) ;
#64431=CARTESIAN_POINT ( 'NONE',  ( -23.98747857548121942, 9.501432345103355104, -41.83194910379017273 ) ) ;
#64432=CARTESIAN_POINT ( 'NONE',  ( -52.45048892661850459, 15.03803514841137812, -62.52259457201746073 ) ) ;
#64439=VECTOR ( 'NONE', #44754, 1000.000000000000000 ) ;
#64440=CARTESIAN_POINT ( 'NONE',  ( 38.42095780754793566, 9.297684251045556181, 71.71026093375481025 ) ) ;
#64441=CARTESIAN_POINT ( 'NONE',  ( 173.7124655175693988, 72.83929305610512017, 89.05859609801423460 ) ) ;
#64446=CARTESIAN_POINT ( 'NONE',  ( 93.32756701508621688, 22.89083686918419502, 13.77822573322123212 ) ) ;
#64447=B_SPLINE_CURVE_WITH_KNOTS ( 'NONE', 3,
 ( #16602, #5697, #6042, #53184, #5013, #26821, #21531, #27855, #54580, #27501, #10628, #782, #38407, #22234, #33144, #43674, #32100, #65150, #59851, #6405, #49298, #38771, #53536, #26479, #47915, #37358, #21201, #7806, #34197, #2523, #7464, #23297, #17661, #18008, #2869, #6750, #65866, #44377, #66908, #29589, #66221, #8145, #39458, #2185, #34551 ),
 .UNSPECIFIED., .F., .F.,
 ( 4, 2, 2, 2, 2, 2, 2, 2, 1, 2, 2, 2, 2, 2, 2, 2, 2, 2, 2, 2, 2, 2, 4 ),
 ( 1.734723475976807094E-18, 0.001467747071934203101, 0.002201620607901302266, 0.002935494143868401865, 0.004403241215802589786, 0.005870988287736776841, 0.007338735359670963895, 0.008072608895638043111, 0.008806482431605120592, 0.009540355967572199808, 0.01027422950353927902, 0.01174197657547347388, 0.01247585011144059300, 0.01320972364740771211, 0.01467747071934199198, 0.01541134425530912150, 0.01614521779127624929, 0.01761296486321049098, 0.01908071193514473962, 0.01981458547111185353, 0.02054845900707896050, 0.02201620607901318138, 0.02348395315094738839 ),
 .UNSPECIFIED. ) ;
#64448=CARTESIAN_POINT ( 'NONE',  ( 188.2962140587030149, 87.71627202537837320, -18.95942837431084627 ) ) ;
#64451=CARTESIAN_POINT ( 'NONE',  ( 86.62931800182293784, -170.0000000000000000, 17.86753698201564688 ) ) ;
#64452=CARTESIAN_POINT ( 'NONE',  ( 46.13856685535756696, 9.381502944822520007, -12.94178744436969275 ) ) ;
#64456=CARTESIAN_POINT ( 'NONE',  ( 164.1352994389932007, 64.33767534192695337, 60.30451892934298286 ) ) ;
#64460=CARTESIAN_POINT ( 'NONE',  ( 94.02861641584115659, 23.15570573563315904, -44.57244623153589203 ) ) ;
#64463=CARTESIAN_POINT ( 'NONE',  ( 155.7262569076171701, 56.30477153194512852, 17.41501643175935143 ) ) ;
#64464=CARTESIAN_POINT ( 'NONE',  ( -15.22837983954869223, 8.497513067427652445, 92.55061580248207065 ) ) ;
#64467=ADVANCED_FACE ( 'NONE', ( #17579 ), #39044, .T. ) ;
#64469=CARTESIAN_POINT ( 'NONE',  ( -56.02027488966933078, 14.94257193099085690, 72.11473951196722965 ) ) ;
#64471=EDGE_CURVE ( 'NONE', #57040, #64426, #41319, .T. ) ;
#64472=EDGE_LOOP ( 'NONE', ( #1601, #42692 ) ) ;
#64475=CARTESIAN_POINT ( 'NONE',  ( 107.9301116202191650, 27.82606182274594886, 29.96094684213162651 ) ) ;
#64478=CARTESIAN_POINT ( 'NONE',  ( -61.51762070241280611, 16.51067482779404116, -65.75066130139710197 ) ) ;
#64480=B_SPLINE_CURVE_WITH_KNOTS ( 'NONE', 3,
 ( #39264, #62361, #62714, #24738, #46874, #56741, #38919, #68338, #12524, #28711, #9243, #14516, #30010, #66013, #19442, #25084, #1985, #55073, #46173, #14175, #23084, #50157, #67312, #45836, #17810, #19098, #8558, #3614, #3967, #35638, #25436, #57089, #8901, #12182, #60366, #30353, #67997, #67646 ),
 .UNSPECIFIED., .F., .F.,
 ( 4, 2, 2, 2, 2, 2, 2, 2, 2, 2, 2, 2, 2, 2, 2, 2, 2, 2, 4 ),
 ( 1.430489624538199204E-17, 0.003908178031105504456, 0.005862267046658207678, 0.007816356062210911768, 0.009770445077763615857, 0.01172453409331631821, 0.01270157860109266158, 0.01367862310886900669, 0.01465566761664534833, 0.01563271212442169170, 0.01660975663219803680, 0.01758680113997438191, 0.01954089015552706865, 0.02051793466330342069, 0.02149497917107977274, 0.02344906818663248030, 0.02540315720218519133, 0.02735724621773790582, 0.03126542424884329319 ),
 .UNSPECIFIED. ) ;
#64481=CARTESIAN_POINT ( 'NONE',  ( -3.862560291631540021, 7.672660553664875316, 4.398781296712932942 ) ) ;
#64483=CARTESIAN_POINT ( 'NONE',  ( 164.7598791907599320, 63.54825436415271867, 92.40245794402351009 ) ) ;
#64487=ORIENTED_EDGE ( 'NONE', *, *, #6081, .F. ) ;
#64489=CARTESIAN_POINT ( 'NONE',  ( -48.23389383802710739, 13.99288361739331599, -45.84916994387870659 ) ) ;
#64492=CARTESIAN_POINT ( 'NONE',  ( 8.763528846667103522, 7.383598436776580343, 40.15354979696406446 ) ) ;
#64494=CARTESIAN_POINT ( 'NONE',  ( -82.76871759908607373, 25.01134596399992205, 85.32081939002443960 ) ) ;
#64495=FACE_OUTER_BOUND ( 'NONE', #48090, .T. ) ;
#64499=EDGE_CURVE ( 'NONE', #30746, #8782, #63115, .T. ) ;
#64502=CARTESIAN_POINT ( 'NONE',  ( -51.77439426130687394, 13.82695438436703306, 44.56726461004345197 ) ) ;
#64505=EDGE_CURVE ( 'NONE', #8018, #8573, #34611, .T. ) ;
#64506=CARTESIAN_POINT ( 'NONE',  ( -60.95805269991215880, 17.39401718769326521, -47.34644918853374662 ) ) ;
#64507=DIRECTION ( 'NONE',  ( -0.000000000000000000, 1.000000000000000000, -0.000000000000000000 ) ) ;
#64508=CARTESIAN_POINT ( 'NONE',  ( 151.3309484205705360, 53.03078371058071383, -66.15348108964258245 ) ) ;
#64511=CARTESIAN_POINT ( 'NONE',  ( -157.0077369422018023, 70.81157624963286423, -42.59393186173343082 ) ) ;
#64513=VERTEX_POINT ( 'NONE', #54410 ) ;
#64514=CARTESIAN_POINT ( 'NONE',  ( 65.62985354949972816, 14.32996029952553663, -9.342276637876624434 ) ) ;
#64516=CARTESIAN_POINT ( 'NONE',  ( -24.69013852392472685, 9.595969721133672081, 88.11818326750967856 ) ) ;
#64517=CARTESIAN_POINT ( 'NONE',  ( -149.9471644042847345, 65.87751327280743396, 3.885972380641331547 ) ) ;
#64518=CARTESIAN_POINT ( 'NONE',  ( 187.9007786055418308, 85.78077355327275200, -40.58561043776339261 ) ) ;
#64519=CARTESIAN_POINT ( 'NONE',  ( 19.75784582661441391, 6.660183274347810212, 43.88284034533711520 ) ) ;
#64520=CARTESIAN_POINT ( 'NONE',  ( -149.0793230056187042, 65.13495668545753858, 84.40313663166193692 ) ) ;
#64525=CARTESIAN_POINT ( 'NONE',  ( -14.19447842053094000, 7.389800932646227949, 14.73911132003235736 ) ) ;
#64532=CARTESIAN_POINT ( 'NONE',  ( 187.2296622856350723, 86.53808614709454616, 59.34610297735440554 ) ) ;
#64533=CARTESIAN_POINT ( 'NONE',  ( -154.0718453320784249, 68.14976693162388699, 59.10962140803805198 ) ) ;
#64534=CARTESIAN_POINT ( 'NONE',  ( 22.15943197741200166, 7.796127622097902332, 6.705548799778502378 ) ) ;
#64539=CARTESIAN_POINT ( 'NONE',  ( 20.36314374176838271, 6.689939636827347158, 58.39567505551136861 ) ) ;
#64541=CARTESIAN_POINT ( 'NONE',  ( 12.69192874957003703, 6.421326776602846564, -76.69892586780029831 ) ) ;
#64548=CARTESIAN_POINT ( 'NONE',  ( 173.5837434292114096, 71.34409607026157119, 36.52054170544656841 ) ) ;
#64549=CARTESIAN_POINT ( 'NONE',  ( -133.3958821919892728, 51.63629593114585958, -42.92790141718640484 ) ) ;
#64550=CARTESIAN_POINT ( 'NONE',  ( 46.76970822239468362, 9.482505381172245507, -68.49923864311128341 ) ) ;
#64551=LINE ( 'NONE', #5797, #23166 ) ;
#64556=CARTESIAN_POINT ( 'NONE',  ( 199.9103251464699724, 101.6434290204575746, 15.64108102732007488 ) ) ;
#64557=ORIENTED_EDGE ( 'NONE', *, *, #18430, .F. ) ;
#64558=ORIENTED_EDGE ( 'NONE', *, *, #47020, .T. ) ;
#64561=ORIENTED_EDGE ( 'NONE', *, *, #55107, .T. ) ;
#64562=CARTESIAN_POINT ( 'NONE',  ( 111.1829448509513441, 30.43012797723692486, 71.41128605587280731 ) ) ;
#64563=CARTESIAN_POINT ( 'NONE',  ( 103.1664446665382826, 26.83710903202776166, -94.59076984783679620 ) ) ;
#64566=CARTESIAN_POINT ( 'NONE',  ( 110.2429982417149574, 29.99119854320845846, -77.76698815611739235 ) ) ;
#64567=EDGE_CURVE ( 'NONE', #5410, #12998, #45264, .T. ) ;
#64568=CARTESIAN_POINT ( 'NONE',  ( 85.05122279459726542, 18.88829753553988411, -89.66790706224459484 ) ) ;
#64570=CARTESIAN_POINT ( 'NONE',  ( -55.05276343752908730, 15.72344139423347720, -8.371773407996169425 ) ) ;
#64576=CARTESIAN_POINT ( 'NONE',  ( -142.9756886485677398, 60.11539876121631920, -46.00802361820244357 ) ) ;
#64577=CARTESIAN_POINT ( 'NONE',  ( -168.1839487819771080, 83.25723186408070831, -63.40587985515518454 ) ) ;
#64579=CARTESIAN_POINT ( 'NONE',  ( -145.9095871962850026, 61.18682730038538864, -35.72809995561637919 ) ) ;
#64585=CARTESIAN_POINT ( 'NONE',  ( 56.67004931728209982, 12.31690113431407951, 94.99999999999866418 ) ) ;
#64590=CARTESIAN_POINT ( 'NONE',  ( 92.53566308513175898, 21.52138666710687076, -65.51745770271240588 ) ) ;
#64593=CARTESIAN_POINT ( 'NONE',  ( -99.11448999425215334, 31.20120877265619086, 4.359154089478449734 ) ) ;
#64594=CARTESIAN_POINT ( 'NONE',  ( -99.97541017369785266, 31.62502926470683917, -62.20652744093037256 ) ) ;
#64601=CARTESIAN_POINT ( 'NONE',  ( 104.7042813665017746, 27.49927371769996753, -65.18629986727883363 ) ) ;
#64602=CARTESIAN_POINT ( 'NONE',  ( -74.39861643904072253, 21.81123504700007132, -63.28798662571114164 ) ) ;
#64603=FACE_OUTER_BOUND ( 'NONE', #7723, .T. ) ;
#64604=CARTESIAN_POINT ( 'NONE',  ( 46.85361596800670725, 10.51535167202354337, -42.13511323660575414 ) ) ;
#64606=ORIENTED_EDGE ( 'NONE', *, *, #14912, .F. ) ;
#64607=CARTESIAN_POINT ( 'NONE',  ( -109.3553681454883844, 36.52260784104392854, -18.21015660155229199 ) ) ;
#64608=ORIENTED_EDGE ( 'NONE', *, *, #46058, .T. ) ;
#64609=CARTESIAN_POINT ( 'NONE',  ( -34.74312654625183683, 10.15703162223800327, 4.134442808324870988 ) ) ;
#64610=CARTESIAN_POINT ( 'NONE',  ( -85.64954339472194533, 25.10532946445850300, 94.41971732200894962 ) ) ;
#64611=CARTESIAN_POINT ( 'NONE',  ( 90.51709546286271291, 21.85407654229979713, 57.63841953243931471 ) ) ;
#64612=CARTESIAN_POINT ( 'NONE',  ( 151.7819978880463623, 53.35998893001566046, -21.67396922968716311 ) ) ;
#64620=ORIENTED_EDGE ( 'NONE', *, *, #19695, .F. ) ;
#64624=EDGE_CURVE ( 'NONE', #56740, #8018, #11865, .T. ) ;
#64625=CARTESIAN_POINT ( 'NONE',  ( 46.65860211212413589, 10.48377752989033951, -68.00529549296528842 ) ) ;
#64626=CARTESIAN_POINT ( 'NONE',  ( -2.355184675731021304, 6.596450510445358795, 32.47880294032771786 ) ) ;
#64629=CARTESIAN_POINT ( 'NONE',  ( 92.18267540243923008, 22.46369443246546638, 85.84941083122645011 ) ) ;
#64637=CARTESIAN_POINT ( 'NONE',  ( -167.0073208999199323, 82.02183861952782706, -46.56420129388767037 ) ) ;
#64639=CARTESIAN_POINT ( 'NONE',  ( -180.4401457064375904, 95.66269784892554640, 90.33214016306547478 ) ) ;
#64640=EDGE_LOOP ( 'NONE', ( #43249, #38272 ) ) ;
#64646=CARTESIAN_POINT ( 'NONE',  ( -157.0033029063690719, 70.80749022588149444, 92.34162853283143590 ) ) ;
#64650=CARTESIAN_POINT ( 'NONE',  ( 136.1081004736419686, 42.80058051492063953, 29.85254608541649191 ) ) ;
#64653=CARTESIAN_POINT ( 'NONE',  ( -7.825402957745083654, 6.891034867348165172, 56.96013162991089018 ) ) ;
#64654=EDGE_CURVE ( 'NONE', #49052, #60277, #40438, .T. ) ;
#64655=CARTESIAN_POINT ( 'NONE',  ( 160.4986104110022893, 61.33701824525266488, 16.93016324216665680 ) ) ;
#64656=CARTESIAN_POINT ( 'NONE',  ( 23.09119322872580682, 6.844329382916375160, -95.00000000000133582 ) ) ;
#64659=ORIENTED_EDGE ( 'NONE', *, *, #34581, .T. ) ;
#64660=CARTESIAN_POINT ( 'NONE',  ( -76.77329340382465261, 21.60914066444071935, -8.497956380613862493 ) ) ;
#64661=CARTESIAN_POINT ( 'NONE',  ( -59.94781924509481286, 16.04872117907065387, 43.50492361771002692 ) ) ;
#64662=CARTESIAN_POINT ( 'NONE',  ( 150.5538013146980347, 53.70974888488126453, 12.97725223995403709 ) ) ;
#64663=ORIENTED_EDGE ( 'NONE', *, *, #64995, .F. ) ;
#64664=CARTESIAN_POINT ( 'NONE',  ( -173.5394735271662512, 87.59446374803710000, 30.82169460664101734 ) ) ;
#64673=CARTESIAN_POINT ( 'NONE',  ( -180.5200658187031593, 97.35517482626555363, 37.05475405369923436 ) ) ;
#64674=CARTESIAN_POINT ( 'NONE',  ( 130.3281282802763315, 40.49854652972195623, 57.21990522415401159 ) ) ;
#64676=EDGE_LOOP ( 'NONE', ( #4094, #32244, #47286, #33865 ) ) ;
#64677=AXIS2_PLACEMENT_3D ( 'NONE', #33314, #43492, #48403 ) ;
#64680=CARTESIAN_POINT ( 'NONE',  ( -133.3122825023497171, 52.81354457049841500, -95.00000000000133582 ) ) ;
#64682=AXIS2_PLACEMENT_3D ( 'NONE', #10909, #53464, #4600 ) ;
#64684=CARTESIAN_POINT ( 'NONE',  ( 69.38689814754611973, 14.24120947374744794, 87.03124869162181199 ) ) ;
#64688=ORIENTED_EDGE ( 'NONE', *, *, #53799, .T. ) ;
#64691=ORIENTED_EDGE ( 'NONE', *, *, #22700, .F. ) ;
#64692=CYLINDRICAL_SURFACE ( 'NONE', #46455, 7.500000000000020428 ) ;
#64693=CARTESIAN_POINT ( 'NONE',  ( 211.3917124729450165, 115.9987099435923597, -67.27654017559783028 ) ) ;
#64695=CARTESIAN_POINT ( 'NONE',  ( -71.97434903038468690, 19.88430675376529777, 7.650924302885536044 ) ) ;
#64696=CARTESIAN_POINT ( 'NONE',  ( -36.50102476951193609, 10.47699908632348276, -90.95548803688076589 ) ) ;
#64697=DIRECTION ( 'NONE',  ( 1.000000000000000000, 0.000000000000000000, -0.000000000000000000 ) ) ;
#64698=CARTESIAN_POINT ( 'NONE',  ( 198.2682806192667329, 97.92400992302502516, 86.53030137829317425 ) ) ;
#64699=CARTESIAN_POINT ( 'NONE',  ( 160.4986104110022893, 61.33701824525265778, -63.60348852922437146 ) ) ;
#64702=CYLINDRICAL_SURFACE ( 'NONE', #68954, 7.500000000000013323 ) ;
#64703=ORIENTED_EDGE ( 'NONE', *, *, #54622, .F. ) ;
#64704=EDGE_LOOP ( 'NONE', ( #11567, #29113, #38617, #42457 ) ) ;
#64705=CARTESIAN_POINT ( 'NONE',  ( -81.00507684688699328, 23.22613445438386748, 45.04825155395133862 ) ) ;
#64708=CARTESIAN_POINT ( 'NONE',  ( 45.89268866913130296, 10.36133864615983136, 41.17961490824062309 ) ) ;
#64709=CARTESIAN_POINT ( 'NONE',  ( -25.98312968277007329, 8.759224980175247310, 59.40908211529054483 ) ) ;
#64715=CARTESIAN_POINT ( 'NONE',  ( -130.1938957973835329, 50.61368074696266461, 31.95741200596453879 ) ) ;
#64718=CARTESIAN_POINT ( 'NONE',  ( -149.5074843970971017, 65.50121172469319220, 30.72082123989904545 ) ) ;
#64719=CARTESIAN_POINT ( 'NONE',  ( 59.08638499266953659, 11.79550614876701431, 57.76452535348534667 ) ) ;
#64720=CARTESIAN_POINT ( 'NONE',  ( -4.502148936856958272, 7.704491846230413721, 71.20160539119055443 ) ) ;
#64721=PRODUCT_DEFINITION_SHAPE ( 'NONE', 'NONE',  #65913 ) ;
#64733=CARTESIAN_POINT ( 'NONE',  ( 136.3292018078238925, 42.93753790426541883, -77.45239417490056155 ) ) ;
#64734=CARTESIAN_POINT ( 'NONE',  ( 70.45466089417030275, 14.52203022703029589, 38.29938007412685153 ) ) ;
#64740=CARTESIAN_POINT ( 'NONE',  ( 80.72161230109723817, 17.48902961068031203, 5.720643767644356892 ) ) ;
#64747=CARTESIAN_POINT ( 'NONE',  ( 93.33480479917548678, 21.81892021443993102, 13.76463275447737900 ) ) ;
#64752=CARTESIAN_POINT ( 'NONE',  ( 154.0293889979057269, 55.02370422818218287, 30.22901195537932395 ) ) ;
#64756=DIRECTION ( 'NONE',  ( -1.000000000000000000, 0.000000000000000000, 0.000000000000000000 ) ) ;
#64757=CARTESIAN_POINT ( 'NONE',  ( 134.7720294983483029, 43.15885542353190374, -62.91010168338426212 ) ) ;
#64758=CARTESIAN_POINT ( 'NONE',  ( -142.5042386072304055, 59.74110826975216071, -71.89443917550980245 ) ) ;
#64760=FACE_BOUND ( 'NONE', #17765, .T. ) ;
#64762=CARTESIAN_POINT ( 'NONE',  ( -178.5750994113944614, 94.98114813978521909, 59.99381261644018792 ) ) ;
#64766=CARTESIAN_POINT ( 'NONE',  ( -82.33596576276350731, 24.83688096733768091, 17.63268983951130764 ) ) ;
#64770=CARTESIAN_POINT ( 'NONE',  ( 68.45098769362925850, 13.99935947269948322, 5.294787831159208480 ) ) ;
#64771=CARTESIAN_POINT ( 'NONE',  ( -84.23336401058607237, 25.60798568215574988, 69.81228689596302672 ) ) ;
#64772=CARTESIAN_POINT ( 'NONE',  ( 88.28889510440060917, 21.05995314109334160, -9.159055693011952215 ) ) ;
#64774=CARTESIAN_POINT ( 'NONE',  ( -34.74563762132952149, 11.17960945723138266, 17.60810679087929032 ) ) ;
#64775=ORIENTED_EDGE ( 'NONE', *, *, #21591, .T. ) ;
#64776=CARTESIAN_POINT ( 'NONE',  ( 107.9362503323352627, 27.82881837607799369, -63.11455838136814833 ) ) ;
#64777=EDGE_LOOP ( 'NONE', ( #69184, #62980, #61389, #53494 ) ) ;
#64780=CARTESIAN_POINT ( 'NONE',  ( 104.5269485123011606, 27.42246137840687936, 85.93290527890958685 ) ) ;
#64781=DIRECTION ( 'NONE',  ( 0.000000000000000000, 0.000000000000000000, 1.000000000000000000 ) ) ;
#64782=CARTESIAN_POINT ( 'NONE',  ( 70.02892116572941461, 14.40944430928136732, -13.70672517636600141 ) ) ;
#64783=CARTESIAN_POINT ( 'NONE',  ( -24.61094659556677300, 9.585225265507405723, -39.70484628576755881 ) ) ;
#64784=AXIS2_PLACEMENT_3D ( 'NONE', #5714, #442, #21893 ) ;
#64785=CARTESIAN_POINT ( 'NONE',  ( 211.2559569222079574, 117.6288368612911768, -93.86917793742070160 ) ) ;
#64787=LINE ( 'NONE', #6736, #67927 ) ;
#64788=CARTESIAN_POINT ( 'NONE',  ( -124.9970785861867881, 47.10847819093959288, -23.01876740222969175 ) ) ;
#64792=CARTESIAN_POINT ( 'NONE',  ( 31.95163392065795449, 8.568192436298476267, 63.26676829875925279 ) ) ;
#64793=EDGE_CURVE ( 'NONE', #16235, #40950, #24515, .T. ) ;
#64802=CARTESIAN_POINT ( 'NONE',  ( 187.6511924654682559, 87.00187850361886888, -20.51322464869038242 ) ) ;
#64803=CARTESIAN_POINT ( 'NONE',  ( 212.1978255065451151, 119.0880569674902745, 10.21206011236483135 ) ) ;
#64806=CARTESIAN_POINT ( 'NONE',  ( 45.90128843543705273, 9.343910238294480308, -20.05022534619617858 ) ) ;
#64807=CARTESIAN_POINT ( 'NONE',  ( 209.9944361927105092, 113.8994774711241433, -22.29641758310334865 ) ) ;
#64809=CARTESIAN_POINT ( 'NONE',  ( 164.9706294237033717, 65.04392654036657007, 63.47989634801044900 ) ) ;
#64811=ORIENTED_EDGE ( 'NONE', *, *, #52860, .T. ) ;
#64813=CARTESIAN_POINT ( 'NONE',  ( 94.11595392909980262, 23.18887043179186946, -42.80727100288617493 ) ) ;
#64819=CARTESIAN_POINT ( 'NONE',  ( -1.679734956245725552, 7.575464525743545785, 86.95611724131752851 ) ) ;
#64823=ORIENTED_EDGE ( 'NONE', *, *, #32737, .F. ) ;
#64828=CARTESIAN_POINT ( 'NONE',  ( 104.3805245147141818, 26.26278144139197579, 32.40695671971902669 ) ) ;
#64831=CARTESIAN_POINT ( 'NONE',  ( -60.13226458141420494, 16.10241298991027392, -64.03742039381080531 ) ) ;
#64832=CARTESIAN_POINT ( 'NONE',  ( 33.03722315490661998, 7.666819786578624729, -12.30021257897310605 ) ) ;
#64834=CARTESIAN_POINT ( 'NONE',  ( -157.0079874970173819, 72.18249880494042259, -68.88373919596408257 ) ) ;
#64839=CARTESIAN_POINT ( 'NONE',  ( -47.56466076048273095, 13.83435953640667471, -43.20715939977046816 ) ) ;
#64841=CYLINDRICAL_SURFACE ( 'NONE', #20188, 7.500000000000013323 ) ;
#64842=CARTESIAN_POINT ( 'NONE',  ( 8.480977594057447888, 7.382886909400593112, 35.80792500536700373 ) ) ;
#64844=CARTESIAN_POINT ( 'NONE',  ( 79.37480438318435461, 17.07199765243625578, 92.83494011833366244 ) ) ;
#64846=EDGE_LOOP ( 'NONE', ( #53404, #30204 ) ) ;
#64848=ORIENTED_EDGE ( 'NONE', *, *, #61099, .F. ) ;
#64849=CARTESIAN_POINT ( 'NONE',  ( -8.811275908848678284, 6.956777180392054838, -23.52454203392342791 ) ) ;
#64850=CARTESIAN_POINT ( 'NONE',  ( -169.3240414452573930, 84.46994553661198779, 85.51843480329762315 ) ) ;
#64851=CARTESIAN_POINT ( 'NONE',  ( -54.57280099357649306, 14.55288945003961487, -23.37177340799619785 ) ) ;
#64854=CARTESIAN_POINT ( 'NONE',  ( -57.65574514524056582, 16.43983577669855833, -49.75425646672815105 ) ) ;
#64855=CARTESIAN_POINT ( 'NONE',  ( -8.314488422519708877, 7.931352979988702145, -23.57352014148016650 ) ) ;
#64856=CARTESIAN_POINT ( 'NONE',  ( 154.6667526376337207, 55.50347409140650257, -63.50879352240995956 ) ) ;
#64857=CARTESIAN_POINT ( 'NONE',  ( 18.21423326326597802, 6.590134686181415624, -9.060803352357556406 ) ) ;
#64859=EDGE_LOOP ( 'NONE', ( #39798, #20137, #60189, #60691 ) ) ;
#64863=CARTESIAN_POINT ( 'NONE',  ( -145.3233446620410518, 62.00659513626053609, 17.61759092328014731 ) ) ;
#64864=CARTESIAN_POINT ( 'NONE',  ( -59.45661995832976032, 16.95372133001488990, -90.31914386384646320 ) ) ;
#64866=CARTESIAN_POINT ( 'NONE',  ( -156.6862310659955426, 71.88416263379563986, 13.61984221008611584 ) ) ;
#64869=CARTESIAN_POINT ( 'NONE',  ( 16.28371206594635012, 6.516665886438622657, 45.01470767270525641 ) ) ;
#64870=CARTESIAN_POINT ( 'NONE',  ( 157.4703587214989113, 58.92748579479258808, -77.96873488960135035 ) ) ;
#64872=EDGE_CURVE ( 'NONE', #40691, #15039, #27254, .T. ) ;
#64874=ORIENTED_EDGE ( 'NONE', *, *, #46058, .F. ) ;
#64878=CARTESIAN_POINT ( 'NONE',  ( -156.9900125991010214, 72.16580261738673130, -16.05494244269402060 ) ) ;
#64879=CARTESIAN_POINT ( 'NONE',  ( 33.93974911725172916, 8.773765372885550917, -48.26511037450102037 ) ) ;
#64880=EDGE_CURVE ( 'NONE', #37023, #6692, #15148, .T. ) ;
#64885=VECTOR ( 'NONE', #47182, 1000.000000000000000 ) ;
#64887=CARTESIAN_POINT ( 'NONE',  ( -154.2585856850056132, 68.31650218414625897, 59.25724188130881487 ) ) ;
#64894=CARTESIAN_POINT ( 'NONE',  ( 15.29293866748104413, 6.484959508098438796, -62.36349468914947636 ) ) ;
#64896=ORIENTED_EDGE ( 'NONE', *, *, #61956, .F. ) ;
#64899=CARTESIAN_POINT ( 'NONE',  ( -128.7650348665117122, 48.41336321950709731, -62.32582547038258269 ) ) ;
#64902=CARTESIAN_POINT ( 'NONE',  ( 41.35041461497707616, 8.670465437677179921, -62.70515334933006102 ) ) ;
#64903=ADVANCED_FACE ( 'NONE', ( #39221 ), #1575, .F. ) ;
#64904=CARTESIAN_POINT ( 'NONE',  ( 57.07246224906423038, 12.39953617563782906, -65.46404872146828779 ) ) ;
#64909=CARTESIAN_POINT ( 'NONE',  ( -23.93880457192868505, 8.479983864459171627, -15.73297272197446439 ) ) ;
#64910=CARTESIAN_POINT ( 'NONE',  ( 176.7661391921448057, 74.34902671065451329, 84.35726248129530802 ) ) ;
#64912=ORIENTED_EDGE ( 'NONE', *, *, #18828, .F. ) ;
#64913=CARTESIAN_POINT ( 'NONE',  ( 183.7875981612219789, 82.83906702837187197, 43.80766194854361828 ) ) ;
#64916=CARTESIAN_POINT ( 'NONE',  ( 117.4711568421290195, 33.49899443629672646, 66.02157968639461672 ) ) ;
#64917=CARTESIAN_POINT ( 'NONE',  ( 137.3861614007145135, 44.78548268714475711, 70.47665649296068580 ) ) ;
#64918=FACE_OUTER_BOUND ( 'NONE', #64307, .T. ) ;
#64919=CARTESIAN_POINT ( 'NONE',  ( 81.99350056087827454, 17.89100316059847273, -91.11151605743467030 ) ) ;
#64921=CARTESIAN_POINT ( 'NONE',  ( -189.2826425734429563, 107.1493800926105990, 39.29612140121835040 ) ) ;
#64923=ORIENTED_EDGE ( 'NONE', *, *, #1745, .F. ) ;
#64924=ORIENTED_EDGE ( 'NONE', *, *, #47399, .T. ) ;
#64926=VECTOR ( 'NONE', #12121, 1000.000000000000000 ) ;
#64929=CARTESIAN_POINT ( 'NONE',  ( -147.7925265216585160, 64.04960911618972830, -49.61744604605377873 ) ) ;
#64931=CARTESIAN_POINT ( 'NONE',  ( -166.0012244511291328, 80.97916541034754800, -71.43140414274201078 ) ) ;
#64932=CARTESIAN_POINT ( 'NONE',  ( -148.4259959918497032, 63.26767374754761875, -34.88804037928592550 ) ) ;
#64933=ORIENTED_EDGE ( 'NONE', *, *, #27065, .T. ) ;
#64937=CARTESIAN_POINT ( 'NONE',  ( -130.2196570250629009, 49.40815211106351512, 31.97506308841684941 ) ) ;
#64940=CARTESIAN_POINT ( 'NONE',  ( 87.10672734544988316, 20.64813880796636880, 29.71208757247930521 ) ) ;
#64941=CARTESIAN_POINT ( 'NONE',  ( 81.03898448521320574, 17.58847173596441493, -21.50135784270763040 ) ) ;
#64944=EDGE_CURVE ( 'NONE', #61225, #35602, #33251, .T. ) ;
#64945=CARTESIAN_POINT ( 'NONE',  ( 200.8410151090926377, 101.2014854111317561, 16.30994292411162050 ) ) ;
#64946=CARTESIAN_POINT ( 'NONE',  ( -94.84390436305042726, 29.16104988397310649, 12.18484969651350447 ) ) ;
#64947=CARTESIAN_POINT ( 'NONE',  ( -95.86612279493097333, 29.64021615886203875, -65.46366992558145625 ) ) ;
#64948=VERTEX_POINT ( 'NONE', #61017 ) ;
#64949=ORIENTED_EDGE ( 'NONE', *, *, #27003, .T. ) ;
#64950=CARTESIAN_POINT ( 'NONE',  ( 46.70715146412976537, 9.472433765546997009, 35.69789323664132752 ) ) ;
#64955=CARTESIAN_POINT ( 'NONE',  ( -190.6985136298601731, 109.1272424661242582, -95.00000000000133582 ) ) ;
#64957=CARTESIAN_POINT ( 'NONE',  ( -123.6618353044034535, 46.23845779494349273, 30.94497602649078516 ) ) ;
#64958=CARTESIAN_POINT ( 'NONE',  ( 211.3917124729450165, 115.9987099435923170, 66.94621277672065673 ) ) ;
#64961=CARTESIAN_POINT ( 'NONE',  ( -24.71604178686819608, 9.599501655372943532, 7.538451900758993851 ) ) ;
#64963=CARTESIAN_POINT ( 'NONE',  ( -35.99432170610150195, 10.38324794858010414, 4.893849840022852504 ) ) ;
#64966=CARTESIAN_POINT ( 'NONE',  ( 94.02499804464930833, 23.15433260743125743, 65.32863951667292213 ) ) ;
#64967=CARTESIAN_POINT ( 'NONE',  ( 150.4544126017350720, 52.39556706174412426, -19.44410150025860773 ) ) ;
#64969=EDGE_CURVE ( 'NONE', #7307, #47821, #1065, .T. ) ;
#64970=CARTESIAN_POINT ( 'NONE',  ( -100.4347360276019430, 32.97716872911836106, -76.64346099625136333 ) ) ;
#64975=CARTESIAN_POINT ( 'NONE',  ( 55.91494169499917177, 12.16343363043255899, 66.58477365789052271 ) ) ;
#64977=CARTESIAN_POINT ( 'NONE',  ( -9.765753193741730342, 8.033970690975920093, 3.522221867868848388 ) ) ;
#64978=CARTESIAN_POINT ( 'NONE',  ( 41.80372346091803593, 9.750024116765242610, -62.85510525679180205 ) ) ;
#64979=CARTESIAN_POINT ( 'NONE',  ( -62.41990535723909517, 16.78139727964023109, -95.00000000000133582 ) ) ;
#64982=CARTESIAN_POINT ( 'NONE',  ( 79.79351097043134189, 18.25397826796971756, 87.79632269537491140 ) ) ;
#64990=VECTOR ( 'NONE', #36578, 1000.000000000000000 ) ;
#64991=CARTESIAN_POINT ( 'NONE',  ( -129.6079169496900931, 50.20899308323958365, -35.89371998164833144 ) ) ;
#64992=ORIENTED_EDGE ( 'NONE', *, *, #23312, .T. ) ;
#64995=EDGE_CURVE ( 'NONE', #14111, #27023, #53191, .T. ) ;
#64996=CARTESIAN_POINT ( 'NONE',  ( 198.2581645178918563, 99.52881771501678543, -13.12609424774730371 ) ) ;
#64997=CARTESIAN_POINT ( 'NONE',  ( -144.0355355870767653, 59.67305119280410963, 86.74176708214653786 ) ) ;
#64999=ORIENTED_EDGE ( 'NONE', *, *, #42565, .F. ) ;
#65001=CARTESIAN_POINT ( 'NONE',  ( 84.72546926745364715, 19.84015517905186243, 17.63786239785293830 ) ) ;
#65003=CARTESIAN_POINT ( 'NONE',  ( -94.83091526606384036, 30.26550147229323784, 37.00308990492074201 ) ) ;
#65007=ORIENTED_EDGE ( 'NONE', *, *, #42849, .T. ) ;
#65009=CARTESIAN_POINT ( 'NONE',  ( -71.56718866013693514, 19.74312628447963647, -13.29964426657915766 ) ) ;
#65011=CARTESIAN_POINT ( 'NONE',  ( 152.1153500913667358, 54.85403770686895086, 15.32190511181030601 ) ) ;
#65012=ORIENTED_EDGE ( 'NONE', *, *, #40876, .F. ) ;
#65013=CARTESIAN_POINT ( 'NONE',  ( -173.1211646369891355, 87.12891641440857882, 30.82169460664101734 ) ) ;
#65017=CARTESIAN_POINT ( 'NONE',  ( -142.0747101610765242, 59.40211529287933701, -95.00000000000133582 ) ) ;
#65018=ADVANCED_FACE ( 'NONE', ( #55741 ), #56427, .F. ) ;
#65019=CARTESIAN_POINT ( 'NONE',  ( -32.41982179707235900, 9.753975577087185656, -23.42419288917794873 ) ) ;
#65021=CARTESIAN_POINT ( 'NONE',  ( -180.0154536325056824, 96.73346874014735874, 41.28871520911766879 ) ) ;
#65022=CARTESIAN_POINT ( 'NONE',  ( 129.1310456962234809, 39.80382822048402147, 58.01066127129433880 ) ) ;
#65028=CARTESIAN_POINT ( 'NONE',  ( -48.26386693105755654, 12.96570170253255405, 94.71075846305346602 ) ) ;
#65030=CARTESIAN_POINT ( 'NONE',  ( 69.54076065159397047, 14.28133484589228175, 94.71504016972204454 ) ) ;
#65032=CARTESIAN_POINT ( 'NONE',  ( -126.8005235842505840, 47.09307471149450919, 72.42308343011845295 ) ) ;
#65033=CARTESIAN_POINT ( 'NONE',  ( -55.70897216137028352, 15.90023021009871407, 84.00879926019972288 ) ) ;
#65036=CARTESIAN_POINT ( 'NONE',  ( -98.45346891396377487, 31.99841271297070122, -89.74978154278917941 ) ) ;
#65037=ORIENTED_EDGE ( 'NONE', *, *, #22700, .T. ) ;
#65038=DIRECTION ( 'NONE',  ( -0.000000000000000000, 1.000000000000000000, -0.000000000000000000 ) ) ;
#65040=CARTESIAN_POINT ( 'NONE',  ( 209.5118425285948547, 113.1852661712287329, -64.91501104591304738 ) ) ;
#65043=DIRECTION ( 'NONE',  ( -0.000000000000000000, 1.000000000000000000, -0.000000000000000000 ) ) ;
#65044=CARTESIAN_POINT ( 'NONE',  ( -124.9915686518654638, 47.10215472274616388, 72.46449846362082781 ) ) ;
#65045=CARTESIAN_POINT ( 'NONE',  ( 22.51849650178395379, 7.817407610814553820, 40.83350911454274268 ) ) ;
#65048=CARTESIAN_POINT ( 'NONE',  ( 163.7379901688712778, 64.00402364591249693, -66.34155096030688981 ) ) ;
#65056=CARTESIAN_POINT ( 'NONE',  ( -83.69653436244855982, 24.30167057287991028, 43.48670558365605388 ) ) ;
#65058=CARTESIAN_POINT ( 'NONE',  ( 45.35621884287174765, 10.27694987765648627, 32.82727971635760866 ) ) ;
#65061=ORIENTED_EDGE ( 'NONE', *, *, #15906, .F. ) ;
#65066=CARTESIAN_POINT ( 'NONE',  ( 34.83823433017388282, 8.871835168107974567, -22.24740203346240719 ) ) ;
#65068=CARTESIAN_POINT ( 'NONE',  ( 59.29615173875418321, 11.84060224810188444, 57.64020183933660491 ) ) ;
#65069=CARTESIAN_POINT ( 'NONE',  ( -3.862560291631546239, 7.672660553664875316, 58.08788247764030643 ) ) ;
#65070=CARTESIAN_POINT ( 'NONE',  ( -31.43908319763710679, 10.61114334766713796, -89.00629854612920155 ) ) ;
#65073=CARTESIAN_POINT ( 'NONE',  ( -119.6995109608660925, 42.54844499216736153, -73.49440844546555240 ) ) ;
#65077=CARTESIAN_POINT ( 'NONE',  ( 159.2319614735955895, 59.03334608081208046, -24.08327306185856997 ) ) ;
#65080=CARTESIAN_POINT ( 'NONE',  ( 140.0614732283738988, 45.29930344725074320, -74.58837468684397720 ) ) ;
#65084=CARTESIAN_POINT ( 'NONE',  ( 81.03898448521321995, 17.58847173596441849, 5.343192747756050132 ) ) ;
#65086=CARTESIAN_POINT ( 'NONE',  ( -71.59086462055188349, 19.75139532313338364, 35.41821401656284962 ) ) ;
#65087=VERTEX_POINT ( 'NONE', #4010 ) ;
#65090=CYLINDRICAL_SURFACE ( 'NONE', #10580, 7.500000000000013323 ) ;
#65092=CARTESIAN_POINT ( 'NONE',  ( 86.62931800182293784, 19.42108912189598158, 2.867536982015618019 ) ) ;
#65093=EDGE_CURVE ( 'NONE', #48407, #11965, #52868, .T. ) ;
#65099=CARTESIAN_POINT ( 'NONE',  ( 31.91383250562745388, 8.564461488297011371, 37.90219752839882972 ) ) ;
#65100=CARTESIAN_POINT ( 'NONE',  ( 63.99027454648600610, 13.93445177372598742, 29.86079229877851660 ) ) ;
#65107=CARTESIAN_POINT ( 'NONE',  ( -148.6471085600699382, 64.76880961642447687, -76.62049576393286543 ) ) ;
#65112=FACE_BOUND ( 'NONE', #56953, .T. ) ;
#65113=CARTESIAN_POINT ( 'NONE',  ( -2.355184675731015975, 6.596450510445362347, -74.89939942152702201 ) ) ;
#65114=CARTESIAN_POINT ( 'NONE',  ( -174.7903139851459855, 90.53182997092834228, 72.49021236485279474 ) ) ;
#65115=CARTESIAN_POINT ( 'NONE',  ( 111.0232121500226299, 29.24301703641567229, -89.61153874658104712 ) ) ;
#65116=B_SPLINE_CURVE_WITH_KNOTS ( 'NONE', 3,
 ( #14761, #57683, #36913, #9493, #30951, #25683, #53405, #63980, #26698, #31976, #47112, #37238, #68576, #5240, #20377, #41846, #53063, #48131, #36571, #9839, #43809, #52725, #4551, #26016, #68904, #42184, #63652, #10167, #4892, #26359, #47795, #21083, #42527, #45217, #29057, #1977, #55781, #39258, #27989, #49433, #44526, #12175, #23076, #2320 ),
 .UNSPECIFIED., .F., .F.,
 ( 4, 2, 2, 2, 2, 2, 2, 2, 2, 2, 2, 2, 2, 2, 2, 2, 2, 2, 2, 2, 2, 4 ),
 ( 0.000000000000000000, 0.001472974678681650317, 0.002209462018022476885, 0.002945949357363303236, 0.004418924036044937290, 0.005891898714726570042, 0.007364873393408203663, 0.008101360732749023075, 0.008837848072089841620, 0.01031082275077147524, 0.01178379742945310713, 0.01252028476879392047, 0.01325677210813473554, 0.01472974678681636569, 0.01546623412615717556, 0.01620272146549799064, 0.01767569614417961732, 0.01914867082286124400, 0.01988515816220205387, 0.02062164550154286721, 0.02209462018022449042, 0.02356759485890611364 ),
 .UNSPECIFIED. ) ;
#65117=CARTESIAN_POINT ( 'NONE',  ( -120.5002574492099257, 44.22930148497321312, -37.19622962122973320 ) ) ;
#65118=CARTESIAN_POINT ( 'NONE',  ( -81.89510452344295288, 24.66033552777454574, 4.287486826232798975 ) ) ;
#65121=CARTESIAN_POINT ( 'NONE',  ( -71.28077210551055032, 19.64439276383075850, -95.00000000000133582 ) ) ;
#65124=CARTESIAN_POINT ( 'NONE',  ( 86.62931800182293784, 20.48449268398422518, -23.97701360844805407 ) ) ;
#65132=CARTESIAN_POINT ( 'NONE',  ( 108.0746788553144313, 28.99562660843912099, 83.61346235993913467 ) ) ;
#65133=LINE ( 'NONE', #16927, #61589 ) ;
#65134=CARTESIAN_POINT ( 'NONE',  ( 63.01563776193090405, 12.67277567978497643, -8.876140241706053757 ) ) ;
#65136=CARTESIAN_POINT ( 'NONE',  ( -25.07735481787161191, 9.648965052008776411, -46.79695794318186586 ) ) ;
#65137=CARTESIAN_POINT ( 'NONE',  ( -48.71337292867759317, 14.10768470390589435, -65.54550437577125876 ) ) ;
#65138=DIRECTION ( 'NONE',  ( 0.000000000000000000, -1.000000000000000000, 0.000000000000000000 ) ) ;
#65139=CARTESIAN_POINT ( 'NONE',  ( -120.6420427933462207, 44.31795133507804962, -20.92911245906258699 ) ) ;
#65142=CARTESIAN_POINT ( 'NONE',  ( 33.77444274891858811, 8.756048688386671941, 59.29431779835010730 ) ) ;
#65143=CARTESIAN_POINT ( 'NONE',  ( 181.0840389613909736, 78.60582251573003987, 56.15314469597509373 ) ) ;
#65144=CARTESIAN_POINT ( 'NONE',  ( -169.1116812882276577, 84.24296059722696839, 71.52038224641596287 ) ) ;
#65147=CARTESIAN_POINT ( 'NONE',  ( 62.53356220515464514, 13.59349015304565000, -23.87614024170608573 ) ) ;
#65148=ORIENTED_EDGE ( 'NONE', *, *, #29123, .T. ) ;
#65149=CARTESIAN_POINT ( 'NONE',  ( 93.08073375333745503, 22.79826000593201485, 6.534512623384266305 ) ) ;
#65150=CARTESIAN_POINT ( 'NONE',  ( -14.92903005859420951, 7.458185427130749723, 66.87855674452464427 ) ) ;
#65151=CARTESIAN_POINT ( 'NONE',  ( 212.0104729185450765, 118.7959000526602722, 11.55940993411821793 ) ) ;
#65153=CARTESIAN_POINT ( 'NONE',  ( 45.34143264614440483, 9.256465810451189213, -20.86148856102304094 ) ) ;
#65155=FACE_BOUND ( 'NONE', #61949, .T. ) ;
#65156=CARTESIAN_POINT ( 'NONE',  ( -55.05276343752909440, 14.68156374112638041, -35.21632399845986328 ) ) ;
#65159=DIRECTION ( 'NONE',  ( -0.000000000000000000, 1.000000000000000000, -0.000000000000000000 ) ) ;
#65160=CARTESIAN_POINT ( 'NONE',  ( 90.30732934992394689, 21.77797012484620964, -36.76760811582850863 ) ) ;
#65161=CARTESIAN_POINT ( 'NONE',  ( -55.05276343752909440, 15.72344139423348430, 57.16187836339483397 ) ) ;
#65163=CARTESIAN_POINT ( 'NONE',  ( 152.1327777395850660, 53.61712543276775023, 15.33955938004834607 ) ) ;
#65164=VECTOR ( 'NONE', #12103, 1000.000000000000000 ) ;
#65165=DIRECTION ( 'NONE',  ( -0.000000000000000000, 1.000000000000000000, -0.000000000000000000 ) ) ;
#65170=EDGE_LOOP ( 'NONE', ( #13625, #28731, #42637, #65479 ) ) ;
#65173=CARTESIAN_POINT ( 'NONE',  ( 39.40195752203892710, 8.409560354027393103, -62.46436805589144114 ) ) ;
#65174=CARTESIAN_POINT ( 'NONE',  ( 105.2506154496929298, 26.63995206619727796, 42.71361730424104053 ) ) ;
#65177=CARTESIAN_POINT ( 'NONE',  ( 36.31593203568480988, 8.028139509847019184, -23.11534131364107836 ) ) ;
#65180=CARTESIAN_POINT ( 'NONE',  ( -154.8006992380338716, 70.15733562427988090, -63.82271102350273395 ) ) ;
#65181=CARTESIAN_POINT ( 'NONE',  ( 64.94098077424392557, 14.16208887966257102, 3.203578031880352839 ) ) ;
#65183=B_SPLINE_CURVE_WITH_KNOTS ( 'NONE', 3,
 ( #38952, #55105, #6929, #18184, #28379, #50538, #49826, #34016, #55458, #50189, #23471, #44910, #35669, #40583, #66649, #13519, #56418, #67340, #14209, #61355, #8934, #8239, #57122, #67000 ),
 .UNSPECIFIED., .F., .F.,
 ( 4, 2, 2, 2, 2, 2, 2, 2, 2, 2, 2, 4 ),
 ( 0.000000000000000000, 0.001398572767507159443, 0.002097859151260731466, 0.002797145535014303273, 0.004195718302521427370, 0.005594291070028550167, 0.006992863837535672963, 0.007692150221289229158, 0.008391436605042785352, 0.009790009372549946312, 0.01048929575630352419, 0.01118858214005710207 ),
 .UNSPECIFIED. ) ;
#65185=CARTESIAN_POINT ( 'NONE',  ( -54.08816720029311398, 15.46531105893042302, -35.26310301817208881 ) ) ;
#65186=CARTESIAN_POINT ( 'NONE',  ( 63.01563776193091826, 13.70579113808094718, -77.56524142263344856 ) ) ;
#65187=CARTESIAN_POINT ( 'NONE',  ( -150.3214134925456449, 66.19890482612721883, -88.53518711165342836 ) ) ;
#65190=DIRECTION ( 'NONE',  ( -0.000000000000000000, 1.000000000000000000, -0.000000000000000000 ) ) ;
#65191=ORIENTED_EDGE ( 'NONE', *, *, #3335, .F. ) ;
#65195=ORIENTED_EDGE ( 'NONE', *, *, #62495, .F. ) ;
#65196=CARTESIAN_POINT ( 'NONE',  ( -10.46803069297985900, 7.077485182625206761, -9.050212947433250221 ) ) ;
#65197=CARTESIAN_POINT ( 'NONE',  ( -165.6956608327360811, 80.66498882796977909, 93.08182273110395499 ) ) ;
#65200=CARTESIAN_POINT ( 'NONE',  ( -62.55320287144887459, 17.87319849854531029, -42.47875363776260826 ) ) ;
#65201=CARTESIAN_POINT ( 'NONE',  ( -11.14668121284976188, 8.139398342256733088, -9.344527173102546769 ) ) ;
#65203=CARTESIAN_POINT ( 'NONE',  ( 23.24028701062093916, 6.853614888934262517, -15.19644949956558655 ) ) ;
#65206=B_SPLINE_CURVE_WITH_KNOTS ( 'NONE', 3,
 ( #68176, #40728, #30190, #62888, #25948, #9425, #47378, #56924, #57613, #68833, #30882, #51643, #3451, #57265, #46011, #42117, #52326, #19624, #63575, #8389, #29834, #14357, #25613, #3114, #46346, #24576, #47047, #68506, #41776, #62546, #63232, #22388, #42459, #16068, #64963, #36847, #16758, #64609, #5174, #54027, #58625, #47724, #26969, #15729 ),
 .UNSPECIFIED., .F., .F.,
 ( 4, 2, 2, 2, 2, 2, 2, 2, 2, 2, 2, 2, 2, 2, 2, 2, 2, 2, 2, 2, 2, 4 ),
 ( 7.152448122690996019E-18, 0.001476829494128814504, 0.002215244241193227610, 0.002953658988257641151, 0.004430488482386469966, 0.005907317976515297914, 0.007384147470644126729, 0.008122562217708542004, 0.008860976964772959014, 0.01033780645890178783, 0.01181463595303061838, 0.01255305070009503365, 0.01329146544715945066, 0.01476829494128827948, 0.01550670968835269822, 0.01624512443541711870, 0.01772195392954596660, 0.01919878342367481450, 0.01993719817073924191, 0.02067561291780366586, 0.02215244241193249294, 0.02362927190606132349 ),
 .UNSPECIFIED. ) ;
#65207=ORIENTED_EDGE ( 'NONE', *, *, #35262, .T. ) ;
#65208=ORIENTED_EDGE ( 'NONE', *, *, #66168, .T. ) ;
#65210=LINE ( 'NONE', #22997, #7354 ) ;
#65211=CARTESIAN_POINT ( 'NONE',  ( -59.95908162666859909, 17.10002565866494706, -90.72874173270432152 ) ) ;
#65214=CARTESIAN_POINT ( 'NONE',  ( -7.825402957745087207, -170.0000000000000000, -62.26262132240749736 ) ) ;
#65215=EDGE_CURVE ( 'NONE', #16185, #64139, #32119, .T. ) ;
#65217=CARTESIAN_POINT ( 'NONE',  ( 22.53041628628730564, 6.810083298012989061, 40.83674206048191024 ) ) ;
#65218=CARTESIAN_POINT ( 'NONE',  ( 141.3036441389950539, 47.31002705502925920, -17.71872056072848878 ) ) ;
#65219=VERTEX_POINT ( 'NONE', #15253 ) ;
#65222=CARTESIAN_POINT ( 'NONE',  ( -55.05276343752909440, 15.72344139423348430, 45.31732777293115788 ) ) ;
#65223=CARTESIAN_POINT ( 'NONE',  ( -7.825402957745085430, 6.891034867348157178, 18.27103044898354511 ) ) ;
#65224=CARTESIAN_POINT ( 'NONE',  ( 59.95259601283824225, 11.98300577492411101, -23.22648120359055923 ) ) ;
#65225=CARTESIAN_POINT ( 'NONE',  ( -38.92726670956012924, 10.94099576009806363, 64.07225517871486886 ) ) ;
#65226=CARTESIAN_POINT ( 'NONE',  ( 197.3700262219431067, 98.41176242030790888, 65.18205950884318156 ) ) ;
#65227=ORIENTED_EDGE ( 'NONE', *, *, #12559, .T. ) ;
#65228=CARTESIAN_POINT ( 'NONE',  ( 188.5653887627528036, 88.01608521313130495, 63.04380369743464740 ) ) ;
#65230=CARTESIAN_POINT ( 'NONE',  ( -0.3255842968951684346, 7.525381170773409956, -42.42579087474055655 ) ) ;
#65232=CARTESIAN_POINT ( 'NONE',  ( -84.96580414052108665, 24.82184094495578819, -38.53758876423822244 ) ) ;
#65234=DIRECTION ( 'NONE',  ( -0.000000000000000000, 1.000000000000000000, -0.000000000000000000 ) ) ;
#65235=CARTESIAN_POINT ( 'NONE',  ( 8.288451200428832877, 6.376395059685423305, -69.37159842231915263 ) ) ;
#65239=VECTOR ( 'NONE', #54663, 1000.000000000000000 ) ;
#65241=LINE ( 'NONE', #42738, #17424 ) ;
#65245=MECHANICAL_DESIGN_GEOMETRIC_PRESENTATION_REPRESENTATION('',(#63151),#32657);
#65246=ADVANCED_FACE ( 'NONE', ( #16281 ), #14896, .F. ) ;
#65249=CARTESIAN_POINT ( 'NONE',  ( 178.3973431913384218, 75.93084153045994356, 83.46876488482124046 ) ) ;
#65254=FACE_OUTER_BOUND ( 'NONE', #35879, .T. ) ;
#65258=CARTESIAN_POINT ( 'NONE',  ( 140.9141742510256847, 47.05414327990549594, 61.26423157896623906 ) ) ;
#65259=CARTESIAN_POINT ( 'NONE',  ( -73.79615177260656367, 20.52570924097572203, -36.89085579558944517 ) ) ;
#65263=CARTESIAN_POINT ( 'NONE',  ( -52.67596829228261868, 15.09584868440940220, -23.00177376059447099 ) ) ;
#65270=EDGE_CURVE ( 'NONE', #35238, #16646, #66377, .T. ) ;
#65272=CARTESIAN_POINT ( 'NONE',  ( -130.9590960505229873, 49.92041220780520661, 86.26984079606188516 ) ) ;
#65273=ORIENTED_EDGE ( 'NONE', *, *, #52182, .F. ) ;
#65274=CARTESIAN_POINT ( 'NONE',  ( 62.04382205963243280, 13.48099884269681148, 17.92121075436126532 ) ) ;
#65277=CARTESIAN_POINT ( 'NONE',  ( -126.3458714439411352, 46.79154809309479646, 30.61994787315707001 ) ) ;
#65280=CARTESIAN_POINT ( 'NONE',  ( 86.62931800182293784, 20.48449268398422518, 29.71208757247930521 ) ) ;
#65281=CARTESIAN_POINT ( 'NONE',  ( 81.04675113612958626, 17.59091904316106536, -11.44449432899062202 ) ) ;
#65283=CARTESIAN_POINT ( 'NONE',  ( 89.87518614971253328, 20.55373388674513535, -76.94423166383461421 ) ) ;
#65290=CARTESIAN_POINT ( 'NONE',  ( 45.36109889487606495, 9.259412558041159258, 41.99414667629699238 ) ) ;
#65291=CYLINDRICAL_SURFACE ( 'NONE', #31744, 7.500000000000013323 ) ;
#65292=FACE_OUTER_BOUND ( 'NONE', #15728, .T. ) ;
#65297=CARTESIAN_POINT ( 'NONE',  ( 209.6642862813004911, 115.2127693334913801, -49.46362703668027194 ) ) ;
#65300=CARTESIAN_POINT ( 'NONE',  ( 65.40383840050414221, 14.27443447873231186, -50.34691897934524718 ) ) ;
#65301=CARTESIAN_POINT ( 'NONE',  ( 39.40195752203891999, 9.424259417798147354, -35.61981746542776506 ) ) ;
#65302=CARTESIAN_POINT ( 'NONE',  ( 8.000000000000007105, 249.8719672152120381, -95.00000000000133582 ) ) ;
#65304=ORIENTED_EDGE ( 'NONE', *, *, #27295, .T. ) ;
#65306=ORIENTED_EDGE ( 'NONE', *, *, #53600, .F. ) ;
#65311=CARTESIAN_POINT ( 'NONE',  ( 88.28889510440060917, 21.05995314109330963, 71.37459607837911335 ) ) ;
#65312=CYLINDRICAL_SURFACE ( 'NONE', #17423, 7.500000000000013323 ) ;
#65314=CARTESIAN_POINT ( 'NONE',  ( -142.6736406357357794, 58.59303246027003098, 94.99999999999866418 ) ) ;
#65326=CARTESIAN_POINT ( 'NONE',  ( -108.9136445001389859, 36.28030794288189753, -65.85060173500423275 ) ) ;
#65327=CARTESIAN_POINT ( 'NONE',  ( 83.49613381502568643, 19.43408251395296205, 84.07914609096779657 ) ) ;
#65330=CARTESIAN_POINT ( 'NONE',  ( -189.2442476610617916, 107.0963225822736007, -14.83136874092102708 ) ) ;
#65332=CARTESIAN_POINT ( 'NONE',  ( -172.7173255566597163, 88.18461381371096763, -49.71195716475001092 ) ) ;
#65334=CARTESIAN_POINT ( 'NONE',  ( -128.9863978264384627, 49.78205252558956317, -35.57704840273653701 ) ) ;
#65336=CARTESIAN_POINT ( 'NONE',  ( 204.6977192012829789, -170.0000000000000000, -78.17048162308530834 ) ) ;
#65344=CARTESIAN_POINT ( 'NONE',  ( 164.2809400227150718, 64.46036035961996902, -94.16440510607482395 ) ) ;
#65348=CARTESIAN_POINT ( 'NONE',  ( -173.1211646369891355, -170.0000000000000000, -34.71195716474998960 ) ) ;
#65350=CARTESIAN_POINT ( 'NONE',  ( 117.4711568421290195, 33.49899443629672646, 12.33247850546726454 ) ) ;
#65361=CARTESIAN_POINT ( 'NONE',  ( -35.83016564023557748, 11.37623363089854678, -90.41096227095786730 ) ) ;
#65362=ADVANCED_FACE ( 'NONE', ( #50386 ), #61960, .F. ) ;
#65363=CARTESIAN_POINT ( 'NONE',  ( -15.27594996066617128, 8.502079791899653571, -70.75202261163761364 ) ) ;
#65369=CARTESIAN_POINT ( 'NONE',  ( -76.10382222627281124, 22.43453174720079701, -35.56271879029210936 ) ) ;
#65372=CARTESIAN_POINT ( 'NONE',  ( -37.92542950990690542, 10.74638084523341419, -19.74604464320939456 ) ) ;
#65374=CARTESIAN_POINT ( 'NONE',  ( -38.54881010929334906, 10.86689971295294121, -67.22396423449106351 ) ) ;
#65375=CARTESIAN_POINT ( 'NONE',  ( 18.19858669090300296, 7.596860100017452488, 71.46566277036495762 ) ) ;
#65383=CARTESIAN_POINT ( 'NONE',  ( -34.06864996337442619, 10.03773626259442153, -35.78902194044933083 ) ) ;
#65384=CARTESIAN_POINT ( 'NONE',  ( -106.7799677022395031, 35.12603236357178815, 85.70035464166211625 ) ) ;
#65387=CARTESIAN_POINT ( 'NONE',  ( -127.6861178856153458, 47.68458428355326362, 72.26108953896540754 ) ) ;
#65388=CARTESIAN_POINT ( 'NONE',  ( -59.74946260537818432, 17.03883958539088539, 85.65039846766379128 ) ) ;
#65389=CARTESIAN_POINT ( 'NONE',  ( 79.14242532928585661, 17.00090225993928073, 64.56634896141592606 ) ) ;
#65394=CARTESIAN_POINT ( 'NONE',  ( 211.8476521439973226, 116.6941316755177240, -68.38290356003247439 ) ) ;
#65396=CARTESIAN_POINT ( 'NONE',  ( -72.76696720809547969, 20.16136115364205139, 15.73114799941608588 ) ) ;
#65397=CARTESIAN_POINT ( 'NONE',  ( -118.6727642982647666, 43.09863379477474865, 62.86749931588654761 ) ) ;
#65398=CARTESIAN_POINT ( 'NONE',  ( -47.61380558691495679, 12.81230778489788591, 11.95980790945447758 ) ) ;
#65403=CARTESIAN_POINT ( 'NONE',  ( 110.2429982417149574, -170.0000000000000000, -62.76698815611734972 ) ) ;
#65405=DIRECTION ( 'NONE',  ( -0.000000000000000000, 1.000000000000000000, -0.000000000000000000 ) ) ;
#65407=CARTESIAN_POINT ( 'NONE',  ( -81.23297981660236644, 23.31577157498399089, 44.96949360496901704 ) ) ;
#65408=CARTESIAN_POINT ( 'NONE',  ( -23.98747857548121942, 9.501432345103358657, -68.67649969425383460 ) ) ;
#65409=CARTESIAN_POINT ( 'NONE',  ( 45.76405797021008937, 10.34101216371941590, 41.39308771693118416 ) ) ;
#65410=VECTOR ( 'NONE', #45331, 1000.000000000000000 ) ;
#65411=CARTESIAN_POINT ( 'NONE',  ( 130.3245512970361233, 39.33195360491887982, -10.04568308804323529 ) ) ;
#65413=ORIENTED_EDGE ( 'NONE', *, *, #19891, .T. ) ;
#65416=CARTESIAN_POINT ( 'NONE',  ( 32.38493285958205803, 8.611594965040678673, -18.93455897652550135 ) ) ;
#65417=CARTESIAN_POINT ( 'NONE',  ( 181.5072453427590347, 79.03352099595184654, 2.464043515047717570 ) ) ;
#65418=B_SPLINE_CURVE_WITH_KNOTS ( 'NONE', 3,
 ( #1393, #65417, #23900, #66828, #18621, #40076, #22848, #13351, #34810, #62831, #68448, #42400, #41376, #37118, #26225, #42735, #9709, #20945, #57889, #52937, #36789, #14970, #50977, #68774, #15327, #20255, #57550, #20590, #56248, #14631, #46639, #4087, #4763, #36437, #2792, #31502, #42053, #63861, #69117, #53279, #8061, #58230, #10046, #47663 ),
 .UNSPECIFIED., .F., .F.,
 ( 4, 2, 2, 2, 2, 2, 2, 2, 2, 2, 2, 2, 2, 2, 2, 2, 2, 2, 2, 2, 2, 4 ),
 ( 0.02814986980477067122, 0.02995274102020796525, 0.03085417662792662788, 0.03175561223564529051, 0.03355848345108267128, 0.03536135466652005205, 0.03716422588195743282, 0.03896709709739481359, 0.03986853270511350744, 0.04076996831283219436, 0.04167140392055088127, 0.04257283952826957513, 0.04347427513598826898, 0.04437571074370695590, 0.04527714635142565669, 0.04617858195914434360, 0.04798145317458173131, 0.04978432439001910514, 0.05158719560545649285, 0.05339006682089388056, 0.05519293803633126133, 0.05699580925176864904 ),
 .UNSPECIFIED. ) ;
#65419=CARTESIAN_POINT ( 'NONE',  ( -5.888165822225390755, 7.780336669456523246, 18.02069410080496681 ) ) ;
#65420=CARTESIAN_POINT ( 'NONE',  ( -1.454841858088672613, 7.566772088227303072, 60.49456332401662451 ) ) ;
#65421=ADVANCED_FACE ( 'NONE', ( #3571 ), #35935, .F. ) ;
#65422=SURFACE_SIDE_STYLE ('',( #28838 ) ) ;
#65425=CARTESIAN_POINT ( 'NONE',  ( -122.8118341587044995, 44.49743491855738853, -76.11102093153681380 ) ) ;
#65429=DIRECTION ( 'NONE',  ( 0.000000000000000000, -1.000000000000000000, 0.000000000000000000 ) ) ;
#65431=CARTESIAN_POINT ( 'NONE',  ( -128.7359167797845600, 49.61038851545254147, -89.14962691298688924 ) ) ;
#65436=EDGE_LOOP ( 'NONE', ( #64324, #1925, #503, #28053 ) ) ;
#65438=CARTESIAN_POINT ( 'NONE',  ( -78.66644367742111399, 22.32174330031316956, 45.41820113967312977 ) ) ;
#65440=CARTESIAN_POINT ( 'NONE',  ( 128.0762755119335452, 38.04197700431935658, -92.41578206806259743 ) ) ;
#65446=CARTESIAN_POINT ( 'NONE',  ( 89.88695630745282017, 20.55793566325393940, 17.14005976452316560 ) ) ;
#65453=CARTESIAN_POINT ( 'NONE',  ( 31.90170717962883984, 8.563261373066637816, 37.65398698468158756 ) ) ;
#65454=CARTESIAN_POINT ( 'NONE',  ( -173.9526029538035914, 89.57590038685107459, -49.67757543776112072 ) ) ;
#65455=CARTESIAN_POINT ( 'NONE',  ( -126.8005235842505840, 47.09307471149450919, -8.110568341272605508 ) ) ;
#65460=CARTESIAN_POINT ( 'NONE',  ( 140.9141742510256563, 47.05414327990548884, -72.95852137335218401 ) ) ;
#65464=FACE_BOUND ( 'NONE', #53752, .T. ) ;
#65465=CARTESIAN_POINT ( 'NONE',  ( -3.868882431147339318, 6.665575841812209745, -76.13890115071046694 ) ) ;
#65467=CARTESIAN_POINT ( 'NONE',  ( -144.2155061717026285, 61.10843690942980544, -10.14790075599239216 ) ) ;
#65469=CARTESIAN_POINT ( 'NONE',  ( -0.3255842968951683236, 7.525381170773409067, 38.10786089665049303 ) ) ;
#65474=CARTESIAN_POINT ( 'NONE',  ( -14.56151485655250433, 8.434196591921335084, 34.28149470285157463 ) ) ;
#65475=CARTESIAN_POINT ( 'NONE',  ( 161.7209903610255139, 61.03262545641849357, 16.26150805458010495 ) ) ;
#65476=CARTESIAN_POINT ( 'NONE',  ( 93.32756701508618846, 22.89083686918419502, -13.06632485724244397 ) ) ;
#65477=ORIENTED_EDGE ( 'NONE', *, *, #59054, .F. ) ;
#65479=ORIENTED_EDGE ( 'NONE', *, *, #30519, .T. ) ;
#65482=CARTESIAN_POINT ( 'NONE',  ( 103.4246886032334061, 26.94746784261150552, 87.65654458658119097 ) ) ;
#65483=FACE_OUTER_BOUND ( 'NONE', #46835, .T. ) ;
#65484=CARTESIAN_POINT ( 'NONE',  ( 67.92995549349549833, 13.86623459444476225, -22.06271008403504652 ) ) ;
#65485=CARTESIAN_POINT ( 'NONE',  ( -29.51272929882556539, 10.30144624948893828, -35.56467666911228065 ) ) ;
#65486=DIRECTION ( 'NONE',  ( -0.000000000000000000, 0.000000000000000000, -1.000000000000000000 ) ) ;
#65488=CARTESIAN_POINT ( 'NONE',  ( -118.6727642982647666, 43.09863379477475576, -17.66615245550452329 ) ) ;
#65489=EDGE_LOOP ( 'NONE', ( #64896, #63837 ) ) ;
#65491=CARTESIAN_POINT ( 'NONE',  ( 38.90907126433564400, 9.359889524363181224, 71.75838489642698903 ) ) ;
#65492=CARTESIAN_POINT ( 'NONE',  ( 173.8575673535406452, 71.59843387604337295, 61.62534631081166481 ) ) ;
#65499=CARTESIAN_POINT ( 'NONE',  ( 94.14197848494937659, 23.19876128416617789, 10.37775773208338492 ) ) ;
#65500=CARTESIAN_POINT ( 'NONE',  ( 187.0788993276712233, 86.37277723143235164, -21.39429512477833129 ) ) ;
#65501=CARTESIAN_POINT ( 'NONE',  ( 13.84704553156521811, 7.452804552247568992, 57.11067823459568160 ) ) ;
#65504=CARTESIAN_POINT ( 'NONE',  ( 39.40195752203892710, 8.409560354027385998, -8.775266874964067654 ) ) ;
#65506=FACE_BOUND ( 'NONE', #3655, .T. ) ;
#65507=CARTESIAN_POINT ( 'NONE',  ( -57.43251939610648549, 15.33203492375495181, -49.84526837728627413 ) ) ;
#65514=CARTESIAN_POINT ( 'NONE',  ( 93.08174259058944244, 22.79847752828720786, -39.46674160480419857 ) ) ;
#65517=CARTESIAN_POINT ( 'NONE',  ( -50.53243683205840853, 14.55237037207939643, 70.66630208468741614 ) ) ;
#65519=CARTESIAN_POINT ( 'NONE',  ( 208.9585401441655392, 114.1617785893844115, 69.74089473411397933 ) ) ;
#65522=CARTESIAN_POINT ( 'NONE',  ( 56.66775172211442424, 11.28938863449062069, 14.47032970562600696 ) ) ;
#65527=CARTESIAN_POINT ( 'NONE',  ( 116.4569059613810680, 32.98885890446639735, 94.99999999999866418 ) ) ;
#65528=CARTESIAN_POINT ( 'NONE',  ( 109.3079614081140676, 28.45126415661783525, 44.56732555389881867 ) ) ;
#65529=EDGE_CURVE ( 'NONE', #31812, #52659, #23651, .T. ) ;
#65534=CARTESIAN_POINT ( 'NONE',  ( 39.40195752203891999, 8.409560354027407314, -35.61981746542776506 ) ) ;
#65535=CARTESIAN_POINT ( 'NONE',  ( 162.0812592823605200, 62.62783216273700049, 42.84411675552712495 ) ) ;
#65536=CARTESIAN_POINT ( 'NONE',  ( 103.9685899589048148, 27.18106603025991674, 6.150318247617813761 ) ) ;
#65537=CARTESIAN_POINT ( 'NONE',  ( 65.62985354949977079, 14.32996029952554373, 17.50227395258704277 ) ) ;
#65539=CARTESIAN_POINT ( 'NONE',  ( 107.9213359589208920, 28.92595015506874745, -9.430594635280971971 ) ) ;
#65540=CARTESIAN_POINT ( 'NONE',  ( 61.08522853873727598, 13.26388801693371811, -35.95693286015492163 ) ) ;
#65541=CARTESIAN_POINT ( 'NONE',  ( -7.825402957745085430, 7.899365992529253866, -89.10717191287116634 ) ) ;
#65542=CARTESIAN_POINT ( 'NONE',  ( -151.1225012833390338, 66.89247819254583760, -88.66664194563858814 ) ) ;
#65543=CARTESIAN_POINT ( 'NONE',  ( -173.1211646369891071, 88.63826465341152527, 18.97714401617737323 ) ) ;
#65544=CARTESIAN_POINT ( 'NONE',  ( 93.82901523493131890, 22.00453947897597828, 88.77271230041061756 ) ) ;
#65552=CARTESIAN_POINT ( 'NONE',  ( -47.80896875121165834, 12.85816703949531359, 39.77673797478080076 ) ) ;
#65553=DIRECTION ( 'NONE',  ( -0.000000000000000000, 1.000000000000000000, -0.000000000000000000 ) ) ;
#65554=DIRECTION ( 'NONE',  ( -0.000000000000000000, 0.000000000000000000, -1.000000000000000000 ) ) ;
#65556=CARTESIAN_POINT ( 'NONE',  ( -58.75378739419586793, 16.75118858561006618, -49.25797758003430005 ) ) ;
#65559=CARTESIAN_POINT ( 'NONE',  ( -71.67841390531691559, 19.78168466957078664, -72.19491188520656522 ) ) ;
#65561=ORIENTED_EDGE ( 'NONE', *, *, #36767, .F. ) ;
#65566=CARTESIAN_POINT ( 'NONE',  ( -143.7133518487517279, 60.70463114991427034, 16.14514466890094724 ) ) ;
#65567=CARTESIAN_POINT ( 'NONE',  ( -61.90435325615973738, 17.67681010539238429, -93.32376335434845771 ) ) ;
#65570=CARTESIAN_POINT ( 'NONE',  ( -102.2801239173131052, 32.78103895658057354, -50.01457726497594081 ) ) ;
#65573=CARTESIAN_POINT ( 'NONE',  ( 137.6104751318277124, 44.92718313329110202, -23.17606804121535902 ) ) ;
#65577=B_SPLINE_CURVE_WITH_KNOTS ( 'NONE', 3,
 ( #30185, #35808, #62883, #51298, #46007, #19268, #67819, #41080, #14353, #57260, #30877, #51974, #14684, #68502, #3789, #25259, #46694, #68172, #4143, #37174, #10436, #26285, #47720, #58969, #48391, #42113, #59653, #21684, #64256, #54377, #10783, #27655, #64958, #227, #52995, #32257, #31907, #53337, #16413, #42787, #69181, #21009, #58621, #16754, #42454, #4816, #26964, #53690, #38215, #43134 ),
 .UNSPECIFIED., .F., .F.,
 ( 4, 2, 2, 2, 2, 2, 2, 2, 2, 2, 2, 2, 2, 2, 2, 2, 2, 2, 2, 2, 2, 2, 2, 2, 4 ),
 ( 0.03126542424884323768, 0.03330676804260256085, 0.03534811183636187709, 0.03738945563012119333, 0.03943079942388051651, 0.04045147132076019197, 0.04147214321763986744, 0.04249281511451954291, 0.04351348701139921837, 0.04555483080515859706, 0.04657550270203830028, 0.04759617459891800351, 0.04810651054735787940, 0.04861684649579775530, 0.04963751839267750710, 0.05065819028955724501, 0.05167886218643699681, 0.05269953408331674166, 0.05372020598019648652, 0.05474087787707623831, 0.05576154977395598317, 0.05780289356771556308, 0.05984423736147514994, 0.06188558115523473679, 0.06392692494899432365 ),
 .UNSPECIFIED. ) ;
#65579=CARTESIAN_POINT ( 'NONE',  ( -156.6862310659956279, 71.88416263379569671, -13.22470838037755492 ) ) ;
#65581=CARTESIAN_POINT ( 'NONE',  ( 55.52750043885183828, 11.05966813607792609, -16.86601971481237072 ) ) ;
#65583=UNCERTAINTY_MEASURE_WITH_UNIT (LENGTH_MEASURE( 1.000000000000000082E-05 ), #3143, 'distance_accuracy_value', 'NONE');
#65584=CARTESIAN_POINT ( 'NONE',  ( -49.45858366215605173, 13.25262207532077952, 32.81574071421050576 ) ) ;
#65586=ORIENTED_EDGE ( 'NONE', *, *, #21898, .T. ) ;
#65588=CARTESIAN_POINT ( 'NONE',  ( -151.2497169612549044, 65.66843968092749151, 72.41451540298392331 ) ) ;
#65589=CARTESIAN_POINT ( 'NONE',  ( -6.840165690716690783, 7.836465889224641046, -50.36917416540237724 ) ) ;
#65591=CARTESIAN_POINT ( 'NONE',  ( -172.7402246477008703, 86.70495794627620967, -88.40105834567735599 ) ) ;
#65593=FACE_BOUND ( 'NONE', #7677, .T. ) ;
#65594=CARTESIAN_POINT ( 'NONE',  ( -190.6985136298601731, 109.1272424661242582, 87.66052266422059347 ) ) ;
#65603=CARTESIAN_POINT ( 'NONE',  ( 43.97326221476411945, 9.047815246749999929, -63.99822409915773136 ) ) ;
#65607=B_SPLINE_CURVE_WITH_KNOTS ( 'NONE', 3,
 ( #39423, #55601, #11998, #66526, #60874, #7430, #1445, #6371, #22548, #28882, #33472, #50334, #50670, #13057, #45043, #23945, #7772, #29222, #45394, #18672, #61581, #65469, #54894, #30959, #45746, #52061, #30267, #62263, #56997, #67903, #52405, #46425, #8111, #68249, #61907, #24649, #14082, #13731, #56291, #57341, #24994, #15118, #19353 ),
 .UNSPECIFIED., .F., .F.,
 ( 4, 2, 2, 2, 2, 2, 2, 2, 1, 2, 2, 2, 2, 2, 2, 2, 2, 2, 2, 2, 2, 4 ),
 ( 0.000000000000000000, 0.001466540241398137275, 0.002199810362097205912, 0.002933080482796274549, 0.004399620724194417895, 0.005866160965592561241, 0.007332701206990704587, 0.008065971327689776260, 0.008799241448388847933, 0.009532511569087917871, 0.01026578168978698954, 0.01173232193118513289, 0.01319886217258327450, 0.01466540241398141785, 0.01539867253468047911, 0.01613194265537953864, 0.01759848289677766464, 0.01906502313817578717, 0.01979829325887484670, 0.02053156337957390970, 0.02199810362097203223, 0.02346464386237015476 ),
 .UNSPECIFIED. ) ;
#65610=CARTESIAN_POINT ( 'NONE',  ( -132.1053471785562863, 50.72188866504426130, -91.87369984681103574 ) ) ;
#65617=CARTESIAN_POINT ( 'NONE',  ( 133.8566784816069060, 42.60093787723653236, -24.17876034193199786 ) ) ;
#65620=DIRECTION ( 'NONE',  ( 0.000000000000000000, 0.000000000000000000, 1.000000000000000000 ) ) ;
#65621=CARTESIAN_POINT ( 'NONE',  ( 136.9654665832768217, 44.52067472585214603, 70.68427344918816857 ) ) ;
#65622=CARTESIAN_POINT ( 'NONE',  ( -71.17819443284078318, 19.60909329639483190, -42.12447784558203523 ) ) ;
#65625=CYLINDRICAL_SURFACE ( 'NONE', #29399, 7.500000000000013323 ) ;
#65626=CARTESIAN_POINT ( 'NONE',  ( -51.77431913897919458, 14.86466849149170777, -9.108735933062128254 ) ) ;
#65628=CARTESIAN_POINT ( 'NONE',  ( -124.1033713525885958, 45.32626312604504193, -8.282396413194451412 ) ) ;
#65631=CARTESIAN_POINT ( 'NONE',  ( -168.1811549361196967, 83.25427431521136157, -74.70477187311568912 ) ) ;
#65632=CARTESIAN_POINT ( 'NONE',  ( -128.9955982454845866, 48.57000285068010470, 84.97439690926448463 ) ) ;
#65633=VERTEX_POINT ( 'NONE', #20782 ) ;
#65634=CARTESIAN_POINT ( 'NONE',  ( 55.91494169499919309, 12.16343363043255721, 12.89567247696315988 ) ) ;
#65636=CARTESIAN_POINT ( 'NONE',  ( -132.0958200534848004, 50.71531800824803327, 33.89524248677182783 ) ) ;
#65639=CARTESIAN_POINT ( 'NONE',  ( 90.51709546286275554, 21.85407654229979713, 30.79386894197559599 ) ) ;
#65641=CARTESIAN_POINT ( 'NONE',  ( -78.66644367742109978, 23.39876645725288640, -23.27090004125422595 ) ) ;
#65642=CARTESIAN_POINT ( 'NONE',  ( 90.91465859190773813, 20.92790537681859675, -76.32607979879988136 ) ) ;
#65651=CYLINDRICAL_SURFACE ( 'NONE', #57027, 7.500000000000020428 ) ;
#65654=CARTESIAN_POINT ( 'NONE',  ( 208.0306608271317828, 112.7988899307265740, -50.54803444713732574 ) ) ;
#65655=EDGE_CURVE ( 'NONE', #31358, #33561, #49143, .T. ) ;
#65657=CARTESIAN_POINT ( 'NONE',  ( -103.2169245450825485, 33.25885825286820818, 57.40773309695661197 ) ) ;
#65659=CARTESIAN_POINT ( 'NONE',  ( -24.18258876560172865, 8.512344710720686436, -44.77552165097223025 ) ) ;
#65663=CARTESIAN_POINT ( 'NONE',  ( -24.71645982722741408, 9.599558729461493911, 14.20614957612933082 ) ) ;
#65666=CARTESIAN_POINT ( 'NONE',  ( -8.314575874103555364, 6.922894809783096903, -50.41807073194386390 ) ) ;
#65668=CARTESIAN_POINT ( 'NONE',  ( -84.22570405563703844, 24.51726571826275602, 69.82089765687976524 ) ) ;
#65669=CARTESIAN_POINT ( 'NONE',  ( 126.3580464630938422, 38.22944795020833197, 36.70972463671400732 ) ) ;
#65670=CARTESIAN_POINT ( 'NONE',  ( 38.90907126433565821, 9.359889524363181224, 18.06928371549960133 ) ) ;
#65672=CARTESIAN_POINT ( 'NONE',  ( 117.4396227366912626, 33.48307633470226818, -95.00000000000133582 ) ) ;
#65674=CARTESIAN_POINT ( 'NONE',  ( 211.3822731854152721, 115.9841935232942376, 93.81720800102199576 ) ) ;
#65677=CARTESIAN_POINT ( 'NONE',  ( 55.56634333706183071, 12.09342294753930069, 63.15602334383434169 ) ) ;
#65678=CARTESIAN_POINT ( 'NONE',  ( 11.81843724556921238, 7.412394300769734379, -63.49552996665384796 ) ) ;
#65679=CARTESIAN_POINT ( 'NONE',  ( -190.3061188229048639, 108.5745819235681751, -38.23057545279792890 ) ) ;
#65680=EDGE_CURVE ( 'NONE', #4867, #23369, #15167, .T. ) ;
#65684=CARTESIAN_POINT ( 'NONE',  ( 94.11387023963305865, 23.18808022568910943, 91.49174497375973658 ) ) ;
#65685=VERTEX_POINT ( 'NONE', #54418 ) ;
#65688=CARTESIAN_POINT ( 'NONE',  ( -189.2352924136013712, 107.0839554967701019, -15.71323334688268858 ) ) ;
#65689=CARTESIAN_POINT ( 'NONE',  ( -131.6133495896316958, 50.37677745548733554, 16.13319187600255589 ) ) ;
#65690=CARTESIAN_POINT ( 'NONE',  ( -165.9154624515710168, 80.89088623112733956, -40.11032779023376094 ) ) ;
#65692=CARTESIAN_POINT ( 'NONE',  ( -167.3151846658799968, 80.89015936597813550, 87.25299558331532523 ) ) ;
#65695=CARTESIAN_POINT ( 'NONE',  ( -7.330690860789851548, 6.858814156830896458, -8.573520141480127421 ) ) ;
#65696=CARTESIAN_POINT ( 'NONE',  ( -145.3279998500303236, 60.71393190715789956, -21.70027410468134121 ) ) ;
#65697=CARTESIAN_POINT ( 'NONE',  ( -5.183193881612059073, 7.740932022135016410, -62.73915333014450368 ) ) ;
#65702=CARTESIAN_POINT ( 'NONE',  ( -60.47589866267034608, 17.25153113855766662, 5.786362127798294175 ) ) ;
#65703=CARTESIAN_POINT ( 'NONE',  ( 203.9276061909314706, 105.2889220654479061, -51.32593103262161094 ) ) ;
#65707=CARTESIAN_POINT ( 'NONE',  ( 22.89634831467702369, 6.832298124325687283, -40.61357525750717201 ) ) ;
#65709=CARTESIAN_POINT ( 'NONE',  ( 116.6436511186860372, 33.08230081168869674, 14.18392456913904098 ) ) ;
#65712=CARTESIAN_POINT ( 'NONE',  ( 80.34841469379381351, 18.42674688750400946, 94.99999999999866418 ) ) ;
#65713=AXIS2_PLACEMENT_3D ( 'NONE', #7366, #44983, #66464 ) ;
#65718=CARTESIAN_POINT ( 'NONE',  ( -149.5074843970971301, -170.0000000000000000, -96.00193171241933499 ) ) ;
#65719=DIRECTION ( 'NONE',  ( 0.000000000000000000, 0.000000000000000000, 1.000000000000000000 ) ) ;
#65720=ORIENTED_EDGE ( 'NONE', *, *, #36455, .T. ) ;
#65722=DIRECTION ( 'NONE',  ( -0.8118923937861950435, -0.5838071093367415143, 0.000000000000000000 ) ) ;
#65726=CARTESIAN_POINT ( 'NONE',  ( -37.07086358537073778, 10.58360809068249964, -10.99546437007133903 ) ) ;
#65727=CARTESIAN_POINT ( 'NONE',  ( 112.1009898303695422, 30.86414810229296890, 44.39243416794982977 ) ) ;
#65728=CARTESIAN_POINT ( 'NONE',  ( -133.0835080491124813, 52.64966140620838786, 9.123835301881490167 ) ) ;
#65729=CARTESIAN_POINT ( 'NONE',  ( 18.88468164817599160, 7.626722602998419198, 57.52385489813911335 ) ) ;
#65735=CARTESIAN_POINT ( 'NONE',  ( -102.2801239173131052, 33.91021738430207222, 3.674523915951417585 ) ) ;
#65736=CARTESIAN_POINT ( 'NONE',  ( -38.87848244732137459, 10.93141945332450149, -43.80061360289953143 ) ) ;
#65738=CARTESIAN_POINT ( 'NONE',  ( -94.97822228984884418, 29.22367841510387620, 93.45206955416084327 ) ) ;
#65739=CARTESIAN_POINT ( 'NONE',  ( -143.7151964745329167, 59.41799441280377181, 33.44955188324686191 ) ) ;
#65741=CARTESIAN_POINT ( 'NONE',  ( -71.42546113164833343, 20.75891408601219368, -13.75210804638004447 ) ) ;
#65742=CARTESIAN_POINT ( 'NONE',  ( 84.73231936899556160, 18.78199960571076232, 56.78476454528978223 ) ) ;
#65743=VERTEX_POINT ( 'NONE', #28765 ) ;
#65746=CARTESIAN_POINT ( 'NONE',  ( 32.56927464314651388, 7.618924692399913212, 34.31139869032508471 ) ) ;
#65748=ORIENTED_EDGE ( 'NONE', *, *, #53684, .T. ) ;
#65749=CARTESIAN_POINT ( 'NONE',  ( 188.4937788906149194, 86.43336847120863808, 38.00740919242073090 ) ) ;
#65754=CARTESIAN_POINT ( 'NONE',  ( -48.04019567818505010, 12.91272349839805678, 13.64414622740702221 ) ) ;
#65755=CARTESIAN_POINT ( 'NONE',  ( 150.9184679586218749, 52.73111408630722963, -39.96492359852010168 ) ) ;
#65764=VERTEX_POINT ( 'NONE', #38970 ) ;
#65765=EDGE_CURVE ( 'NONE', #37519, #14111, #6949, .T. ) ;
#65766=CARTESIAN_POINT ( 'NONE',  ( -84.54326985437107567, 24.64760594531649573, 42.60397884493846732 ) ) ;
#65767=CIRCLE ( 'NONE', #9566, 243.4957430088094839 ) ;
#65768=CARTESIAN_POINT ( 'NONE',  ( 153.2523375521184619, 55.69936538551844052, -76.67477878150734227 ) ) ;
#65770=EDGE_CURVE ( 'NONE', #19626, #45314, #38691, .T. ) ;
#65771=CARTESIAN_POINT ( 'NONE',  ( -31.43908319763709969, 9.591432048623765638, 57.06100499665286208 ) ) ;
#65772=AXIS2_PLACEMENT_3D ( 'NONE', #20550, #40625, #30428 ) ;
#65774=EDGE_LOOP ( 'NONE', ( #53052, #36203, #57268, #2594 ) ) ;
#65775=EDGE_LOOP ( 'NONE', ( #38190, #7397, #51383, #66658 ) ) ;
#65778=CARTESIAN_POINT ( 'NONE',  ( 32.03384598935271299, 8.576372641735996893, -14.81213577935862347 ) ) ;
#65779=DIRECTION ( 'NONE',  ( 0.000000000000000000, 0.000000000000000000, 1.000000000000000000 ) ) ;
#65786=ORIENTED_EDGE ( 'NONE', *, *, #22475, .F. ) ;
#65788=CARTESIAN_POINT ( 'NONE',  ( 163.2886151008987952, 62.32020850087169350, -21.51899005548487764 ) ) ;
#65790=CARTESIAN_POINT ( 'NONE',  ( -169.1005390226459326, 82.76152663947084420, -9.020552741055981372 ) ) ;
#65791=CARTESIAN_POINT ( 'NONE',  ( 141.2470358420065395, 46.06959063280891797, -69.06272708122817505 ) ) ;
#65793=EDGE_CURVE ( 'NONE', #32664, #68152, #34741, .T. ) ;
#65797=CARTESIAN_POINT ( 'NONE',  ( -61.68940124183719576, 17.61226241086874467, 94.99999999999866418 ) ) ;
#65798=CARTESIAN_POINT ( 'NONE',  ( -125.8938041572051389, -170.0000000000000000, 57.46449846362076386 ) ) ;
#65799=CARTESIAN_POINT ( 'NONE',  ( 9.057575839850587229, 6.378493414438676012, 40.83252881098174214 ) ) ;
#65806=CARTESIAN_POINT ( 'NONE',  ( -143.7151964745329735, 59.41799441280379313, -73.92865047860787797 ) ) ;
#65807=CARTESIAN_POINT ( 'NONE',  ( -149.5074843970971017, 64.17983161892347255, 72.56537183036277838 ) ) ;
#65813=CARTESIAN_POINT ( 'NONE',  ( 32.29578462738147238, 8.602609172809797755, 39.82485796498851727 ) ) ;
#65815=CARTESIAN_POINT ( 'NONE',  ( -180.5954680880247167, 97.44843622358462198, -42.85213204725202729 ) ) ;
#65816=CARTESIAN_POINT ( 'NONE',  ( -130.6002960060536111, 49.67125682092488859, -21.42867186308118477 ) ) ;
#65821=LINE ( 'NONE', #11627, #61336 ) ;
#65823=CARTESIAN_POINT ( 'NONE',  ( -155.1204242627070187, 70.44799358128193489, -47.29331144879449766 ) ) ;
#65824=CARTESIAN_POINT ( 'NONE',  ( -3.857727530059795740, 6.665032499723452908, -63.39330917866369219 ) ) ;
#65825=CARTESIAN_POINT ( 'NONE',  ( -179.2210908201801374, 95.76260491022614474, 69.55831908347232684 ) ) ;
#65829=CARTESIAN_POINT ( 'NONE',  ( 70.26840926437850499, 15.51363403943109631, -95.00000000000133582 ) ) ;
#65833=CARTESIAN_POINT ( 'NONE',  ( 117.7447573007802930, 32.50990724960316669, 10.75687092132448086 ) ) ;
#65834=CARTESIAN_POINT ( 'NONE',  ( -52.74963828369503460, 15.11526739861312940, -89.26458726870900762 ) ) ;
#65840=CARTESIAN_POINT ( 'NONE',  ( 80.71682498289318630, 18.54204664833076777, -65.52526976266784686 ) ) ;
#65841=CARTESIAN_POINT ( 'NONE',  ( 115.9806768122906959, 32.75124074837841448, 85.95842849936387609 ) ) ;
#65844=CARTESIAN_POINT ( 'NONE',  ( -24.32471770265758693, 9.546495606312143778, -45.24190841075698444 ) ) ;
#65845=PLANE ( 'NONE',  #17542 ) ;
#65846=CARTESIAN_POINT ( 'NONE',  ( -149.5074843970971301, -170.0000000000000000, -76.65738112195568021 ) ) ;
#65847=DIRECTION ( 'NONE',  ( -0.000000000000000000, 1.000000000000000000, -0.000000000000000000 ) ) ;
#65852=CARTESIAN_POINT ( 'NONE',  ( 176.4367926094704728, 74.03315361639846515, 57.76155730348418160 ) ) ;
#65855=CARTESIAN_POINT ( 'NONE',  ( -172.3038663181179970, 87.72015621195183144, 72.66624519710477159 ) ) ;
#65856=CARTESIAN_POINT ( 'NONE',  ( -166.3205068063721512, 81.30869308872871670, -18.54204906781616558 ) ) ;
#65859=AXIS2_PLACEMENT_3D ( 'NONE', #29489, #3456, #23532 ) ;
#65863=CARTESIAN_POINT ( 'NONE',  ( 102.7938674513919040, 26.67851209377773358, -42.41119417710807937 ) ) ;
#65866=CARTESIAN_POINT ( 'NONE',  ( -11.78792974237933677, 7.181513757308656487, 58.08769183103347444 ) ) ;
#65870=CARTESIAN_POINT ( 'NONE',  ( 207.4867844023104340, 110.2451255333963474, -10.00719937993713238 ) ) ;
#65871=FACE_BOUND ( 'NONE', #27950, .T. ) ;
#65873=CARTESIAN_POINT ( 'NONE',  ( -59.95707852844799390, 16.05120821151901822, -48.41212873588224141 ) ) ;
#65881=CARTESIAN_POINT ( 'NONE',  ( 209.6642862813005763, 115.2127693334914085, 57.91457532517448215 ) ) ;
#65892=CARTESIAN_POINT ( 'NONE',  ( 102.8518012651273779, 25.61025413220827929, 38.40957065262233527 ) ) ;
#65893=ORIENTED_EDGE ( 'NONE', *, *, #43336, .F. ) ;
#65896=CARTESIAN_POINT ( 'NONE',  ( 164.0073343966822392, 64.23003864582457823, 40.59522386251838100 ) ) ;
#65897=CARTESIAN_POINT ( 'NONE',  ( 107.9342863085848023, 28.93180871323604109, 3.115243763729523163 ) ) ;
#65898=CARTESIAN_POINT ( 'NONE',  ( 63.50537371531942199, 13.81987663608982864, 17.96841034875761878 ) ) ;
#65902=VECTOR ( 'NONE', #41424, 1000.000000000000000 ) ;
#65903=CARTESIAN_POINT ( 'NONE',  ( -149.5074843970971017, 65.50121172469319220, -7.968279941028269420 ) ) ;
#65904=CARTESIAN_POINT ( 'NONE',  ( -131.6399667378751417, 51.62465701391630546, -10.72301646190411795 ) ) ;
#65907=CARTESIAN_POINT ( 'NONE',  ( 80.27305752291051988, 17.34925310068689441, 86.90588607176617586 ) ) ;
#65908=AXIS2_PLACEMENT_3D ( 'NONE', #57024, #3900, #46106 ) ;
#65913=PRODUCT_DEFINITION ( 'UNKNOWN', '', #68124, #31743 ) ;
#65915=DIRECTION ( 'NONE',  ( -0.000000000000000000, 1.000000000000000000, -0.000000000000000000 ) ) ;
#65916=CARTESIAN_POINT ( 'NONE',  ( -174.2736917738521925, 89.94190505570455230, 84.59568540053871288 ) ) ;
#65917=CARTESIAN_POINT ( 'NONE',  ( -50.14771795543004629, 13.42081263859818208, -21.56642457232588939 ) ) ;
#65921=CARTESIAN_POINT ( 'NONE',  ( -58.33157376762795110, 16.63098604184964202, -35.96663671462522416 ) ) ;
#65922=EDGE_CURVE ( 'NONE', #43301, #17942, #46658, .T. ) ;
#65924=CARTESIAN_POINT ( 'NONE',  ( -77.72491324796695267, 21.96482567905606587, -76.91587359936697510 ) ) ;
#65925=CARTESIAN_POINT ( 'NONE',  ( -15.08468253268399906, 7.472949889606722351, 35.66772536392182502 ) ) ;
#65928=EDGE_CURVE ( 'NONE', #41738, #15521, #45284, .T. ) ;
#65931=VERTEX_POINT ( 'NONE', #11429 ) ;
#65932=CARTESIAN_POINT ( 'NONE',  ( -146.5309471467636513, 62.99917515507674892, 18.26406283408425324 ) ) ;
#65933=CARTESIAN_POINT ( 'NONE',  ( -55.05276343752910151, 15.72344139423345588, -88.90542517938717992 ) ) ;
#65934=CARTESIAN_POINT ( 'NONE',  ( -165.9121868482146454, 80.88751546905565704, 36.23135190961774299 ) ) ;
#65935=CARTESIAN_POINT ( 'NONE',  ( 112.1100957124161539, 30.86846953551572170, -23.85696266999899606 ) ) ;
#65936=CARTESIAN_POINT ( 'NONE',  ( -109.6829043543429236, 36.70322915510440254, -95.00000000000133582 ) ) ;
#65943=CARTESIAN_POINT ( 'NONE',  ( -14.32120159453990205, 7.401444311907545703, 7.013986508477913162 ) ) ;
#65944=CARTESIAN_POINT ( 'NONE',  ( 35.65685430025423841, 7.951642554322392087, -63.44794714536580926 ) ) ;
#65945=CARTESIAN_POINT ( 'NONE',  ( 62.53328835682437159, 12.56090025569836932, -23.87614024170609639 ) ) ;
#65947=EDGE_CURVE ( 'NONE', #56201, #57172, #39434, .T. ) ;
#65948=CARTESIAN_POINT ( 'NONE',  ( -47.55360235114367384, 12.79819361309568393, 37.30471606777894067 ) ) ;
#65949=CARTESIAN_POINT ( 'NONE',  ( 204.6977192012829789, 108.0580384837234931, 71.05227132923315025 ) ) ;
#65952=CARTESIAN_POINT ( 'NONE',  ( 203.1414537950836063, 105.9225671689748509, -63.32313587288669510 ) ) ;
#65954=CARTESIAN_POINT ( 'NONE',  ( -167.9853834315979668, 81.58767916550901589, 16.96324577511894560 ) ) ;
#65955=CARTESIAN_POINT ( 'NONE',  ( -81.90020664963799391, 23.57971581008656869, -49.38679830630213274 ) ) ;
#65956=FACE_BOUND ( 'NONE', #52865, .T. ) ;
#65957=CARTESIAN_POINT ( 'NONE',  ( -190.3787397234653724, 108.6757967724292513, 88.09417750515896728 ) ) ;
#65958=VECTOR ( 'NONE', #33316, 1000.000000000000000 ) ;
#65960=CIRCLE ( 'NONE', #46852, 243.4957430088094839 ) ;
#65962=CARTESIAN_POINT ( 'NONE',  ( -132.4819073909166036, 50.98736898418874119, -65.63572201618941904 ) ) ;
#65963=CARTESIAN_POINT ( 'NONE',  ( -104.5740066103012964, 35.09687312794778080, -76.50358383647001403 ) ) ;
#65964=CARTESIAN_POINT ( 'NONE',  ( 45.36109889487606495, 9.259412558041157482, -65.38405568555769776 ) ) ;
#65965=CARTESIAN_POINT ( 'NONE',  ( 15.78827728214693416, 6.500811158483328356, 18.17015708224157322 ) ) ;
#65966=ORIENTED_EDGE ( 'NONE', *, *, #1303, .T. ) ;
#65971=CARTESIAN_POINT ( 'NONE',  ( 177.2960928338502242, 74.86012380916936593, 84.01690539734444485 ) ) ;
#65975=CARTESIAN_POINT ( 'NONE',  ( 174.9053416555736646, 72.57849647436444229, -48.00675063682053434 ) ) ;
#65976=CARTESIAN_POINT ( 'NONE',  ( -175.9852529046322331, 90.37283472601130541, -62.11202431634223586 ) ) ;
#65980=CARTESIAN_POINT ( 'NONE',  ( -174.7869898116916545, 88.99756909636809610, 18.83855922235676772 ) ) ;
#65981=CARTESIAN_POINT ( 'NONE',  ( 8.000000000000007105, 249.8719672152120381, -95.00000000000133582 ) ) ;
#65984=CARTESIAN_POINT ( 'NONE',  ( -189.7334103489410211, 107.7745063523401257, 35.72630607762302191 ) ) ;
#65987=CARTESIAN_POINT ( 'NONE',  ( -72.21947956767114363, 21.03570528348188873, 7.233083253217232667 ) ) ;
#65990=CARTESIAN_POINT ( 'NONE',  ( -132.1645230123639010, 50.76361971363044745, 87.68261071308809562 ) ) ;
#65992=CARTESIAN_POINT ( 'NONE',  ( 81.76092782665033099, 17.81692437267513895, -37.61113886829519259 ) ) ;
#65994=ORIENTED_EDGE ( 'NONE', *, *, #1597, .F. ) ;
#65995=CARTESIAN_POINT ( 'NONE',  ( -142.6264002846224059, 58.55577336362197371, 62.06999168838819259 ) ) ;
#65996=AXIS2_PLACEMENT_3D ( 'NONE', #5969, #38338, #5627 ) ;
#65997=CARTESIAN_POINT ( 'NONE',  ( 79.91920957766409117, 18.29292522273512489, 40.60004261239478041 ) ) ;
#65999=CARTESIAN_POINT ( 'NONE',  ( 185.1647878987786271, 82.82967084668432278, -23.18872253868788391 ) ) ;
#66001=CARTESIAN_POINT ( 'NONE',  ( 135.6842057900327347, 42.53841116629840968, -9.390205697492525871 ) ) ;
#66004=CARTESIAN_POINT ( 'NONE',  ( 87.11228333101216492, 19.58587579906928866, -62.66611478937539204 ) ) ;
#66005=EDGE_CURVE ( 'NONE', #49272, #9033, #32699, .T. ) ;
#66012=CARTESIAN_POINT ( 'NONE',  ( 39.88971011078924533, 8.472992116645421845, 29.91383430596324189 ) ) ;
#66013=CARTESIAN_POINT ( 'NONE',  ( 197.6316695787931792, 97.13022718399022892, -14.44928575426319028 ) ) ;
#66014=FACE_OUTER_BOUND ( 'NONE', #55796, .T. ) ;
#66017=CARTESIAN_POINT ( 'NONE',  ( 206.3053863259449656, 110.3084416756849464, -36.45535708260618435 ) ) ;
#66018=CARTESIAN_POINT ( 'NONE',  ( -71.17984086584777970, 20.67393782512344202, -68.94505476070409600 ) ) ;
#66020=CARTESIAN_POINT ( 'NONE',  ( -102.7456062648101494, 33.01749955571777662, 57.36362509687879907 ) ) ;
#66021=CARTESIAN_POINT ( 'NONE',  ( -24.70911172866234651, 8.583078995053025295, -46.16381964219784351 ) ) ;
#66022=CARTESIAN_POINT ( 'NONE',  ( 164.0158927577712973, 62.92463143894075017, -74.16841973653133380 ) ) ;
#66028=CARTESIAN_POINT ( 'NONE',  ( -71.70022581596595046, 19.78923414567082517, 94.40528620588804642 ) ) ;
#66029=CARTESIAN_POINT ( 'NONE',  ( -81.00507684688696486, 23.22613445438386393, 71.89280214441502892 ) ) ;
#66036=CARTESIAN_POINT ( 'NONE',  ( 39.08370485336855182, 8.368158338059329182, 83.60250626382003247 ) ) ;
#66038=CARTESIAN_POINT ( 'NONE',  ( 58.08938767906775524, 12.61185010801508710, 69.83399136998372114 ) ) ;
#66040=CARTESIAN_POINT ( 'NONE',  ( -12.78319349481551370, 8.274445259016799170, 16.41990438160611987 ) ) ;
#66043=CARTESIAN_POINT ( 'NONE',  ( 126.3732561463888970, 38.23795180971329444, -17.24332148280019439 ) ) ;
#66047=CARTESIAN_POINT ( 'NONE',  ( -37.39246151129641049, 11.66872370876246201, -38.22934263161189250 ) ) ;
#66050=CARTESIAN_POINT ( 'NONE',  ( -166.5806157913017387, 80.13147666146447534, 88.32463021072648246 ) ) ;
#66052=CARTESIAN_POINT ( 'NONE',  ( -118.4553071845215015, 41.78724769484931301, -43.51166089188798480 ) ) ;
#66055=CARTESIAN_POINT ( 'NONE',  ( -142.5211356634642073, 58.47296527616904882, -18.20987446567380985 ) ) ;
#66056=CARTESIAN_POINT ( 'NONE',  ( -1.455067768715154530, 7.566780179921183347, -65.79655557177798642 ) ) ;
#66060=EDGE_LOOP ( 'NONE', ( #3599, #53159 ) ) ;
#66061=DIRECTION ( 'NONE',  ( 0.000000000000000000, 0.000000000000000000, 1.000000000000000000 ) ) ;
#66062=CARTESIAN_POINT ( 'NONE',  ( 204.6977192012829789, 106.3443248447423599, -51.32593103262161094 ) ) ;
#66065=CARTESIAN_POINT ( 'NONE',  ( 16.77391662606471456, 6.533867394142988339, -35.56755799161265941 ) ) ;
#66067=CARTESIAN_POINT ( 'NONE',  ( 117.0069443446175512, 33.26475960880694061, 13.51689491381812402 ) ) ;
#66070=CARTESIAN_POINT ( 'NONE',  ( 179.4074606910091347, 78.34362448405025248, 71.01390593598598855 ) ) ;
#66072=VERTEX_POINT ( 'NONE', #44134 ) ;
#66073=AXIS2_PLACEMENT_3D ( 'NONE', #59832, #38044, #64781 ) ;
#66074=CARTESIAN_POINT ( 'NONE',  ( -71.22878586122432409, 19.62649588091170116, -14.77281325402038448 ) ) ;
#66076=CARTESIAN_POINT ( 'NONE',  ( 39.40195752203892710, -170.0000000000000000, 37.41383430596326320 ) ) ;
#66078=CARTESIAN_POINT ( 'NONE',  ( 162.6190874793280443, 61.76782592053313437, 31.45076619963536757 ) ) ;
#66081=VERTEX_POINT ( 'NONE', #43786 ) ;
#66084=CARTESIAN_POINT ( 'NONE',  ( -33.83558513595455253, 9.996963989836508802, -8.861627575112802191 ) ) ;
#66085=CARTESIAN_POINT ( 'NONE',  ( 110.2429982417149574, 29.99119854320843714, 44.61121420573733332 ) ) ;
#66088=ORIENTED_EDGE ( 'NONE', *, *, #21073, .T. ) ;
#66090=ORIENTED_EDGE ( 'NONE', *, *, #30646, .F. ) ;
#66093=CARTESIAN_POINT ( 'NONE',  ( -108.6622665321722963, 37.28993738537008795, 7.227033062257481433 ) ) ;
#66094=CARTESIAN_POINT ( 'NONE',  ( -102.2801239173131194, -170.0000000000000000, 11.17452391595143091 ) ) ;
#66095=CARTESIAN_POINT ( 'NONE',  ( 163.5430354047457229, -170.0000000000000000, 94.99999999999866418 ) ) ;
#66098=CARTESIAN_POINT ( 'NONE',  ( -126.7989199172159260, 47.09198523267864545, 57.50526014522036178 ) ) ;
#66099=CARTESIAN_POINT ( 'NONE',  ( -73.81801970646054656, 21.60231032711190835, -10.04354702328394922 ) ) ;
#66104=CARTESIAN_POINT ( 'NONE',  ( -173.9048502674867507, 88.00429107724478683, -88.43178570352854706 ) ) ;
#66117=EDGE_CURVE ( 'NONE', #33721, #59065, #6867, .T. ) ;
#66118=B_SPLINE_CURVE_WITH_KNOTS ( 'NONE', 3,
 ( #54357, #10767, #54716, #26947, #49432, #38195, #6544, #918, #48725, #32578, #31887, #21668, #37851, #65281, #6184, #38545, #16736, #43461, #54002, #10419, #208, #17076, #5151, #43116, #26608, #59988, #48047, #22367, #27641, #69503, #21323, #43808, #49080, #64941, #1263, #42770, #5494, #22719, #27988, #64237, #32237, #16047, #44157, #15707, #37498 ),
 .UNSPECIFIED., .F., .F.,
 ( 4, 2, 2, 2, 2, 2, 2, 2, 2, 2, 2, 1, 2, 2, 2, 2, 2, 2, 2, 2, 2, 2, 4 ),
 ( 1.440969542111313559E-17, 0.001502898956853370317, 0.002254348435280046584, 0.003005797913706723286, 0.004508696870560116587, 0.005260146348986829284, 0.006011595827413541981, 0.007514494784267002937, 0.009017393741120462158, 0.01052029269797392225, 0.01127174217640064882, 0.01202319165482737540, 0.01277464113325410024, 0.01352609061168082681, 0.01502898956853427996, 0.01578043904696100480, 0.01653188852538773138, 0.01803478748224117759, 0.01953768643909462380, 0.02028913591752134690, 0.02104058539594807348, 0.02254348435280155438, 0.02404638330965503529 ),
 .UNSPECIFIED. ) ;
#66122=CARTESIAN_POINT ( 'NONE',  ( -107.6591239831840170, 35.59818735115023713, -90.95842461620235042 ) ) ;
#66127=CYLINDRICAL_SURFACE ( 'NONE', #24131, 7.500000000000020428 ) ;
#66129=CARTESIAN_POINT ( 'NONE',  ( -80.54757501605355685, 23.04700348514568020, 45.18237135369550828 ) ) ;
#66130=CARTESIAN_POINT ( 'NONE',  ( 154.4617654203035784, 56.60942201271839025, -77.35331686145707408 ) ) ;
#66131=CARTESIAN_POINT ( 'NONE',  ( 46.84154678921878912, 10.51341196666389344, 36.43198548304936679 ) ) ;
#66132=CARTESIAN_POINT ( 'NONE',  ( -24.41864932425148282, 8.543938959778815345, 67.21142328142714462 ) ) ;
#66135=CARTESIAN_POINT ( 'NONE',  ( 110.2429982417149574, 29.99119854320846201, 29.61121420573730489 ) ) ;
#66136=VERTEX_POINT ( 'NONE', #28316 ) ;
#66137=CARTESIAN_POINT ( 'NONE',  ( 32.89501968360929851, 8.663558833820820482, -12.51357414923122136 ) ) ;
#66140=CARTESIAN_POINT ( 'NONE',  ( 141.3340962699191437, 47.33011414407334883, 91.38631405835374721 ) ) ;
#66143=ORIENTED_EDGE ( 'NONE', *, *, #51686, .T. ) ;
#66144=B_SPLINE_CURVE_WITH_KNOTS ( 'NONE', 3,
 ( #21330, #58611, #64246, #37507, #41762, #26275, #15024, #69510, #58960, #52650, #42445, #16404, #10775, #63562, #32247, #37165, #31896, #37861, #59309, #10427, #53680, #53328, #48382, #25932, #11121, #26954, #31549, #58273, #218, #57936, #4474, #47363, #21676, #25601, #32586, #68820, #20641, #47711, #47035, #42102, #68493, #20298, #15372, #36834 ),
 .UNSPECIFIED., .F., .F.,
 ( 4, 2, 2, 2, 2, 2, 2, 2, 2, 2, 2, 2, 2, 2, 2, 2, 2, 2, 2, 2, 2, 4 ),
 ( 0.02814986980477066775, 0.02995274102020799301, 0.03085417662792663829, 0.03175561223564528357, 0.03355848345108266434, 0.03536135466652004511, 0.03716422588195742588, 0.03896709709739480665, 0.03986853270511349356, 0.04076996831283218048, 0.04167140392055087433, 0.04257283952826956125, 0.04347427513598825510, 0.04437571074370694202, 0.04527714635142563587, 0.04617858195914432973, 0.04798145317458170356, 0.04978432439001907739, 0.05158719560545646510, 0.05339006682089383893, 0.05519293803633121970, 0.05699580925176860047 ),
 .UNSPECIFIED. ) ;
#66146=ORIENTED_EDGE ( 'NONE', *, *, #8738, .T. ) ;
#66149=CARTESIAN_POINT ( 'NONE',  ( 70.51601918574516503, 14.53832276813545121, 64.39593449160031469 ) ) ;
#66150=CARTESIAN_POINT ( 'NONE',  ( -126.7183033021620844, 48.24754605562520027, -88.63661005779232482 ) ) ;
#66154=CARTESIAN_POINT ( 'NONE',  ( -125.8938041572051389, -170.0000000000000000, 91.80904905408446837 ) ) ;
#66155=CARTESIAN_POINT ( 'NONE',  ( 8.288451200428832877, 6.376395059685423305, 38.00660393953555172 ) ) ;
#66156=ORIENTED_EDGE ( 'NONE', *, *, #47078, .T. ) ;
#66158=CARTESIAN_POINT ( 'NONE',  ( -62.48965350618345838, 16.80247907725181733, -68.55831454992926410 ) ) ;
#66159=CARTESIAN_POINT ( 'NONE',  ( 130.9163507021337409, 39.67702886032468967, -90.30179768571910870 ) ) ;
#66163=CARTESIAN_POINT ( 'NONE',  ( 94.12811352634520290, 22.11743943276050928, 9.843555910658421837 ) ) ;
#66168=EDGE_CURVE ( 'NONE', #34548, #16719, #66673, .T. ) ;
#66169=EDGE_CURVE ( 'NONE', #15908, #29791, #61375, .T. ) ;
#66170=CARTESIAN_POINT ( 'NONE',  ( 68.80707543459442377, 15.13014033538981984, 86.22508746598937535 ) ) ;
#66172=CARTESIAN_POINT ( 'NONE',  ( -178.5750994113943761, 94.98114813978523330, -47.38438974541455195 ) ) ;
#66173=CARTESIAN_POINT ( 'NONE',  ( -179.7387526106833775, 96.39435599882348527, -92.36184407879430580 ) ) ;
#66174=CARTESIAN_POINT ( 'NONE',  ( -143.3263687017172288, 59.10892259956421668, -91.74752380608748581 ) ) ;
#66175=DIRECTION ( 'NONE',  ( 0.000000000000000000, 0.000000000000000000, 1.000000000000000000 ) ) ;
#66176=EDGE_CURVE ( 'NONE', #33459, #14549, #60358, .T. ) ;
#66178=CYLINDRICAL_SURFACE ( 'NONE', #41054, 7.500000000000013323 ) ;
#66180=ORIENTED_EDGE ( 'NONE', *, *, #22710, .F. ) ;
#66182=CARTESIAN_POINT ( 'NONE',  ( -155.1359377029286009, 70.46175948311802983, -37.33043500810457260 ) ) ;
#66183=DIRECTION ( 'NONE',  ( -0.000000000000000000, 1.000000000000000000, -0.000000000000000000 ) ) ;
#66184=CARTESIAN_POINT ( 'NONE',  ( -36.38071096718370967, 11.47804921491337993, 43.37945295078770158 ) ) ;
#66187=CARTESIAN_POINT ( 'NONE',  ( -12.85736381479377499, 7.270939470456537101, -91.02940243108859875 ) ) ;
#66190=CARTESIAN_POINT ( 'NONE',  ( -13.47517652744367034, 8.334971000693560228, 42.57234634832188647 ) ) ;
#66191=CARTESIAN_POINT ( 'NONE',  ( 111.1767565371974626, 29.31586421952251698, 2.810169317169238568 ) ) ;
#66192=CARTESIAN_POINT ( 'NONE',  ( -53.37047711001667949, 15.27679796346806640, -89.09340216910368326 ) ) ;
#66199=CARTESIAN_POINT ( 'NONE',  ( 46.42281973867196854, 9.426811321855158354, 66.90762843771246082 ) ) ;
#66206=CARTESIAN_POINT ( 'NONE',  ( -173.1211646369891355, 87.12891641440857882, -49.71195716475001092 ) ) ;
#66207=CARTESIAN_POINT ( 'NONE',  ( 39.40195752203891999, 9.424259417798142024, -62.46436805589144114 ) ) ;
#66211=CARTESIAN_POINT ( 'NONE',  ( 178.1999009735082495, 75.73911533785327777, 70.57996378539579041 ) ) ;
#66212=B_SPLINE_CURVE_WITH_KNOTS ( 'NONE', 3,
 ( #43670, #65147, #46111, #34886, #51409, #19037, #67583, #56324, #40838, #19382, #2520, #55988, #45778, #3220, #62297, #29945, #24677, #45425, #66905, #40491, #35219, #14108, #3550, #51056, #18700, #35570, #57030, #13083, #8845, #61942, #30295, #51744, #50703, #40155, #25021, #23973, #34547, #7802, #29252, #61607, #13422, #8142, #29586 ),
 .UNSPECIFIED., .F., .F.,
 ( 4, 2, 2, 2, 2, 2, 2, 2, 2, 2, 2, 2, 1, 2, 2, 2, 2, 2, 2, 2, 2, 4 ),
 ( 0.02379577142314830140, 0.02527778373276529794, 0.02601878988757378580, 0.02675979604238227366, 0.02824180835199925285, 0.02972382066161623204, 0.03046482681642473031, 0.03120583297123322858, 0.03268784528085023899, 0.03416985759046724247, 0.03565186990008424595, 0.03639287605489275462, 0.03713388220970126330, 0.03787488836450975810, 0.03861589451931826678, 0.04009790682893527719, 0.04157991913855228761, 0.04306193144816929802, 0.04380293760297780670, 0.04454394375778630843, 0.04602595606740331191, 0.04750796837702032926 ),
 .UNSPECIFIED. ) ;
#66220=CARTESIAN_POINT ( 'NONE',  ( 103.8325688302027174, 27.12251147381402561, -47.32372234173669057 ) ) ;
#66221=CARTESIAN_POINT ( 'NONE',  ( -10.23867141318106100, 7.059827648235816433, 57.34201402450064222 ) ) ;
#66222=CARTESIAN_POINT ( 'NONE',  ( 14.81290967676421921, 7.477658233646008235, 56.90665333537696569 ) ) ;
#66225=FACE_BOUND ( 'NONE', #27040, .T. ) ;
#66230=CARTESIAN_POINT ( 'NONE',  ( -179.5109681715917986, 96.11572638569519711, 7.512143929769561801 ) ) ;
#66231=CARTESIAN_POINT ( 'NONE',  ( 153.2282895792478996, 54.42637815496157572, 3.875255574263929859 ) ) ;
#66234=ORIENTED_EDGE ( 'NONE', *, *, #25519, .F. ) ;
#66235=CARTESIAN_POINT ( 'NONE',  ( 58.09607305250594322, 11.58497620657514915, 4.785656767381915699 ) ) ;
#66236=CARTESIAN_POINT ( 'NONE',  ( -62.15799747763099248, 16.70234469631020247, 62.20972612752362352 ) ) ;
#66239=EDGE_LOOP ( 'NONE', ( #44700, #843, #20335, #7035 ) ) ;
#66240=EDGE_CURVE ( 'NONE', #37469, #40902, #57487, .T. ) ;
#66243=DIRECTION ( 'NONE',  ( -0.000000000000000000, 1.000000000000000000, -0.000000000000000000 ) ) ;
#66246=CARTESIAN_POINT ( 'NONE',  ( 45.04020069093781586, 10.22779424730543241, 69.22824337619731239 ) ) ;
#66249=CARTESIAN_POINT ( 'NONE',  ( -156.9262190792699414, 72.10659547035876926, -68.01882500604709492 ) ) ;
#66250=CARTESIAN_POINT ( 'NONE',  ( 69.49112875363887554, 15.30845942322121367, 6.676346884528112646 ) ) ;
#66251=FACE_OUTER_BOUND ( 'NONE', #8220, .T. ) ;
#66255=CARTESIAN_POINT ( 'NONE',  ( 63.01563776193090405, 13.70579113808098271, -35.72069083216973695 ) ) ;
#66256=CARTESIAN_POINT ( 'NONE',  ( -131.2955621888335429, 51.38237199780172659, -20.79447557564050797 ) ) ;
#66258=CARTESIAN_POINT ( 'NONE',  ( 114.4640969196985907, 30.88424258798505306, -22.78190138875784143 ) ) ;
#66262=CARTESIAN_POINT ( 'NONE',  ( 91.48187668755954860, 21.13368548676794845, 85.14416980506385357 ) ) ;
#66269=CARTESIAN_POINT ( 'NONE',  ( 177.0110682437508274, 75.98481089748381123, 3.650247767581047409 ) ) ;
#66270=CARTESIAN_POINT ( 'NONE',  ( -50.51700111023805562, 13.51182830536852997, -9.878698120772499536 ) ) ;
#66271=CARTESIAN_POINT ( 'NONE',  ( 106.6228877857910646, 27.24245963308691998, -9.992007454249797860 ) ) ;
#66273=CARTESIAN_POINT ( 'NONE',  ( 211.0188980202574101, 117.2649575585887050, 94.44936189044236130 ) ) ;
#66274=DIRECTION ( 'NONE',  ( -0.000000000000000000, 1.000000000000000000, -0.000000000000000000 ) ) ;
#66279=ORIENTED_EDGE ( 'NONE', *, *, #46121, .T. ) ;
#66281=CARTESIAN_POINT ( 'NONE',  ( 63.49941241090381538, 13.81848793187418245, -23.87614024170608928 ) ) ;
#66282=CARTESIAN_POINT ( 'NONE',  ( 182.7686108735401262, 81.77235358504609053, -77.89035669591841327 ) ) ;
#66283=CARTESIAN_POINT ( 'NONE',  ( -167.6566265204789659, 82.70140535081091571, 43.46458241691903623 ) ) ;
#66288=CARTESIAN_POINT ( 'NONE',  ( -179.9997297618090784, -170.0000000000000000, 94.99999999999866418 ) ) ;
#66294=B_SPLINE_CURVE_WITH_KNOTS ( 'NONE', 3,
 ( #66819, #62566, #14379, #13342, #35833, #57286, #23551, #18614, #34799, #56237, #67171, #2781, #18959, #40405, #42810, #9442, #42476, #25632, #46722, #26651, #53017, #53360, #36516, #64278, #41796, #25967, #68195, #31250, #51999, #48086, #69544, #57971, #41455, #21363, #14711, #36865, #20000, #10460, #16086, #25283, #4505, #20331, #62907, #63253 ),
 .UNSPECIFIED., .F., .F.,
 ( 4, 2, 2, 2, 2, 2, 2, 2, 2, 2, 2, 2, 2, 2, 2, 2, 2, 2, 2, 2, 2, 4 ),
 ( 0.02495775893651561508, 0.02650251144344302479, 0.02804726395037043796, 0.02959201645729784766, 0.03113676896422525736, 0.03268152147115267053, 0.03345389772461636324, 0.03422627397808006289, 0.03577102648500746218, 0.03654340273847116877, 0.03731577899193487535, 0.03808815524539857500, 0.03886053149886228159, 0.04040528400578970170, 0.04117766025925340828, 0.04195003651271711487, 0.04349478901964453498, 0.04503954152657195509, 0.04581191778003566861, 0.04658429403349938214, 0.04812904654042685082, 0.04967379904735432644 ),
 .UNSPECIFIED. ) ;
#66295=DIRECTION ( 'NONE',  ( -0.000000000000000000, 1.000000000000000000, -0.000000000000000000 ) ) ;
#66296=CARTESIAN_POINT ( 'NONE',  ( -12.39701069459754201, 7.231688578592714300, 4.805392785045681237 ) ) ;
#66298=CARTESIAN_POINT ( 'NONE',  ( 93.23851390434869302, 22.85739692998905070, -93.44079555661757297 ) ) ;
#66302=CARTESIAN_POINT ( 'NONE',  ( 198.8732368717152212, 100.3103976497390875, 68.28400160539764840 ) ) ;
#66303=VERTEX_POINT ( 'NONE', #11010 ) ;
#66304=CARTESIAN_POINT ( 'NONE',  ( -57.42826130032241849, 16.37596353166460617, -76.67885148864655775 ) ) ;
#66305=CARTESIAN_POINT ( 'NONE',  ( 202.7506655727288774, 105.3943386412348815, -63.41604910222725522 ) ) ;
#66307=CARTESIAN_POINT ( 'NONE',  ( -180.4654253355437277, 95.69358270527506249, -43.76251724624543726 ) ) ;
#66309=CARTESIAN_POINT ( 'NONE',  ( -165.6398193834832000, 79.16932278174806470, 10.86641610212712905 ) ) ;
#66311=FACE_BOUND ( 'NONE', #64192, .T. ) ;
#66312=CARTESIAN_POINT ( 'NONE',  ( -189.2375912283856394, 107.0871308750787563, 91.70900086444785870 ) ) ;
#66313=ORIENTED_EDGE ( 'NONE', *, *, #4660, .T. ) ;
#66315=CARTESIAN_POINT ( 'NONE',  ( -132.6161619568759420, 51.08240647571223292, -72.59421541500523745 ) ) ;
#66319=CARTESIAN_POINT ( 'NONE',  ( 157.4703587214989113, 57.65129005721575339, 44.40946747225338953 ) ) ;
#66323=CARTESIAN_POINT ( 'NONE',  ( 187.8308247327058211, 85.70400899947037487, 93.79355304541221017 ) ) ;
#66326=EDGE_CURVE ( 'NONE', #17944, #67205, #35199, .T. ) ;
#66327=CARTESIAN_POINT ( 'NONE',  ( 176.6214367443247681, 74.20967084876664899, -37.67839354686518760 ) ) ;
#66328=CARTESIAN_POINT ( 'NONE',  ( -179.2262621278717631, 94.19039042964666919, -64.67118848797289843 ) ) ;
#66331=DIRECTION ( 'NONE',  ( -0.000000000000000000, 1.000000000000000000, -0.000000000000000000 ) ) ;
#66332=CARTESIAN_POINT ( 'NONE',  ( -180.2244609727085844, 95.39945930389649220, 9.053060466247467630 ) ) ;
#66335=DIRECTION ( 'NONE',  ( -0.000000000000000000, 1.000000000000000000, -0.000000000000000000 ) ) ;
#66336=CARTESIAN_POINT ( 'NONE',  ( -29.04400972079232091, 10.22852224114065223, -8.861140687333856292 ) ) ;
#66337=CARTESIAN_POINT ( 'NONE',  ( -53.14657859411973106, 15.21831473227210374, -8.614006834922252054 ) ) ;
#66338=EDGE_CURVE ( 'NONE', #4893, #10403, #13527, .T. ) ;
#66341=CARTESIAN_POINT ( 'NONE',  ( 110.2429982417149432, 28.88204397445229077, -35.92243756565368784 ) ) ;
#66343=EDGE_CURVE ( 'NONE', #52913, #65764, #11621, .T. ) ;
#66344=CARTESIAN_POINT ( 'NONE',  ( 46.90141780929662474, 9.503798448769774865, -43.62445339352620977 ) ) ;
#66347=CARTESIAN_POINT ( 'NONE',  ( -124.8192061951466485, 45.78944360187998086, 84.36447601993580747 ) ) ;
#66348=ORIENTED_EDGE ( 'NONE', *, *, #10065, .F. ) ;
#66349=CARTESIAN_POINT ( 'NONE',  ( 79.82127737190242556, 17.20935440217363421, -46.47800199947357669 ) ) ;
#66350=VECTOR ( 'NONE', #49801, 1000.000000000000000 ) ;
#66352=CARTESIAN_POINT ( 'NONE',  ( -126.7989199172159829, 47.09198523267866676, 30.66070955475667148 ) ) ;
#66353=CARTESIAN_POINT ( 'NONE',  ( 79.54836217416617217, 18.17815803851262402, 34.72743815142386836 ) ) ;
#66358=CARTESIAN_POINT ( 'NONE',  ( -180.0154536325057109, 96.73346874014735874, -12.40038597180966917 ) ) ;
#66362=CARTESIAN_POINT ( 'NONE',  ( 39.40195752203892710, 8.409560354027384221, 44.91383430596327742 ) ) ;
#66365=CARTESIAN_POINT ( 'NONE',  ( 208.9583973663597476, 114.1615900753670445, -50.01439015974929703 ) ) ;
#66367=CARTESIAN_POINT ( 'NONE',  ( -109.5025362253418280, 36.60371748273997383, 66.95027869359381612 ) ) ;
#66368=CARTESIAN_POINT ( 'NONE',  ( -23.93965512371324067, 8.480096402797094868, -43.32224293081845445 ) ) ;
#66372=ORIENTED_EDGE ( 'NONE', *, *, #22596, .F. ) ;
#66373=EDGE_LOOP ( 'NONE', ( #68720, #60805, #30432, #924 ) ) ;
#66375=DIRECTION ( 'NONE',  ( 0.000000000000000000, 0.000000000000000000, 1.000000000000000000 ) ) ;
#66376=CARTESIAN_POINT ( 'NONE',  ( -86.17927900504984962, 25.32700542568493418, 64.77477121631265788 ) ) ;
#66377=B_SPLINE_CURVE_WITH_KNOTS ( 'NONE', 3,
 ( #48267, #10999, #21549, #32461, #53894, #5716, #27172, #68378, #63092, #38430, #50028, #55649, #54948, #65522, #16959, #28215, #17317, #49316, #59873, #60235, #60581, #1147, #6769, #39474, #11690, #33164, #23313, #43348, #43690, #12049, #27520, #17678, #44040, #66235, #7483, #48607, #12749, #32808, #28575, #39143, #38791, #44760, #445, #22953 ),
 .UNSPECIFIED., .F., .F.,
 ( 4, 2, 2, 2, 2, 2, 2, 2, 2, 2, 2, 2, 2, 2, 2, 2, 2, 2, 2, 2, 2, 4 ),
 ( 1.471961680016038988E-17, 0.001482469635030012013, 0.002223704452545010972, 0.002964939270060010582, 0.004447408905090008933, 0.005929878540120007285, 0.007412348175150002168, 0.008153582992665003512, 0.008894817810180005724, 0.01037728744521001709, 0.01185975708024002845, 0.01260099189775503760, 0.01334222671527004501, 0.01482469635030006158, 0.01556593116781506379, 0.01630716598533006600, 0.01778963562036006349, 0.01927210525539005403, 0.02001334007290505104, 0.02075457489042004805, 0.02223704452545005941, 0.02371951416048007424 ),
 .UNSPECIFIED. ) ;
#66378=FACE_OUTER_BOUND ( 'NONE', #10236, .T. ) ;
#66379=LINE ( 'NONE', #39281, #13082 ) ;
#66382=CARTESIAN_POINT ( 'NONE',  ( -97.86516199987806885, 31.71158167298307617, -21.75180431999427810 ) ) ;
#66383=CARTESIAN_POINT ( 'NONE',  ( 38.42384008295177722, 8.283891555743466029, 71.71024313779651038 ) ) ;
#66384=CARTESIAN_POINT ( 'NONE',  ( 32.99392442438140449, 7.662387294680161887, 94.99999999999866418 ) ) ;
#66387=VERTEX_POINT ( 'NONE', #50397 ) ;
#66388=CARTESIAN_POINT ( 'NONE',  ( 59.94652978725887493, 13.01168383647461546, 71.00508481107152647 ) ) ;
#66390=CARTESIAN_POINT ( 'NONE',  ( -10.24974837193994404, 8.069704751038628388, 17.88514665569731577 ) ) ;
#66394=CARTESIAN_POINT ( 'NONE',  ( 126.3580464630938422, 38.22944795020838882, -16.97937654421329867 ) ) ;
#66397=CARTESIAN_POINT ( 'NONE',  ( -189.2346268516247392, 107.0830361517165130, -15.05455062662797339 ) ) ;
#66398=CARTESIAN_POINT ( 'NONE',  ( -33.38294402636582703, 10.93918551420889784, -35.55683350427927536 ) ) ;
#66402=CARTESIAN_POINT ( 'NONE',  ( -165.9814687844695129, 79.51750121246506353, 94.33608907707005642 ) ) ;
#66405=CARTESIAN_POINT ( 'NONE',  ( -143.2471548081023229, 59.04577938365769540, -19.63009637662464613 ) ) ;
#66409=DIRECTION ( 'NONE',  ( 0.000000000000000000, 0.000000000000000000, 1.000000000000000000 ) ) ;
#66414=CARTESIAN_POINT ( 'NONE',  ( -149.5074843970971017, 65.50121172469319220, 30.72082123989904545 ) ) ;
#66415=CARTESIAN_POINT ( 'NONE',  ( 19.53470118933706701, 6.649487981843462236, -49.52081999872682161 ) ) ;
#66416=CARTESIAN_POINT ( 'NONE',  ( 116.9197133427647231, 33.22079464767577406, 6.812707058480746092 ) ) ;
#66417=EDGE_LOOP ( 'NONE', ( #28495, #23004, #52535, #63011 ) ) ;
#66418=CARTESIAN_POINT ( 'NONE',  ( 60.62939143133408493, 12.13148391928981162, 30.18601119527468413 ) ) ;
#66425=CARTESIAN_POINT ( 'NONE',  ( -13.45956523846224684, 8.333781915634247639, -74.71914061966306519 ) ) ;
#66430=CARTESIAN_POINT ( 'NONE',  ( -71.17984086584780812, 20.67393782512344558, -42.10050417024042702 ) ) ;
#66435=AXIS2_PLACEMENT_3D ( 'NONE', #21194, #20841, #42640 ) ;
#66436=CARTESIAN_POINT ( 'NONE',  ( 139.6326990672751549, 46.22017155708127945, 32.21984060566606445 ) ) ;
#66437=CARTESIAN_POINT ( 'NONE',  ( -178.5848962563134137, 94.99295350784005620, 43.48377260447168879 ) ) ;
#66439=CARTESIAN_POINT ( 'NONE',  ( 17.72748965151694023, 7.577488030789626627, 71.60839833991708758 ) ) ;
#66444=CARTESIAN_POINT ( 'NONE',  ( 211.5877208647112866, 116.2968205280715637, -94.50629413778540311 ) ) ;
#66445=CARTESIAN_POINT ( 'NONE',  ( -32.41627406084105445, 9.753381371531506971, -35.36528594626865640 ) ) ;
#66446=CARTESIAN_POINT ( 'NONE',  ( -95.42918619675315028, 29.43458666617156183, 88.58648633754481239 ) ) ;
#66447=CARTESIAN_POINT ( 'NONE',  ( -142.0081215801269821, 58.07066293384867350, 37.92100431141785322 ) ) ;
#66448=CARTESIAN_POINT ( 'NONE',  ( -133.1527834403229917, 51.46311219732124442, 66.86934462543963775 ) ) ;
#66449=CARTESIAN_POINT ( 'NONE',  ( -75.65611349188964141, 22.26947559308020175, -22.64443753553979377 ) ) ;
#66450=ORIENTED_EDGE ( 'NONE', *, *, #67137, .F. ) ;
#66451=CARTESIAN_POINT ( 'NONE',  ( 86.62931800182293784, 19.42108912189599579, 71.55663816294304524 ) ) ;
#66453=CARTESIAN_POINT ( 'NONE',  ( -94.91535552559176381, 30.30508792700360488, -94.76622093189627094 ) ) ;
#66454=CARTESIAN_POINT ( 'NONE',  ( 184.3994103300443612, 82.02159554764421046, 43.55099592434475397 ) ) ;
#66458=CARTESIAN_POINT ( 'NONE',  ( -10.23531775138760835, 8.068923942586303966, -50.02458151933852548 ) ) ;
#66462=CARTESIAN_POINT ( 'NONE',  ( -106.6583005646425732, 35.06113698500919895, -90.11032198025695550 ) ) ;
#66464=DIRECTION ( 'NONE',  ( 0.000000000000000000, 0.000000000000000000, 1.000000000000000000 ) ) ;
#66469=CARTESIAN_POINT ( 'NONE',  ( -11.57931195747592312, 7.164335452024273465, -63.25124850868342463 ) ) ;
#66470=CARTESIAN_POINT ( 'NONE',  ( -36.37663950036512261, 10.45389057208229033, 43.38300827802142834 ) ) ;
#66471=CARTESIAN_POINT ( 'NONE',  ( 139.3067271572849677, 44.81402783181199823, -38.36495864216608709 ) ) ;
#66477=CARTESIAN_POINT ( 'NONE',  ( 35.44311777160621091, 8.940232499250166498, -9.900466562469301124 ) ) ;
#66479=CIRCLE ( 'NONE', #30504, 242.4895526022646379 ) ;
#66480=CARTESIAN_POINT ( 'NONE',  ( -1.327237339235001645, 7.561837009978233048, 68.21302253756950051 ) ) ;
#66485=DIRECTION ( 'NONE',  ( -0.000000000000000000, 1.000000000000000000, -0.000000000000000000 ) ) ;
#66487=CARTESIAN_POINT ( 'NONE',  ( -124.3331814159187303, 45.47486189329072914, -76.59758970666941025 ) ) ;
#66489=CARTESIAN_POINT ( 'NONE',  ( 162.0835148203877054, 61.32844276806160622, -22.71226385295197048 ) ) ;
#66497=LINE ( 'NONE', #50638, #2509 ) ;
#66498=CARTESIAN_POINT ( 'NONE',  ( -149.5074843970971301, -170.0000000000000000, 38.22082123989905966 ) ) ;
#66500=CARTESIAN_POINT ( 'NONE',  ( 66.73467315386237431, 14.60276727483218018, 70.68858689679898077 ) ) ;
#66504=CARTESIAN_POINT ( 'NONE',  ( 163.2911130186310800, 63.63047778106600560, -38.88797379336740789 ) ) ;
#66506=CARTESIAN_POINT ( 'NONE',  ( 157.4703587214989113, 57.65129005721575339, -36.12418429913763163 ) ) ;
#66509=CARTESIAN_POINT ( 'NONE',  ( 70.52174251456412435, 15.58109049973242932, 90.85735943127390613 ) ) ;
#66510=CARTESIAN_POINT ( 'NONE',  ( 32.03384598935271299, 8.576372641735984459, 38.87696540156872516 ) ) ;
#66511=CARTESIAN_POINT ( 'NONE',  ( -175.1895962157336726, 90.99110972060687175, -49.43342400943532766 ) ) ;
#66512=CARTESIAN_POINT ( 'NONE',  ( -131.7724154034330297, 50.48821165954356616, -10.90495122044228182 ) ) ;
#66513=CARTESIAN_POINT ( 'NONE',  ( 152.3102623290679674, 53.74757787434987222, 69.20218478440308729 ) ) ;
#66515=CARTESIAN_POINT ( 'NONE',  ( 129.4987365823222092, 38.85470922756775281, -76.47662530583420448 ) ) ;
#66517=CARTESIAN_POINT ( 'NONE',  ( 137.4031600461560458, 44.79620770172218869, -76.98055282418557965 ) ) ;
#66518=CARTESIAN_POINT ( 'NONE',  ( -13.45956523846224684, 8.333781915634252968, 59.50361233265537919 ) ) ;
#66520=VECTOR ( 'NONE', #65429, 1000.000000000000000 ) ;
#66521=CARTESIAN_POINT ( 'NONE',  ( -152.9143627383494959, 68.46626892668653852, -35.61578214405540876 ) ) ;
#66525=CARTESIAN_POINT ( 'NONE',  ( -123.6618353044033967, 46.23845779494347852, -49.58867574490025731 ) ) ;
#66526=CARTESIAN_POINT ( 'NONE',  ( -6.125624616441582404, 7.794071945221087816, 44.92450289403895169 ) ) ;
#66528=CARTESIAN_POINT ( 'NONE',  ( -47.68743014591520080, 12.82957810971108259, -68.08236959171381386 ) ) ;
#66529=CARTESIAN_POINT ( 'NONE',  ( -1.455067768715152310, 7.566780179921178906, -12.10745439085062714 ) ) ;
#66531=CARTESIAN_POINT ( 'NONE',  ( -11.78188048797445475, 8.190559674012726887, 31.23928352507218165 ) ) ;
#66533=CARTESIAN_POINT ( 'NONE',  ( 112.5554747942045992, 29.96654954475020460, 3.128152278745223835 ) ) ;
#66534=EDGE_LOOP ( 'NONE', ( #69357, #4692 ) ) ;
#66535=CARTESIAN_POINT ( 'NONE',  ( -95.05323930133205579, 30.36974142673411592, -40.44390620904788136 ) ) ;
#66537=CARTESIAN_POINT ( 'NONE',  ( 105.4375968828853587, 26.72149058755206141, -64.50356492661067875 ) ) ;
#66539=CARTESIAN_POINT ( 'NONE',  ( 39.89582146299186860, 9.488756994579086168, -8.775266874964069430 ) ) ;
#66540=CARTESIAN_POINT ( 'NONE',  ( 43.97326221476411945, 9.047815246749991047, 70.22452885316067750 ) ) ;
#66544=DIRECTION ( 'NONE',  ( 0.000000000000000000, 0.000000000000000000, 1.000000000000000000 ) ) ;
#66545=EDGE_CURVE ( 'NONE', #49086, #20757, #15005, .T. ) ;
#66546=FACE_OUTER_BOUND ( 'NONE', #26760, .T. ) ;
#66547=CARTESIAN_POINT ( 'NONE',  ( -166.3175803736862690, 79.86140754556167565, 68.33441179371222063 ) ) ;
#66551=CARTESIAN_POINT ( 'NONE',  ( 174.9053416555736646, 72.57849647436444229, 59.37145172503423396 ) ) ;
#66554=CARTESIAN_POINT ( 'NONE',  ( 107.9342863085848165, 28.93180871323605885, 56.80434494465688999 ) ) ;
#66555=CARTESIAN_POINT ( 'NONE',  ( -169.1122507277982834, 84.24359299875007423, -21.72154401521961020 ) ) ;
#66556=DIRECTION ( 'NONE',  ( -0.000000000000000000, 1.000000000000000000, -0.000000000000000000 ) ) ;
#66557=ORIENTED_EDGE ( 'NONE', *, *, #13276, .T. ) ;
#66558=CARTESIAN_POINT ( 'NONE',  ( 104.3759779378692656, 27.35691041569132764, -38.72384540243022144 ) ) ;
#66559=CARTESIAN_POINT ( 'NONE',  ( 17.72748965151693312, 7.577488030789625739, -35.76980402193765940 ) ) ;
#66563=FACE_BOUND ( 'NONE', #52324, .T. ) ;
#66570=CARTESIAN_POINT ( 'NONE',  ( 32.03384598935269878, 8.576372641736000446, -68.50123696028599340 ) ) ;
#66571=DIRECTION ( 'NONE',  ( 0.000000000000000000, 0.000000000000000000, 1.000000000000000000 ) ) ;
#66573=CARTESIAN_POINT ( 'NONE',  ( 208.0306608271317543, 112.7988899307265598, 56.83016791471741413 ) ) ;
#66574=CARTESIAN_POINT ( 'NONE',  ( 81.76092782665035941, 17.81692437267514251, -64.45568945875886868 ) ) ;
#66575=VECTOR ( 'NONE', #49520, 1000.000000000000000 ) ;
#66581=LINE ( 'NONE', #2895, #57621 ) ;
#66583=CARTESIAN_POINT ( 'NONE',  ( -85.75222301046100881, 25.14826148333819944, -66.95125014471969394 ) ) ;
#66584=FACE_OUTER_BOUND ( 'NONE', #15475, .T. ) ;
#66585=EDGE_CURVE ( 'NONE', #48880, #68633, #25117, .T. ) ;
#66589=EDGE_CURVE ( 'NONE', #34631, #44954, #32044, .T. ) ;
#66590=CARTESIAN_POINT ( 'NONE',  ( 164.8433205901838789, 64.93586312665799198, 38.31213353503791552 ) ) ;
#66592=CARTESIAN_POINT ( 'NONE',  ( 107.0447263249840972, 28.53200276018955250, 17.05477231794132109 ) ) ;
#66595=CARTESIAN_POINT ( 'NONE',  ( -47.56466076048272384, 13.83435953640667293, 10.48194178115690534 ) ) ;
#66596=CARTESIAN_POINT ( 'NONE',  ( -129.4036885357273547, 50.06837984316181434, -8.937056684793262207 ) ) ;
#66597=CARTESIAN_POINT ( 'NONE',  ( -152.2894885175273032, 67.91392929472267781, -89.02504389548720098 ) ) ;
#66600=DIRECTION ( 'NONE',  ( -0.000000000000000000, 1.000000000000000000, -0.000000000000000000 ) ) ;
#66604=LINE ( 'NONE', #3265, #35824 ) ;
#66605=CARTESIAN_POINT ( 'NONE',  ( 179.0091171455098333, 77.94933395983137814, 2.743929071994786639 ) ) ;
#66607=DIRECTION ( 'NONE',  ( -1.000000000000000000, 0.000000000000000000, 0.000000000000000000 ) ) ;
#66609=CARTESIAN_POINT ( 'NONE',  ( 199.7415218581341776, 101.4249224381273535, 84.75794127139820944 ) ) ;
#66611=CARTESIAN_POINT ( 'NONE',  ( -73.81689110552358102, 20.53332132481498817, -75.18638386565793041 ) ) ;
#66613=ORIENTED_EDGE ( 'NONE', *, *, #23919, .T. ) ;
#66618=CARTESIAN_POINT ( 'NONE',  ( 188.4365915667138722, 87.87248959723055464, -69.06054871186299238 ) ) ;
#66619=CARTESIAN_POINT ( 'NONE',  ( -38.80556650104458072, 11.94251439360623124, 89.95992065018027972 ) ) ;
#66620=CARTESIAN_POINT ( 'NONE',  ( -99.11448999425216755, 31.20120877265620507, -49.32994709144890066 ) ) ;
#66621=CARTESIAN_POINT ( 'NONE',  ( -102.2801239173131052, 32.78103895658058065, 3.674523915951417141 ) ) ;
#66623=CARTESIAN_POINT ( 'NONE',  ( 137.5911612413395630, 44.91497189902067788, -10.17040840536950341 ) ) ;
#66624=ORIENTED_EDGE ( 'NONE', *, *, #25721, .F. ) ;
#66628=CARTESIAN_POINT ( 'NONE',  ( 187.4794072207230897, 86.81249290409115815, 94.43195144249413886 ) ) ;
#66631=CARTESIAN_POINT ( 'NONE',  ( 56.66775172211441003, 11.28938863449062069, -12.37422088483766736 ) ) ;
#66635=ORIENTED_EDGE ( 'NONE', *, *, #35023, .T. ) ;
#66636=CARTESIAN_POINT ( 'NONE',  ( 42.03719354205841086, 9.783015072457470040, -62.93830268630524927 ) ) ;
#66638=CARTESIAN_POINT ( 'NONE',  ( 197.9868529032976312, 99.18611233336802968, -74.03116428711561525 ) ) ;
#66640=CARTESIAN_POINT ( 'NONE',  ( -174.7869898116916545, 88.99756909636809610, -34.85054195857060222 ) ) ;
#66642=CARTESIAN_POINT ( 'NONE',  ( -167.9889421625799741, 81.59140042431232587, 5.987724995526459537 ) ) ;
#66644=FACE_BOUND ( 'NONE', #14424, .T. ) ;
#66649=CARTESIAN_POINT ( 'NONE',  ( -99.01681023176691099, 31.15382287136410966, -89.44744109731372816 ) ) ;
#66651=VERTEX_POINT ( 'NONE', #65807 ) ;
#66652=B_SPLINE_CURVE_WITH_KNOTS ( 'NONE', 3,
 ( #65121, #48218, #59822, #54547, #10950, #48913, #60537, #751, #21849, #16917, #43293, #11637, #38737, #32068, #1099, #27123, #60181, #59477, #26792, #43 ),
 .UNSPECIFIED., .F., .F.,
 ( 4, 2, 2, 2, 2, 2, 2, 2, 2, 4 ),
 ( 0.000000000000000000, 0.001349456565742324261, 0.002024184848613473382, 0.002698913131484622502, 0.004048369697226901660, 0.005397826262969181686, 0.006747282828711460845, 0.008096739394453740871, 0.009446195960196020897, 0.01079565252593830092 ),
 .UNSPECIFIED. ) ;
#66654=CARTESIAN_POINT ( 'NONE',  ( 150.5538013146980632, 53.70974888488129295, 66.66635342088143545 ) ) ;
#66658=ORIENTED_EDGE ( 'NONE', *, *, #17306, .F. ) ;
#66659=CARTESIAN_POINT ( 'NONE',  ( -127.9486647835774420, 47.86116766339740991, -88.87777986370316796 ) ) ;
#66660=CARTESIAN_POINT ( 'NONE',  ( -7.825402957745085430, -170.0000000000000000, -50.41807073194384259 ) ) ;
#66665=CARTESIAN_POINT ( 'NONE',  ( 150.0516754638056511, 53.34587188591232376, 35.77407304044231751 ) ) ;
#66668=CARTESIAN_POINT ( 'NONE',  ( 116.6681538161788723, 33.09439081574001307, 60.05510480527172490 ) ) ;
#66670=CARTESIAN_POINT ( 'NONE',  ( -0.3747453031323939587, 6.520267647591904137, 9.782624009045733260 ) ) ;
#66673=LINE ( 'NONE', #34309, #24773 ) ;
#66674=EDGE_CURVE ( 'NONE', #68287, #59320, #40182, .T. ) ;
#66675=CARTESIAN_POINT ( 'NONE',  ( -25.07901552294942960, 9.649193085547777216, -11.99012566281456493 ) ) ;
#66681=CARTESIAN_POINT ( 'NONE',  ( 117.6916924104495479, 32.48309187151379973, -42.40661573811005525 ) ) ;
#66683=CARTESIAN_POINT ( 'NONE',  ( -75.43271753227891452, 22.18711452892411629, 17.85784068024286952 ) ) ;
#66684=CARTESIAN_POINT ( 'NONE',  ( 46.13320811200731697, 9.380653113584038749, -46.46381765439975453 ) ) ;
#66685=CARTESIAN_POINT ( 'NONE',  ( -169.8885678771097787, 85.07765565657315676, -75.83859972875634980 ) ) ;
#66689=VECTOR ( 'NONE', #17449, 1000.000000000000000 ) ;
#66695=CARTESIAN_POINT ( 'NONE',  ( 141.0804878838241336, 45.96076546397618756, -14.59318871261416284 ) ) ;
#66697=CARTESIAN_POINT ( 'NONE',  ( 15.78827728214693416, 7.507518794609596924, -89.20804527961313113 ) ) ;
#66698=CARTESIAN_POINT ( 'NONE',  ( -152.2964402771108894, 66.58174574061953876, -35.34709794641883462 ) ) ;
#66701=CARTESIAN_POINT ( 'NONE',  ( 106.6192711434718916, 27.24117154335862523, 57.38488479179707724 ) ) ;
#66704=CARTESIAN_POINT ( 'NONE',  ( 67.55134213333076332, 13.77030723107740684, -22.36941340431874892 ) ) ;
#66706=CARTESIAN_POINT ( 'NONE',  ( -109.3432140528234697, 36.51591785955880454, 67.43805915958625974 ) ) ;
#66707=DIRECTION ( 'NONE',  ( -0.000000000000000000, 1.000000000000000000, -0.000000000000000000 ) ) ;
#66709=ORIENTED_EDGE ( 'NONE', *, *, #14595, .F. ) ;
#66710=ORIENTED_EDGE ( 'NONE', *, *, #34346, .F. ) ;
#66712=CYLINDRICAL_SURFACE ( 'NONE', #29647, 7.500000000000020428 ) ;
#66715=CARTESIAN_POINT ( 'NONE',  ( -74.08448404088061068, 20.62888684035922893, 85.66122281550805440 ) ) ;
#66719=DIRECTION ( 'NONE',  ( -0.000000000000000000, 1.000000000000000000, -0.000000000000000000 ) ) ;
#66722=VECTOR ( 'NONE', #24332, 1000.000000000000000 ) ;
#66723=CARTESIAN_POINT ( 'NONE',  ( 62.52762183777209515, 13.59210632617625336, 44.81296093922131263 ) ) ;
#66724=CARTESIAN_POINT ( 'NONE',  ( 32.03309158115232691, 7.565157987341259549, 92.53824449203030156 ) ) ;
#66729=CARTESIAN_POINT ( 'NONE',  ( -11.57950265606958062, 8.174070387114795722, 17.26848926542448126 ) ) ;
#66731=CARTESIAN_POINT ( 'NONE',  ( -143.3925773749111841, 59.16144459815139101, 15.72631132447487445 ) ) ;
#66733=CARTESIAN_POINT ( 'NONE',  ( -62.41990535723909517, 16.78139727964023109, -95.00000000000133582 ) ) ;
#66734=CARTESIAN_POINT ( 'NONE',  ( -109.6660553119434951, 36.69391917620600907, -68.03064822489363905 ) ) ;
#66736=CARTESIAN_POINT ( 'NONE',  ( 133.8566784816069060, 42.60093787723653236, -24.17876034193199786 ) ) ;
#66737=CIRCLE ( 'NONE', #36383, 243.4957430088094839 ) ;
#66743=CARTESIAN_POINT ( 'NONE',  ( -189.7987719395349302, 107.8653664616570751, -12.38560667400269466 ) ) ;
#66748=CARTESIAN_POINT ( 'NONE',  ( -121.1775535805057018, 43.46577565517551278, -36.56175226999291539 ) ) ;
#66750=CARTESIAN_POINT ( 'NONE',  ( -0.5658006089934851657, 7.533733779014712084, -71.70916268580941733 ) ) ;
#66751=CARTESIAN_POINT ( 'NONE',  ( 150.9302598651331664, 53.98378566185801475, 86.91002861488426845 ) ) ;
#66753=CARTESIAN_POINT ( 'NONE',  ( 159.9814610548901328, 60.91953805293818647, -90.23667429834375753 ) ) ;
#66755=CARTESIAN_POINT ( 'NONE',  ( -156.4966862384868875, 71.70877417666513054, 40.99359700224837155 ) ) ;
#66757=CARTESIAN_POINT ( 'NONE',  ( -78.66644367742111399, -170.0000000000000000, -23.27090004125422595 ) ) ;
#66759=B_SPLINE_CURVE_WITH_KNOTS ( 'NONE', 3,
 ( #283, #49501, #1339, #55137, #10844, #59373, #60066, #12246, #22442, #66078, #6258, #59027, #17868, #32649, #27360, #6962, #33709, #49155, #16473, #38623, #44233, #644, #28412, #32315, #48802, #22096, #17148, #17507, #49862, #48448, #11185, #53743, #5900, #43190, #43538, #54793, #11525, #22793, #54433, #16808, #37927, #5565, #27019, #38267 ),
 .UNSPECIFIED., .F., .F.,
 ( 4, 2, 2, 2, 2, 2, 2, 2, 2, 2, 2, 2, 2, 2, 2, 2, 2, 2, 2, 2, 2, 4 ),
 ( 0.02638217555535139758, 0.02805347641364865779, 0.02972477727194591801, 0.03139607813024317823, 0.03306737898854043844, 0.03390302941768908590, 0.03473867984683773336, 0.03640998070513500051, 0.03724563113428361327, 0.03808128156343221909, 0.03891693199258083186, 0.03975258242172943768, 0.04058823285087805044, 0.04142388328002666320, 0.04225953370917527596, 0.04309518413832388872, 0.04476648499662110037, 0.04643778585491830507, 0.04810908671321550978, 0.04978038757151272142, 0.05145168842980993307, 0.05312298928810713777 ),
 .UNSPECIFIED. ) ;
#66761=CARTESIAN_POINT ( 'NONE',  ( 55.51547041749726219, 11.05727559334826715, 37.07079845792744521 ) ) ;
#66762=ORIENTED_EDGE ( 'NONE', *, *, #43755, .F. ) ;
#66763=ORIENTED_EDGE ( 'NONE', *, *, #34722, .T. ) ;
#66764=CARTESIAN_POINT ( 'NONE',  ( 173.7263186949344060, 72.85225335320953377, 35.32616919366697772 ) ) ;
#66767=CARTESIAN_POINT ( 'NONE',  ( 22.89234820949994287, 6.832052815347871899, -72.28072174863926591 ) ) ;
#66769=CARTESIAN_POINT ( 'NONE',  ( -9.779603649692306888, 8.034615131607074190, -62.50484457767164770 ) ) ;
#66776=CARTESIAN_POINT ( 'NONE',  ( 176.7247530015161772, 75.70727164389336394, -91.29928768740779788 ) ) ;
#66779=CARTESIAN_POINT ( 'NONE',  ( 139.6150621148398443, 46.20856238844174158, 41.84163371379585783 ) ) ;
#66780=CARTESIAN_POINT ( 'NONE',  ( 116.6436511186860798, 33.08230081168869674, 41.02847515960270641 ) ) ;
#66782=CARTESIAN_POINT ( 'NONE',  ( 130.7260570116704343, 40.73146260246713268, 70.68603471735700339 ) ) ;
#66783=CARTESIAN_POINT ( 'NONE',  ( 21.74799039132243905, 7.772294950329605712, 68.93910645723609321 ) ) ;
#66786=EDGE_LOOP ( 'NONE', ( #41562, #61638, #45001, #37051 ) ) ;
#66789=DIRECTION ( 'NONE',  ( 0.000000000000000000, 0.000000000000000000, 1.000000000000000000 ) ) ;
#66790=CARTESIAN_POINT ( 'NONE',  ( -96.26904753919785662, 29.83064565795647027, 87.21136816703879902 ) ) ;
#66794=CARTESIAN_POINT ( 'NONE',  ( -71.15374617000809110, 20.66492714610672721, -15.76073736046750717 ) ) ;
#66797=CARTESIAN_POINT ( 'NONE',  ( -102.2801239173131052, 33.91021738430207932, 30.51907450641510522 ) ) ;
#66807=CARTESIAN_POINT ( 'NONE',  ( -8.800520192024523070, 7.964629484975262130, -50.37068912721758096 ) ) ;
#66808=CARTESIAN_POINT ( 'NONE',  ( 151.7819978880463623, 53.35998893001568177, -48.51851982015085696 ) ) ;
#66812=VERTEX_POINT ( 'NONE', #8796 ) ;
#66818=CARTESIAN_POINT ( 'NONE',  ( 156.5890478960376413, 58.24007662587944623, -63.00753038278813989 ) ) ;
#66819=CARTESIAN_POINT ( 'NONE',  ( -102.2801239173131052, 32.78103895658057354, -23.17002667451225406 ) ) ;
#66820=CARTESIAN_POINT ( 'NONE',  ( -31.43908319763710679, 9.591432048623762086, 72.06100499665289760 ) ) ;
#66825=CARTESIAN_POINT ( 'NONE',  ( -118.4622862908119032, 41.79153065058248018, 39.16645702020448994 ) ) ;
#66828=CARTESIAN_POINT ( 'NONE',  ( 182.5617509987553433, 80.11195108039726165, 2.607952352358541948 ) ) ;
#66830=CARTESIAN_POINT ( 'NONE',  ( -6.125624616441583292, 7.794071945221086040, 18.07995230357528982 ) ) ;
#66832=AXIS2_PLACEMENT_3D ( 'NONE', #50530, #44558, #8319 ) ;
#66833=B_SPLINE_CURVE_WITH_KNOTS ( 'NONE', 3,
 ( #25981, #31947, #59691, #32633, #43170, #37910, #64646, #54059, #4519, #59010, #36883, #69559, #5546, #42823, #27001, #59356, #5885, #58318, #10827, #48430, #5209, #266, #69220, #38248, #47414, #10137, #68868, #27343, #48781, #26665, #32294, #31265, #48101, #52693, #20691, #21722, #21380, #22077, #53725, #43518, #64997, #16790, #42151, #63613, #4860, #15423, #42495, #31595, #53035, #26326, #21047, #63951, #37210, #58660, #53377, #38964, #18542, #49485, #28044, #44922 ),
 .UNSPECIFIED., .F., .F.,
 ( 4, 2, 2, 2, 2, 2, 2, 2, 2, 2, 2, 2, 2, 2, 2, 2, 2, 2, 2, 2, 2, 2, 2, 2, 2, 2, 2, 2, 2, 4 ),
 ( 0.000000000000000000, 0.001056649052740852267, 0.002113298105481704534, 0.003169947158222556367, 0.003698271684592982500, 0.004226596210963409067, 0.005283245263704308171, 0.006339894316445206408, 0.007396543369186105513, 0.008453192421927005484, 0.01056649052740882798, 0.01162313958014971234, 0.01267978863289059670, 0.01479308673837232031, 0.01690638484385404566, 0.01796303389659492308, 0.01901968294933580050, 0.02113298105481760739, 0.02218963010755855073, 0.02324627916029949753, 0.02535957726578140156, 0.02641622631852235531, 0.02747287537126330906, 0.02852952442400426281, 0.02958617347674521655, 0.03011449800311571598, 0.03064282252948621887, 0.03169947158222722466, 0.03275612063496822352, 0.03381276968770922930 ),
 .UNSPECIFIED. ) ;
#66839=ORIENTED_EDGE ( 'NONE', *, *, #8191, .F. ) ;
#66842=CARTESIAN_POINT ( 'NONE',  ( 70.02892116572940040, 14.40944430928137088, 66.82692659502507126 ) ) ;
#66843=CARTESIAN_POINT ( 'NONE',  ( 139.6359093656973869, 45.02518919224744565, -65.58120096399879628 ) ) ;
#66846=DIRECTION ( 'NONE',  ( -0.000000000000000000, 1.000000000000000000, -0.000000000000000000 ) ) ;
#66852=CARTESIAN_POINT ( 'NONE',  ( 164.4761273435911733, 64.62485394454745347, -46.35385866967215662 ) ) ;
#66853=CYLINDRICAL_SURFACE ( 'NONE', #42577, 7.500000000000020428 ) ;
#66855=CARTESIAN_POINT ( 'NONE',  ( 158.3604774538084712, 58.34594647925807465, -36.16383203810991631 ) ) ;
#66857=CARTESIAN_POINT ( 'NONE',  ( -95.52093927227215886, 30.58993121475387866, 14.43474828004453236 ) ) ;
#66858=CARTESIAN_POINT ( 'NONE',  ( 63.69010119909405887, 13.86368654881940188, 83.52517702392452748 ) ) ;
#66861=CARTESIAN_POINT ( 'NONE',  ( 84.72546926745363294, 19.84015517905183401, -9.206688192610737786 ) ) ;
#66862=CARTESIAN_POINT ( 'NONE',  ( -126.3508039230932525, 46.79479538767115798, -8.069153307770244865 ) ) ;
#66863=CARTESIAN_POINT ( 'NONE',  ( 37.36156881963844256, 9.166256500377349070, -89.57976542891690031 ) ) ;
#66864=CARTESIAN_POINT ( 'NONE',  ( 129.6961120139403363, 38.96846414226715893, -76.61255697058514613 ) ) ;
#66867=CARTESIAN_POINT ( 'NONE',  ( -15.13464256769235838, 8.488509377255649468, 66.15861208254587211 ) ) ;
#66870=CARTESIAN_POINT ( 'NONE',  ( -152.2873556200145231, 67.91256772393731467, -49.28212837332362284 ) ) ;
#66871=CARTESIAN_POINT ( 'NONE',  ( 207.8407634284390895, 112.5209879629463927, -10.15859321470372123 ) ) ;
#66873=CARTESIAN_POINT ( 'NONE',  ( -35.99414836699284592, 11.40630460607620478, 31.73781940164764492 ) ) ;
#66874=DIRECTION ( 'NONE',  ( -0.000000000000000000, 1.000000000000000000, -0.000000000000000000 ) ) ;
#66875=CARTESIAN_POINT ( 'NONE',  ( -8.673273193496447320, 6.947386154991765039, -89.14335558532187065 ) ) ;
#66876=CARTESIAN_POINT ( 'NONE',  ( -47.80193682758675067, 12.85650137125658787, -71.54144132489784624 ) ) ;
#66877=CARTESIAN_POINT ( 'NONE',  ( -6.840165690716682789, 7.836465889224659698, -23.52462357493867273 ) ) ;
#66880=DIRECTION ( 'NONE',  ( -0.000000000000000000, 1.000000000000000000, -0.000000000000000000 ) ) ;
#66881=CARTESIAN_POINT ( 'NONE',  ( -60.66241560458684035, 16.25736033771447708, 5.970147805581513367 ) ) ;
#66886=EDGE_LOOP ( 'NONE', ( #7579, #64487 ) ) ;
#66887=CARTESIAN_POINT ( 'NONE',  ( 107.9301116202192077, 27.82606182274594175, -77.41725551972304231 ) ) ;
#66888=B_SPLINE_CURVE_WITH_KNOTS ( 'NONE', 3,
 ( #32439, #65855, #32782, #27148, #17653, #65144, #53867, #37704, #54210, #60557, #7093, #12374, #43318, #49288, #6034, #28553, #49999, #17291, #27495, #59843, #1831, #23289, #776, #1125, #28192, #44734, #59153, #10973, #60206, #11664, #48579, #33496, #21871, #22228, #25018, #46451, #13418, #55625, #60902, #51741, #3548, #61605, #34881, #45776, #62294, #39803 ),
 .UNSPECIFIED., .F., .F.,
 ( 4, 2, 2, 2, 2, 2, 2, 2, 2, 2, 2, 2, 2, 2, 2, 2, 2, 2, 2, 2, 2, 2, 4 ),
 ( 1.387778780781445676E-17, 0.003635178948345809194, 0.005452768422518706852, 0.007270357896691604510, 0.008179152633778018211, 0.009087947370864430177, 0.01090553684503732870, 0.01181433158212377016, 0.01272312631921020988, 0.01363192105629665134, 0.01454071579338309106, 0.01544951053046953078, 0.01635830526755597050, 0.01726710000464240849, 0.01817589474172884648, 0.01908468947881530181, 0.01999348421590176061, 0.02090227895298821595, 0.02181107369007466781, 0.02362866316424764440, 0.02544625263842061405, 0.02726384211259358370, 0.02908143158676655682 ),
 .UNSPECIFIED. ) ;
#66889=CARTESIAN_POINT ( 'NONE',  ( 39.40195752203891999, 9.424259417798147354, -8.775266874964067654 ) ) ;
#66890=CARTESIAN_POINT ( 'NONE',  ( 41.81982603358025585, 8.735900550613189708, 71.37462574018115902 ) ) ;
#66893=CARTESIAN_POINT ( 'NONE',  ( -15.22778517348776361, 7.486636596785420039, 92.55426355724088694 ) ) ;
#66894=DIRECTION ( 'NONE',  ( -0.8160245890732938934, -0.5780171883497599028, 0.000000000000000000 ) ) ;
#66901=CARTESIAN_POINT ( 'NONE',  ( 45.23132793708834498, 9.239011044489725322, -92.01594079018720151 ) ) ;
#66902=CARTESIAN_POINT ( 'NONE',  ( 110.2429982417149432, 29.99119854320847267, 56.45576479620100940 ) ) ;
#66905=CARTESIAN_POINT ( 'NONE',  ( 55.76255201544532980, 12.13275766515752352, -18.34786871411591136 ) ) ;
#66908=CARTESIAN_POINT ( 'NONE',  ( -11.14445507968271265, 7.129894202659275315, 57.73002498924695658 ) ) ;
#66909=CARTESIAN_POINT ( 'NONE',  ( -84.55373779407985069, 24.65190748253135666, -20.44369671590408188 ) ) ;
#66910=DIRECTION ( 'NONE',  ( 0.000000000000000000, 0.000000000000000000, 1.000000000000000000 ) ) ;
#66911=CARTESIAN_POINT ( 'NONE',  ( 174.9161599490639958, 73.97365196673300147, -21.15566724134466980 ) ) ;
#66912=CARTESIAN_POINT ( 'NONE',  ( 8.711335105127083978, 6.377209569302061176, -94.18985153538824306 ) ) ;
#66918=CARTESIAN_POINT ( 'NONE',  ( 32.38493285958206513, 8.611594965040680449, -72.62366015745288905 ) ) ;
#66919=CYLINDRICAL_SURFACE ( 'NONE', #18649, 7.500000000000020428 ) ;
#66921=CARTESIAN_POINT ( 'NONE',  ( 79.19345177405119784, 17.01649702043280143, -69.15554048193783387 ) ) ;
#66923=AXIS2_PLACEMENT_3D ( 'NONE', #3567, #41208, #3234 ) ;
#66927=CARTESIAN_POINT ( 'NONE',  ( 198.4045886930828999, 99.71425793793706305, -47.91473179564368934 ) ) ;
#66931=CARTESIAN_POINT ( 'NONE',  ( -81.90266786693713641, 23.58030232261292269, -62.67706780553669432 ) ) ;
#66935=VERTEX_POINT ( 'NONE', #9827 ) ;
#66936=ORIENTED_EDGE ( 'NONE', *, *, #13490, .F. ) ;
#66939=CARTESIAN_POINT ( 'NONE',  ( 23.03578842369135060, 6.840884649289439956, 8.724805532731496172 ) ) ;
#66942=CARTESIAN_POINT ( 'NONE',  ( -53.13788504024111603, 15.21566150156364472, -49.98378873765529562 ) ) ;
#66943=CARTESIAN_POINT ( 'NONE',  ( -51.34562532494749831, 14.75613283840037226, 17.51063492481643635 ) ) ;
#66944=CARTESIAN_POINT ( 'NONE',  ( -133.3316503378477194, 52.82738260200862612, -16.67245717274693817 ) ) ;
#66945=CARTESIAN_POINT ( 'NONE',  ( 116.5096233816162226, 31.89062767870469273, -20.70603978022794678 ) ) ;
#66946=CARTESIAN_POINT ( 'NONE',  ( 81.76212856587197564, 18.87332718082998184, -49.03296493046755700 ) ) ;
#66947=DIRECTION ( 'NONE',  ( 0.000000000000000000, 0.000000000000000000, 1.000000000000000000 ) ) ;
#66952=CARTESIAN_POINT ( 'NONE',  ( -177.1171839969303790, 93.24095453296547475, 85.64081015030684796 ) ) ;
#66954=CARTESIAN_POINT ( 'NONE',  ( 110.2429982417149432, 28.88204397445231564, -9.077886975189997543 ) ) ;
#66956=CARTESIAN_POINT ( 'NONE',  ( -149.5074843970971017, 65.50121172469320641, -88.50193171241930656 ) ) ;
#66961=CARTESIAN_POINT ( 'NONE',  ( -12.77647591501652258, 7.263973827022343954, 31.96032565673792547 ) ) ;
#66963=CARTESIAN_POINT ( 'NONE',  ( 14.80291736570134198, 7.477373894757625372, -8.722967785034317245 ) ) ;
#66964=ORIENTED_EDGE ( 'NONE', *, *, #60699, .F. ) ;
#66969=CARTESIAN_POINT ( 'NONE',  ( -34.56507149095983777, 11.14725472196901102, 84.58056017436020113 ) ) ;
#66971=CARTESIAN_POINT ( 'NONE',  ( 208.5889601154909485, 111.8333159387241551, -77.09575200716440690 ) ) ;
#66975=CARTESIAN_POINT ( 'NONE',  ( -102.7456062648101920, 33.01749955571781925, 3.674523915951419362 ) ) ;
#66978=CARTESIAN_POINT ( 'NONE',  ( 129.5193594945038740, 38.86618897895345981, -37.38643059234041033 ) ) ;
#66980=ORIENTED_EDGE ( 'NONE', *, *, #3842, .T. ) ;
#66982=CARTESIAN_POINT ( 'NONE',  ( 187.8218355889145244, 87.19036431598357240, 93.79717328677281785 ) ) ;
#66983=CARTESIAN_POINT ( 'NONE',  ( -13.78709718204646961, 7.352743657744182038, 6.194210338890429490 ) ) ;
#66985=CARTESIAN_POINT ( 'NONE',  ( -23.95096213915836358, 8.481591526885939203, -69.17300232734811516 ) ) ;
#66988=EDGE_CURVE ( 'NONE', #37405, #32357, #47100, .T. ) ;
#66992=DIRECTION ( 'NONE',  ( -0.000000000000000000, 1.000000000000000000, -0.000000000000000000 ) ) ;
#66993=CARTESIAN_POINT ( 'NONE',  ( -62.14837099232446604, 17.75045801599140916, -67.11862576860336560 ) ) ;
#66994=CARTESIAN_POINT ( 'NONE',  ( 197.3700262219430783, 98.41176242030789467, -69.04069344347526282 ) ) ;
#66997=CARTESIAN_POINT ( 'NONE',  ( -172.3555096094762007, 86.27981310770638856, -88.43010234907279710 ) ) ;
#66999=CARTESIAN_POINT ( 'NONE',  ( -48.04019567818507142, 12.91272349839804612, 67.33324740833442945 ) ) ;
#67000=CARTESIAN_POINT ( 'NONE',  ( -102.2801239173131052, 32.78103895658057354, -88.70367844590326456 ) ) ;
#67001=B_SPLINE_CURVE_WITH_KNOTS ( 'NONE', 3,
 ( #64570, #44137, #29039, #6160, #66337, #17412, #23416, #65626, #18129, #28679, #38891, #22353, #28318, #39238, #32903, #27973, #49417, #27622, #39581, #43445, #33960, #49064, #61032, #60334, #44853, #12154, #12857, #50135, #33620, #43788, #49762, #60684, #54341, #1245, #22697, #899, #34311, #55395, #55759, #65263, #54698, #7585, #55048, #11788 ),
 .UNSPECIFIED., .F., .F.,
 ( 4, 2, 2, 2, 2, 2, 2, 2, 2, 2, 2, 2, 2, 2, 2, 2, 2, 2, 2, 2, 2, 4 ),
 ( 7.949501638480626889E-18, 0.001488594467279739410, 0.002232891700919614753, 0.002977188934559490529, 0.004465783401839220831, 0.005954377869118950700, 0.007442972336398679702, 0.008187269570038539432, 0.008931566803678396560, 0.01042016127095812469, 0.01190875573823785109, 0.01265305297187772036, 0.01339735020551758964, 0.01488594467279732124, 0.01563024190643718531, 0.01637453914007705111, 0.01786313360735678271, 0.01935172807463651432, 0.02009602530827637665, 0.02084032254191623551, 0.02232891700919593589, 0.02381751147647563974 ),
 .UNSPECIFIED. ) ;
#67002=ORIENTED_EDGE ( 'NONE', *, *, #17068, .F. ) ;
#67005=DIRECTION ( 'NONE',  ( 0.000000000000000000, 0.000000000000000000, 1.000000000000000000 ) ) ;
#67008=VERTEX_POINT ( 'NONE', #4541 ) ;
#67009=CARTESIAN_POINT ( 'NONE',  ( -189.3176006225846777, 107.1977018681081830, -94.62771892500191484 ) ) ;
#67010=CARTESIAN_POINT ( 'NONE',  ( -38.78626392836186909, 11.93872315530319916, -95.00000000000133582 ) ) ;
#67011=VERTEX_POINT ( 'NONE', #15101 ) ;
#67015=CARTESIAN_POINT ( 'NONE',  ( 151.8005253678162489, 54.62151558044535449, 31.97340054755885674 ) ) ;
#67022=CARTESIAN_POINT ( 'NONE',  ( 56.28782924480456984, 12.23883190161852141, -39.86895606791594560 ) ) ;
#67024=VECTOR ( 'NONE', #34024, 1000.000000000000000 ) ;
#67025=CARTESIAN_POINT ( 'NONE',  ( 154.5976934653194235, 55.45027480068274173, 83.64124856708572509 ) ) ;
#67028=CARTESIAN_POINT ( 'NONE',  ( -102.2801239173131052, 32.78103895658057354, -50.01457726497594081 ) ) ;
#67030=CARTESIAN_POINT ( 'NONE',  ( -180.5668408223793904, 97.41302302526328560, -95.00000000000133582 ) ) ;
#67032=AXIS2_PLACEMENT_3D ( 'NONE', #12364, #7788, #66894 ) ;
#67033=CARTESIAN_POINT ( 'NONE',  ( -78.66644367742109978, 23.39876645725288284, 3.573650549209446137 ) ) ;
#67037=ORIENTED_EDGE ( 'NONE', *, *, #51085, .F. ) ;
#67039=ORIENTED_EDGE ( 'NONE', *, *, #51552, .F. ) ;
#67040=CYLINDRICAL_SURFACE ( 'NONE', #60465, 7.500000000000013323 ) ;
#67041=CARTESIAN_POINT ( 'NONE',  ( 79.52639011421918269, 18.17129627604990461, 39.67221152056748679 ) ) ;
#67044=CARTESIAN_POINT ( 'NONE',  ( 188.2988323915788271, 86.21831227955482291, -14.81084150280703149 ) ) ;
#67045=EDGE_CURVE ( 'NONE', #48053, #16484, #58680, .T. ) ;
#67046=CARTESIAN_POINT ( 'NONE',  ( 141.3445468829084746, 46.13338528906590597, -16.17497209548320214 ) ) ;
#67047=CARTESIAN_POINT ( 'NONE',  ( -85.90077524418997257, 26.30132018890135726, -13.77631410858295880 ) ) ;
#67048=CARTESIAN_POINT ( 'NONE',  ( -52.45048892661851170, 15.03803514841138167, 44.85560778983723651 ) ) ;
#67053=CARTESIAN_POINT ( 'NONE',  ( 164.8471526211111495, 63.62172173173267709, 65.13593242948432760 ) ) ;
#67055=CARTESIAN_POINT ( 'NONE',  ( -189.4248691432192686, 107.3461292335514514, 63.53451367963538843 ) ) ;
#67056=CARTESIAN_POINT ( 'NONE',  ( 188.5645326065591121, 86.51153908883290455, -44.34441675984400177 ) ) ;
#67057=CARTESIAN_POINT ( 'NONE',  ( -109.7793173546317149, 36.75648380851389874, 65.14726243352887991 ) ) ;
#67058=CARTESIAN_POINT ( 'NONE',  ( -30.95355748062277002, 9.511738996772324484, -50.31719736520188491 ) ) ;
#67060=EDGE_LOOP ( 'NONE', ( #59686, #64933, #26108, #4300 ) ) ;
#67063=VERTEX_POINT ( 'NONE', #21741 ) ;
#67066=CARTESIAN_POINT ( 'NONE',  ( -71.21406923660235577, 19.62143231925333708, 92.51346753887716545 ) ) ;
#67067=CARTESIAN_POINT ( 'NONE',  ( -80.31691774066408129, 22.95709084517031684, 72.08272523424967915 ) ) ;
#67068=CARTESIAN_POINT ( 'NONE',  ( 69.74037587279245543, 14.33355757956376131, -39.86277765393460726 ) ) ;
#67071=CARTESIAN_POINT ( 'NONE',  ( -57.65574514524056582, 16.43983577669857254, 30.77939530466288076 ) ) ;
#67072=CARTESIAN_POINT ( 'NONE',  ( -96.43817545481739728, 31.02509717589737193, -20.39993158404129403 ) ) ;
#67074=EDGE_CURVE ( 'NONE', #33435, #12795, #5566, .T. ) ;
#67077=CARTESIAN_POINT ( 'NONE',  ( 55.56634333706183781, 12.09342294753929004, 36.31147275337062297 ) ) ;
#67081=CARTESIAN_POINT ( 'NONE',  ( -1.876547441458561005, 6.576559737910138814, -47.49213133585988800 ) ) ;
#67083=CARTESIAN_POINT ( 'NONE',  ( -190.0468231512975592, 108.2116162189844601, -45.51018160493545395 ) ) ;
#67085=DIRECTION ( 'NONE',  ( 0.000000000000000000, 0.000000000000000000, 1.000000000000000000 ) ) ;
#67087=CYLINDRICAL_SURFACE ( 'NONE', #25535, 7.500000000000020428 ) ;
#67088=CARTESIAN_POINT ( 'NONE',  ( 129.1052153257903683, 39.78893484542955150, -10.85527751303051680 ) ) ;
#67089=VECTOR ( 'NONE', #49159, 1000.000000000000000 ) ;
#67090=ORIENTED_EDGE ( 'NONE', *, *, #67370, .T. ) ;
#67092=CARTESIAN_POINT ( 'NONE',  ( 128.0882145863933488, 39.20607399008167704, -48.34255653863539948 ) ) ;
#67093=CARTESIAN_POINT ( 'NONE',  ( -36.00304714721387001, 11.40794940913595745, -36.84546968814971990 ) ) ;
#67095=CARTESIAN_POINT ( 'NONE',  ( -165.7899950883215752, 79.32217045577998249, 93.63443330788398100 ) ) ;
#67096=ORIENTED_EDGE ( 'NONE', *, *, #19682, .F. ) ;
#67097=CARTESIAN_POINT ( 'NONE',  ( -124.1033713525886100, 45.32626312604505614, -35.12694700365814526 ) ) ;
#67098=CARTESIAN_POINT ( 'NONE',  ( -145.3109762780891003, 60.69959559383373460, -9.235023672830337205 ) ) ;
#67099=CARTESIAN_POINT ( 'NONE',  ( 93.85477471612979627, 22.01426047292340371, -95.00000000000133582 ) ) ;
#67101=CARTESIAN_POINT ( 'NONE',  ( 162.1106586665143254, 62.65159119643226404, 84.67060130219428515 ) ) ;
#67103=DIRECTION ( 'NONE',  ( -0.000000000000000000, 1.000000000000000000, -0.000000000000000000 ) ) ;
#67104=CARTESIAN_POINT ( 'NONE',  ( 127.1040286383415321, 37.49395136275127527, 33.73642883490668964 ) ) ;
#67105=CARTESIAN_POINT ( 'NONE',  ( 204.6977192012829789, 106.3443248447423599, 29.20772073876942088 ) ) ;
#67106=CARTESIAN_POINT ( 'NONE',  ( 21.88606409348644277, 6.772455198693818623, -47.39240431891337124 ) ) ;
#67112=CARTESIAN_POINT ( 'NONE',  ( -6.140532312358493172, 7.793717686835318403, -89.24918225055428422 ) ) ;
#67116=CARTESIAN_POINT ( 'NONE',  ( -167.6566265204789943, 82.70140535081094413, 16.62003182645536725 ) ) ;
#67118=CARTESIAN_POINT ( 'NONE',  ( 23.24028701062094271, 6.853614888934262517, -68.88555068049299734 ) ) ;
#67120=CYLINDRICAL_SURFACE ( 'NONE', #41049, 7.500000000000013323 ) ;
#67122=FACE_OUTER_BOUND ( 'NONE', #46090, .T. ) ;
#67123=CARTESIAN_POINT ( 'NONE',  ( -29.51272929882557960, 10.30144624948894361, 44.96897510227874051 ) ) ;
#67128=CARTESIAN_POINT ( 'NONE',  ( 206.2957331585308793, 110.2946564621822887, -78.04361713855180938 ) ) ;
#67131=CARTESIAN_POINT ( 'NONE',  ( 140.9141742510256847, 47.05414327990549594, 34.41968098850252744 ) ) ;
#67133=CARTESIAN_POINT ( 'NONE',  ( -133.3316503378477762, 52.82738260200861902, 10.17209341771672193 ) ) ;
#67134=EDGE_CURVE ( 'NONE', #39251, #57393, #59762, .T. ) ;
#67135=CARTESIAN_POINT ( 'NONE',  ( 69.72564955710448942, 15.37006465677309563, -66.70557166199922960 ) ) ;
#67137=EDGE_CURVE ( 'NONE', #41887, #52905, #17732, .T. ) ;
#67140=CARTESIAN_POINT ( 'NONE',  ( 209.8254370498217725, 113.6481017352174518, -92.02841627014599624 ) ) ;
#67141=CARTESIAN_POINT ( 'NONE',  ( -49.98055992077275533, 13.37998597487507801, -90.87642535906408625 ) ) ;
#67143=CARTESIAN_POINT ( 'NONE',  ( -147.7860806339124622, 62.73248524776226276, 30.90810370450622102 ) ) ;
#67144=CARTESIAN_POINT ( 'NONE',  ( -128.9925397612932443, 48.56800623462824973, 58.13062048391246606 ) ) ;
#67145=CARTESIAN_POINT ( 'NONE',  ( -76.33235143960692426, 22.51916353135073834, -8.639353371581263374 ) ) ;
#67146=ORIENTED_EDGE ( 'NONE', *, *, #27089, .T. ) ;
#67148=EDGE_LOOP ( 'NONE', ( #38966, #28632, #12305, #63210 ) ) ;
#67149=CARTESIAN_POINT ( 'NONE',  ( 34.45817031441433897, 7.817703378455677310, 31.75217239037434780 ) ) ;
#67152=CARTESIAN_POINT ( 'NONE',  ( 188.5662303205146486, 86.51341602961785782, 37.40710550623141728 ) ) ;
#67162=CARTESIAN_POINT ( 'NONE',  ( -156.7487895666416478, 70.57327586518562157, -17.44133594024488332 ) ) ;
#67165=CARTESIAN_POINT ( 'NONE',  ( -60.95805269991219433, 17.39401718769329364, 60.03175317332093641 ) ) ;
#67171=CARTESIAN_POINT ( 'NONE',  ( -96.45845418068300603, 29.92035703021965531, -20.42477309577358824 ) ) ;
#67173=CARTESIAN_POINT ( 'NONE',  ( 141.3445468829085030, 46.13338528906591307, -43.01952268594691020 ) ) ;
#67176=CARTESIAN_POINT ( 'NONE',  ( -155.7457403566965866, 71.01814553754118720, 60.87164375294486263 ) ) ;
#67177=CARTESIAN_POINT ( 'NONE',  ( -122.3963566076408540, 44.23346594671848919, 31.46867208311915221 ) ) ;
#67180=ORIENTED_EDGE ( 'NONE', *, *, #62910, .T. ) ;
#67181=DIRECTION ( 'NONE',  ( -0.8118923937861950435, -0.5838071093367415143, 0.000000000000000000 ) ) ;
#67183=CARTESIAN_POINT ( 'NONE',  ( 116.9200705848630548, 32.09536795999727588, 40.56517214532210858 ) ) ;
#67184=CARTESIAN_POINT ( 'NONE',  ( 93.85477471612979627, 22.01426047292340371, -95.00000000000133582 ) ) ;
#67187=CARTESIAN_POINT ( 'NONE',  ( 164.9559213734324885, 63.71338633026439879, -16.23612744046200618 ) ) ;
#67188=CARTESIAN_POINT ( 'NONE',  ( -24.09190246691234805, -170.0000000000000000, -95.00000000000133582 ) ) ;
#67189=CARTESIAN_POINT ( 'NONE',  ( 65.41496713438824884, 13.24164235279044988, 71.27981269759310123 ) ) ;
#67190=CARTESIAN_POINT ( 'NONE',  ( 134.3135005523731706, 42.87884033955815255, 2.676193764966367628 ) ) ;
#67197=CARTESIAN_POINT ( 'NONE',  ( 68.94309019697860208, 15.16533147648752156, 68.77903629494470295 ) ) ;
#67201=CARTESIAN_POINT ( 'NONE',  ( 162.6205203824432033, 63.07332653227187791, -38.16676261939332448 ) ) ;
#67205=VERTEX_POINT ( 'NONE', #28063 ) ;
#67206=CARTESIAN_POINT ( 'NONE',  ( -95.21085197937823352, 30.44372064875429018, 13.73146625934893095 ) ) ;
#67208=CARTESIAN_POINT ( 'NONE',  ( 70.50774432417125581, 15.57735247846618165, 90.51896257976297022 ) ) ;
#67212=CARTESIAN_POINT ( 'NONE',  ( 84.26390409839194717, 19.68678207880319420, -9.343633932740562642 ) ) ;
#67213=CARTESIAN_POINT ( 'NONE',  ( -165.9122696334865168, 79.44688201528256855, 36.23136382548763379 ) ) ;
#67214=CARTESIAN_POINT ( 'NONE',  ( -147.9110140428198861, 62.83667129753960268, -88.66273618399704048 ) ) ;
#67216=CARTESIAN_POINT ( 'NONE',  ( 132.9440032680862487, 40.87616997986734191, -77.81562762824698609 ) ) ;
#67218=CARTESIAN_POINT ( 'NONE',  ( -95.63694837622351486, 30.64472169584719552, 68.35390755590003664 ) ) ;
#67220=CARTESIAN_POINT ( 'NONE',  ( -14.33060720034883673, 8.412649192293191192, 60.69540906425582705 ) ) ;
#67223=CARTESIAN_POINT ( 'NONE',  ( -152.4930836497867688, 68.09400557494207362, -49.19664785734511980 ) ) ;
#67226=CARTESIAN_POINT ( 'NONE',  ( -38.45778834351241926, 11.87434869453507247, 40.37145622466209716 ) ) ;
#67227=CARTESIAN_POINT ( 'NONE',  ( -152.5046761101291963, 66.76407727525179325, -62.27860238260412018 ) ) ;
#67228=DIRECTION ( 'NONE',  ( -0.000000000000000000, 1.000000000000000000, -0.000000000000000000 ) ) ;
#67229=CARTESIAN_POINT ( 'NONE',  ( -51.34325167237333432, 13.71819364263222241, -63.03792477884681489 ) ) ;
#67231=CARTESIAN_POINT ( 'NONE',  ( 175.8855729601531834, 73.50624012737692681, 4.536635858610266858 ) ) ;
#67232=CARTESIAN_POINT ( 'NONE',  ( -61.75956139478100937, 16.58288496614413177, 7.606635706506060579 ) ) ;
#67235=CARTESIAN_POINT ( 'NONE',  ( -99.99439884168255332, 32.75762661251358310, -35.35557488724050756 ) ) ;
#67237=CARTESIAN_POINT ( 'NONE',  ( 106.6192711434718490, 27.24117154335862168, -76.83786816052128188 ) ) ;
#67238=CARTESIAN_POINT ( 'NONE',  ( 46.85361596800670725, 10.51535167202354160, -15.29056264614206384 ) ) ;
#67240=FACE_OUTER_BOUND ( 'NONE', #10787, .T. ) ;
#67243=B_SPLINE_CURVE_WITH_KNOTS ( 'NONE', 3,
 ( #29561, #41507, #62959, #14766, #67227, #36231, #57688, #9498, #29916, #24304, #19011, #3192, #40463, #25690, #68582, #20383, #41852, #35189, #56644, #8464, #51375, #21089, #20736, #5917, #31983, #11202, #26021, #32332, #10514, #42534, #37245, #48138, #32671, #26705, #58026, #48465, #42193, #4900, #63987, #63657, #36579, #4558, #43555, #47451 ),
 .UNSPECIFIED., .F., .F.,
 ( 4, 2, 2, 2, 2, 2, 2, 2, 2, 2, 2, 2, 2, 2, 2, 2, 2, 2, 2, 2, 2, 4 ),
 ( 0.000000000000000000, 0.003433139681083573636, 0.004291424601354481248, 0.005149709521625388427, 0.006866279362167105639, 0.007724564282437977256, 0.008582849202708844535, 0.009441134122979715285, 0.01029941904325058430, 0.01201598888379235702, 0.01373255872433412975, 0.01459084364460501611, 0.01544912856487590420, 0.01630741348514679057, 0.01716569840541767866, 0.01888226824595941669, 0.02059883808650115472, 0.02145712300677206016, 0.02231540792704296561, 0.02403197776758486323, 0.02574854760812675739, 0.02746511744866865501 ),
 .UNSPECIFIED. ) ;
#67244=CARTESIAN_POINT ( 'NONE',  ( 57.80731956814545214, 12.55178936583606131, -91.45004045484938615 ) ) ;
#67246=VERTEX_POINT ( 'NONE', #53744 ) ;
#67251=CARTESIAN_POINT ( 'NONE',  ( 103.8055367708241477, 27.11070767929349756, 67.83620103106419208 ) ) ;
#67255=CARTESIAN_POINT ( 'NONE',  ( 109.7732660198864210, 29.77277639096405792, -35.92243756565368784 ) ) ;
#67256=CARTESIAN_POINT ( 'NONE',  ( 22.51849650178395024, 7.817407610814548491, -39.70014265684829269 ) ) ;
#67259=FACE_BOUND ( 'NONE', #1045, .T. ) ;
#67268=CARTESIAN_POINT ( 'NONE',  ( -174.7903139851459287, 90.53182997092831386, 18.80111118392543190 ) ) ;
#67269=CARTESIAN_POINT ( 'NONE',  ( 8.722750525486095086, 6.377265220791373146, 88.66693184439566267 ) ) ;
#67276=EDGE_CURVE ( 'NONE', #48157, #65219, #52211, .T. ) ;
#67280=CARTESIAN_POINT ( 'NONE',  ( -81.67992981004169906, 23.49232121719085953, -76.33213373116126377 ) ) ;
#67287=CARTESIAN_POINT ( 'NONE',  ( 40.38495044702528247, 9.554194848483442470, 56.80706957984675398 ) ) ;
#67289=CARTESIAN_POINT ( 'NONE',  ( 23.09784929786603058, 6.844738137842330872, 12.36717293848776400 ) ) ;
#67292=CARTESIAN_POINT ( 'NONE',  ( -51.13576748034040520, 14.70354244225167051, 4.572286290533843278 ) ) ;
#67294=EDGE_CURVE ( 'NONE', #45287, #629, #50570, .T. ) ;
#67295=CARTESIAN_POINT ( 'NONE',  ( 116.6734749296698652, 31.97209464358269315, -12.68594914507928451 ) ) ;
#67296=CARTESIAN_POINT ( 'NONE',  ( 81.74250361646210195, 18.86685472882139081, -37.61107281654683732 ) ) ;
#67297=FACE_OUTER_BOUND ( 'NONE', #63571, .T. ) ;
#67301=CARTESIAN_POINT ( 'NONE',  ( 180.2565361171341181, 79.19912802278403774, 2.497854800821170951 ) ) ;
#67302=CARTESIAN_POINT ( 'NONE',  ( -52.66507163626138777, 14.05394608175175186, -8.745596592972852079 ) ) ;
#67303=CARTESIAN_POINT ( 'NONE',  ( 201.6034029841261770, 102.1956603101140644, 16.70862505107374218 ) ) ;
#67304=CARTESIAN_POINT ( 'NONE',  ( -30.58710862550656273, 9.453045329524901064, -89.05181077067686601 ) ) ;
#67305=CARTESIAN_POINT ( 'NONE',  ( 204.4529252293439754, 107.7183975564644953, 82.89604892619028931 ) ) ;
#67306=CARTESIAN_POINT ( 'NONE',  ( 210.0055645826033413, 115.7254585628713954, 31.38593627897014215 ) ) ;
#67307=CARTESIAN_POINT ( 'NONE',  ( -73.09185868250597196, 20.27574131633382137, -64.41869867121339155 ) ) ;
#67308=CARTESIAN_POINT ( 'NONE',  ( -14.19493007850031319, 7.389842975086042820, 33.64835350072206666 ) ) ;
#67310=CARTESIAN_POINT ( 'NONE',  ( 13.84704553156522344, 7.452804552247568104, -23.42297353679536442 ) ) ;
#67312=CARTESIAN_POINT ( 'NONE',  ( 197.3685896092615621, 96.80423329231979324, -18.60473238905292703 ) ) ;
#67315=CARTESIAN_POINT ( 'NONE',  ( -145.5195986658808351, 62.16746116576785397, 5.020210888928557935 ) ) ;
#67316=CARTESIAN_POINT ( 'NONE',  ( 185.7267155939802876, 84.90388481853126734, -76.46461293044741581 ) ) ;
#67317=CARTESIAN_POINT ( 'NONE',  ( -38.94425962551733988, 11.96984520263672636, 91.57215036848938894 ) ) ;
#67318=CARTESIAN_POINT ( 'NONE',  ( -101.8145602049405767, 32.54453702486150490, -35.01457726497591239 ) ) ;
#67321=CARTESIAN_POINT ( 'NONE',  ( 9.689943677145725687, 7.388265075009368132, -47.39164370131542370 ) ) ;
#67322=CARTESIAN_POINT ( 'NONE',  ( 133.8566784816069628, 41.42467568809806977, -36.02331093239566684 ) ) ;
#67324=VERTEX_POINT ( 'NONE', #25839 ) ;
#67325=CARTESIAN_POINT ( 'NONE',  ( 188.5857024137486349, 88.03875867569850300, 90.36958172790924948 ) ) ;
#67327=DIRECTION ( 'NONE',  ( -0.000000000000000000, 1.000000000000000000, -0.000000000000000000 ) ) ;
#67328=CARTESIAN_POINT ( 'NONE',  ( -25.81763596640059433, 8.735969132042862739, -74.63268230678318105 ) ) ;
#67331=CARTESIAN_POINT ( 'NONE',  ( 45.35621884287174055, 10.27694987765648271, -74.55092264549712411 ) ) ;
#67333=CARTESIAN_POINT ( 'NONE',  ( 199.9103251464699724, 101.6434290204575746, -64.89257074407096582 ) ) ;
#67335=CARTESIAN_POINT ( 'NONE',  ( -179.8996803435689174, 95.00451760716445904, -38.99053287237702392 ) ) ;
#67337=CARTESIAN_POINT ( 'NONE',  ( -24.18158274621863413, 9.527343002918314596, 62.60597738986891869 ) ) ;
#67339=CARTESIAN_POINT ( 'NONE',  ( -47.68742944762959013, 12.82957801017945698, 66.14038351141603300 ) ) ;
#67340=CARTESIAN_POINT ( 'NONE',  ( -100.2050497862850023, 31.73888266434120453, -88.98404108870900586 ) ) ;
#67341=EDGE_LOOP ( 'NONE', ( #51656, #37150 ) ) ;
#67343=CARTESIAN_POINT ( 'NONE',  ( -130.2196570250629293, 49.40815211106346538, -75.40313927343784428 ) ) ;
#67344=CARTESIAN_POINT ( 'NONE',  ( -109.3386876948163859, 37.66246927061207828, -71.94451923632995261 ) ) ;
#67345=CARTESIAN_POINT ( 'NONE',  ( -54.08504625707234936, 14.42374043447185983, -35.26311519142592488 ) ) ;
#67349=DIRECTION ( 'NONE',  ( -0.000000000000000000, 1.000000000000000000, -0.000000000000000000 ) ) ;
#67352=EDGE_LOOP ( 'NONE', ( #44932, #13573, #19417, #37231 ) ) ;
#67353=ORIENTED_EDGE ( 'NONE', *, *, #67510, .T. ) ;
#67355=CARTESIAN_POINT ( 'NONE',  ( 152.6804161981488619, 55.27286404993343183, 31.13324756182342412 ) ) ;
#67360=CARTESIAN_POINT ( 'NONE',  ( -176.3896317155479778, 90.84057090619019448, 4.712634550793983301 ) ) ;
#67365=CARTESIAN_POINT ( 'NONE',  ( 158.1697021771102527, 58.19565064619519745, 83.10739206537702728 ) ) ;
#67366=CARTESIAN_POINT ( 'NONE',  ( 204.6977192012829789, -170.0000000000000000, 2.363170148305746565 ) ) ;
#67369=CARTESIAN_POINT ( 'NONE',  ( 12.46704290855393182, 6.417105965824394076, 57.63022159756878438 ) ) ;
#67370=EDGE_CURVE ( 'NONE', #51909, #64139, #53476, .T. ) ;
#67372=CARTESIAN_POINT ( 'NONE',  ( -71.15968973604427106, 20.66697821823242265, 91.53401883404465877 ) ) ;
#67375=CARTESIAN_POINT ( 'NONE',  ( 82.94943325692331371, 18.19803534719805782, -49.86125457933553662 ) ) ;
#67377=ADVANCED_FACE ( 'NONE', ( #21237 ), #47607, .F. ) ;
#67379=DIRECTION ( 'NONE',  ( 0.000000000000000000, 0.000000000000000000, 1.000000000000000000 ) ) ;
#67380=DIRECTION ( 'NONE',  ( -0.000000000000000000, 1.000000000000000000, -0.000000000000000000 ) ) ;
#67382=CARTESIAN_POINT ( 'NONE',  ( 181.9406741394862479, 79.47484497224792221, -9.417459808242304220 ) ) ;
#67383=CARTESIAN_POINT ( 'NONE',  ( -120.1259246007803370, 42.81147313035988589, 69.78542509041207609 ) ) ;
#67384=CARTESIAN_POINT ( 'NONE',  ( -85.10909119100207931, 25.97025675005452428, -19.64294555054678426 ) ) ;
#67385=CARTESIAN_POINT ( 'NONE',  ( -180.4651598106648294, 97.28730001475651079, -13.81580514006593674 ) ) ;
#67386=CARTESIAN_POINT ( 'NONE',  ( -54.57263979903869711, 15.59415114099631161, 30.31732777293113656 ) ) ;
#67389=CARTESIAN_POINT ( 'NONE',  ( -109.7156874346697748, 37.87149323084329211, 12.19027536507073783 ) ) ;
#67391=CARTESIAN_POINT ( 'NONE',  ( 164.3577270662354124, 63.21061577643035179, 60.77331709976006380 ) ) ;
#67392=CYLINDRICAL_SURFACE ( 'NONE', #23926, 7.500000000000013323 ) ;
#67399=CARTESIAN_POINT ( 'NONE',  ( 177.3657905147444467, 74.92740221268464040, -90.88983617643496871 ) ) ;
#67402=CARTESIAN_POINT ( 'NONE',  ( -60.98168946575805904, 17.40090852531920262, 42.43695973922503129 ) ) ;
#67406=CARTESIAN_POINT ( 'NONE',  ( 41.04298124592206420, 8.628434602995477931, 83.77720471021285675 ) ) ;
#67411=CARTESIAN_POINT ( 'NONE',  ( -119.5576859660651081, 42.46117483543969939, 7.254307368285498825 ) ) ;
#67413=CARTESIAN_POINT ( 'NONE',  ( 132.9440032680863624, 40.87616997986732770, -24.12652644731961615 ) ) ;
#67414=CARTESIAN_POINT ( 'NONE',  ( 20.35964562795319921, 7.697260051881320564, -10.20843155924452539 ) ) ;
#67415=CARTESIAN_POINT ( 'NONE',  ( -108.9452487746634262, 36.29752968355630571, -72.83582910382180842 ) ) ;
#67417=ORIENTED_EDGE ( 'NONE', *, *, #23437, .T. ) ;
#67419=CARTESIAN_POINT ( 'NONE',  ( 132.2818448028687612, 41.65267246304673421, -50.85966255019037874 ) ) ;
#67420=CARTESIAN_POINT ( 'NONE',  ( -127.6992109187851980, 47.69334801994794759, 3.981565830366440739 ) ) ;
#67422=CARTESIAN_POINT ( 'NONE',  ( 188.2086267457325448, 87.61890531228284829, -46.08538211307052990 ) ) ;
#67423=EDGE_LOOP ( 'NONE', ( #48189, #32338, #6177, #9901 ) ) ;
#67425=EDGE_CURVE ( 'NONE', #63280, #44375, #17490, .T. ) ;
#67426=CARTESIAN_POINT ( 'NONE',  ( -31.43908319763709969, 9.591432048623758533, -23.47264677473818395 ) ) ;
#67431=CARTESIAN_POINT ( 'NONE',  ( 150.2755237883188499, 53.50786132674227247, 92.72454620485628141 ) ) ;
#67433=ORIENTED_EDGE ( 'NONE', *, *, #43753, .T. ) ;
#67434=CARTESIAN_POINT ( 'NONE',  ( 129.1310456962234809, 39.80382822048401437, -76.21209168102404874 ) ) ;
#67436=CARTESIAN_POINT ( 'NONE',  ( -156.9919426121902575, 72.16759471857101005, 38.78368848896538879 ) ) ;
#67442=CARTESIAN_POINT ( 'NONE',  ( 15.78827728214693416, -170.0000000000000000, -23.67439350822212774 ) ) ;
#67443=ORIENTED_EDGE ( 'NONE', *, *, #19603, .T. ) ;
#67445=CARTESIAN_POINT ( 'NONE',  ( 56.30011474572736319, 11.21470186335419861, 33.96431529039685415 ) ) ;
#67448=CARTESIAN_POINT ( 'NONE',  ( -166.2065256787326177, 81.19093426984588291, 14.39615283784645072 ) ) ;
#67449=EDGE_CURVE ( 'NONE', #24801, #13412, #28323, .T. ) ;
#67450=CARTESIAN_POINT ( 'NONE',  ( 18.89064107370902690, 6.619789970027396997, -63.03085641855517451 ) ) ;
#67453=DIRECTION ( 'NONE',  ( 0.000000000000000000, 0.000000000000000000, 1.000000000000000000 ) ) ;
#67456=VECTOR ( 'NONE', #39578, 1000.000000000000000 ) ;
#67459=CARTESIAN_POINT ( 'NONE',  ( 211.3757499519975909, 117.8130818709823302, -67.24546217480406085 ) ) ;
#67460=CARTESIAN_POINT ( 'NONE',  ( 139.1306635769909121, 45.89653412152166823, 31.67232335441821078 ) ) ;
#67461=CYLINDRICAL_SURFACE ( 'NONE', #6696, 7.500000000000020428 ) ;
#67462=CARTESIAN_POINT ( 'NONE',  ( -125.8938041572051389, 47.69968343338780414, 18.77539728269342945 ) ) ;
#67465=ORIENTED_EDGE ( 'NONE', *, *, #48505, .F. ) ;
#67468=CARTESIAN_POINT ( 'NONE',  ( -49.66937262962775890, 13.30390939630160929, -91.17893582821346854 ) ) ;
#67469=CARTESIAN_POINT ( 'NONE',  ( -48.85164209420741344, 14.14099498278764244, -92.18124229352110888 ) ) ;
#67471=CARTESIAN_POINT ( 'NONE',  ( 70.46579300139244140, 15.56614468937218909, -42.22221902765776491 ) ) ;
#67472=CARTESIAN_POINT ( 'NONE',  ( -118.3948752128398638, 42.92869324237091178, 38.41731472785173906 ) ) ;
#67473=CARTESIAN_POINT ( 'NONE',  ( -166.7068579965637127, 80.26142964949320913, -72.95228584046991216 ) ) ;
#67477=CARTESIAN_POINT ( 'NONE',  ( -180.2625951943601024, 95.44595303765449046, -93.59349302508864810 ) ) ;
#67478=CARTESIAN_POINT ( 'NONE',  ( 81.57915404881514121, 18.81499384983930057, 58.50637853310414727 ) ) ;
#67480=CARTESIAN_POINT ( 'NONE',  ( 86.62931800182293784, 19.42108912189597092, -50.82156419891174437 ) ) ;
#67484=CARTESIAN_POINT ( 'NONE',  ( 36.76746179515744473, 8.081433644308900099, 17.59563346917418869 ) ) ;
#67485=CARTESIAN_POINT ( 'NONE',  ( -15.27594996066617483, 8.502079791899657124, -43.90747202117393755 ) ) ;
#67489=CARTESIAN_POINT ( 'NONE',  ( -109.4059773746700444, 36.55056299043143753, -93.85300586226982489 ) ) ;
#67492=CARTESIAN_POINT ( 'NONE',  ( -57.43883374585517032, 16.37892664338858850, 71.77631074466216887 ) ) ;
#67493=CARTESIAN_POINT ( 'NONE',  ( 15.78827728214693416, -170.0000000000000000, -96.70804527961315955 ) ) ;
#67494=EDGE_LOOP ( 'NONE', ( #10868, #3086 ) ) ;
#67496=CARTESIAN_POINT ( 'NONE',  ( -56.73992761491503245, 15.14028026131270366, -89.09451971216485333 ) ) ;
#67497=CARTESIAN_POINT ( 'NONE',  ( -37.92542950990691963, 10.74638084523341952, 33.94305653771795761 ) ) ;
#67498=CARTESIAN_POINT ( 'NONE',  ( 139.6359093656974153, 45.02518919224743144, -38.73665037353510598 ) ) ;
#67501=VERTEX_POINT ( 'NONE', #54194 ) ;
#67502=CARTESIAN_POINT ( 'NONE',  ( -153.1031717208031750, 68.63449618039562949, 58.47953369091288067 ) ) ;
#67503=CARTESIAN_POINT ( 'NONE',  ( 110.2429982417149290, 28.88204397445231209, 29.61121420573730489 ) ) ;
#67504=CARTESIAN_POINT ( 'NONE',  ( -58.10608953386397246, 15.52134062643864354, -49.57095537761784954 ) ) ;
#67506=CARTESIAN_POINT ( 'NONE',  ( -179.5109681715918555, 96.11572638569523974, -73.02150784162149932 ) ) ;
#67507=CARTESIAN_POINT ( 'NONE',  ( 129.1998560374819647, 39.84370217048449092, 84.81121093761140628 ) ) ;
#67510=EDGE_CURVE ( 'NONE', #47754, #59735, #38418, .T. ) ;
#67513=CARTESIAN_POINT ( 'NONE',  ( 133.8566784816069344, 41.42467568809808398, 29.51034083899533300 ) ) ;
#67516=CARTESIAN_POINT ( 'NONE',  ( 197.8436586345020203, 97.39326576892285914, 33.60968991493576397 ) ) ;
#67517=CARTESIAN_POINT ( 'NONE',  ( 111.8699272271189358, 29.64190505307782075, -77.59217791608018899 ) ) ;
#67518=CARTESIAN_POINT ( 'NONE',  ( 110.2429982417149432, 29.99119854320846201, -35.92243756565368784 ) ) ;
#67519=CARTESIAN_POINT ( 'NONE',  ( 182.4910189501783577, 80.03877586733645444, -90.03880345596023460 ) ) ;
#67524=DIRECTION ( 'NONE',  ( -0.000000000000000000, 1.000000000000000000, -0.000000000000000000 ) ) ;
#67525=AXIS2_PLACEMENT_3D ( 'NONE', #25233, #13293, #34749 ) ;
#67527=CARTESIAN_POINT ( 'NONE',  ( 63.01563776193091826, 13.70579113808095251, 56.65751152968497451 ) ) ;
#67528=CARTESIAN_POINT ( 'NONE',  ( 139.9689050549367266, 45.23922256703520617, 86.29823414930417869 ) ) ;
#67531=CARTESIAN_POINT ( 'NONE',  ( 164.9706294237034001, 65.04392654036659849, -43.89830601384430508 ) ) ;
#67532=AXIS2_PLACEMENT_3D ( 'NONE', #4133, #48056, #9756 ) ;
#67536=CARTESIAN_POINT ( 'NONE',  ( 164.6406716478538783, 63.44801348349341197, -45.84013439700346026 ) ) ;
#67540=CARTESIAN_POINT ( 'NONE',  ( 55.92717366837369042, 12.16587666349906982, 88.52872284767667566 ) ) ;
#67542=CARTESIAN_POINT ( 'NONE',  ( 79.13041963748369767, 18.04952109592811738, -16.99722329755391570 ) ) ;
#67543=CARTESIAN_POINT ( 'NONE',  ( -173.1211646369891355, 88.63826465341151106, -88.40105834567734178 ) ) ;
#67544=CARTESIAN_POINT ( 'NONE',  ( -33.83558513595455253, 9.996963989836508802, -62.55072875604015792 ) ) ;
#67545=CARTESIAN_POINT ( 'NONE',  ( 88.28889510440058075, 21.05995314109330963, 44.53004548791538753 ) ) ;
#67547=CARTESIAN_POINT ( 'NONE',  ( -101.3537077702550988, 33.43904726487055257, 72.32055988684196279 ) ) ;
#67548=CARTESIAN_POINT ( 'NONE',  ( -15.07533778868020313, 8.482826962130836534, 66.39636851612516466 ) ) ;
#67550=CARTESIAN_POINT ( 'NONE',  ( 151.6178224291901131, 54.48737267587417676, -12.08258827898731802 ) ) ;
#67551=CARTESIAN_POINT ( 'NONE',  ( 211.8382652195006983, 118.5282575235990095, -14.66487468951659068 ) ) ;
#67552=CARTESIAN_POINT ( 'NONE',  ( -33.83721310978700103, 11.01869210665938681, 30.60599803115480810 ) ) ;
#67554=CARTESIAN_POINT ( 'NONE',  ( 61.72676562228498653, 12.37728358935400941, 83.60623520330705105 ) ) ;
#67556=CARTESIAN_POINT ( 'NONE',  ( -0.7211439451572427828, 7.539282923622933730, -13.65695759729669234 ) ) ;
#67557=CARTESIAN_POINT ( 'NONE',  ( 174.6176230994777541, 72.30829341023246570, 13.80334415398240111 ) ) ;
#67558=CARTESIAN_POINT ( 'NONE',  ( -56.96214175905167565, 15.20165595797839586, 18.22969659526463815 ) ) ;
#67562=CARTESIAN_POINT ( 'NONE',  ( 102.8458551240039611, 25.60773946375956456, -71.53149621033008998 ) ) ;
#67564=CARTESIAN_POINT ( 'NONE',  ( 45.36109889487607205, 9.259412558041161034, 68.83869726676070400 ) ) ;
#67566=CARTESIAN_POINT ( 'NONE',  ( -0.9745282055893963458, 6.541451027421887332, 94.42703022882983532 ) ) ;
#67568=CARTESIAN_POINT ( 'NONE',  ( -109.7156874346698174, 37.87149323084328500, -14.65427522539294536 ) ) ;
#67569=ORIENTED_EDGE ( 'NONE', *, *, #57328, .T. ) ;
#67572=CARTESIAN_POINT ( 'NONE',  ( -166.2028193222418793, 79.74385139484273566, 62.25590132581950087 ) ) ;
#67574=EDGE_LOOP ( 'NONE', ( #68662, #65994 ) ) ;
#67577=VECTOR ( 'NONE', #30, 1000.000000000000000 ) ;
#67579=CARTESIAN_POINT ( 'NONE',  ( 103.1695711638930959, 26.83837309506526481, 61.41201509413315307 ) ) ;
#67583=CARTESIAN_POINT ( 'NONE',  ( 60.40531521312253460, 13.11276739283242421, -23.41139328403251696 ) ) ;
#67587=CARTESIAN_POINT ( 'NONE',  ( 22.51798020284706681, 7.817376421459703018, -46.33885551830132243 ) ) ;
#67588=CARTESIAN_POINT ( 'NONE',  ( -142.8556048422594813, 60.01994222009840030, 41.69565126987502168 ) ) ;
#67589=CARTESIAN_POINT ( 'NONE',  ( 211.8476521439974078, 116.6941316755177525, 38.99529880182225838 ) ) ;
#67590=FACE_BOUND ( 'NONE', #29100, .T. ) ;
#67591=EDGE_CURVE ( 'NONE', #66072, #17942, #1551, .T. ) ;
#67593=ORIENTED_EDGE ( 'NONE', *, *, #6886, .F. ) ;
#67595=VERTEX_POINT ( 'NONE', #24313 ) ;
#67597=CARTESIAN_POINT ( 'NONE',  ( -132.6540878434535955, 52.34298938643414090, 88.49361340196719539 ) ) ;
#67598=CARTESIAN_POINT ( 'NONE',  ( 33.46033188299909256, 8.722678254080101112, -74.54781320571061087 ) ) ;
#67600=CARTESIAN_POINT ( 'NONE',  ( 22.45676458343273296, 6.805709986489419272, 87.75587017291512382 ) ) ;
#67604=CARTESIAN_POINT ( 'NONE',  ( 197.9868529032976028, 99.18611233336802968, -47.18661369665191785 ) ) ;
#67605=ORIENTED_EDGE ( 'NONE', *, *, #43505, .T. ) ;
#67607=CARTESIAN_POINT ( 'NONE',  ( 110.2429982417149574, 29.99119854320845846, -89.61153874658103291 ) ) ;
#67609=CARTESIAN_POINT ( 'NONE',  ( -83.14462298835726983, 24.07775853418029754, -75.49557268907416585 ) ) ;
#67614=CARTESIAN_POINT ( 'NONE',  ( 39.88975917505626256, 9.487965272711656795, 56.75838489642696771 ) ) ;
#67616=CARTESIAN_POINT ( 'NONE',  ( 104.7042813665017178, 27.49927371769997464, 15.34735190411218575 ) ) ;
#67623=CARTESIAN_POINT ( 'NONE',  ( -33.96986881321595320, 10.02034822982698437, 84.33807109151561576 ) ) ;
#67624=CARTESIAN_POINT ( 'NONE',  ( -54.57263979903869711, 15.59415114099631161, 3.472777182467472468 ) ) ;
#67625=CARTESIAN_POINT ( 'NONE',  ( 92.91022130985207639, -170.0000000000000000, 94.99999999999866418 ) ) ;
#67628=CARTESIAN_POINT ( 'NONE',  ( 85.67165909753201447, 20.15791549876374589, -35.86735994369028191 ) ) ;
#67629=DIRECTION ( 'NONE',  ( 0.000000000000000000, 0.000000000000000000, 1.000000000000000000 ) ) ;
#67633=CARTESIAN_POINT ( 'NONE',  ( 46.70715146412977958, 9.472433765547009443, 8.853342646177644326 ) ) ;
#67634=CARTESIAN_POINT ( 'NONE',  ( -180.1186349629460892, 96.86022136641703639, 89.28841826848275787 ) ) ;
#67635=CARTESIAN_POINT ( 'NONE',  ( 86.62931800182293784, -170.0000000000000000, -50.82156419891174437 ) ) ;
#67636=CARTESIAN_POINT ( 'NONE',  ( -190.6985136298601731, 109.1272424661242582, 60.81597207375692449 ) ) ;
#67637=CARTESIAN_POINT ( 'NONE',  ( 135.3579907212798901, 42.33677458448931930, -89.82451751908253357 ) ) ;
#67638=CARTESIAN_POINT ( 'NONE',  ( 39.40195752203892710, 8.409560354027387774, -89.30891864635511013 ) ) ;
#67639=CARTESIAN_POINT ( 'NONE',  ( 212.1325383547231525, 118.9860748747654640, 91.47708763404254739 ) ) ;
#67640=CARTESIAN_POINT ( 'NONE',  ( 208.0306608271318680, 112.7988899307265740, 29.98561732425369897 ) ) ;
#67641=CARTESIAN_POINT ( 'NONE',  ( 63.01563776193091826, -170.0000000000000000, -50.72069083216976537 ) ) ;
#67642=CARTESIAN_POINT ( 'NONE',  ( -109.7290872258107157, 36.72869630780159156, 36.99980377389978514 ) ) ;
#67644=DIRECTION ( 'NONE',  ( -0.000000000000000000, 1.000000000000000000, -0.000000000000000000 ) ) ;
#67646=CARTESIAN_POINT ( 'NONE',  ( 204.6977192012829789, 106.3443248447423599, -24.48138044215792419 ) ) ;
#67647=EDGE_LOOP ( 'NONE', ( #38429, #50167, #5239, #24642 ) ) ;
#67648=CARTESIAN_POINT ( 'NONE',  ( -144.7530445311634253, 61.54314312182903279, 5.570716979441686867 ) ) ;
#67649=B_SPLINE_CURVE_WITH_KNOTS ( 'NONE', 3,
 ( #17061, #21658, #16389, #38897, #23061, #33276, #55054, #22011, #16723, #27978, #44860, #62428, #29722, #40615, #56108, #56808, #66684, #24798, #51532, #18823, #55767, #39928, #66344, #61386, #46235, #1964, #18478, #13208, #40280, #35350, #30077, #19161, #29044, #23421, #45202, #12864, #34672, #24460, #50830, #62067, #24111, #7924, #2308, #57153, #18133 ),
 .UNSPECIFIED., .F., .F.,
 ( 4, 2, 2, 2, 2, 2, 2, 2, 2, 2, 2, 2, 2, 1, 2, 2, 2, 2, 2, 2, 2, 2, 4 ),
 ( 0.02352719711393055912, 0.02499986300757016042, 0.02573619595438996974, 0.02647252890120978253, 0.02794519479484938035, 0.02941786068848897817, 0.03015419363530878749, 0.03089052658212860375, 0.03236319247576824321, 0.03309952542258805946, 0.03383585836940787572, 0.03530852426304752906, 0.03604485720986734532, 0.03678119015668715464, 0.03751752310350696396, 0.03825385605032678021, 0.03972652194396640579, 0.04119918783760603831, 0.04267185373124567083, 0.04340818667806546627, 0.04414451962488526171, 0.04561718551852485259, 0.04708985141216444348 ),
 .UNSPECIFIED. ) ;
#67650=CARTESIAN_POINT ( 'NONE',  ( 188.0103583326377645, 87.39896620268125105, -67.67879652845185490 ) ) ;
#67651=CARTESIAN_POINT ( 'NONE',  ( -145.3233446620410518, 62.00659513626053609, 71.30669210420751369 ) ) ;
#67652=DIRECTION ( 'NONE',  ( 0.000000000000000000, 0.000000000000000000, 1.000000000000000000 ) ) ;
#67653=CARTESIAN_POINT ( 'NONE',  ( 33.03722315490659867, 7.666819786578623841, -39.14476316943679990 ) ) ;
#67654=CARTESIAN_POINT ( 'NONE',  ( -107.7893514267588415, 35.66840175773125310, 6.061804979893113732 ) ) ;
#67655=CARTESIAN_POINT ( 'NONE',  ( 9.837735240994037511, 7.389327806910505281, -47.59081060985023015 ) ) ;
#67656=CARTESIAN_POINT ( 'NONE',  ( 127.2202105166096402, 37.55913282978156786, -47.02660944393614528 ) ) ;
#67661=ADVANCED_FACE ( 'NONE', ( #30967 ), #4907, .F. ) ;
#67664=ADVANCED_FACE ( 'NONE', ( #26027 ), #47459, .F. ) ;
#67665=CARTESIAN_POINT ( 'NONE',  ( -24.93568128341082968, 8.613819379861709535, -65.89388286627800539 ) ) ;
#67667=EDGE_CURVE ( 'NONE', #36637, #17944, #62966, .T. ) ;
#67669=CARTESIAN_POINT ( 'NONE',  ( 13.14401442664830810, 6.430459733718340232, 17.69285561637535409 ) ) ;
#67672=CARTESIAN_POINT ( 'NONE',  ( 210.0122310839192039, 115.7355030290287630, 15.17826746070574373 ) ) ;
#67673=CIRCLE ( 'NONE', #15932, 243.4957430088094839 ) ;
#67675=CARTESIAN_POINT ( 'NONE',  ( 94.12988949694086216, 22.11811104795078009, -16.24132341548559921 ) ) ;
#67676=CARTESIAN_POINT ( 'NONE',  ( -23.98747857548121232, 9.501432345103353327, 65.54625325806455294 ) ) ;
#67678=CARTESIAN_POINT ( 'NONE',  ( -49.43915770973591606, 13.24768844696976089, 69.65966800992838159 ) ) ;
#67682=CARTESIAN_POINT ( 'NONE',  ( -3.252497086158844919, 6.636017118948018378, 58.49502237739417154 ) ) ;
#67687=CARTESIAN_POINT ( 'NONE',  ( 152.1381498073141358, 54.87048121475570639, 58.45773527022319627 ) ) ;
#67689=CARTESIAN_POINT ( 'NONE',  ( -49.14234466229832776, 13.17605306081208560, -47.33992328543903483 ) ) ;
#67697=CARTESIAN_POINT ( 'NONE',  ( 179.4279766878530324, 76.94722012158234747, -51.05200850905019649 ) ) ;
#67698=DIRECTION ( 'NONE',  ( 0.000000000000000000, 0.000000000000000000, 1.000000000000000000 ) ) ;
#67700=ORIENTED_EDGE ( 'NONE', *, *, #791, .F. ) ;
#67703=CARTESIAN_POINT ( 'NONE',  ( -7.825402957745083654, 6.891034867348166060, 3.271030448983516692 ) ) ;
#67705=CARTESIAN_POINT ( 'NONE',  ( -85.36298448216594181, 26.07611629625834127, 41.33332117284104612 ) ) ;
#67706=CARTESIAN_POINT ( 'NONE',  ( -31.43908319763709969, 10.61114334766716105, -23.47264677473818395 ) ) ;
#67707=CARTESIAN_POINT ( 'NONE',  ( 137.3958226571047021, 43.60243650158410844, 3.536823183464083087 ) ) ;
#67709=CARTESIAN_POINT ( 'NONE',  ( 116.6457744947906576, 31.95847117670280113, -47.33623488816716218 ) ) ;
#67710=CARTESIAN_POINT ( 'NONE',  ( 8.288451200428832877, 6.376395059685424194, 64.85115452999926333 ) ) ;
#67712=CARTESIAN_POINT ( 'NONE',  ( -72.19799221038252313, 21.02813487613374477, 87.79774528419648050 ) ) ;
#67718=VERTEX_POINT ( 'NONE', #40817 ) ;
#67720=CARTESIAN_POINT ( 'NONE',  ( -143.8566410313463564, 59.53044870492035301, 70.02296563317230493 ) ) ;
#67724=AXIS2_PLACEMENT_3D ( 'NONE', #19555, #68105, #13932 ) ;
#67725=CARTESIAN_POINT ( 'NONE',  ( -123.4416615615272974, 44.90042688650400038, 72.05607892409608439 ) ) ;
#67729=CARTESIAN_POINT ( 'NONE',  ( -47.80251179448168841, 13.89045662648309154, 39.80133545766267389 ) ) ;
#67733=CARTESIAN_POINT ( 'NONE',  ( 105.4193882736795871, 26.71329717705293305, 58.19139437044036356 ) ) ;
#67735=CARTESIAN_POINT ( 'NONE',  ( 164.9709596662455340, 63.72607097915128094, 64.01767799798439285 ) ) ;
#67739=CARTESIAN_POINT ( 'NONE',  ( 164.0298848570287191, 62.93631132702880393, -66.79358054371351727 ) ) ;
#67740=EDGE_LOOP ( 'NONE', ( #18966, #45108, #14319, #28346 ) ) ;
#67746=CARTESIAN_POINT ( 'NONE',  ( -78.66644367742111399, 22.32174330031318377, 57.26275173013680586 ) ) ;
#67749=CARTESIAN_POINT ( 'NONE',  ( -56.02289203441037557, 15.98631679403369965, 45.27020485907997482 ) ) ;
#67751=CARTESIAN_POINT ( 'NONE',  ( -33.12994257348895388, 10.89587983539684934, -76.97276311505544300 ) ) ;
#67752=CARTESIAN_POINT ( 'NONE',  ( 33.03722315490661998, 7.666819786578624729, 68.23343919241794708 ) ) ;
#67753=CARTESIAN_POINT ( 'NONE',  ( 9.823983574062877366, 6.382904402091118534, -20.74781057506424631 ) ) ;
#67756=CARTESIAN_POINT ( 'NONE',  ( -2.355184675731019528, 6.596450510445359683, -48.05484883106331040 ) ) ;
#67759=CARTESIAN_POINT ( 'NONE',  ( 63.98971758354224448, 12.90030016320049100, -62.61274705208756330 ) ) ;
#67760=CARTESIAN_POINT ( 'NONE',  ( 133.8566784816069344, 41.42467568809809109, -24.17876034193199786 ) ) ;
#67761=CARTESIAN_POINT ( 'NONE',  ( 23.09590709048884349, 7.852755081912510704, -14.46865910473645656 ) ) ;
#67762=CARTESIAN_POINT ( 'NONE',  ( -109.5142642360664382, 36.61018064014775319, -71.40685367841822995 ) ) ;
#67764=B_SPLINE_CURVE_WITH_KNOTS ( 'NONE', 3,
 ( #4579, #26044, #47475, #1039, #48846, #59070, #38313, #42886, #15825, #32012, #38670, #58720, #37973, #26730, #43586, #27060, #21440, #54837, #59417, #65408, #53440, #48159, #18708, #64351, #22138, #16164, #10535, #37618, #60116, #49202, #11936, #17198, #64014, #22490, #10887, #33408, #5604, #5270, #16856, #6658, #32358, #28108, #53782, #49551 ),
 .UNSPECIFIED., .F., .F.,
 ( 4, 2, 2, 2, 2, 2, 2, 2, 2, 2, 2, 2, 2, 2, 2, 2, 2, 2, 2, 2, 2, 4 ),
 ( 0.000000000000000000, 0.001473754749730514079, 0.002210632124595768300, 0.002947509499461028158, 0.004421264249191557416, 0.005895018998922086674, 0.007368773748652615065, 0.008105651123517878393, 0.008842528498383139118, 0.01031628324811366230, 0.01179003799784418549, 0.01252691537270942887, 0.01326379274757467051, 0.01473754749730515207, 0.01547442487217037463, 0.01621130224703559719, 0.01768505699676600762, 0.01915881174649641458, 0.01989568912136160939, 0.02063256649622680419, 0.02210632124595719034, 0.02358007599568757648 ),
 .UNSPECIFIED. ) ;
#67768=CARTESIAN_POINT ( 'NONE',  ( 130.3281282802763315, 40.49854652972196334, -50.15829713770070697 ) ) ;
#67771=CARTESIAN_POINT ( 'NONE',  ( 188.5838389098763059, 88.03667982118678026, -43.41585238266635827 ) ) ;
#67772=ORIENTED_EDGE ( 'NONE', *, *, #54937, .F. ) ;
#67774=EDGE_LOOP ( 'NONE', ( #8713, #19068 ) ) ;
#67780=CARTESIAN_POINT ( 'NONE',  ( 164.2142767676857318, 64.40413161136414999, 87.29693986084237167 ) ) ;
#67782=CARTESIAN_POINT ( 'NONE',  ( -62.14837099232445894, 17.75045801599140560, 13.41502600278767154 ) ) ;
#67784=CARTESIAN_POINT ( 'NONE',  ( -151.2511071212631464, 67.00426547928871912, 45.52856916683464306 ) ) ;
#67786=CARTESIAN_POINT ( 'NONE',  ( -99.98930671699733352, 31.63190627461932181, 30.86207369873248041 ) ) ;
#67790=CARTESIAN_POINT ( 'NONE',  ( 56.19211641164835669, 11.19288081156168246, 34.19031576763088509 ) ) ;
#67793=CARTESIAN_POINT ( 'NONE',  ( -170.2951623264596606, 85.51757001115471724, 18.43718488514699416 ) ) ;
#67794=CARTESIAN_POINT ( 'NONE',  ( 23.03578842369136481, 6.840884649289441732, -71.80884623865955518 ) ) ;
#67798=CARTESIAN_POINT ( 'NONE',  ( 157.4703587214989113, 57.65129005721576760, -51.12418429913766005 ) ) ;
#67801=CARTESIAN_POINT ( 'NONE',  ( 211.7318474105134385, 118.3631723164074714, -73.28989541382324546 ) ) ;
#67802=CARTESIAN_POINT ( 'NONE',  ( 137.6104751318277408, 44.92718313329108071, 30.51303313971197895 ) ) ;
#67803=FACE_OUTER_BOUND ( 'NONE', #67060, .T. ) ;
#67805=CARTESIAN_POINT ( 'NONE',  ( -102.2801239173131052, 32.78103895658057354, -76.85912785543962400 ) ) ;
#67810=CARTESIAN_POINT ( 'NONE',  ( -121.5680658099883829, 44.89994870382100345, -48.55882814402620795 ) ) ;
#67812=CARTESIAN_POINT ( 'NONE',  ( -48.39076722402981545, 12.99581395652485405, -92.93256446017095129 ) ) ;
#67815=CARTESIAN_POINT ( 'NONE',  ( 67.93317348534930034, 14.90531593353392026, -37.53674462394790368 ) ) ;
#67818=CARTESIAN_POINT ( 'NONE',  ( -118.6302575928420566, 43.07263081214308897, 40.00705528920811105 ) ) ;
#67819=CARTESIAN_POINT ( 'NONE',  ( 207.8484262634767106, 110.7633525054914259, 56.73326111006115013 ) ) ;
#67820=ORIENTED_EDGE ( 'NONE', *, *, #6991, .T. ) ;
#67822=CARTESIAN_POINT ( 'NONE',  ( -106.6711220790662651, 36.20923238211246797, 31.93402958823944715 ) ) ;
#67825=CARTESIAN_POINT ( 'NONE',  ( 82.80776120605499102, 19.20888523483863963, -90.50563713883087757 ) ) ;
#67828=ORIENTED_EDGE ( 'NONE', *, *, #58111, .T. ) ;
#67829=CARTESIAN_POINT ( 'NONE',  ( 8.000000000000007105, 249.8719672152120381, -95.00000000000133582 ) ) ;
#67831=CARTESIAN_POINT ( 'NONE',  ( 37.70910994512003356, 9.209110272746713122, 3.258713980646935404 ) ) ;
#67833=CARTESIAN_POINT ( 'NONE',  ( 35.65685430025423841, 7.951642554322393863, 17.08570462602523321 ) ) ;
#67834=CARTESIAN_POINT ( 'NONE',  ( -15.07533778868020491, 8.482826962130840087, -40.98183384572956811 ) ) ;
#67835=AXIS2_PLACEMENT_3D ( 'NONE', #37347, #68675, #57786 ) ;
#67837=CARTESIAN_POINT ( 'NONE',  ( -35.17718245314463843, 11.25729435722175964, -9.466008116007795792 ) ) ;
#67839=DIRECTION ( 'NONE',  ( 0.000000000000000000, 0.000000000000000000, 1.000000000000000000 ) ) ;
#67842=CARTESIAN_POINT ( 'NONE',  ( -55.05276343752908730, 15.72344139423348430, 72.16187836339486239 ) ) ;
#67843=CARTESIAN_POINT ( 'NONE',  ( -190.0468231512976445, 108.2116162189844744, 8.178919575991894675 ) ) ;
#67847=CARTESIAN_POINT ( 'NONE',  ( -31.93184248720558926, 9.672312402099827011, 45.21645440618920020 ) ) ;
#67848=CARTESIAN_POINT ( 'NONE',  ( 155.2870855780215038, 57.23765125306422163, -36.43485218074236087 ) ) ;
#67853=CARTESIAN_POINT ( 'NONE',  ( -156.1477286774994298, 71.38742644140636173, 68.56236523163960328 ) ) ;
#67856=CARTESIAN_POINT ( 'NONE',  ( -118.4063383664799574, 41.75753822095644097, 38.63033520264055198 ) ) ;
#67859=CARTESIAN_POINT ( 'NONE',  ( -174.7903139851460139, 90.53182997092832807, -61.73254058746562123 ) ) ;
#67860=CARTESIAN_POINT ( 'NONE',  ( 127.0856473832366049, 38.63797330894008297, 87.46917552659634509 ) ) ;
#67861=CARTESIAN_POINT ( 'NONE',  ( 117.4830770399667585, 32.37795270233553424, 39.13512077466761951 ) ) ;
#67864=CARTESIAN_POINT ( 'NONE',  ( -118.9468627709229338, 42.08677365399184822, -66.41956046915954914 ) ) ;
#67866=CARTESIAN_POINT ( 'NONE',  ( 203.1420903260745945, 104.2307086582027154, 44.08919628120091261 ) ) ;
#67868=CARTESIAN_POINT ( 'NONE',  ( 187.2384682876461852, 86.54721710842891014, 41.12445451989140821 ) ) ;
#67869=CARTESIAN_POINT ( 'NONE',  ( 185.4689022896543804, 83.15310303704600869, -91.31778852048856265 ) ) ;
#67874=CARTESIAN_POINT ( 'NONE',  ( 160.5018603162735360, 61.33906090758087970, -23.65429127533722209 ) ) ;
#67877=CARTESIAN_POINT ( 'NONE',  ( 66.07923263163412742, 14.44036440557998091, 57.30743532950679509 ) ) ;
#67878=CARTESIAN_POINT ( 'NONE',  ( 128.2147605031037472, 38.12058270760483936, 85.74602399063695657 ) ) ;
#67882=ORIENTED_EDGE ( 'NONE', *, *, #60582, .T. ) ;
#67883=CARTESIAN_POINT ( 'NONE',  ( 162.0862735437575566, 62.63196145447161456, -49.55485834045765614 ) ) ;
#67885=CARTESIAN_POINT ( 'NONE',  ( 157.4703587214989113, 57.65129005721576760, -51.12418429913766005 ) ) ;
#67888=CARTESIAN_POINT ( 'NONE',  ( -95.88693721180811735, 30.76307528361165922, 15.10402982153757989 ) ) ;
#67889=CARTESIAN_POINT ( 'NONE',  ( -130.1964689553232688, 49.39217932424202218, 44.28062280936351414 ) ) ;
#67894=CARTESIAN_POINT ( 'NONE',  ( 151.6192474229129061, 53.24103268919208887, 59.05513162150372608 ) ) ;
#67895=CARTESIAN_POINT ( 'NONE',  ( 93.32756701508620267, 22.89083686918420568, 40.62277632368491709 ) ) ;
#67896=ORIENTED_EDGE ( 'NONE', *, *, #18453, .T. ) ;
#67897=CARTESIAN_POINT ( 'NONE',  ( -99.10674985723790087, 32.31836975419496838, 58.05168674522651884 ) ) ;
#67898=CARTESIAN_POINT ( 'NONE',  ( -14.56151485655250255, 8.434196591921336861, 61.12604529331529335 ) ) ;
#67902=CARTESIAN_POINT ( 'NONE',  ( 102.7983318509014907, 26.68040613344516032, 36.06500074359141905 ) ) ;
#67903=CARTESIAN_POINT ( 'NONE',  ( -1.454841858088672391, 7.566772088227303072, 33.65001273355291289 ) ) ;
#67904=CARTESIAN_POINT ( 'NONE',  ( 56.30971345544048035, 11.21639176274772431, 94.42806938231223057 ) ) ;
#67905=CARTESIAN_POINT ( 'NONE',  ( 186.5979919519638202, 85.84756789133382426, 15.05375570133903551 ) ) ;
#67907=CARTESIAN_POINT ( 'NONE',  ( 209.6525588430077960, 113.3929734759396837, -49.46103483128387523 ) ) ;
#67908=CARTESIAN_POINT ( 'NONE',  ( 177.7960900018545090, 75.34533826015461955, 16.70855730554400154 ) ) ;
#67909=CARTESIAN_POINT ( 'NONE',  ( -58.76006735892197952, 15.70681061434693326, 4.448567267148194837 ) ) ;
#67914=ORIENTED_EDGE ( 'NONE', *, *, #6319, .F. ) ;
#67915=CARTESIAN_POINT ( 'NONE',  ( 102.7435092758397843, 25.56449004647816992, -69.99619280892473228 ) ) ;
#67919=CARTESIAN_POINT ( 'NONE',  ( -75.01314391403411719, 20.96328762434825066, 4.505560061529784832 ) ) ;
#67921=CARTESIAN_POINT ( 'NONE',  ( -6.538175632604766641, 6.809790034551946647, 83.88688884445680571 ) ) ;
#67924=CARTESIAN_POINT ( 'NONE',  ( -73.81689110552356681, 20.53332132481499883, 59.03636908666045713 ) ) ;
#67925=CARTESIAN_POINT ( 'NONE',  ( -165.6210506643949145, 79.15024150453835716, 65.46751455689062027 ) ) ;
#67927=VECTOR ( 'NONE', #65138, 1000.000000000000000 ) ;
#67930=CARTESIAN_POINT ( 'NONE',  ( -152.2964402771108894, 66.58174574061952455, 45.18655382497220074 ) ) ;
#67931=CYLINDRICAL_SURFACE ( 'NONE', #65908, 7.500000000000013323 ) ;
#67932=CARTESIAN_POINT ( 'NONE',  ( 181.0840389613909736, 78.60582251573003987, -9.380507075415925655 ) ) ;
#67941=CARTESIAN_POINT ( 'NONE',  ( 12.03162622199373821, 7.415834979634797541, 70.85525387039702139 ) ) ;
#67942=CARTESIAN_POINT ( 'NONE',  ( 209.9944361927104808, 113.8994774711241433, 31.39268359782400353 ) ) ;
#67943=CARTESIAN_POINT ( 'NONE',  ( 11.80882841624966773, 6.405741128846195842, -90.33718337654195807 ) ) ;
#67948=CARTESIAN_POINT ( 'NONE',  ( -118.6791382831902695, 43.10256062345757755, 89.73259551560695968 ) ) ;
#67949=CARTESIAN_POINT ( 'NONE',  ( 32.15613847490628530, 8.588587416860168133, -71.91613580555670637 ) ) ;
#67951=CARTESIAN_POINT ( 'NONE',  ( 11.74169691668609872, 6.404809784504847059, 84.88065130995101981 ) ) ;
#67953=ORIENTED_EDGE ( 'NONE', *, *, #68458, .T. ) ;
#67955=CARTESIAN_POINT ( 'NONE',  ( 199.7286177451875346, 101.4075663537892211, -49.46260000570829618 ) ) ;
#67957=CARTESIAN_POINT ( 'NONE',  ( -83.69653436244854561, 24.30167057287991028, 16.64215499319238489 ) ) ;
#67961=ORIENTED_EDGE ( 'NONE', *, *, #22078, .T. ) ;
#67962=VECTOR ( 'NONE', #59391, 1000.000000000000000 ) ;
#67964=CARTESIAN_POINT ( 'NONE',  ( 9.057575839850585453, 6.378493414438676901, -39.70112296040927902 ) ) ;
#67965=CARTESIAN_POINT ( 'NONE',  ( -109.1616641287093188, 37.56478347858660527, -93.21238446277425282 ) ) ;
#67966=CARTESIAN_POINT ( 'NONE',  ( 16.27765348919937338, 6.516472002017813736, 3.170157082241544799 ) ) ;
#67969=B_SPLINE_CURVE_WITH_KNOTS ( 'NONE', 3,
 ( #39109, #44359, #34533, #55974, #66893, #7786, #40141, #8127, #38751, #12013, #33486, #6732, #28179, #68263, #25360, #46440, #13748, #30625, #46792, #51729, #29929, #52745, #3536, #15132, #62278, #56660, #4238, #52072, #14096, #20067, #67921, #19025, #9862, #61921, #57701, #51394, #25007, #40476, #57013, #31319, #19367, #47467, #35555, #8832, #36594, #41868, #9164, #46097, #41520, #25702, #19718, #20398, #41178, #67566, #9511 ),
 .UNSPECIFIED., .F., .F.,
 ( 4, 2, 2, 2, 2, 2, 2, 2, 2, 2, 2, 2, 2, 2, 2, 2, 2, 2, 2, 1, 2, 2, 2, 2, 2, 2, 2, 4 ),
 ( 0.000000000000000000, 0.001947696403339872848, 0.002921544605009829872, 0.003895392806679787330, 0.004869241008349744354, 0.005843089210019701378, 0.006816937411689658402, 0.007790785613359616293, 0.009738482016699530341, 0.01071233021836948823, 0.01168617842003944439, 0.01266002662170940228, 0.01363387482337935844, 0.01460772302504931806, 0.01558157122671927422, 0.01752926763005918306, 0.01850311583172913749, 0.01947696403339909191, 0.02045081223506904633, 0.02142466043673900075, 0.02239850863840895517, 0.02337235684007890613, 0.02434620504174886055, 0.02532005324341881497, 0.02726774964675867871, 0.02824159784842859497, 0.02921544605009850776, 0.03116314245343833333 ),
 .UNSPECIFIED. ) ;
#67972=CARTESIAN_POINT ( 'NONE',  ( -31.77355346681724058, 9.646350159722794970, 83.90614663642915616 ) ) ;
#67974=CARTESIAN_POINT ( 'NONE',  ( 173.6024011093111028, 72.73634049052010653, -71.17273619272620522 ) ) ;
#67977=CARTESIAN_POINT ( 'NONE',  ( 102.7435092758398270, 25.56449004647818413, -43.15164221846109172 ) ) ;
#67978=CARTESIAN_POINT ( 'NONE',  ( 86.14890207173841929, 20.31981596387579714, -35.82156419891172305 ) ) ;
#67981=ORIENTED_EDGE ( 'NONE', *, *, #21796, .F. ) ;
#67982=CARTESIAN_POINT ( 'NONE',  ( -85.35172689181705152, 26.07142112926220889, -72.89607453545865212 ) ) ;
#67983=CARTESIAN_POINT ( 'NONE',  ( -0.6829546400373119885, 6.531019546548238353, -94.16435833651152620 ) ) ;
#67985=CARTESIAN_POINT ( 'NONE',  ( -125.8938041572051389, -170.0000000000000000, -15.56915330777026973 ) ) ;
#67986=CARTESIAN_POINT ( 'NONE',  ( 63.01563776193091826, -170.0000000000000000, 29.81296093922127710 ) ) ;
#67987=CARTESIAN_POINT ( 'NONE',  ( -190.6985136298602015, 109.1272424661243434, 69.71826505393651985 ) ) ;
#67989=CARTESIAN_POINT ( 'NONE',  ( 198.3462436126384318, 99.64019527131947029, 94.40446352108099859 ) ) ;
#67990=CARTESIAN_POINT ( 'NONE',  ( 209.6642862813004911, 115.2127693334913374, 31.07002473471074921 ) ) ;
#67991=CARTESIAN_POINT ( 'NONE',  ( -76.77329340382468104, 21.60914066444073356, -62.18705756154123776 ) ) ;
#67994=CARTESIAN_POINT ( 'NONE',  ( 11.21312910819263031, 7.403355431336986037, -22.13777925856294360 ) ) ;
#67995=EDGE_LOOP ( 'NONE', ( #25636, #1886 ) ) ;
#67997=CARTESIAN_POINT ( 'NONE',  ( 203.9276061909314421, 105.2889220654478919, -24.48138044215792419 ) ) ;
#68000=B_SPLINE_CURVE_WITH_KNOTS ( 'NONE', 3,
 ( #34649, #3650, #13857, #51836, #2970, #25123, #57125, #8598, #61699, #40939, #61358, #3308, #51159, #67687, #56084, #46553, #62398, #36010, #7899, #13524, #2617, #19477, #40252, #8937, #68034, #29020, #50460, #23728, #45175, #24081, #66654, #18449, #50801, #37727, #10296, #37374, #42322, #47925, #10641, #89, #57811, #15928, #31765, #20863, #63435, #64117, #48261, #20175, #15248, #25810 ),
 .UNSPECIFIED., .F., .F.,
 ( 4, 2, 2, 2, 2, 2, 2, 2, 2, 2, 2, 2, 2, 2, 2, 2, 2, 2, 2, 2, 2, 2, 2, 2, 4 ),
 ( 0.02688458561150013082, 0.02770990876165290578, 0.02853523191180568422, 0.03018587821211125150, 0.03183652451241681530, 0.03266184766256959721, 0.03348717081272237911, 0.03513781711302788741, 0.03678846341333340264, 0.03761378656348616373, 0.03843910971363892481, 0.03926443286379169284, 0.04008975601394445393, 0.04174040231425002467, 0.04256572546440282045, 0.04339104861455563011, 0.04421637176470843283, 0.04504169491486123555, 0.04586701806501403134, 0.04669234121516684100, 0.04834298751547252276, 0.04916831066562538100, 0.04999363381577824617, 0.05164428011608401814, 0.05329492641638979705 ),
 .UNSPECIFIED. ) ;
#68004=CARTESIAN_POINT ( 'NONE',  ( 36.08729376665094435, 8.001156100723207487, -36.37417898027339191 ) ) ;
#68006=CARTESIAN_POINT ( 'NONE',  ( 12.47451846520756291, 7.423604437114561527, -49.75163395661968480 ) ) ;
#68015=CARTESIAN_POINT ( 'NONE',  ( 8.480442907658517271, 6.376693431076493113, 12.37499517304073571 ) ) ;
#68020=CARTESIAN_POINT ( 'NONE',  ( 177.0075766083212159, 74.58167636505950782, -76.86931686656495799 ) ) ;
#68022=CARTESIAN_POINT ( 'NONE',  ( 88.30010642107258434, 19.99780058782973313, -9.161515012596032292 ) ) ;
#68023=CARTESIAN_POINT ( 'NONE',  ( -172.3018509397888351, 86.22053936367350957, 18.94384451952671000 ) ) ;
#68025=EDGE_CURVE ( 'NONE', #20757, #26499, #58538, .T. ) ;
#68029=B_SPLINE_CURVE_WITH_KNOTS ( 'NONE', 3,
 ( #33483, #22215, #39435, #28175, #11296, #34176, #27837, #32768, #16585, #49274, #49627, #1110, #17273, #16925, #38042, #6729, #11647, #44721, #5672, #1456, #22911, #7080, #33816, #6020, #38748, #60192, #12009, #49987, #44356, #43652, #1817, #65840, #33125, #17638, #60888, #12710, #27135, #54555, #39106, #48568, #48921, #402, #21860, #27480 ),
 .UNSPECIFIED., .F., .F.,
 ( 4, 2, 2, 2, 2, 2, 2, 2, 2, 2, 2, 2, 2, 2, 2, 2, 2, 2, 2, 2, 2, 4 ),
 ( 0.02416815208377490545, 0.02567033257376880734, 0.02642142281876576002, 0.02717251306376271269, 0.02867469355375657641, 0.02942578379875351868, 0.03017687404375045748, 0.03167905453374433855, 0.03318123502373822309, 0.03393232526873516536, 0.03468341551373210763, 0.03618559600372597829, 0.03693668624872289280, 0.03768777649371980731, 0.03918995698371364328, 0.04069213747370747924, 0.04219431796370130133, 0.04369649845369513730, 0.04444758869869204487, 0.04519867894368894551, 0.04670085943368275372, 0.04820303992367654805 ),
 .UNSPECIFIED. ) ;
#68031=CARTESIAN_POINT ( 'NONE',  ( -3.857727530059796628, 6.665032499723451132, 70.82944377365473088 ) ) ;
#68034=CARTESIAN_POINT ( 'NONE',  ( 149.9714610887122035, 53.28792066194170474, 63.44660927195447186 ) ) ;
#68035=CARTESIAN_POINT ( 'NONE',  ( -109.3585523124448002, 37.67345343047317385, -66.82677446236121455 ) ) ;
#68036=CARTESIAN_POINT ( 'NONE',  ( -54.57280099357650727, 14.55288945003959178, -50.21632399845989880 ) ) ;
#68038=CARTESIAN_POINT ( 'NONE',  ( -190.6985136298601731, 109.1272424661242582, 94.99999999999866418 ) ) ;
#68044=CARTESIAN_POINT ( 'NONE',  ( 177.7889574972182061, 75.33777460203560850, -50.47746129031760631 ) ) ;
#68046=CARTESIAN_POINT ( 'NONE',  ( 138.4714068233401179, 45.47397885319522004, -91.28743950027845244 ) ) ;
#68047=ORIENTED_EDGE ( 'NONE', *, *, #8491, .T. ) ;
#68053=CARTESIAN_POINT ( 'NONE',  ( -24.61094659556678010, 9.585225265507409276, -12.86029569530389161 ) ) ;
#68056=EDGE_CURVE ( 'NONE', #68729, #33041, #2378, .T. ) ;
#68058=DIRECTION ( 'NONE',  ( -0.000000000000000000, 1.000000000000000000, -0.000000000000000000 ) ) ;
#68061=CARTESIAN_POINT ( 'NONE',  ( 14.80582440982707482, 6.470883766728822373, 71.81066783346395255 ) ) ;
#68062=CARTESIAN_POINT ( 'NONE',  ( 198.2588776805010582, 99.52972231602375075, 32.85139680164935072 ) ) ;
#68063=CARTESIAN_POINT ( 'NONE',  ( -79.31924985377354176, 23.64871657882263989, 84.11086250148999000 ) ) ;
#68067=CARTESIAN_POINT ( 'NONE',  ( 65.62985354949975658, 14.32996029952554018, 44.34682454305074373 ) ) ;
#68071=CARTESIAN_POINT ( 'NONE',  ( 112.5612011511789916, 31.08353758940341294, -77.41542351236350328 ) ) ;
#68073=CARTESIAN_POINT ( 'NONE',  ( 198.4017331595408677, 98.09114638179337931, -74.75484424362443292 ) ) ;
#68074=VECTOR ( 'NONE', #66600, 1000.000000000000000 ) ;
#68076=CARTESIAN_POINT ( 'NONE',  ( -118.8689810167775818, 42.03922634358562505, 62.32420629194420059 ) ) ;
#68077=CARTESIAN_POINT ( 'NONE',  ( -81.00768240531211006, 24.30850321514434143, -22.90011388250445989 ) ) ;
#68080=CARTESIAN_POINT ( 'NONE',  ( -49.13048465129991627, 14.20828170588045403, 42.44559892615119168 ) ) ;
#68081=ORIENTED_EDGE ( 'NONE', *, *, #63110, .T. ) ;
#68083=ORIENTED_EDGE ( 'NONE', *, *, #59197, .F. ) ;
#68084=EDGE_CURVE ( 'NONE', #56804, #28889, #34283, .T. ) ;
#68086=CARTESIAN_POINT ( 'NONE',  ( 105.4375968828853729, 26.72149058755206852, 69.71918802570772300 ) ) ;
#68087=CARTESIAN_POINT ( 'NONE',  ( 112.5010186421628049, 29.94054703519628546, 83.64122026741506488 ) ) ;
#68091=CARTESIAN_POINT ( 'NONE',  ( -142.1950298130309420, 59.49693210460241488, 93.72120968998457613 ) ) ;
#68096=CARTESIAN_POINT ( 'NONE',  ( 178.3559415630091678, 75.89137766528514817, -90.41844760944908899 ) ) ;
#68099=CARTESIAN_POINT ( 'NONE',  ( -62.49137879463568623, 17.85440472148629354, 38.80717417638208389 ) ) ;
#68100=CARTESIAN_POINT ( 'NONE',  ( -37.07436112751821611, 11.60822760208520421, -64.68853167423618800 ) ) ;
#68101=CARTESIAN_POINT ( 'NONE',  ( 32.90953848114695290, 7.653665824624201974, 60.49547482373738916 ) ) ;
#68102=CARTESIAN_POINT ( 'NONE',  ( 46.23333927402088506, 9.396595540482447717, 87.98974472844928130 ) ) ;
#68104=ORIENTED_EDGE ( 'NONE', *, *, #16038, .F. ) ;
#68105=DIRECTION ( 'NONE',  ( -0.000000000000000000, 1.000000000000000000, -0.000000000000000000 ) ) ;
#68106=CARTESIAN_POINT ( 'NONE',  ( 187.5272808203427530, 85.37192123373903030, 59.77628873332410819 ) ) ;
#68108=CARTESIAN_POINT ( 'NONE',  ( 68.95451040317567504, 14.12887482153123564, -65.45849180363892117 ) ) ;
#68109=CARTESIAN_POINT ( 'NONE',  ( 18.19980344696536889, 6.589834367837006823, 57.25328788149280257 ) ) ;
#68111=CARTESIAN_POINT ( 'NONE',  ( 15.78827728214693416, 7.507518794609588042, 3.170157082241545687 ) ) ;
#68117=CARTESIAN_POINT ( 'NONE',  ( 126.6464677212869248, 38.39096133771043640, -45.65458962762210149 ) ) ;
#68118=CARTESIAN_POINT ( 'NONE',  ( -128.1219934350341703, 47.97781708504715681, -35.23767964644014938 ) ) ;
#68119=CARTESIAN_POINT ( 'NONE',  ( -108.1180879163842690, 36.99199941971028238, -37.77984450447672771 ) ) ;
#68120=CARTESIAN_POINT ( 'NONE',  ( 188.5842358232185632, 88.03712271786932320, -44.02448079173893802 ) ) ;
#68124=PRODUCT_DEFINITION_FORMATION_WITH_SPECIFIED_SOURCE ( 'ANY', '', #4024, .NOT_KNOWN. ) ;
#68130=CARTESIAN_POINT ( 'NONE',  ( 158.7714055544899168, 59.95166641265087293, 83.18787582866841035 ) ) ;
#68132=CARTESIAN_POINT ( 'NONE',  ( -62.50103539982530521, 17.85731685071834463, 9.961880401615221814 ) ) ;
#68133=CARTESIAN_POINT ( 'NONE',  ( 126.3541873520043737, 37.07520218256170352, 36.51082573705635070 ) ) ;
#68134=CARTESIAN_POINT ( 'NONE',  ( -154.6085044440278295, 69.98390342970671441, 32.71756333063028421 ) ) ;
#68145=EDGE_CURVE ( 'NONE', #3775, #44530, #68572, .T. ) ;
#68146=CARTESIAN_POINT ( 'NONE',  ( -176.3791001330699260, 90.82833141237287577, -8.597446401251650272 ) ) ;
#68147=CARTESIAN_POINT ( 'NONE',  ( -125.8938041572051389, 47.69968343338778993, 57.46449846362076386 ) ) ;
#68149=CARTESIAN_POINT ( 'NONE',  ( -109.4963484765719244, 37.74981983082538761, 93.77794043553710424 ) ) ;
#68150=EDGE_CURVE ( 'NONE', #38092, #30571, #65206, .T. ) ;
#68152=VERTEX_POINT ( 'NONE', #59659 ) ;
#68153=CARTESIAN_POINT ( 'NONE',  ( -58.76005811686689384, 15.70653557534865108, -9.334115721335656701 ) ) ;
#68155=CARTESIAN_POINT ( 'NONE',  ( 134.0849965622593061, 42.73957449886184179, 29.51034083899532945 ) ) ;
#68156=CARTESIAN_POINT ( 'NONE',  ( 114.6659427952414347, 32.10199811723106933, 43.18690178204667518 ) ) ;
#68157=LINE ( 'NONE', #24896, #42608 ) ;
#68158=CARTESIAN_POINT ( 'NONE',  ( 70.50376765786474209, 15.57629333413343353, -70.55552223763868369 ) ) ;
#68161=ORIENTED_EDGE ( 'NONE', *, *, #55160, .F. ) ;
#68166=CARTESIAN_POINT ( 'NONE',  ( -49.52089322850377329, 13.26777265051996224, -91.33638462665525992 ) ) ;
#68170=CARTESIAN_POINT ( 'NONE',  ( -145.3109762780891288, 60.69959559383372039, 44.45407750809701497 ) ) ;
#68172=CARTESIAN_POINT ( 'NONE',  ( 211.5066273949819902, 116.1727691518061647, 60.35867932873075148 ) ) ;
#68174=CARTESIAN_POINT ( 'NONE',  ( -109.0291978193666580, 37.49173305805087608, 34.73816087405813846 ) ) ;
#68176=CARTESIAN_POINT ( 'NONE',  ( -31.43908319763709258, 9.591432048623765638, 18.37190381572551701 ) ) ;
#68178=CARTESIAN_POINT ( 'NONE',  ( 80.15818551272217007, 18.36718314243334049, 67.88017848172013657 ) ) ;
#68182=CARTESIAN_POINT ( 'NONE',  ( 36.09469435220862721, 9.015003538710486097, 3.820264011147788796 ) ) ;
#68184=CARTESIAN_POINT ( 'NONE',  ( 32.67604596315970866, 7.629767358313821468, 7.241655292760623475 ) ) ;
#68186=CARTESIAN_POINT ( 'NONE',  ( -38.69449158134467126, 11.92067517118076836, -17.93520783166486154 ) ) ;
#68187=ORIENTED_EDGE ( 'NONE', *, *, #29858, .F. ) ;
#68188=CARTESIAN_POINT ( 'NONE',  ( -118.6704545714847114, 43.09717372409259184, -94.02806988937946642 ) ) ;
#68191=CARTESIAN_POINT ( 'NONE',  ( 8.537735592981560373, 7.383000420390737339, -67.92956672507523308 ) ) ;
#68192=CARTESIAN_POINT ( 'NONE',  ( -189.2352924136013144, 107.0839554967700735, 11.13131724358098573 ) ) ;
#68193=CARTESIAN_POINT ( 'NONE',  ( -78.66644367742111399, -170.0000000000000000, 30.41820113967310490 ) ) ;
#68194=CARTESIAN_POINT ( 'NONE',  ( -14.32120159453990205, 7.401444311907545703, -73.51966526291316484 ) ) ;
#68195=CARTESIAN_POINT ( 'NONE',  ( -95.19652294162978023, 29.32558722310179888, -13.15270443607074036 ) ) ;
#68198=CARTESIAN_POINT ( 'NONE',  ( -151.6648563624119106, 67.36546864992756412, 57.86878014402077497 ) ) ;
#68199=CARTESIAN_POINT ( 'NONE',  ( -119.2682179969168317, 42.28333404791698769, 41.67301999128292067 ) ) ;
#68204=CARTESIAN_POINT ( 'NONE',  ( 135.1592029508519488, 43.39714837287904459, 83.30687946948802391 ) ) ;
#68205=CARTESIAN_POINT ( 'NONE',  ( 203.0737501689026772, 105.8313166752871410, -90.18532627228834997 ) ) ;
#68206=DIRECTION ( 'NONE',  ( -0.000000000000000000, 1.000000000000000000, -0.000000000000000000 ) ) ;
#68207=AXIS2_PLACEMENT_3D ( 'NONE', #40736, #51313, #14012 ) ;
#68210=CARTESIAN_POINT ( 'NONE',  ( 197.5334904971816457, 97.00846725096930356, 38.94895049893467842 ) ) ;
#68211=CARTESIAN_POINT ( 'NONE',  ( 114.6632852039171411, 30.98120524556724575, -76.33079645022053228 ) ) ;
#68212=VECTOR ( 'NONE', #16084, 1000.000000000000000 ) ;
#68213=CARTESIAN_POINT ( 'NONE',  ( 182.7686108735401262, 81.77235358504609053, 29.48784566593629108 ) ) ;
#68214=CARTESIAN_POINT ( 'NONE',  ( 186.6368918226156381, 84.40539020454804131, -92.35556283223742469 ) ) ;
#68215=CARTESIAN_POINT ( 'NONE',  ( 181.0840389613909736, 80.03940679743416808, -24.38050707541595230 ) ) ;
#68218=CARTESIAN_POINT ( 'NONE',  ( 173.5844030397475706, 72.71952271766126330, 63.34818945125900314 ) ) ;
#68219=EDGE_CURVE ( 'NONE', #52360, #47781, #51831, .T. ) ;
#68220=ORIENTED_EDGE ( 'NONE', *, *, #15710, .F. ) ;
#68222=CARTESIAN_POINT ( 'NONE',  ( 70.50376765786472788, 15.57629333413343353, 63.66723071467976780 ) ) ;
#68223=CARTESIAN_POINT ( 'NONE',  ( 140.3784951150909706, 45.50429060678176540, 94.41964330782973036 ) ) ;
#68224=CARTESIAN_POINT ( 'NONE',  ( 156.3797504404255960, 58.07856685387021400, 2.641341998005292790 ) ) ;
#68226=CARTESIAN_POINT ( 'NONE',  ( -178.7483298110140026, 93.61800926271540391, 33.35710972951046926 ) ) ;
#68229=CARTESIAN_POINT ( 'NONE',  ( 113.4418023215250457, 31.50656691678295473, -50.22257324304041504 ) ) ;
#68232=CARTESIAN_POINT ( 'NONE',  ( -132.9109786433856470, 51.29129389542020334, 40.78060923209528710 ) ) ;
#68235=CARTESIAN_POINT ( 'NONE',  ( 79.92842440418705507, 18.29578799637230802, -19.88223195959437817 ) ) ;
#68236=CARTESIAN_POINT ( 'NONE',  ( -179.2112745835413250, 95.75131705262997173, -91.51719380277768323 ) ) ;
#68237=CARTESIAN_POINT ( 'NONE',  ( 156.5977259323288422, 56.97512126940428345, 56.29186946110193190 ) ) ;
#68239=B_SPLINE_CURVE_WITH_KNOTS ( 'NONE', 3,
 ( #16045, #10765, #19336, #40792, #35528, #32232, #15704, #46410, #26945, #67889, #56983, #19684, #21666, #62610, #35870, #57325, #52046, #46764, #68232, #42436, #63893, #37154, #10416, #31885, #53315, #54711, #6539, #48722, #1257, #60696, #59983, #49074, #65636, #38191, #17426, #33283, #64937, #28697, #38904, #32915, #6879, #60347, #12512, #66352, #65277, #39252 ),
 .UNSPECIFIED., .F., .F.,
 ( 4, 2, 2, 2, 2, 2, 2, 2, 2, 2, 2, 2, 2, 2, 2, 2, 2, 2, 2, 2, 2, 2, 4 ),
 ( 0.000000000000000000, 0.001615199098318934479, 0.003230398196637868959, 0.004037997745797377615, 0.004845597294956887138, 0.006460796393275913124, 0.007268395942435457342, 0.008075995491595001560, 0.009691194589914039689, 0.01049879413907356569, 0.01130639368823308996, 0.01211399323739261770, 0.01292159278655214197, 0.01453679188487121306, 0.01615199098319028415, 0.01695959053234980321, 0.01776719008150931881, 0.01938238917982828408, 0.02099758827814724935, 0.02180518782730669555, 0.02261278737646613829, 0.02422798647478502376, 0.02584318557310390577 ),
 .UNSPECIFIED. ) ;
#68241=ORIENTED_EDGE ( 'NONE', *, *, #9966, .T. ) ;
#68243=EDGE_LOOP ( 'NONE', ( #28760, #53155, #57869, #54864 ) ) ;
#68246=CARTESIAN_POINT ( 'NONE',  ( 152.2924710224605462, 54.98503313872889464, -11.34835473471603251 ) ) ;
#68247=CARTESIAN_POINT ( 'NONE',  ( -50.89568506533820624, 13.60612807157325932, 85.25567205612109944 ) ) ;
#68248=CARTESIAN_POINT ( 'NONE',  ( 109.7732660198864352, 29.77277639096405792, 44.61121420573733332 ) ) ;
#68249=CARTESIAN_POINT ( 'NONE',  ( -3.253130881186330203, 7.643323950922362719, 31.65042780773105591 ) ) ;
#68251=CARTESIAN_POINT ( 'NONE',  ( 110.2429982417149574, -170.0000000000000000, 29.61121420573730489 ) ) ;
#68252=CARTESIAN_POINT ( 'NONE',  ( 184.0001683447904099, 83.06228184427189376, 3.040735668703873795 ) ) ;
#68253=CARTESIAN_POINT ( 'NONE',  ( 212.1962110267000128, 117.2292732107320745, -44.20259310511458040 ) ) ;
#68254=CARTESIAN_POINT ( 'NONE',  ( 175.3815143714021190, 73.02838262206998365, 14.84218311195780515 ) ) ;
#68259=CARTESIAN_POINT ( 'NONE',  ( -76.10382222627279702, 22.43453174720079701, 71.81548357156262341 ) ) ;
#68261=CARTESIAN_POINT ( 'NONE',  ( 56.30171512201000183, 11.21502580416395745, -66.71341671416431041 ) ) ;
#68263=CARTESIAN_POINT ( 'NONE',  ( -14.61478091870810836, 7.428644888894361920, 88.10153567374477745 ) ) ;
#68265=CARTESIAN_POINT ( 'NONE',  ( -107.0809603157386789, 36.42942792191065848, -9.887358038569741936 ) ) ;
#68267=CARTESIAN_POINT ( 'NONE',  ( -71.17819443284075476, 19.60909329639480703, 65.25372451627271175 ) ) ;
#68268=CARTESIAN_POINT ( 'NONE',  ( 198.0154285049043779, 97.60753634768724396, -94.07841319457926943 ) ) ;
#68271=CARTESIAN_POINT ( 'NONE',  ( -155.1355020251929488, 69.10372769512069624, 33.23808801693751036 ) ) ;
#68272=DIRECTION ( 'NONE',  ( -0.000000000000000000, 0.000000000000000000, -1.000000000000000000 ) ) ;
#68273=CARTESIAN_POINT ( 'NONE',  ( 174.6127059037622757, 72.30368563770913681, -20.71086728071027139 ) ) ;
#68280=CARTESIAN_POINT ( 'NONE',  ( 211.7419975634644516, 116.5322580952101816, 7.208722705538775699 ) ) ;
#68282=CARTESIAN_POINT ( 'NONE',  ( 208.5889601154908632, 111.8333159387241835, 30.28245035469031876 ) ) ;
#68287=VERTEX_POINT ( 'NONE', #55085 ) ;
#68289=CARTESIAN_POINT ( 'NONE',  ( -133.3762944804928736, 52.85946325787776345, 92.42369384535366805 ) ) ;
#68290=CARTESIAN_POINT ( 'NONE',  ( -167.9853834315979384, 81.58767916550895904, -9.881304815344739367 ) ) ;
#68291=DIRECTION ( 'NONE',  ( 0.000000000000000000, 0.000000000000000000, 1.000000000000000000 ) ) ;
#68292=CARTESIAN_POINT ( 'NONE',  ( 21.94853621138365440, 6.775987044338161347, 86.91307455820552264 ) ) ;
#68293=LINE ( 'NONE', #13441, #17591 ) ;
#68298=CARTESIAN_POINT ( 'NONE',  ( -101.8145602049406051, 32.54453702486150490, 72.36362509687884881 ) ) ;
#68302=CARTESIAN_POINT ( 'NONE',  ( -86.06016868996614733, 25.27707703029501829, 12.35716539879548392 ) ) ;
#68303=ORIENTED_EDGE ( 'NONE', *, *, #20198, .F. ) ;
#68304=CARTESIAN_POINT ( 'NONE',  ( -59.96408504033276898, 17.10126854471815605, -10.18249688487181004 ) ) ;
#68306=EDGE_CURVE ( 'NONE', #23284, #29832, #13241, .T. ) ;
#68308=CARTESIAN_POINT ( 'NONE',  ( 8.951900209438534262, 6.378066731449592908, -46.11318404853862063 ) ) ;
#68311=CARTESIAN_POINT ( 'NONE',  ( 132.0440382699655402, 40.34028297386452522, 56.56290485416193548 ) ) ;
#68313=CARTESIAN_POINT ( 'NONE',  ( -24.32567406192871573, 8.531457175616735000, 93.80475582042849680 ) ) ;
#68315=CARTESIAN_POINT ( 'NONE',  ( 173.5836858989432301, 72.71885240881779566, -70.28283204199895806 ) ) ;
#68317=CARTESIAN_POINT ( 'NONE',  ( 108.3819860115547442, 28.02992728837241287, -50.70304034602167320 ) ) ;
#68319=LINE ( 'NONE', #51450, #16336 ) ;
#68323=ADVANCED_FACE ( 'NONE', ( #45234 ), #66712, .F. ) ;
#68325=CARTESIAN_POINT ( 'NONE',  ( -79.14094329813316619, 23.58034730000059653, -76.96000122218161721 ) ) ;
#68328=CARTESIAN_POINT ( 'NONE',  ( -55.05276343752909440, 14.68156374112637863, 45.31732777293115788 ) ) ;
#68329=CARTESIAN_POINT ( 'NONE',  ( 139.3639069815893379, 44.85046254673765986, -92.10545781260216813 ) ) ;
#68330=CARTESIAN_POINT ( 'NONE',  ( -151.2497169612549044, 65.66843968092749151, 18.72541422205654982 ) ) ;
#68331=CARTESIAN_POINT ( 'NONE',  ( -118.9668643994983768, 43.27909474462865091, -66.37097778377670920 ) ) ;
#68333=CARTESIAN_POINT ( 'NONE',  ( -149.5074843970971301, -170.0000000000000000, -15.46827994102828541 ) ) ;
#68334=CARTESIAN_POINT ( 'NONE',  ( -104.5730787903383003, 33.96058035148152499, 45.17567448190496293 ) ) ;
#68336=CARTESIAN_POINT ( 'NONE',  ( -62.03553610864626222, 17.71631625146951805, 88.69311610642812127 ) ) ;
#68337=EDGE_LOOP ( 'NONE', ( #28533, #14742, #21814, #55196 ) ) ;
#68338=CARTESIAN_POINT ( 'NONE',  ( 199.7278513351971299, 99.76879341361770059, -11.34529423773141232 ) ) ;
#68339=ORIENTED_EDGE ( 'NONE', *, *, #35506, .F. ) ;
#68340=CARTESIAN_POINT ( 'NONE',  ( 15.78827728214693416, 7.507518794609589818, -77.36349468914950478 ) ) ;
#68344=CARTESIAN_POINT ( 'NONE',  ( 141.3556389957210513, 47.34429831367556574, -43.22740683371433335 ) ) ;
#68345=CARTESIAN_POINT ( 'NONE',  ( 205.3776734260163153, 109.0011436241188818, -90.01503221354894890 ) ) ;
#68346=CARTESIAN_POINT ( 'NONE',  ( 8.287863202055541834, 7.382585476140734571, -42.53069974475695147 ) ) ;
#68348=CARTESIAN_POINT ( 'NONE',  ( 126.9201538765324386, 37.39093565120714402, -40.65955411680997855 ) ) ;
#68354=DIRECTION ( 'NONE',  ( -1.000000000000000000, 0.000000000000000000, 0.000000000000000000 ) ) ;
#68357=CARTESIAN_POINT ( 'NONE',  ( 10.83046137699561839, 6.392429922561260192, 16.31901005528300175 ) ) ;
#68361=CARTESIAN_POINT ( 'NONE',  ( 173.7246046907419554, 71.47482343504560731, -69.09541590300931091 ) ) ;
#68364=CARTESIAN_POINT ( 'NONE',  ( 93.32502112557678231, 21.81526022999039682, -19.89247016698760362 ) ) ;
#68365=CARTESIAN_POINT ( 'NONE',  ( -25.80443741485379761, 9.749985135376006085, 69.53500943053950323 ) ) ;
#68370=CARTESIAN_POINT ( 'NONE',  ( 126.4633682455862385, 38.28837286275647500, 11.45369110127332313 ) ) ;
#68371=CARTESIAN_POINT ( 'NONE',  ( 133.8566784816069344, 41.42467568809809109, -24.17876034193199786 ) ) ;
#68373=CARTESIAN_POINT ( 'NONE',  ( 8.000000000000007105, 249.8719672152120381, 94.99999999999866418 ) ) ;
#68374=CARTESIAN_POINT ( 'NONE',  ( -49.62489392740900485, 13.29305723289023966, -47.89781638457069590 ) ) ;
#68375=CARTESIAN_POINT ( 'NONE',  ( -125.8938041572051389, -170.0000000000000000, -15.56915330777026973 ) ) ;
#68377=ORIENTED_EDGE ( 'NONE', *, *, #12315, .F. ) ;
#68378=CARTESIAN_POINT ( 'NONE',  ( 59.72526569420002573, 11.93313563009889045, 17.22574484112362825 ) ) ;
#68380=CARTESIAN_POINT ( 'NONE',  ( -60.65612136648952912, 16.25551606627059087, 69.67105917315916486 ) ) ;
#68382=EDGE_LOOP ( 'NONE', ( #56032, #35329, #58689, #48226 ) ) ;
#68384=CARTESIAN_POINT ( 'NONE',  ( -173.5394735271662796, 87.59446374803710000, -76.55650775521371543 ) ) ;
#68385=DIRECTION ( 'NONE',  ( -0.000000000000000000, 1.000000000000000000, -0.000000000000000000 ) ) ;
#68388=FACE_OUTER_BOUND ( 'NONE', #30640, .T. ) ;
#68389=CARTESIAN_POINT ( 'NONE',  ( -4.725257700476000799, 6.708862164351557134, 17.60467424153223348 ) ) ;
#68392=CARTESIAN_POINT ( 'NONE',  ( -85.64924756730680144, 26.19583280090851218, 35.16995575340898483 ) ) ;
#68393=CARTESIAN_POINT ( 'NONE',  ( 149.9611936883170529, 52.04073442100943936, 90.49744601638548147 ) ) ;
#68394=CARTESIAN_POINT ( 'NONE',  ( 93.92910382125423041, 22.04227458821877761, 38.95172454535422446 ) ) ;
#68396=CARTESIAN_POINT ( 'NONE',  ( 133.8566784816069344, 41.42467568809808398, 2.665790248531674678 ) ) ;
#68397=CARTESIAN_POINT ( 'NONE',  ( -27.70115495247213033, 10.02455692117576369, 44.23695096961487394 ) ) ;
#68398=CARTESIAN_POINT ( 'NONE',  ( 203.1414537950835211, 105.9225671689748367, 44.05506648896800215 ) ) ;
#68403=CARTESIAN_POINT ( 'NONE',  ( 67.93317348534930034, 14.90531593353391671, 42.99690714744312459 ) ) ;
#68404=VERTEX_POINT ( 'NONE', #36682 ) ;
#68408=CARTESIAN_POINT ( 'NONE',  ( 117.0069443446175370, 33.26475960880693350, -67.01675685757288647 ) ) ;
#68413=CARTESIAN_POINT ( 'NONE',  ( -124.1033713525885247, 45.32626312604504903, 72.25125535819661593 ) ) ;
#68414=CARTESIAN_POINT ( 'NONE',  ( -86.06525741550316866, 26.37048289224655662, -14.51723273906646305 ) ) ;
#68419=CARTESIAN_POINT ( 'NONE',  ( -109.3585523124447576, 37.67345343047318806, 13.70687730902988477 ) ) ;
#68420=CARTESIAN_POINT ( 'NONE',  ( -86.11230725916330186, 26.39026888680171012, -43.64915368985550259 ) ) ;
#68421=CARTESIAN_POINT ( 'NONE',  ( 116.5854913516927951, 31.92838880174207716, 86.78310992652015443 ) ) ;
#68424=CARTESIAN_POINT ( 'NONE',  ( 103.0463737467386665, 25.69265572325593538, -95.00000000000133582 ) ) ;
#68425=CARTESIAN_POINT ( 'NONE',  ( 159.6725804802006223, 59.38339663535509061, -63.28528528614057791 ) ) ;
#68426=ORIENTED_EDGE ( 'NONE', *, *, #47776, .T. ) ;
#68428=ORIENTED_EDGE ( 'NONE', *, *, #8092, .T. ) ;
#68429=CARTESIAN_POINT ( 'NONE',  ( 38.91512155099543691, 9.360679678889628264, -50.61981746542778637 ) ) ;
#68431=CARTESIAN_POINT ( 'NONE',  ( -36.37229078872272936, 11.47648211215766167, -75.33199238139795284 ) ) ;
#68435=CARTESIAN_POINT ( 'NONE',  ( 8.540853903193184493, 6.376814430361479324, -14.22886706902527898 ) ) ;
#68437=CARTESIAN_POINT ( 'NONE',  ( 18.43272992546528855, 7.606837839440252935, 17.69278249756995081 ) ) ;
#68438=CARTESIAN_POINT ( 'NONE',  ( 188.5645326065591689, 86.51153908883290455, 63.03378560201070258 ) ) ;
#68439=CARTESIAN_POINT ( 'NONE',  ( -122.8118341587044711, 44.49743491855735300, 4.422630839854232221 ) ) ;
#68441=CARTESIAN_POINT ( 'NONE',  ( 130.7260704202055024, 39.56565398554880630, -23.51021375569008853 ) ) ;
#68442=DIRECTION ( 'NONE',  ( -0.000000000000000000, 1.000000000000000000, -0.000000000000000000 ) ) ;
#68444=CARTESIAN_POINT ( 'NONE',  ( 10.82760985890677397, 7.398654328676832925, 16.31652703457590547 ) ) ;
#68446=AXIS2_PLACEMENT_3D ( 'NONE', #63797, #68385, #26502 ) ;
#68448=CARTESIAN_POINT ( 'NONE',  ( 185.5415406465188823, 83.23025870924406888, 3.913947997146966618 ) ) ;
#68451=CARTESIAN_POINT ( 'NONE',  ( -149.5074843970971301, -170.0000000000000000, 57.56537183036274996 ) ) ;
#68452=CARTESIAN_POINT ( 'NONE',  ( 39.40195752203892710, 8.409560354027375340, -77.46436805589148378 ) ) ;
#68454=CARTESIAN_POINT ( 'NONE',  ( 188.4365915667138154, 87.87248959723052621, -42.21599812139930918 ) ) ;
#68458=EDGE_CURVE ( 'NONE', #5523, #2888, #8324, .T. ) ;
#68460=ORIENTED_EDGE ( 'NONE', *, *, #64362, .T. ) ;
#68462=CARTESIAN_POINT ( 'NONE',  ( 116.9200705848630548, 32.09536795999726166, 67.40972273578582019 ) ) ;
#68464=CARTESIAN_POINT ( 'NONE',  ( 128.4157044224114941, 39.39296260757095780, -75.55268868015734540 ) ) ;
#68465=CARTESIAN_POINT ( 'NONE',  ( 126.8947007444828046, 37.37669340849689092, 34.20897586740451146 ) ) ;
#68467=DIRECTION ( 'NONE',  ( 0.000000000000000000, -0.000000000000000000, -1.000000000000000000 ) ) ;
#68474=ORIENTED_EDGE ( 'NONE', *, *, #62422, .T. ) ;
#68475=CARTESIAN_POINT ( 'NONE',  ( -172.3127615181936676, 87.73358064377640630, 4.009540804375925305 ) ) ;
#68476=FACE_OUTER_BOUND ( 'NONE', #13760, .T. ) ;
#68477=CARTESIAN_POINT ( 'NONE',  ( -146.1201263095600780, 62.66021356509617135, -35.61751423064927735 ) ) ;
#68478=CARTESIAN_POINT ( 'NONE',  ( -129.6079169496902068, 50.20899308323962629, 71.48448238020641554 ) ) ;
#68480=LINE ( 'NONE', #36470, #52179 ) ;
#68486=CARTESIAN_POINT ( 'NONE',  ( -129.4036885357273547, 50.06837984316182144, -62.62615786572060728 ) ) ;
#68487=CARTESIAN_POINT ( 'NONE',  ( 63.01563776193091826, 12.67277567978495512, -89.40979201309708913 ) ) ;
#68492=EDGE_LOOP ( 'NONE', ( #15078, #21150, #47906, #67090 ) ) ;
#68493=CARTESIAN_POINT ( 'NONE',  ( 182.7789203043889756, 80.33475476315297215, -63.25125628519738541 ) ) ;
#68494=CARTESIAN_POINT ( 'NONE',  ( -172.3018509397888067, 86.22053936367352378, -34.74525666140065994 ) ) ;
#68497=CARTESIAN_POINT ( 'NONE',  ( 103.4725384926517222, 26.96797537091727293, -73.50340331479570466 ) ) ;
#68500=CARTESIAN_POINT ( 'NONE',  ( 67.54641595172913071, 14.80690682047551476, -37.22417361863564622 ) ) ;
#68501=CARTESIAN_POINT ( 'NONE',  ( -124.1095621208148572, 46.52671329146387791, 45.46233580508904026 ) ) ;
#68502=CARTESIAN_POINT ( 'NONE',  ( 210.4897348480408255, 114.6382060222044572, 58.78115735310451839 ) ) ;
#68504=CARTESIAN_POINT ( 'NONE',  ( -108.6634958860518196, 36.14357436892403541, -11.72466063708648143 ) ) ;
#68505=ORIENTED_EDGE ( 'NONE', *, *, #67074, .T. ) ;
#68506=CARTESIAN_POINT ( 'NONE',  ( -38.26732153931115477, 10.81230693396213738, 7.759653135233770982 ) ) ;
#68510=CARTESIAN_POINT ( 'NONE',  ( 38.91512155099545112, 9.360679678889628264, 3.069283715499573351 ) ) ;
#68512=CARTESIAN_POINT ( 'NONE',  ( 39.40195752203892710, 8.409560354027373563, 3.069283715499574683 ) ) ;
#68514=CARTESIAN_POINT ( 'NONE',  ( -37.37206033059243282, 11.66494618096612967, -20.56726544046575000 ) ) ;
#68516=EDGE_CURVE ( 'NONE', #4373, #38200, #58458, .T. ) ;
#68517=ORIENTED_EDGE ( 'NONE', *, *, #38675, .T. ) ;
#68522=CARTESIAN_POINT ( 'NONE',  ( -190.6985136298602015, 109.1272424661243434, 16.02916387300914280 ) ) ;
#68523=B_SPLINE_CURVE_WITH_KNOTS ( 'NONE', 3,
 ( #13410, #62285, #34182, #8484, #67244, #2855, #19027, #57017, #44727, #28544, #55618, #7789 ),
 .UNSPECIFIED., .F., .F.,
 ( 4, 2, 2, 2, 2, 4 ),
 ( 0.000000000000000000, 0.002485491944061524097, 0.004970983888123048193, 0.007456475832184572723, 0.008699221804215350601, 0.009941967776246129346 ),
 .UNSPECIFIED. ) ;
#68524=CARTESIAN_POINT ( 'NONE',  ( -78.66644367742111399, 23.39876645725287219, -50.11545063171791270 ) ) ;
#68525=CARTESIAN_POINT ( 'NONE',  ( -9.771516655894554759, 7.025139475821121415, -77.02225727686567325 ) ) ;
#68528=CARTESIAN_POINT ( 'NONE',  ( 152.2924710224605462, 54.98503313872889464, -38.19290532517972281 ) ) ;
#68534=CARTESIAN_POINT ( 'NONE',  ( 39.40195752203892710, -170.0000000000000000, -16.27526687496408542 ) ) ;
#68535=CARTESIAN_POINT ( 'NONE',  ( 180.2565361171340612, 79.19912802278402353, -24.34669578964250647 ) ) ;
#68536=CARTESIAN_POINT ( 'NONE',  ( -108.1180879163843116, 36.99199941971028949, 69.59835785737806191 ) ) ;
#68537=CARTESIAN_POINT ( 'NONE',  ( -127.4644500646574272, 48.74852676951793029, -49.75091178047936324 ) ) ;
#68538=VERTEX_POINT ( 'NONE', #9600 ) ;
#68540=CARTESIAN_POINT ( 'NONE',  ( -5.885876544836661672, 6.772369038004089070, -23.32255204279795890 ) ) ;
#68541=CARTESIAN_POINT ( 'NONE',  ( 204.6977192012829789, 108.0580384837234931, -90.01503221354883522 ) ) ;
#68544=CARTESIAN_POINT ( 'NONE',  ( 141.3403471770513136, 46.13063628128490024, 36.44774808231112218 ) ) ;
#68546=CARTESIAN_POINT ( 'NONE',  ( 197.2197025888162045, 96.62026035493821041, 36.04745238432391830 ) ) ;
#68549=CARTESIAN_POINT ( 'NONE',  ( 187.5246323291926842, 86.86207184872507980, 40.69048242448342734 ) ) ;
#68551=LINE ( 'NONE', #9814, #54330 ) ;
#68552=VECTOR ( 'NONE', #18815, 1000.000000000000000 ) ;
#68554=CARTESIAN_POINT ( 'NONE',  ( 174.9161599490640242, 73.97365196673301568, 59.37798453004636912 ) ) ;
#68555=ORIENTED_EDGE ( 'NONE', *, *, #23826, .T. ) ;
#68556=CARTESIAN_POINT ( 'NONE',  ( -108.0980548770427561, 35.83569586822708430, -37.75577146733352407 ) ) ;
#68557=CARTESIAN_POINT ( 'NONE',  ( 126.4375826614094507, 37.12160219610346701, 89.54261223166750483 ) ) ;
#68558=CARTESIAN_POINT ( 'NONE',  ( -57.65733424639442717, 15.39521790791522982, 44.85474620224701425 ) ) ;
#68559=CARTESIAN_POINT ( 'NONE',  ( 152.8672128926847904, 55.41186463791520111, 4.138895294562964899 ) ) ;
#68561=CARTESIAN_POINT ( 'NONE',  ( -173.1211646369891071, 87.12891641440859303, 45.82169460664104577 ) ) ;
#68564=CARTESIAN_POINT ( 'NONE',  ( 117.3145357257065342, 33.41973663092564095, -40.87229264417645425 ) ) ;
#68570=CARTESIAN_POINT ( 'NONE',  ( 141.3403471770513420, 46.13063628128487181, 63.29229867277483379 ) ) ;
#68571=CARTESIAN_POINT ( 'NONE',  ( -180.6209674222601791, 97.47999311542514533, 38.15503575396904523 ) ) ;
#68572=B_SPLINE_CURVE_WITH_KNOTS ( 'NONE', 3,
 ( #3795, #19273, #19982, #31231, #9079, #67825, #41085, #20657, #4487, #51979 ),
 .UNSPECIFIED., .F., .F.,
 ( 4, 2, 2, 2, 4 ),
 ( 0.000000000000000000, 0.002501040261221833608, 0.005002080522443667215, 0.007503120783665500823, 0.01000416104488733443 ),
 .UNSPECIFIED. ) ;
#68573=CARTESIAN_POINT ( 'NONE',  ( 150.0501577908836737, 52.10460126680128212, 64.87989132378601198 ) ) ;
#68574=CARTESIAN_POINT ( 'NONE',  ( 93.87111289824409255, 23.09598275302506920, 39.22769905219760744 ) ) ;
#68576=CARTESIAN_POINT ( 'NONE',  ( 45.35146934743634262, 10.27620685439442028, 15.16236855302814490 ) ) ;
#68579=CARTESIAN_POINT ( 'NONE',  ( 153.4509883044095773, 55.84811350575045452, -23.11593860723543870 ) ) ;
#68580=CARTESIAN_POINT ( 'NONE',  ( 212.0075063341773784, 118.7912820769029594, -18.69025613062296642 ) ) ;
#68581=CARTESIAN_POINT ( 'NONE',  ( 104.7227067006896419, 27.50728936118535017, 32.01079824686573261 ) ) ;
#68582=CARTESIAN_POINT ( 'NONE',  ( -155.7433525314458791, 69.65452735858370659, -64.98229209234851567 ) ) ;
#68584=CARTESIAN_POINT ( 'NONE',  ( 187.0788993276711949, 86.37277723143233743, 5.450255465685347467 ) ) ;
#68585=CARTESIAN_POINT ( 'NONE',  ( 210.9747454890631957, 115.3673079504856105, -39.71291949852400194 ) ) ;
#68590=CARTESIAN_POINT ( 'NONE',  ( 41.34269507549203126, 9.685203600174693506, -23.53625253713786236 ) ) ;
#68591=CARTESIAN_POINT ( 'NONE',  ( -78.19460645047368530, 22.14203592077028304, 3.573650549209445249 ) ) ;
#68594=CARTESIAN_POINT ( 'NONE',  ( 20.74561700410410836, 7.717362891868937425, 43.16396733258935825 ) ) ;
#68595=CARTESIAN_POINT ( 'NONE',  ( -107.2385267828037314, 36.51474259889400997, -21.30232734929181504 ) ) ;
#68597=CARTESIAN_POINT ( 'NONE',  ( -71.97434903038468690, 19.88430675376529777, 61.34002548381291575 ) ) ;
#68599=ORIENTED_EDGE ( 'NONE', *, *, #6009, .F. ) ;
#68601=CARTESIAN_POINT ( 'NONE',  ( -149.5074843970971301, 64.17983161892345834, 30.72082123989904900 ) ) ;
#68602=EDGE_CURVE ( 'NONE', #35856, #8573, #59493, .T. ) ;
#68606=CARTESIAN_POINT ( 'NONE',  ( -144.3945994505580757, 59.96115386701888639, 5.883885038153297664 ) ) ;
#68612=CARTESIAN_POINT ( 'NONE',  ( 209.6525588430077960, 113.3929734759397121, 4.228066349643490263 ) ) ;
#68613=CARTESIAN_POINT ( 'NONE',  ( -143.4048679855201271, 60.45763799613828837, 42.58799473479032116 ) ) ;
#68617=EDGE_CURVE ( 'NONE', #66303, #18940, #29164, .T. ) ;
#68621=CARTESIAN_POINT ( 'NONE',  ( -130.4988625216997775, 50.82592816381205125, 85.88177662789409794 ) ) ;
#68622=CYLINDRICAL_SURFACE ( 'NONE', #8328, 7.500000000000020428 ) ;
#68624=CARTESIAN_POINT ( 'NONE',  ( 17.09380310378440981, 6.545254173319234425, 83.78868157438149922 ) ) ;
#68625=CARTESIAN_POINT ( 'NONE',  ( 10.24659718932696251, 7.392712022583040721, 86.13955876464233086 ) ) ;
#68626=EDGE_LOOP ( 'NONE', ( #27082, #17882 ) ) ;
#68630=CARTESIAN_POINT ( 'NONE',  ( -79.14678386417813272, 22.50468917936072799, 18.57365054920947145 ) ) ;
#68633=VERTEX_POINT ( 'NONE', #22918 ) ;
#68634=ORIENTED_EDGE ( 'NONE', *, *, #8248, .F. ) ;
#68635=CARTESIAN_POINT ( 'NONE',  ( -119.5563837756079266, 43.64229894412653010, 15.31786711092669329 ) ) ;
#68636=CARTESIAN_POINT ( 'NONE',  ( -178.0658882571759989, 92.80593104957419825, 59.52230928071593041 ) ) ;
#68637=CARTESIAN_POINT ( 'NONE',  ( 21.44031696305384926, 6.747195267824408482, 15.62434647642277774 ) ) ;
#68639=CARTESIAN_POINT ( 'NONE',  ( -38.19016260632597692, 10.79737009263853587, 88.12259832690817518 ) ) ;
#68640=CARTESIAN_POINT ( 'NONE',  ( 175.8874477961784635, 74.89984466412603581, -65.14078283235144795 ) ) ;
#68642=CARTESIAN_POINT ( 'NONE',  ( 103.8317086685000135, 26.02720265156212776, -39.52255369601063961 ) ) ;
#68643=CARTESIAN_POINT ( 'NONE',  ( -23.98903001682803193, 8.486614814224626713, 36.72224464285193335 ) ) ;
#68644=CARTESIAN_POINT ( 'NONE',  ( -147.7895256390024485, 64.04409735547008609, -61.80240963661621834 ) ) ;
#68645=ORIENTED_EDGE ( 'NONE', *, *, #13433, .T. ) ;
#68648=CARTESIAN_POINT ( 'NONE',  ( -84.21836162213169530, 25.60181819557221772, -74.52576626856495068 ) ) ;
#68651=DIRECTION ( 'NONE',  ( -0.000000000000000000, 1.000000000000000000, -0.000000000000000000 ) ) ;
#68654=CARTESIAN_POINT ( 'NONE',  ( 130.3019683985926918, 39.31883119822050077, 3.544598928792382697 ) ) ;
#68655=CARTESIAN_POINT ( 'NONE',  ( -152.9121563765243650, 67.12206067149024591, 18.06274683814091020 ) ) ;
#68657=CARTESIAN_POINT ( 'NONE',  ( 210.0122310839192323, 115.7355030290287914, 42.02281805116941626 ) ) ;
#68658=CIRCLE ( 'NONE', #16979, 242.4895526022646379 ) ;
#68659=CARTESIAN_POINT ( 'NONE',  ( 163.2886151008987952, 62.32020850087172192, 5.325560534978804661 ) ) ;
#68660=CARTESIAN_POINT ( 'NONE',  ( -107.0751323097254755, 35.28386110859232616, 32.23120985814819761 ) ) ;
#68662=ORIENTED_EDGE ( 'NONE', *, *, #25985, .F. ) ;
#68667=CARTESIAN_POINT ( 'NONE',  ( 16.27775141556968208, 7.523247835309962106, -77.36349468914949057 ) ) ;
#68670=CYLINDRICAL_SURFACE ( 'NONE', #18735, 7.500000000000020428 ) ;
#68672=CARTESIAN_POINT ( 'NONE',  ( -28.13527276074847450, 10.08983026464524002, 4.134317294375541074 ) ) ;
#68673=CARTESIAN_POINT ( 'NONE',  ( 150.2076397309211586, 52.21780102759851161, -45.51576517098055774 ) ) ;
#68675=DIRECTION ( 'NONE',  ( -0.000000000000000000, 1.000000000000000000, -0.000000000000000000 ) ) ;
#68677=EDGE_CURVE ( 'NONE', #24352, #39302, #44363, .T. ) ;
#68685=CARTESIAN_POINT ( 'NONE',  ( 45.76553115525425852, 10.34124506813255095, -73.94115800944651085 ) ) ;
#68687=CARTESIAN_POINT ( 'NONE',  ( 175.5493994043409884, 73.18740965572598611, -65.50213383789414934 ) ) ;
#68688=CARTESIAN_POINT ( 'NONE',  ( -179.9014775667593540, 95.00669833041663992, -45.42960845675160897 ) ) ;
#68689=CARTESIAN_POINT ( 'NONE',  ( 91.67571176799447130, 21.20498955963028820, -22.03065998410063386 ) ) ;
#68690=CARTESIAN_POINT ( 'NONE',  ( -28.81071653159243340, 10.19258396314335080, 71.58963725187859950 ) ) ;
#68692=CARTESIAN_POINT ( 'NONE',  ( 162.7963212667074231, 63.21900188423068556, 69.04028839148755026 ) ) ;
#68695=CARTESIAN_POINT ( 'NONE',  ( 131.6115093721024607, 41.25402743071399669, 3.006001826248324793 ) ) ;
#68699=CARTESIAN_POINT ( 'NONE',  ( -107.7677210873466294, 36.80113675102408877, -74.49435489715372682 ) ) ;
#68700=CARTESIAN_POINT ( 'NONE',  ( -49.11825192196926793, 13.17012322555987680, -38.10387704635710548 ) ) ;
#68701=EDGE_CURVE ( 'NONE', #10310, #21823, #64787, .T. ) ;
#68703=CARTESIAN_POINT ( 'NONE',  ( -0.4228358876318114024, 7.528738343310879877, 92.55318377967873289 ) ) ;
#68705=VERTEX_POINT ( 'NONE', #56663 ) ;
#68706=CARTESIAN_POINT ( 'NONE',  ( -62.15324028806257672, 16.70091357159901335, 67.12728702411425274 ) ) ;
#68709=EDGE_LOOP ( 'NONE', ( #32954, #972, #12882, #35080 ) ) ;
#68710=CARTESIAN_POINT ( 'NONE',  ( 41.68362887572859421, 9.733053242893493717, 83.95093237084830662 ) ) ;
#68712=DIRECTION ( 'NONE',  ( -0.8118923937861950435, -0.5838071093367415143, 0.000000000000000000 ) ) ;
#68716=CARTESIAN_POINT ( 'NONE',  ( 31.95008798096003133, 7.556925044648908241, -15.29275533313533408 ) ) ;
#68718=CARTESIAN_POINT ( 'NONE',  ( -149.9471644042847061, 65.87751327280744817, -76.64767939074971537 ) ) ;
#68719=CARTESIAN_POINT ( 'NONE',  ( 93.86680996363769225, 22.01878169039502708, 39.19500198369756561 ) ) ;
#68720=ORIENTED_EDGE ( 'NONE', *, *, #16205, .T. ) ;
#68722=CARTESIAN_POINT ( 'NONE',  ( 12.69192874957004236, 6.421326776602847453, 57.52382708451808213 ) ) ;
#68724=CARTESIAN_POINT ( 'NONE',  ( 198.7129816317746531, 100.1061386900356069, 41.23588947464686072 ) ) ;
#68727=EDGE_LOOP ( 'NONE', ( #42515, #15683, #7673, #6653 ) ) ;
#68729=VERTEX_POINT ( 'NONE', #29242 ) ;
#68731=ADVANCED_FACE ( 'NONE', ( #66546 ), #23961, .F. ) ;
#68732=CARTESIAN_POINT ( 'NONE',  ( 198.8687991397275425, 98.67887821384410074, -75.39677907356383457 ) ) ;
#68738=CARTESIAN_POINT ( 'NONE',  ( -156.0300823189602397, 69.91528270335483342, -46.05349014652669126 ) ) ;
#68743=CARTESIAN_POINT ( 'NONE',  ( -84.53753601793928851, 25.73343139558517478, -47.30913981394891721 ) ) ;
#68744=CARTESIAN_POINT ( 'NONE',  ( 103.0087611945305923, 25.67668113601890667, 92.80995230241677518 ) ) ;
#68745=CARTESIAN_POINT ( 'NONE',  ( -155.2836587093739240, 70.59655508952972980, 6.585747873642095129 ) ) ;
#68746=AXIS2_PLACEMENT_3D ( 'NONE', #21822, #1421, #11267 ) ;
#68748=DIRECTION ( 'NONE',  ( 0.000000000000000000, 0.000000000000000000, 1.000000000000000000 ) ) ;
#68749=CARTESIAN_POINT ( 'NONE',  ( -153.2251259997642023, 68.74288695996825993, 85.39013094563341610 ) ) ;
#68751=ADVANCED_FACE ( 'NONE', ( #61925 ), #39443, .F. ) ;
#68754=ORIENTED_EDGE ( 'NONE', *, *, #14057, .F. ) ;
#68756=VECTOR ( 'NONE', #30918, 1000.000000000000000 ) ;
#68758=CARTESIAN_POINT ( 'NONE',  ( 175.0129209324024089, 72.68029375226022637, -93.00527503831655451 ) ) ;
#68760=EDGE_CURVE ( 'NONE', #31066, #27441, #68523, .T. ) ;
#68762=LINE ( 'NONE', #51570, #45021 ) ;
#68764=CARTESIAN_POINT ( 'NONE',  ( 32.14349651933086705, 7.576119504381656711, 62.30723258595453729 ) ) ;
#68765=CARTESIAN_POINT ( 'NONE',  ( 12.69192874957004769, 6.421326776602847453, -23.00982468687297100 ) ) ;
#68766=CARTESIAN_POINT ( 'NONE',  ( 21.43750346857337874, 7.754771113113080538, 15.62753494944939625 ) ) ;
#68767=CARTESIAN_POINT ( 'NONE',  ( 185.5415406465189960, 83.23025870924408309, 57.60304917807435743 ) ) ;
#68768=CARTESIAN_POINT ( 'NONE',  ( -118.6157340058430236, 41.88485941274770141, 13.10580239523996049 ) ) ;
#68771=CARTESIAN_POINT ( 'NONE',  ( 21.74799039132243905, 7.772294950329606600, -11.59454531415493861 ) ) ;
#68772=CARTESIAN_POINT ( 'NONE',  ( 199.7255144154429161, 99.76581417577203581, 57.91832127983512635 ) ) ;
#68773=VERTEX_POINT ( 'NONE', #34873 ) ;
#68774=CARTESIAN_POINT ( 'NONE',  ( 188.5843222076478867, 86.53342480589847696, 10.26064979393518684 ) ) ;
#68776=CARTESIAN_POINT ( 'NONE',  ( 178.4027079424739384, 75.93756746109792743, 43.81623254374778753 ) ) ;
#68777=DIRECTION ( 'NONE',  ( 0.000000000000000000, 0.000000000000000000, 1.000000000000000000 ) ) ;
#68779=CARTESIAN_POINT ( 'NONE',  ( -102.7494334820056707, 34.14986869751098908, -35.01457726497590528 ) ) ;
#68781=CARTESIAN_POINT ( 'NONE',  ( 188.5651904823862708, 88.01586411309102687, -43.11409047739251577 ) ) ;
#68783=VERTEX_POINT ( 'NONE', #66206 ) ;
#68785=CARTESIAN_POINT ( 'NONE',  ( -28.35330809568271704, 9.105138953156455273, -9.132531776435367732 ) ) ;
#68786=CARTESIAN_POINT ( 'NONE',  ( 173.7926097690033771, 71.53801684183484610, 92.29874427387952096 ) ) ;
#68790=CARTESIAN_POINT ( 'NONE',  ( 117.0069443446175370, 33.26475960880692639, 67.20599609474545844 ) ) ;
#68803=CARTESIAN_POINT ( 'NONE',  ( -120.4816138481824908, 43.03185659245512085, -20.78403245137389987 ) ) ;
#68805=CARTESIAN_POINT ( 'NONE',  ( -180.3153482337535820, 95.51031295027645740, -13.22612429021853409 ) ) ;
#68807=ORIENTED_EDGE ( 'NONE', *, *, #5489, .F. ) ;
#68808=CARTESIAN_POINT ( 'NONE',  ( -109.7839076876610562, 37.90938796091269580, 91.47912654843170799 ) ) ;
#68811=ORIENTED_EDGE ( 'NONE', *, *, #65655, .T. ) ;
#68812=CARTESIAN_POINT ( 'NONE',  ( -59.94781924509481286, 16.04872117907065743, -10.18417756321730039 ) ) ;
#68813=CARTESIAN_POINT ( 'NONE',  ( -133.3944793432480367, 52.87251459353621641, -69.00333076711490321 ) ) ;
#68817=CARTESIAN_POINT ( 'NONE',  ( -96.02415295709707266, 29.71480036090586196, -73.50342397880682199 ) ) ;
#68820=CARTESIAN_POINT ( 'NONE',  ( 185.5572090022886016, 83.24697331286186852, -64.53146504295692409 ) ) ;
#68821=CARTESIAN_POINT ( 'NONE',  ( -166.9982296371934467, 80.56207291422407479, -46.55132158310039614 ) ) ;
#68823=CARTESIAN_POINT ( 'NONE',  ( 106.6181401479172308, 28.34160787025143335, -63.69676998527926060 ) ) ;
#68824=CARTESIAN_POINT ( 'NONE',  ( -77.71490760329791669, 23.03637365463981723, 30.46362590998626985 ) ) ;
#68825=CARTESIAN_POINT ( 'NONE',  ( 79.38020582286196714, 17.07365509555548755, 35.22343465671548302 ) ) ;
#68826=CARTESIAN_POINT ( 'NONE',  ( 63.50537371531939357, 13.81987663608981798, -35.72069083216972274 ) ) ;
#68829=EDGE_CURVE ( 'NONE', #48794, #5387, #39794, .T. ) ;
#68831=CARTESIAN_POINT ( 'NONE',  ( -105.8879439778144871, 34.65133284149108306, -22.26253636860239027 ) ) ;
#68833=CARTESIAN_POINT ( 'NONE',  ( -35.99019277275120743, 10.38248800679342310, 16.85316403250221740 ) ) ;
#68834=CARTESIAN_POINT ( 'NONE',  ( 79.91920957766411959, 18.29292522273511068, 67.44459320285845649 ) ) ;
#68835=EDGE_CURVE ( 'NONE', #39142, #40691, #64395, .T. ) ;
#68841=CARTESIAN_POINT ( 'NONE',  ( 34.83825437341838693, 7.859462995505729133, -75.93605119989038599 ) ) ;
#68842=CARTESIAN_POINT ( 'NONE',  ( -98.68609963468202295, 32.11186931716879656, -62.75914624374382100 ) ) ;
#68844=CARTESIAN_POINT ( 'NONE',  ( -36.00304714721387711, 11.40794940913596456, -10.00091909768606335 ) ) ;
#68848=ORIENTED_EDGE ( 'NONE', *, *, #23983, .F. ) ;
#68849=CARTESIAN_POINT ( 'NONE',  ( 59.30258796551119360, 12.87111270082601600, 57.62249339133282433 ) ) ;
#68850=CARTESIAN_POINT ( 'NONE',  ( -25.98312968277007329, 8.759224980175261521, 5.719980934363178449 ) ) ;
#68855=CARTESIAN_POINT ( 'NONE',  ( 152.1381498073141074, 54.87048121475569928, -48.92046709163152229 ) ) ;
#68859=CARTESIAN_POINT ( 'NONE',  ( -154.8006992380339000, 70.15733562427990933, 70.40004192881569622 ) ) ;
#68860=CARTESIAN_POINT ( 'NONE',  ( 173.6700117628886630, 72.79957362875114768, -15.71003057700986716 ) ) ;
#68862=CARTESIAN_POINT ( 'NONE',  ( -128.9843070188472893, 49.78011598923034597, -49.26255782700048513 ) ) ;
#68865=CARTESIAN_POINT ( 'NONE',  ( -6.851003965218993130, 6.829052369041586523, -23.52622361473696699 ) ) ;
#68867=CARTESIAN_POINT ( 'NONE',  ( 198.7123879174244223, 100.1053816708572555, -21.50880716110014035 ) ) ;
#68868=CARTESIAN_POINT ( 'NONE',  ( -151.7300473889874581, 66.08683396307566227, 84.72635355681168789 ) ) ;
#68869=CARTESIAN_POINT ( 'NONE',  ( 136.1310312718401860, 42.81430973242785853, 44.17212115549305906 ) ) ;
#68870=ORIENTED_EDGE ( 'NONE', *, *, #59283, .T. ) ;
#68871=CARTESIAN_POINT ( 'NONE',  ( 197.3685896092616190, 96.80423329231987850, 35.08436879187444646 ) ) ;
#68873=CARTESIAN_POINT ( 'NONE',  ( 184.3966782763551464, 83.48172388049827930, 30.06520294631881285 ) ) ;
#68875=CARTESIAN_POINT ( 'NONE',  ( -102.2801239173131194, 33.91021738430207932, 45.51907450641513009 ) ) ;
#68878=DIRECTION ( 'NONE',  ( 0.000000000000000000, 0.000000000000000000, 1.000000000000000000 ) ) ;
#68880=CARTESIAN_POINT ( 'NONE',  ( -71.97434903038468690, 19.88430675376528711, -19.19362628757813027 ) ) ;
#68883=CARTESIAN_POINT ( 'NONE',  ( -55.54058841405665703, 14.81234591756537888, 45.31732777293116499 ) ) ;
#68886=CARTESIAN_POINT ( 'NONE',  ( -180.6213815675304772, 95.88446356933845038, 38.01213868508001781 ) ) ;
#68890=ORIENTED_EDGE ( 'NONE', *, *, #3440, .T. ) ;
#68891=CARTESIAN_POINT ( 'NONE',  ( -173.1211646369891355, -170.0000000000000000, -95.90105834567735599 ) ) ;
#68895=VECTOR ( 'NONE', #51242, 1000.000000000000000 ) ;
#68896=CARTESIAN_POINT ( 'NONE',  ( 86.62931800182293784, 20.48449268398422518, -23.97701360844805407 ) ) ;
#68897=CARTESIAN_POINT ( 'NONE',  ( 141.2366329129481244, 46.06278879703609874, 62.49230329047843213 ) ) ;
#68899=CARTESIAN_POINT ( 'NONE',  ( -171.4814970982680222, 85.32124710276291069, 45.65206851958718914 ) ) ;
#68901=CARTESIAN_POINT ( 'NONE',  ( 153.2282895792479565, 54.42637815496158993, 57.56435675519129802 ) ) ;
#68904=CARTESIAN_POINT ( 'NONE',  ( 46.80475532923159676, 10.50744084852537163, 9.340717336282994054 ) ) ;
#68907=CARTESIAN_POINT ( 'NONE',  ( 151.1827182658834090, 54.16800928478855326, -20.89999102867709269 ) ) ;
#68908=CARTESIAN_POINT ( 'NONE',  ( -59.24627258934994245, 15.84537569346437458, 85.25633480741510084 ) ) ;
#68909=CARTESIAN_POINT ( 'NONE',  ( 103.1695711638930817, 26.83837309506527546, 34.56746450366944146 ) ) ;
#68912=CARTESIAN_POINT ( 'NONE',  ( 188.5838389098763344, 88.03667982118683710, 10.27324879826098503 ) ) ;
#68914=DIRECTION ( 'NONE',  ( 0.000000000000000000, 0.000000000000000000, 1.000000000000000000 ) ) ;
#68915=B_SPLINE_CURVE_WITH_KNOTS ( 'NONE', 3,
 ( #55313, #65898, #11704, #38448, #7132, #18041, #65537, #43703, #2215, #17330, #6782, #44056, #49678, #33871, #12066, #22969, #44415, #54965, #23665, #820, #28950, #33178, #38805, #39493, #44773, #54611, #59885, #60598, #23329, #66250, #6442, #28228, #60248, #1873, #22269, #34223, #28593, #50046, #55667, #60944, #65181, #12763, #16975, #49329 ),
 .UNSPECIFIED., .F., .F.,
 ( 4, 2, 2, 2, 2, 2, 2, 2, 2, 2, 2, 2, 2, 2, 2, 2, 2, 2, 2, 2, 2, 4 ),
 ( 1.398578778534940505E-17, 0.001487235713946735011, 0.002230853570920115960, 0.002974471427893496910, 0.004461707141840256206, 0.005948942855787015503, 0.007436178569733774800, 0.008179796426707155316, 0.008923414283680533229, 0.01041064999762730467, 0.01189788571157407611, 0.01264150356854745749, 0.01338512142552083888, 0.01487235713946760164, 0.01561597499644099343, 0.01635959285341438349, 0.01784682856736116360, 0.01933406428130794372, 0.02007768213828133724, 0.02082129999525472730, 0.02230853570920151435, 0.02379577142314830140 ),
 .UNSPECIFIED. ) ;
#68918=ORIENTED_EDGE ( 'NONE', *, *, #68701, .F. ) ;
#68919=CARTESIAN_POINT ( 'NONE',  ( -75.43271753227890031, 22.18711452892411273, 71.54694186117023946 ) ) ;
#68922=CARTESIAN_POINT ( 'NONE',  ( 59.72897338775215559, 11.93428797217974591, -76.81118384515825426 ) ) ;
#68926=CARTESIAN_POINT ( 'NONE',  ( 20.74185656603722450, 7.717159106492252896, 31.86164482231723127 ) ) ;
#68927=CARTESIAN_POINT ( 'NONE',  ( 158.3636111008086687, 59.62671916656143623, -62.96873488960133614 ) ) ;
#68931=ORIENTED_EDGE ( 'NONE', *, *, #58076, .F. ) ;
#68933=CARTESIAN_POINT ( 'NONE',  ( -155.1302201283146189, 69.09929365814133462, 43.19023084304400584 ) ) ;
#68934=CARTESIAN_POINT ( 'NONE',  ( 55.56474667084417263, 11.06706367715628581, -42.22808952694573037 ) ) ;
#68938=CARTESIAN_POINT ( 'NONE',  ( -145.3279998500303520, 60.71393190715791377, 5.144276485782331321 ) ) ;
#68940=CARTESIAN_POINT ( 'NONE',  ( -132.4896623150434039, 52.22616402022728721, 41.69918907009083142 ) ) ;
#68942=CARTESIAN_POINT ( 'NONE',  ( 204.6977192012829789, 106.3443248447423599, 2.363170148305747009 ) ) ;
#68943=LINE ( 'NONE', #16175, #36077 ) ;
#68945=CARTESIAN_POINT ( 'NONE',  ( 210.1954643503416094, 114.1986276268024056, 41.81508267376618448 ) ) ;
#68946=CARTESIAN_POINT ( 'NONE',  ( -7.825402957745085430, 7.899365992529246761, 71.96013162991091860 ) ) ;
#68954=AXIS2_PLACEMENT_3D ( 'NONE', #16511, #6652, #54475 ) ;
#68955=CARTESIAN_POINT ( 'NONE',  ( 36.30999198706539488, 9.040534725358943646, -63.12703590951987564 ) ) ;
#68958=CARTESIAN_POINT ( 'NONE',  ( 12.60448962010195473, 7.425467749510118232, 84.38144641662934475 ) ) ;
#68960=DIRECTION ( 'NONE',  ( -0.000000000000000000, 1.000000000000000000, -0.000000000000000000 ) ) ;
#68963=CARTESIAN_POINT ( 'NONE',  ( -86.06489347855098515, 25.27905598459106784, 9.817369700168111279 ) ) ;
#68967=CARTESIAN_POINT ( 'NONE',  ( -123.0348077379026819, 45.83489305753315790, 18.21289688529726192 ) ) ;
#68970=CARTESIAN_POINT ( 'NONE',  ( 126.9201538765324671, 37.39093565120717244, 66.71864824504474711 ) ) ;
#68973=CARTESIAN_POINT ( 'NONE',  ( -38.80050246754539245, 10.91612181589391284, 92.87695660739120740 ) ) ;
#68974=CARTESIAN_POINT ( 'NONE',  ( 152.1327777395850376, 53.61712543276775733, 42.18410997051201861 ) ) ;
#68975=VECTOR ( 'NONE', #12334, 1000.000000000000000 ) ;
#68978=CARTESIAN_POINT ( 'NONE',  ( 107.0477776024379182, 27.43148174916615645, -50.21201981945658588 ) ) ;
#68979=CARTESIAN_POINT ( 'NONE',  ( 135.6647932137617545, 43.70902528961477884, -63.07493546931258521 ) ) ;
#68981=ORIENTED_EDGE ( 'NONE', *, *, #45566, .F. ) ;
#68990=CARTESIAN_POINT ( 'NONE',  ( 136.8102763416569303, 43.23640610422827280, -90.30779350402794137 ) ) ;
#68991=CARTESIAN_POINT ( 'NONE',  ( -156.6692143066620417, 70.50016761530885390, 9.132081936590415339 ) ) ;
#68992=DIRECTION ( 'NONE',  ( -0.8118923937861950435, -0.5838071093367415143, 0.000000000000000000 ) ) ;
#68994=CARTESIAN_POINT ( 'NONE',  ( 65.62848231372478836, 13.29388722724789140, 3.434105544353177830 ) ) ;
#68995=CARTESIAN_POINT ( 'NONE',  ( 164.7167608259061922, 63.51199216609074227, 8.111511345676536422 ) ) ;
#68996=CARTESIAN_POINT ( 'NONE',  ( -7.825402957745087207, -170.0000000000000000, -35.41807073194381417 ) ) ;
#69000=CARTESIAN_POINT ( 'NONE',  ( -60.66790124542881557, 17.30811205907484762, 86.52422518474469371 ) ) ;
#69003=ORIENTED_EDGE ( 'NONE', *, *, #30480, .F. ) ;
#69005=CARTESIAN_POINT ( 'NONE',  ( 23.24047374271773947, 7.861801299833796719, -68.88436191109398976 ) ) ;
#69006=CARTESIAN_POINT ( 'NONE',  ( 116.4569059613810680, 32.98885890446639735, 94.99999999999866418 ) ) ;
#69009=CARTESIAN_POINT ( 'NONE',  ( 136.1037846510192821, 43.98155406734451844, -36.35297218151394105 ) ) ;
#69010=CARTESIAN_POINT ( 'NONE',  ( 210.9029460956748210, 117.0873171135434774, -93.27756825301547394 ) ) ;
#69015=ORIENTED_EDGE ( 'NONE', *, *, #60126, .F. ) ;
#69020=CARTESIAN_POINT ( 'NONE',  ( 66.35539324779723813, 14.50870466687347360, -90.19136351260330287 ) ) ;
#69022=CARTESIAN_POINT ( 'NONE',  ( 183.9887307715836755, 83.05100282186906213, -9.962353762427376580 ) ) ;
#69023=CARTESIAN_POINT ( 'NONE',  ( 173.6710158776851074, 71.42507420636738402, -71.74642395748696799 ) ) ;
#69025=CARTESIAN_POINT ( 'NONE',  ( 87.11228333101212229, 19.58587579906928156, -8.977013608448025650 ) ) ;
#69026=DIRECTION ( 'NONE',  ( -0.000000000000000000, 1.000000000000000000, -0.000000000000000000 ) ) ;
#69029=VERTEX_POINT ( 'NONE', #59411 ) ;
#69030=CARTESIAN_POINT ( 'NONE',  ( -123.6619986853278164, 45.04188181212060016, -35.24979993431918501 ) ) ;
#69034=CARTESIAN_POINT ( 'NONE',  ( 150.9184679586218749, 52.73111408630720831, 13.72417758240726293 ) ) ;
#69035=CARTESIAN_POINT ( 'NONE',  ( -0.6787582498729884950, 7.537756487205481193, 89.00659339660666092 ) ) ;
#69038=ORIENTED_EDGE ( 'NONE', *, *, #59771, .T. ) ;
#69046=CARTESIAN_POINT ( 'NONE',  ( 32.82008564316742394, 8.655929161490991675, 94.71415288098671681 ) ) ;
#69048=CARTESIAN_POINT ( 'NONE',  ( 136.4481901104277597, 44.19676283245976833, -90.17176020796104297 ) ) ;
#69052=CARTESIAN_POINT ( 'NONE',  ( -1.096061481932294690, 7.553048580900439291, 7.450378931708088182 ) ) ;
#69054=CARTESIAN_POINT ( 'NONE',  ( -155.1204242627069902, 70.44799358128196332, -74.13786203925820928 ) ) ;
#69058=CARTESIAN_POINT ( 'NONE',  ( 103.5849290181278803, 27.01613348792538716, -20.03964120650123348 ) ) ;
#69059=DIRECTION ( 'NONE',  ( 0.000000000000000000, 0.000000000000000000, 1.000000000000000000 ) ) ;
#69060=CARTESIAN_POINT ( 'NONE',  ( 8.287863202055540057, 7.382585476140733682, 38.00295202663408389 ) ) ;
#69070=CARTESIAN_POINT ( 'NONE',  ( 201.6034029841261770, 102.1956603101140644, -63.82502672031729674 ) ) ;
#69072=CARTESIAN_POINT ( 'NONE',  ( -10.24974837193994759, 8.069704751038640822, -8.959403934766353217 ) ) ;
#69073=CARTESIAN_POINT ( 'NONE',  ( 150.4544126017351005, 52.39556706174411005, -73.13320268118599188 ) ) ;
#69078=B_SPLINE_CURVE_WITH_KNOTS ( 'NONE', 3,
 ( #6701, #55943, #50655, #44326, #7050, #2475, #44690, #66509, #67208, #40449, #45026, #12680, #39072, #18301, #13042, #35172, #49594, #66170, #17960, #34503, #45731, #40109, #1426, #34842, #18656, #23930, #45380, #66858, #49953, #1789, #34146, #61565, #61894, #13381, #56277, #28147, #8094, #22883, #7415, #51012, #23246, #18997, #39409, #60857, #55581, #67540, #30251, #25326, #3508, #3861, #53669, #26606, #3174, #58599, #46069, #14062, #5146, #64585 ),
 .UNSPECIFIED., .F., .F.,
 ( 4, 2, 2, 2, 2, 2, 2, 2, 2, 2, 2, 2, 2, 2, 2, 2, 2, 2, 2, 2, 2, 2, 2, 2, 2, 2, 2, 2, 4 ),
 ( 0.000000000000000000, 0.002011591002436438277, 0.003017386503654637901, 0.004023182004872837524, 0.005028977506091036713, 0.006034773007309235902, 0.007040568508527436827, 0.008046364009745635149, 0.009052159510963836073, 0.01005795501218203526, 0.01206954601461843364, 0.01307534151583663630, 0.01408113701705483722, 0.01508693251827303815, 0.01609272801949123907, 0.01709852352070944173, 0.01810431902192764092, 0.02011591002436405665, 0.02112170552558225237, 0.02212750102680045156, 0.02313329652801864728, 0.02413909202923684647, 0.02514488753045504565, 0.02615068303167324484, 0.02715647853289144056, 0.02816227403410963975, 0.03017386503654603466, 0.03117966053776423385, 0.03218545603898243651 ),
 .UNSPECIFIED. ) ;
#69079=ORIENTED_EDGE ( 'NONE', *, *, #19048, .T. ) ;
#69080=ADVANCED_FACE ( 'NONE', ( #11929 ), #54830, .F. ) ;
#69081=CARTESIAN_POINT ( 'NONE',  ( 70.51522979775972999, 15.57935281015687146, -15.87393280675930285 ) ) ;
#69083=CARTESIAN_POINT ( 'NONE',  ( -86.10360257264196093, 26.38663017581290404, -41.61327775500715376 ) ) ;
#69084=CARTESIAN_POINT ( 'NONE',  ( 104.0890294065521289, 26.13727058016808513, 86.45864299650676799 ) ) ;
#69085=CARTESIAN_POINT ( 'NONE',  ( -149.9475539515598541, 65.87716206616008208, 18.87627064943539423 ) ) ;
#69088=AXIS2_PLACEMENT_3D ( 'NONE', #14277, #45587, #62462 ) ;
#69090=CARTESIAN_POINT ( 'NONE',  ( 188.2988323915788271, 86.21831227955479449, -41.65539209327070580 ) ) ;
#69100=CARTESIAN_POINT ( 'NONE',  ( 92.30447928123513179, 22.50875695451826530, -92.09038778501471256 ) ) ;
#69102=B_SPLINE_CURVE_WITH_KNOTS ( 'NONE', 3,
 ( #33635, #917, #55064, #22366, #6882, #44524, #39597, #28337, #6183, #65999, #49783, #53061, #10164, #17799, #39255, #60700, #31626, #47793, #69254, #54355, #7599, #18835, #3010, #45562, #46245, #30427, #2318, #67044, #7934, #56824, #40291, #18487, #29733, #29386, #51876, #61734, #24120, #3687, #23768, #8638, #24471, #67382, #45214, #51544 ),
 .UNSPECIFIED., .F., .F.,
 ( 4, 2, 2, 2, 2, 2, 2, 2, 2, 2, 2, 2, 2, 2, 2, 2, 2, 2, 2, 2, 2, 4 ),
 ( 0.02814986980477066775, 0.02995274102020804158, 0.03085417662792674237, 0.03175561223564544316, 0.03355848345108281700, 0.03536135466652019083, 0.03716422588195756466, 0.03896709709739493849, 0.03986853270511362540, 0.04076996831283231232, 0.04167140392055099923, 0.04257283952826968615, 0.04347427513598837306, 0.04437571074370705304, 0.04527714635142573996, 0.04617858195914442687, 0.04798145317458180070, 0.04978432439001917453, 0.05158719560545654836, 0.05339006682089392219, 0.05519293803633129603, 0.05699580925176866986 ),
 .UNSPECIFIED. ) ;
#69104=FACE_OUTER_BOUND ( 'NONE', #66417, .T. ) ;
#69107=CARTESIAN_POINT ( 'NONE',  ( 14.80205238535216949, 6.470775952815779775, -23.62538962562426192 ) ) ;
#69108=CARTESIAN_POINT ( 'NONE',  ( -7.825402957745085430, 7.899365992529248537, -35.41807073194381417 ) ) ;
#69112=CARTESIAN_POINT ( 'NONE',  ( 19.54475376904846939, 6.649964688461122542, 70.85535027690984577 ) ) ;
#69114=CARTESIAN_POINT ( 'NONE',  ( 9.280894575734579988, 7.385644305345134164, 6.909217225878244051 ) ) ;
#69116=ORIENTED_EDGE ( 'NONE', *, *, #22312, .T. ) ;
#69117=CARTESIAN_POINT ( 'NONE',  ( 184.0013086981203969, 81.60415045669147105, 16.88678854673017327 ) ) ;
#69122=CARTESIAN_POINT ( 'NONE',  ( 58.09877917144280701, 12.61383386832654452, -75.74971096422066807 ) ) ;
#69126=CARTESIAN_POINT ( 'NONE',  ( -24.70354720400823112, 8.582324684301857687, -12.63687245714519136 ) ) ;
#69127=CARTESIAN_POINT ( 'NONE',  ( 198.8732368717152212, 100.3103976497391301, 14.59490042447026603 ) ) ;
#69132=CARTESIAN_POINT ( 'NONE',  ( 110.2429982417149432, 28.88204397445228722, 71.45576479620103783 ) ) ;
#69135=CARTESIAN_POINT ( 'NONE',  ( 130.3019683985926349, 39.31883119822051498, 30.38914951925604413 ) ) ;
#69138=CARTESIAN_POINT ( 'NONE',  ( 159.9864727992238329, 59.63397373978884275, -90.23824594202466187 ) ) ;
#69140=VECTOR ( 'NONE', #57732, 1000.000000000000000 ) ;
#69141=CARTESIAN_POINT ( 'NONE',  ( 89.21005684773504640, 20.31770592753387561, -50.36762118906799657 ) ) ;
#69150=CARTESIAN_POINT ( 'NONE',  ( -118.9468627709229054, 42.08677365399180559, -12.73045928823215078 ) ) ;
#69154=CARTESIAN_POINT ( 'NONE',  ( -179.9014775667593256, 95.00669833041662571, -18.58505786628793288 ) ) ;
#69157=CARTESIAN_POINT ( 'NONE',  ( -143.8794621588509131, 59.54894433207191895, -47.27635651071666700 ) ) ;
#69159=CARTESIAN_POINT ( 'NONE',  ( -105.2272522001715203, 35.43984897390651412, 84.78553490936539561 ) ) ;
#69162=CARTESIAN_POINT ( 'NONE',  ( -62.53989795537026453, 16.81768094534200486, -15.36652373032253571 ) ) ;
#69163=CARTESIAN_POINT ( 'NONE',  ( -95.52093927227220149, 30.58993121475389287, 68.12384946097193961 ) ) ;
#69165=CARTESIAN_POINT ( 'NONE',  ( 59.13912479700537261, 11.80663573504270580, -90.47641827390418712 ) ) ;
#69166=CARTESIAN_POINT ( 'NONE',  ( -95.05546640093039912, 29.25972325950978359, 9.094772062743739838 ) ) ;
#69167=CARTESIAN_POINT ( 'NONE',  ( -151.1146011326114262, 65.55487790163387274, -88.67329123693549775 ) ) ;
#69168=EDGE_LOOP ( 'NONE', ( #12832, #44276, #13215, #54951, #892, #15054, #64663, #64044, #32936, #25399, #28140, #9530, #20823, #66372, #49828, #21220, #10082, #46075 ) ) ;
#69171=CARTESIAN_POINT ( 'NONE',  ( -166.5686015187718283, 80.11916873959171426, -38.55272842176326265 ) ) ;
#69174=EDGE_CURVE ( 'NONE', #45231, #35894, #12330, .T. ) ;
#69177=CARTESIAN_POINT ( 'NONE',  ( 79.22946426532585917, 17.02750615740071538, 35.96478783741785890 ) ) ;
#69180=CARTESIAN_POINT ( 'NONE',  ( 41.80869235728137312, 9.750404582811613707, -50.24005329498232442 ) ) ;
#69181=CARTESIAN_POINT ( 'NONE',  ( 209.5118425285947978, 113.1852661712287187, 69.30774190640538279 ) ) ;
#69184=ORIENTED_EDGE ( 'NONE', *, *, #43567, .F. ) ;
#69186=CARTESIAN_POINT ( 'NONE',  ( -14.92903005859421306, 7.458185427130750611, -40.49964561733013113 ) ) ;
#69187=CARTESIAN_POINT ( 'NONE',  ( 86.62931800182293784, 20.48449268398422163, 71.55663816294304524 ) ) ;
#69188=CARTESIAN_POINT ( 'NONE',  ( 93.43270425363546394, 22.93046121381055613, 60.89014534178737392 ) ) ;
#69189=CARTESIAN_POINT ( 'NONE',  ( 155.7262569076171417, 56.30477153194512141, -9.429534158704324653 ) ) ;
#69193=CARTESIAN_POINT ( 'NONE',  ( 37.70762885381311236, 8.195134395012283690, -62.65420549904246172 ) ) ;
#69195=CARTESIAN_POINT ( 'NONE',  ( -34.06637338149494809, 11.05895377318623574, -23.00161039628460458 ) ) ;
#69202=CARTESIAN_POINT ( 'NONE',  ( 13.37708032728285268, 7.441924986912759721, -76.96957816635067218 ) ) ;
#69203=CARTESIAN_POINT ( 'NONE',  ( -189.8071159312682994, 107.8771087123619736, 8.698159761132112422 ) ) ;
#69206=CARTESIAN_POINT ( 'NONE',  ( -7.336760511143403107, 6.859209474528212169, 30.11558103944718923 ) ) ;
#69208=CARTESIAN_POINT ( 'NONE',  ( 151.8005253678161921, 54.62151558044534028, -48.56025122383216086 ) ) ;
#69209=AXIS2_PLACEMENT_3D ( 'NONE', #27400, #21776, #21434 ) ;
#69212=CARTESIAN_POINT ( 'NONE',  ( -189.5329886872043232, 107.4958891766010680, -17.39794636820806417 ) ) ;
#69213=CARTESIAN_POINT ( 'NONE',  ( 179.0091171455097765, 77.94933395983136393, -24.10062151846888412 ) ) ;
#69214=CARTESIAN_POINT ( 'NONE',  ( -107.7677210873466578, 36.80113675102408877, 59.72839805516473888 ) ) ;
#69216=VERTEX_POINT ( 'NONE', #12633 ) ;
#69218=CARTESIAN_POINT ( 'NONE',  ( -0.3747453031323926265, 6.520267647591904137, -17.06192658141792862 ) ) ;
#69220=CARTESIAN_POINT ( 'NONE',  ( -153.7071867110339838, 67.82509357424204666, 85.68967940371055647 ) ) ;
#69222=CARTESIAN_POINT ( 'NONE',  ( 136.3292018078239494, 42.93753790426546146, 29.92580818695415701 ) ) ;
#69225=CARTESIAN_POINT ( 'NONE',  ( 81.76212856587196143, 18.87332718082996763, 4.656136250459809389 ) ) ;
#69226=CARTESIAN_POINT ( 'NONE',  ( 164.6561571795775194, 64.77723933022093661, 12.28447893835758542 ) ) ;
#69228=ORIENTED_EDGE ( 'NONE', *, *, #68145, .F. ) ;
#69230=CARTESIAN_POINT ( 'NONE',  ( 173.7225111622554437, 72.84868911716897344, 65.11675756556223860 ) ) ;
#69233=CARTESIAN_POINT ( 'NONE',  ( -102.2801239173131194, 32.78103895658057354, -35.01457726497591239 ) ) ;
#69239=CYLINDRICAL_SURFACE ( 'NONE', #45516, 7.500000000000013323 ) ;
#69241=CARTESIAN_POINT ( 'NONE',  ( -179.6470915626257465, 94.69856161161348496, 34.61518667817517070 ) ) ;
#69244=CARTESIAN_POINT ( 'NONE',  ( 115.0485321076020284, 32.28990710985444679, -37.64332603850842673 ) ) ;
#69251=CARTESIAN_POINT ( 'NONE',  ( 134.3172730033263633, 41.70277427218489663, 71.35489142945908725 ) ) ;
#69252=CARTESIAN_POINT ( 'NONE',  ( -166.9969673948021409, 80.56076768517783648, 42.65932412964239973 ) ) ;
#69253=CARTESIAN_POINT ( 'NONE',  ( 127.4992165631961285, 38.87141012667725448, 59.84453210894926656 ) ) ;
#69254=CARTESIAN_POINT ( 'NONE',  ( 188.2950202724320832, 86.21411212788221690, -18.96334599335139259 ) ) ;
#69257=CARTESIAN_POINT ( 'NONE',  ( -8.320534640989473374, 7.931748412542462212, 71.96013162991094703 ) ) ;
#69259=VERTEX_POINT ( 'NONE', #14015 ) ;
#69262=CARTESIAN_POINT ( 'NONE',  ( -62.48811917300399443, 16.80201428380103934, 92.54160460740271787 ) ) ;
#69265=CARTESIAN_POINT ( 'NONE',  ( -109.4660948262506537, 36.58364455021701644, 89.53602648964154298 ) ) ;
#69267=CARTESIAN_POINT ( 'NONE',  ( 187.2384682876462136, 86.54721710842893856, 14.27990392942774633 ) ) ;
#69269=B_SPLINE_CURVE_WITH_KNOTS ( 'NONE', 3,
 ( #16617, #27515, #64463, #53549, #798, #37045, #22250, #53890, #5381, #16275, #65163, #16956, #26836, #31768, #59870, #69034, #21545, #53198, #11686, #5026, #52856, #4682, #26147, #47579, #42992, #26492, #47927, #69398, #21217, #42662, #64119, #15930, #37376, #58833, #18363, #28930, #45439, #44035, #66231, #33852, #33517, #54945, #6763, #55643, #7480, #50716, #23647 ),
 .UNSPECIFIED., .F., .F.,
 ( 4, 2, 2, 2, 2, 2, 2, 2, 2, 2, 2, 1, 2, 2, 2, 2, 2, 2, 2, 2, 2, 2, 2, 4 ),
 ( 0.000000000000000000, 0.003297771944418890870, 0.004122214930523575641, 0.004946657916628260411, 0.006595543888837629085, 0.007419986874942339876, 0.008244429861047052402, 0.009068872847151762326, 0.009893315833256473985, 0.01154220180546592679, 0.01236664479157065580, 0.01319108777767538133, 0.01401553076378011034, 0.01483997374988483761, 0.01566441673598956835, 0.01648885972209429562, 0.01813774569430378139, 0.01896218868040854336, 0.01978663166651330532, 0.02061107465261806729, 0.02143551763872282578, 0.02308440361093234625, 0.02473328958314187018, 0.02638217555535139064 ),
 .UNSPECIFIED. ) ;
#69272=CARTESIAN_POINT ( 'NONE',  ( -97.21566814336060247, 31.39773419228200524, -90.65435922756391562 ) ) ;
#69274=CARTESIAN_POINT ( 'NONE',  ( -71.27103490383373696, 20.70545763375147530, 66.03643395433377350 ) ) ;
#69276=CARTESIAN_POINT ( 'NONE',  ( 62.53328835682431475, 12.56090025569836754, -77.56524142263340593 ) ) ;
#69277=CARTESIAN_POINT ( 'NONE',  ( -77.72491324796696688, 21.96482567905608008, 3.617778172024071370 ) ) ;
#69278=CARTESIAN_POINT ( 'NONE',  ( -120.6739978760425913, 44.33795494230366785, 70.35544155365153074 ) ) ;
#69279=CARTESIAN_POINT ( 'NONE',  ( -55.05276343752910151, 14.68156374112636620, 3.472777182467474244 ) ) ;
#69280=CARTESIAN_POINT ( 'NONE',  ( 197.2510943223972504, 96.65903929707269526, 89.47520902944462762 ) ) ;
#69281=CARTESIAN_POINT ( 'NONE',  ( 164.6598737201887559, 64.78038692612514637, -72.67496918674851258 ) ) ;
#69282=ORIENTED_EDGE ( 'NONE', *, *, #53288, .F. ) ;
#69283=CARTESIAN_POINT ( 'NONE',  ( -71.26675986148644881, 19.63956187826082811, 66.01101777128145898 ) ) ;
#69287=CARTESIAN_POINT ( 'NONE',  ( -156.7487895666417046, 70.57327586518567841, 36.24776524068245465 ) ) ;
#69288=CARTESIAN_POINT ( 'NONE',  ( 59.29597493004737174, 11.84030339376940510, -36.68987112816819973 ) ) ;
#69296=CARTESIAN_POINT ( 'NONE',  ( -133.2787743207940991, 52.78950725740543959, 39.45582838502271272 ) ) ;
#69301=CARTESIAN_POINT ( 'NONE',  ( 207.8675797643809631, 110.7908513421272119, 43.51807350428817500 ) ) ;
#69303=CYLINDRICAL_SURFACE ( 'NONE', #274, 7.500000000000013323 ) ;
#69307=VECTOR ( 'NONE', #67380, 1000.000000000000000 ) ;
#69313=CARTESIAN_POINT ( 'NONE',  ( -165.6212796729685124, 79.15047440262053158, -15.67432408031424806 ) ) ;
#69314=CARTESIAN_POINT ( 'NONE',  ( 133.8566784816069060, 41.42467568809810530, -77.86786152285937135 ) ) ;
#69316=CARTESIAN_POINT ( 'NONE',  ( -189.9638655956219679, 108.0957249433520246, -72.18686446978868787 ) ) ;
#69320=CARTESIAN_POINT ( 'NONE',  ( -99.31850058233797540, 31.30166762705807670, 71.75812556856945434 ) ) ;
#69322=DIRECTION ( 'NONE',  ( -0.000000000000000000, 1.000000000000000000, -0.000000000000000000 ) ) ;
#69326=B_SPLINE_CURVE_WITH_KNOTS ( 'NONE', 3,
 ( #8048, #23546, #18256, #61518, #29161, #56232, #30208, #7713, #3466, #14018, #9095, #45688, #56939, #67165, #40745, #46025, #29852, #50963, #39715, #35126, #51319, #45332, #61170, #57282, #2775, #41102, #13337, #35478, #62561, #55895, #12995, #56582, #18954, #2429, #40400, #61846, #51658, #35829, #67492, #30544, #24927, #46360, #23886, #67842 ),
 .UNSPECIFIED., .F., .F.,
 ( 4, 2, 2, 2, 2, 2, 2, 2, 2, 2, 2, 2, 1, 2, 2, 2, 2, 2, 2, 1, 2, 2, 4 ),
 ( 0.02381751147647563627, 0.02531129726520768564, 0.02605819015957370685, 0.02680508305393972807, 0.02829886884267176356, 0.02979265463140379558, 0.03053954752576982720, 0.03128644042013585536, 0.03278022620886791860, 0.03427401199759996103, 0.03576779778633200346, 0.03651469068069800039, 0.03726158357506400426, 0.03800847646943000119, 0.03875536936379600506, 0.04024915515252804055, 0.04174294094126008298, 0.04323672672999212541, 0.04398361962435815009, 0.04473051251872417478, 0.04547740541309019946, 0.04622429830745622414, 0.04771808409618829433 ),
 .UNSPECIFIED. ) ;
#69328=CARTESIAN_POINT ( 'NONE',  ( -118.8691191306315034, 43.21907118237573542, 13.91607852633928566 ) ) ;
#69329=CARTESIAN_POINT ( 'NONE',  ( -177.1539090641757355, 91.73101548694627638, 71.50528903873359354 ) ) ;
#69330=CARTESIAN_POINT ( 'NONE',  ( 16.28371206594635368, 6.516665886438622657, 18.17015708224157322 ) ) ;
#69334=CIRCLE ( 'NONE', #61524, 242.4895526022646379 ) ;
#69335=CARTESIAN_POINT ( 'NONE',  ( 154.6667526376336923, 55.50347409140649546, 43.86940883944475189 ) ) ;
#69337=CYLINDRICAL_SURFACE ( 'NONE', #32759, 7.500000000000020428 ) ;
#69338=CARTESIAN_POINT ( 'NONE',  ( -24.19091603582231542, 8.513464105188679909, 39.65939032213886861 ) ) ;
#69342=FACE_BOUND ( 'NONE', #21452, .T. ) ;
#69343=AXIS2_PLACEMENT_3D ( 'NONE', #49066, #38530, #44140 ) ;
#69346=CARTESIAN_POINT ( 'NONE',  ( 117.1658080721356470, 32.21846976819855257, -94.19636932247044570 ) ) ;
#69347=CARTESIAN_POINT ( 'NONE',  ( -119.2804658695888378, 43.47213805166353495, -45.96062334567895391 ) ) ;
#69351=ADVANCED_FACE ( 'NONE', ( #57962 ), #10116, .F. ) ;
#69352=CARTESIAN_POINT ( 'NONE',  ( -154.0775378574014383, 68.15437918458555089, 17.34221547010214692 ) ) ;
#69353=CARTESIAN_POINT ( 'NONE',  ( -125.8938041572051389, 47.69968343338780414, -61.75825448869760237 ) ) ;
#69354=CARTESIAN_POINT ( 'NONE',  ( 67.92995549349548412, 13.86623459444478534, 4.781840506428621573 ) ) ;
#69356=CARTESIAN_POINT ( 'NONE',  ( 88.52077179907882964, 21.14145351760141267, -9.215479869664170209 ) ) ;
#69357=ORIENTED_EDGE ( 'NONE', *, *, #24669, .F. ) ;
#69362=CARTESIAN_POINT ( 'NONE',  ( 110.2429982417149574, 29.99119854320843714, -9.077886975189997543 ) ) ;
#69364=CARTESIAN_POINT ( 'NONE',  ( -142.5042386072304055, 59.74110826975218203, 62.32831377680863483 ) ) ;
#69365=CARTESIAN_POINT ( 'NONE',  ( 8.000000000000007105, 249.8719672152120381, -95.00000000000133582 ) ) ;
#69367=CARTESIAN_POINT ( 'NONE',  ( 208.9325386374517279, 114.1236747564815772, -91.31446213177319748 ) ) ;
#69371=VERTEX_POINT ( 'NONE', #31574 ) ;
#69372=CARTESIAN_POINT ( 'NONE',  ( 70.02892116572942882, 14.40944430928136732, -40.55127576682969703 ) ) ;
#69373=CARTESIAN_POINT ( 'NONE',  ( 181.8106359728740529, 80.78261033454286633, 83.02753339407779265 ) ) ;
#69377=EDGE_CURVE ( 'NONE', #19968, #6351, #9849, .T. ) ;
#69379=CARTESIAN_POINT ( 'NONE',  ( 181.0840389613909736, 80.03940679743416808, -24.38050707541595230 ) ) ;
#69380=CARTESIAN_POINT ( 'NONE',  ( -85.90441187606242579, 25.21188850826091254, -13.74108820849124335 ) ) ;
#69384=CARTESIAN_POINT ( 'NONE',  ( 42.03492317486908547, 8.766487167902370814, -23.30212316240421444 ) ) ;
#69385=LINE ( 'NONE', #32105, #43223 ) ;
#69391=ORIENTED_EDGE ( 'NONE', *, *, #46065, .F. ) ;
#69394=CARTESIAN_POINT ( 'NONE',  ( 87.11239765416378589, 20.65008247340817249, -35.82156419891170884 ) ) ;
#69398=CARTESIAN_POINT ( 'NONE',  ( 150.2809931605061990, 52.27058242113234598, 7.911800210953336077 ) ) ;
#69399=CARTESIAN_POINT ( 'NONE',  ( -14.46498759803290746, 8.425214076810821240, 87.80158803776117793 ) ) ;
#69407=CARTESIAN_POINT ( 'NONE',  ( 45.20784367118678659, 10.25355619695782927, 86.30875473536740117 ) ) ;
#69412=CARTESIAN_POINT ( 'NONE',  ( 67.54641595172914492, 14.80690682047551121, 70.15402874321907234 ) ) ;
#69414=CARTESIAN_POINT ( 'NONE',  ( 37.47081272996201307, 8.166145978397521432, -9.024001403194343851 ) ) ;
#69415=CARTESIAN_POINT ( 'NONE',  ( 160.2883311361769358, 61.16711613734477027, 43.86358491700874396 ) ) ;
#69416=CARTESIAN_POINT ( 'NONE',  ( 163.9335029509016692, 62.85601444701051577, 94.42016238087119007 ) ) ;
#69417=CARTESIAN_POINT ( 'NONE',  ( 88.28780346671267409, 19.99350429399659745, 29.89382215203381676 ) ) ;
#69418=EDGE_LOOP ( 'NONE', ( #50154, #35827 ) ) ;
#69419=CARTESIAN_POINT ( 'NONE',  ( 105.4376736768159049, 27.81988511842610023, -22.34144044879345969 ) ) ;
#69420=DIRECTION ( 'NONE',  ( -0.000000000000000000, 1.000000000000000000, -0.000000000000000000 ) ) ;
#69421=CARTESIAN_POINT ( 'NONE',  ( -30.95341298663138119, 10.53108683215057084, 30.21645440618916112 ) ) ;
#69422=CARTESIAN_POINT ( 'NONE',  ( 197.5344433744249102, 98.61756151884685551, 38.95244195491510908 ) ) ;
#69430=CARTESIAN_POINT ( 'NONE',  ( -55.05276343752908730, 15.72344139423348430, 72.16187836339486239 ) ) ;
#69431=CARTESIAN_POINT ( 'NONE',  ( -35.99414836699283882, 11.40630460607619945, 58.58236999211133877 ) ) ;
#69433=CARTESIAN_POINT ( 'NONE',  ( 150.8925291903903201, 52.71218673668931842, -74.11121607790209964 ) ) ;
#69434=DIRECTION ( 'NONE',  ( -0.000000000000000000, 1.000000000000000000, -0.000000000000000000 ) ) ;
#69439=CARTESIAN_POINT ( 'NONE',  ( 66.30636076182547356, 14.49616748423541068, -9.619026385704664506 ) ) ;
#69441=CARTESIAN_POINT ( 'NONE',  ( 104.5164129159900170, 26.32100697179284765, 85.91093688393655725 ) ) ;
#69442=CARTESIAN_POINT ( 'NONE',  ( -156.8773151811562911, 72.06122063279302381, 12.79581229564695022 ) ) ;
#69451=CARTESIAN_POINT ( 'NONE',  ( -155.1359377029286009, 70.46175948311802983, -10.48588441764089474 ) ) ;
#69452=CARTESIAN_POINT ( 'NONE',  ( 33.44035656425387515, 8.720466003183664938, -38.54271289854762017 ) ) ;
#69453=CARTESIAN_POINT ( 'NONE',  ( -37.38781680082738745, 10.64362327909142714, 59.96723102333222499 ) ) ;
#69454=CARTESIAN_POINT ( 'NONE',  ( 204.3129818922372749, 107.5244029525888863, 56.05227132923313604 ) ) ;
#69457=CARTESIAN_POINT ( 'NONE',  ( -156.4960819023051215, 70.34114605623869920, 67.83986282103712995 ) ) ;
#69459=CARTESIAN_POINT ( 'NONE',  ( -6.843910203392213454, 7.836697961436720483, -35.46655999132715209 ) ) ;
#69460=CARTESIAN_POINT ( 'NONE',  ( 187.5325688887159004, 85.37769363979911930, 67.52131414333028658 ) ) ;
#69462=CARTESIAN_POINT ( 'NONE',  ( -86.09999398724994535, 25.29376521564874380, -41.58702898857048069 ) ) ;
#69464=CARTESIAN_POINT ( 'NONE',  ( 63.01563776193090405, 13.70579113808097382, -62.56524142263340593 ) ) ;
#69465=CARTESIAN_POINT ( 'NONE',  ( 13.37820144534469158, 6.435512790162279728, -62.75700969552578101 ) ) ;
#69471=CARTESIAN_POINT ( 'NONE',  ( 173.6710158776851358, 71.42507420636738402, 35.63177840436776478 ) ) ;
#69472=CARTESIAN_POINT ( 'NONE',  ( -128.1384526288949814, 47.98891607499718504, -49.58460275042809684 ) ) ;
#69473=CARTESIAN_POINT ( 'NONE',  ( 39.88971011078922402, 8.472992116645418292, -77.46436805589146957 ) ) ;
#69474=CARTESIAN_POINT ( 'NONE',  ( 63.01563776193091826, 13.70579113808094718, -77.56524142263344856 ) ) ;
#69477=CARTESIAN_POINT ( 'NONE',  ( -24.93568128341082968, 8.613819379861704206, -12.20478168535062835 ) ) ;
#69478=CARTESIAN_POINT ( 'NONE',  ( 174.4960269704457119, 72.19444789407123153, 86.89327852742059122 ) ) ;
#69480=CARTESIAN_POINT ( 'NONE',  ( 117.4830770399668012, 32.37795270233551292, 65.97967136513133823 ) ) ;
#69483=CARTESIAN_POINT ( 'NONE',  ( 128.3889472838589256, 39.37765603157609462, -65.21099523326392955 ) ) ;
#69484=CARTESIAN_POINT ( 'NONE',  ( -190.6985136298601731, 109.1272424661242582, -95.00000000000133582 ) ) ;
#69486=DIRECTION ( 'NONE',  ( -0.000000000000000000, 1.000000000000000000, -0.000000000000000000 ) ) ;
#69487=CARTESIAN_POINT ( 'NONE',  ( 85.83240444548572157, 19.15035268578635907, -89.54263933694141997 ) ) ;
#69493=CARTESIAN_POINT ( 'NONE',  ( -120.4586945679390482, 43.01762219615311977, -10.37801267066958388 ) ) ;
#69495=CARTESIAN_POINT ( 'NONE',  ( -173.1211646369891071, 87.12891641440859303, -22.86740657428632773 ) ) ;
#69496=CARTESIAN_POINT ( 'NONE',  ( -173.1211646369891071, 88.63826465341152527, -61.55650775521367279 ) ) ;
#69497=CARTESIAN_POINT ( 'NONE',  ( -144.9439644317224065, 60.40328483334192100, -48.26935030906360424 ) ) ;
#69503=CARTESIAN_POINT ( 'NONE',  ( 79.93126905972559371, 17.24332478304278382, -19.86064041717387241 ) ) ;
#69504=CARTESIAN_POINT ( 'NONE',  ( -131.6399667378751701, 51.62465701391632678, -64.41211764283146124 ) ) ;
#69505=CARTESIAN_POINT ( 'NONE',  ( 59.67833965117457495, 11.92331751763832237, -90.19013027095671475 ) ) ;
#69507=CARTESIAN_POINT ( 'NONE',  ( -95.52163045714284806, 29.47808868198297105, -72.62058247320986482 ) ) ;
#69510=CARTESIAN_POINT ( 'NONE',  ( 183.9986899696430953, 81.60141257362811018, -77.49343821721251402 ) ) ;
#69514=CARTESIAN_POINT ( 'NONE',  ( 110.2429982417149574, 29.99119854320845846, -77.76698815611739235 ) ) ;
#69515=CARTESIAN_POINT ( 'NONE',  ( -71.15374617000811952, 20.66492714610676273, 37.92836382045980770 ) ) ;
#69516=EDGE_CURVE ( 'NONE', #45282, #29497, #29748, .T. ) ;
#69519=CARTESIAN_POINT ( 'NONE',  ( 46.80475532923158255, 10.50744084852537163, -44.34838384464438832 ) ) ;
#69522=CARTESIAN_POINT ( 'NONE',  ( -102.7502407665687372, 33.01985383847078026, -8.170026674512229192 ) ) ;
#69523=B_SPLINE_CURVE_WITH_KNOTS ( 'NONE', 3,
 ( #49022, #69454, #21274, #26210, #47647, #15312, #862, #42384, #42039, #42721, #63499, #58894, #64178, #53948, #10710, #37795, #36773, #53614, #10033, #48321, #31488, #52921, #32518, #4746, #49378, #1208, #12460, #1924, #65226, #13163, #7184, #29331, #50095, #29002, #50445, #17746, #66302, #23382, #38490, #44821, #34272, #18089, #11751, #22315, #23712, #55719, #39884, #7543, #44468, #65949 ),
 .UNSPECIFIED., .F., .F.,
 ( 4, 2, 2, 2, 2, 2, 2, 2, 2, 2, 2, 2, 2, 2, 2, 2, 2, 2, 2, 2, 2, 2, 2, 2, 4 ),
 ( 0.03296461860586798881, 0.03492857779726591533, 0.03689253698866384878, 0.03885649618006177530, 0.04082045537145970182, 0.04278441456285763528, 0.04376639415855656384, 0.04474837375425549241, 0.04573035334995442097, 0.04671233294565334954, 0.04720332274350281382, 0.04769431254135228504, 0.04867629213705121360, 0.04965827173275014217, 0.05064025132844907073, 0.05162223092414799930, 0.05260421051984692786, 0.05358619011554585643, 0.05456816971124478499, 0.05555014930694372050, 0.05653212890264264906, 0.05849608809404049925, 0.06046004728543834250, 0.06242400647683619269, 0.06438796566823404288 ),
 .UNSPECIFIED. ) ;
#69524=ORIENTED_EDGE ( 'NONE', *, *, #21752, .F. ) ;
#69526=CARTESIAN_POINT ( 'NONE',  ( -14.19493007850031141, 7.389842975086041044, -46.88529827066894029 ) ) ;
#69527=CYLINDRICAL_SURFACE ( 'NONE', #29585, 7.500000000000013323 ) ;
#69528=CARTESIAN_POINT ( 'NONE',  ( 94.02861641584118502, 23.15570573563316614, 62.80575613031886917 ) ) ;
#69529=CARTESIAN_POINT ( 'NONE',  ( 154.6667526376337491, 55.50347409140650257, -9.819692341482584297 ) ) ;
#69530=CARTESIAN_POINT ( 'NONE',  ( 38.42095780754792855, 9.297684251045552628, 18.02115975282741189 ) ) ;
#69538=CARTESIAN_POINT ( 'NONE',  ( 57.09527843067915143, 12.40436368789087318, 59.54664166497151712 ) ) ;
#69543=CARTESIAN_POINT ( 'NONE',  ( -61.90200967450776659, 16.62550425046104863, -93.31852439468944738 ) ) ;
#69544=CARTESIAN_POINT ( 'NONE',  ( -96.00016893459647349, 29.70347032303887147, -11.56214555964269941 ) ) ;
#69545=EDGE_CURVE ( 'NONE', #14540, #59876, #64270, .T. ) ;
#69546=CARTESIAN_POINT ( 'NONE',  ( 79.43281949162772548, 18.14250680856633480, 88.76187498690042332 ) ) ;
#69551=DIRECTION ( 'NONE',  ( -0.000000000000000000, 1.000000000000000000, -0.000000000000000000 ) ) ;
#69552=CARTESIAN_POINT ( 'NONE',  ( -132.4819073909166036, 50.98736898418874119, 14.89792975520157547 ) ) ;
#69553=CARTESIAN_POINT ( 'NONE',  ( -106.4728934171454284, 36.10295170132725673, 58.64049600876298740 ) ) ;
#69555=CARTESIAN_POINT ( 'NONE',  ( -180.1361238728360377, 95.29182030496930622, 94.68613861460413261 ) ) ;
#69557=LINE ( 'NONE', #47756, #55998 ) ;
#69558=CARTESIAN_POINT ( 'NONE',  ( 94.12988949694079110, 22.11811104795075522, 64.29232835590543971 ) ) ;
#69559=CARTESIAN_POINT ( 'NONE',  ( -156.8975660802013010, 70.71010336351562842, 90.58301405942083306 ) ) ;
#69562=VERTEX_POINT ( 'NONE', #1643 ) ;
#69563=CYLINDRICAL_SURFACE ( 'NONE', #53652, 7.500000000000013323 ) ;
ENDSEC;
END-ISO-10303-21;
